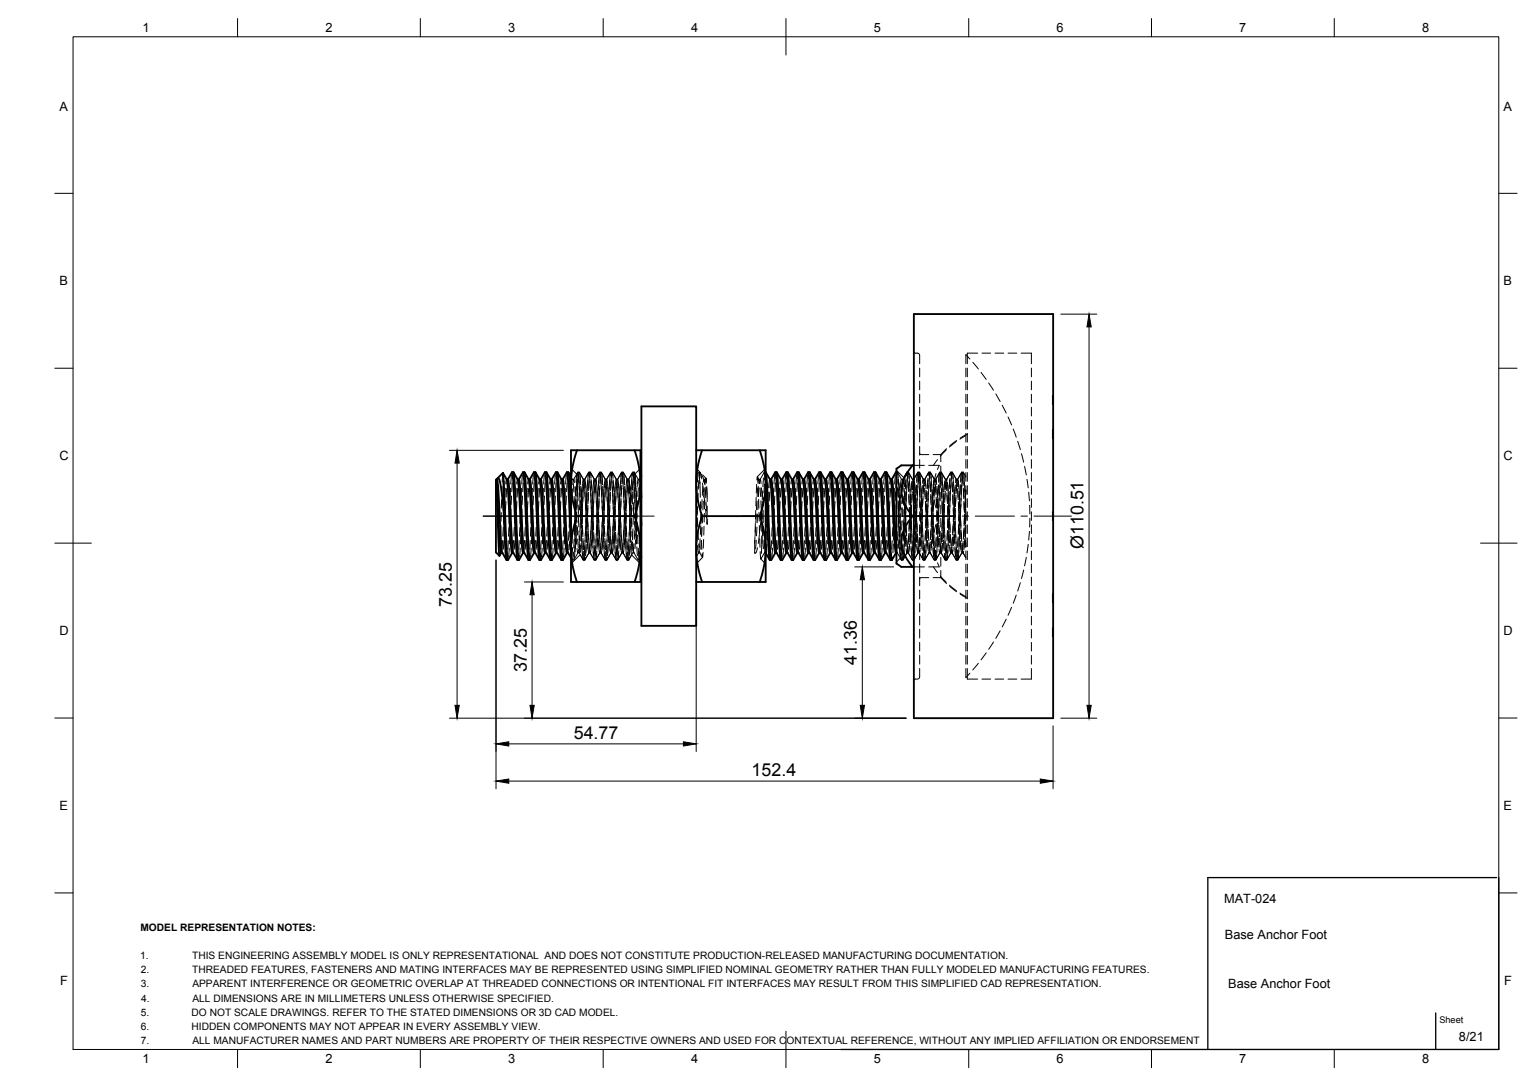
ISO-10303-21;
HEADER;
/* Generated by software containing ST-Developer
 * from STEP Tools, Inc. (www.steptools.com) 
 */

FILE_DESCRIPTION(
/* description */ ('STEP AP214'),
/* implementation_level */ '2;1');

FILE_NAME(
/* name */ 'Base Anchor Foot.step',
/* time_stamp */ '2026-11-14T06:34:07-08:00',
/* author */ (''),
/* organization */ (''),
/* preprocessor_version */ 'ST-DEVELOPER v20.2',
/* originating_system */ 'Autodesk Translation Framework v15.17.0.0',
/* authorisation */ '');

FILE_SCHEMA (('AUTOMOTIVE_DESIGN { 1 0 10303 214 3 1 1 }'));
ENDSEC;

DATA;
#10=MECHANICAL_DESIGN_GEOMETRIC_PRESENTATION_REPRESENTATION('',(#7314,#7315,#7316,#7317),#310623);
#11=ORIENTED_CLOSED_SHELL('',*,#93766,.F.);
#12=BREP_WITH_VOIDS('Body3',#93767,(#11));
#1065=SPHERICAL_SURFACE('',#104324,64.4688722290585);
#1066=SPHERICAL_SURFACE('',#104326,25.0876428025235);
#1067=SPHERICAL_SURFACE('',#104511,25.2860803025235);
#1539=(
BOUNDED_CURVE()
B_SPLINE_CURVE(2,(#275566,#275567,#275568),.UNSPECIFIED.,.F.,.F.)
B_SPLINE_CURVE_WITH_KNOTS((3,3),(0.701923076923077,0.701927534605613),
 .UNSPECIFIED.)
CURVE()
GEOMETRIC_REPRESENTATION_ITEM()
RATIONAL_B_SPLINE_CURVE((1.,0.99988654925346,0.999773624463427))
REPRESENTATION_ITEM('')
);
#1540=(
BOUNDED_CURVE()
B_SPLINE_CURVE(2,(#275574,#275575,#275576,#275577,#275578,#275579,#275580,
#275581,#275582,#275583,#275584,#275585,#275586,#275587,#275588,#275589,
#275590,#275591,#275592),.UNSPECIFIED.,.F.,.F.)
B_SPLINE_CURVE_WITH_KNOTS((3,2,2,2,2,2,2,2,2,3),(0.682692307692308,0.684615384615385,
0.686538461538462,0.688461538461538,0.690384615384615,0.692307692307692,
0.694230769230769,0.696153846153846,0.698076923076923,0.699514511997895),
 .UNSPECIFIED.)
CURVE()
GEOMETRIC_REPRESENTATION_ITEM()
RATIONAL_B_SPLINE_CURVE((1.,0.951056516295154,1.,0.951056516295154,1.,0.951056516295154,
1.,0.951056516295154,1.,0.951056516295154,1.,0.951056516295154,1.,0.951056516295154,
1.,0.951056516295154,1.,0.963412482837523,0.981526687366426))
REPRESENTATION_ITEM('')
);
#1541=(
BOUNDED_CURVE()
B_SPLINE_CURVE(2,(#275594,#275595,#275596,#275597,#275598,#275599,#275600,
#275601,#275602,#275603,#275604,#275605,#275606,#275607,#275608,#275609,
#275610,#275611,#275612,#275613,#275614),.UNSPECIFIED.,.F.,.F.)
B_SPLINE_CURVE_WITH_KNOTS((3,2,2,2,2,2,2,2,2,2,3),(0.682692307692308,0.684615384615385,
0.686538461538462,0.688461538461538,0.690384615384615,0.692307692307692,
0.694230769230769,0.696153846153846,0.698076923076923,0.7,0.701923076923077),
 .UNSPECIFIED.)
CURVE()
GEOMETRIC_REPRESENTATION_ITEM()
RATIONAL_B_SPLINE_CURVE((1.,0.951056516295154,1.,0.951056516295154,1.,0.951056516295154,
1.,0.951056516295154,1.,0.951056516295154,1.,0.951056516295154,1.,0.951056516295154,
1.,0.951056516295154,1.,0.951056516295154,1.,0.951056516295154,1.))
REPRESENTATION_ITEM('')
);
#1542=(
BOUNDED_CURVE()
B_SPLINE_CURVE(2,(#275619,#275620,#275621,#275622,#275623,#275624,#275625,
#275626,#275627,#275628,#275629,#275630,#275631,#275632,#275633,#275634,
#275635,#275636,#275637,#275638,#275639),.UNSPECIFIED.,.F.,.F.)
B_SPLINE_CURVE_WITH_KNOTS((3,2,2,2,2,2,2,2,2,2,3),(0.663461538461538,0.665384615384615,
0.667307692307692,0.669230769230769,0.671153846153846,0.673076923076923,
0.675,0.676923076923077,0.678846153846154,0.680769230769231,0.682692307692308),
 .UNSPECIFIED.)
CURVE()
GEOMETRIC_REPRESENTATION_ITEM()
RATIONAL_B_SPLINE_CURVE((1.,0.951056516295154,1.,0.951056516295154,1.,0.951056516295154,
1.,0.951056516295154,1.,0.951056516295154,1.,0.951056516295154,1.,0.951056516295154,
1.,0.951056516295154,1.,0.951056516295154,1.,0.951056516295154,1.))
REPRESENTATION_ITEM('')
);
#1543=(
BOUNDED_CURVE()
B_SPLINE_CURVE(2,(#275640,#275641,#275642,#275643,#275644,#275645,#275646,
#275647,#275648,#275649,#275650,#275651,#275652,#275653,#275654,#275655,
#275656,#275657,#275658,#275659,#275660),.UNSPECIFIED.,.F.,.F.)
B_SPLINE_CURVE_WITH_KNOTS((3,2,2,2,2,2,2,2,2,2,3),(0.663461538461538,0.665384615384615,
0.667307692307692,0.669230769230769,0.671153846153846,0.673076923076923,
0.675,0.676923076923077,0.678846153846154,0.680769230769231,0.682692307692308),
 .UNSPECIFIED.)
CURVE()
GEOMETRIC_REPRESENTATION_ITEM()
RATIONAL_B_SPLINE_CURVE((1.,0.951056516295154,1.,0.951056516295154,1.,0.951056516295154,
1.,0.951056516295154,1.,0.951056516295154,1.,0.951056516295154,1.,0.951056516295154,
1.,0.951056516295154,1.,0.951056516295154,1.,0.951056516295154,1.))
REPRESENTATION_ITEM('')
);
#1544=(
BOUNDED_CURVE()
B_SPLINE_CURVE(2,(#275665,#275666,#275667,#275668,#275669,#275670,#275671,
#275672,#275673,#275674,#275675,#275676,#275677,#275678,#275679,#275680,
#275681,#275682,#275683,#275684,#275685),.UNSPECIFIED.,.F.,.F.)
B_SPLINE_CURVE_WITH_KNOTS((3,2,2,2,2,2,2,2,2,2,3),(0.644230769230769,0.646153846153846,
0.648076923076923,0.65,0.651923076923077,0.653846153846154,0.655769230769231,
0.657692307692308,0.659615384615385,0.661538461538462,0.663461538461538),
 .UNSPECIFIED.)
CURVE()
GEOMETRIC_REPRESENTATION_ITEM()
RATIONAL_B_SPLINE_CURVE((1.,0.951056516295154,1.,0.951056516295154,1.,0.951056516295154,
1.,0.951056516295154,1.,0.951056516295154,1.,0.951056516295154,1.,0.951056516295154,
1.,0.951056516295154,1.,0.951056516295154,1.,0.951056516295154,1.))
REPRESENTATION_ITEM('')
);
#1545=(
BOUNDED_CURVE()
B_SPLINE_CURVE(2,(#275686,#275687,#275688,#275689,#275690,#275691,#275692,
#275693,#275694,#275695,#275696,#275697,#275698,#275699,#275700,#275701,
#275702,#275703,#275704,#275705,#275706),.UNSPECIFIED.,.F.,.F.)
B_SPLINE_CURVE_WITH_KNOTS((3,2,2,2,2,2,2,2,2,2,3),(0.644230769230769,0.646153846153846,
0.648076923076923,0.65,0.651923076923077,0.653846153846154,0.655769230769231,
0.657692307692308,0.659615384615385,0.661538461538462,0.663461538461538),
 .UNSPECIFIED.)
CURVE()
GEOMETRIC_REPRESENTATION_ITEM()
RATIONAL_B_SPLINE_CURVE((1.,0.951056516295154,1.,0.951056516295154,1.,0.951056516295154,
1.,0.951056516295154,1.,0.951056516295154,1.,0.951056516295154,1.,0.951056516295154,
1.,0.951056516295154,1.,0.951056516295154,1.,0.951056516295154,1.))
REPRESENTATION_ITEM('')
);
#1546=(
BOUNDED_CURVE()
B_SPLINE_CURVE(2,(#275712,#275713,#275714,#275715,#275716,#275717,#275718,
#275719,#275720),.UNSPECIFIED.,.F.,.F.)
B_SPLINE_CURVE_WITH_KNOTS((3,2,2,2,3),(0.618568719050757,0.619230769230769,
0.621153846153846,0.623076923076923,0.625),.UNSPECIFIED.)
CURVE()
GEOMETRIC_REPRESENTATION_ITEM()
RATIONAL_B_SPLINE_CURVE((0.977902315623412,0.983150418057436,1.,0.951056516295154,
1.,0.951056516295154,1.,0.951056516295154,1.))
REPRESENTATION_ITEM('')
);
#1547=(
BOUNDED_CURVE()
B_SPLINE_CURVE(2,(#275723,#275724,#275725,#275726,#275727,#275728,#275729,
#275730,#275731,#275732,#275733),.UNSPECIFIED.,.F.,.F.)
B_SPLINE_CURVE_WITH_KNOTS((3,2,2,2,2,3),(0.616175777003085,0.617307692307692,
0.619230769230769,0.621153846153846,0.623076923076923,0.625),
 .UNSPECIFIED.)
CURVE()
GEOMETRIC_REPRESENTATION_ITEM()
RATIONAL_B_SPLINE_CURVE((0.976296596823935,0.971192063301508,1.,0.951056516295154,
1.,0.951056516295154,1.,0.951056516295154,1.,0.951056516295154,1.))
REPRESENTATION_ITEM('')
);
#1548=(
BOUNDED_CURVE()
B_SPLINE_CURVE(2,(#276333,#276334,#276335),.UNSPECIFIED.,.F.,.F.)
B_SPLINE_CURVE_WITH_KNOTS((3,3),(-7.37746868484566,-5.33580039117808),
 .UNSPECIFIED.)
CURVE()
GEOMETRIC_REPRESENTATION_ITEM()
RATIONAL_B_SPLINE_CURVE((1.82136720504436,1.96225044864938,1.96225044864938))
REPRESENTATION_ITEM('')
);
#1549=(
BOUNDED_CURVE()
B_SPLINE_CURVE(2,(#276339,#276340,#276341),.UNSPECIFIED.,.F.,.F.)
B_SPLINE_CURVE_WITH_KNOTS((3,3),(3.29413209751051,5.33580039117807),
 .UNSPECIFIED.)
CURVE()
GEOMETRIC_REPRESENTATION_ITEM()
RATIONAL_B_SPLINE_CURVE((1.82136720504436,1.96225044864938,1.96225044864938))
REPRESENTATION_ITEM('')
);
#1550=(
BOUNDED_CURVE()
B_SPLINE_CURVE(2,(#276343,#276344,#276345),.UNSPECIFIED.,.F.,.F.)
B_SPLINE_CURVE_WITH_KNOTS((3,3),(5.33580039117807,7.37746868484567),
 .UNSPECIFIED.)
CURVE()
GEOMETRIC_REPRESENTATION_ITEM()
RATIONAL_B_SPLINE_CURVE((1.96225044864938,1.96225044864939,1.82136720504436))
REPRESENTATION_ITEM('')
);
#1551=(
BOUNDED_CURVE()
B_SPLINE_CURVE(2,(#276348,#276349,#276350),.UNSPECIFIED.,.F.,.F.)
B_SPLINE_CURVE_WITH_KNOTS((3,3),(-5.33580039117808,-3.2941320975105),
 .UNSPECIFIED.)
CURVE()
GEOMETRIC_REPRESENTATION_ITEM()
RATIONAL_B_SPLINE_CURVE((1.96225044864938,1.96225044864938,1.82136720504436))
REPRESENTATION_ITEM('')
);
#1552=(
BOUNDED_CURVE()
B_SPLINE_CURVE(2,(#276352,#276353,#276354),.UNSPECIFIED.,.F.,.F.)
B_SPLINE_CURVE_WITH_KNOTS((3,3),(-7.37746868484565,-5.33580039117808),
 .UNSPECIFIED.)
CURVE()
GEOMETRIC_REPRESENTATION_ITEM()
RATIONAL_B_SPLINE_CURVE((1.82136720504435,1.96225044864937,1.96225044864937))
REPRESENTATION_ITEM('')
);
#1553=(
BOUNDED_CURVE()
B_SPLINE_CURVE(2,(#276356,#276357,#276358),.UNSPECIFIED.,.F.,.F.)
B_SPLINE_CURVE_WITH_KNOTS((3,3),(3.29413209751051,5.33580039117807),
 .UNSPECIFIED.)
CURVE()
GEOMETRIC_REPRESENTATION_ITEM()
RATIONAL_B_SPLINE_CURVE((1.82136720504436,1.96225044864937,1.96225044864937))
REPRESENTATION_ITEM('')
);
#1554=(
BOUNDED_CURVE()
B_SPLINE_CURVE(2,(#276360,#276361,#276362),.UNSPECIFIED.,.F.,.F.)
B_SPLINE_CURVE_WITH_KNOTS((3,3),(5.33580039117807,7.37746868484565),
 .UNSPECIFIED.)
CURVE()
GEOMETRIC_REPRESENTATION_ITEM()
RATIONAL_B_SPLINE_CURVE((1.96225044864937,1.96225044864937,1.82136720504436))
REPRESENTATION_ITEM('')
);
#1555=(
BOUNDED_CURVE()
B_SPLINE_CURVE(2,(#276365,#276366,#276367),.UNSPECIFIED.,.F.,.F.)
B_SPLINE_CURVE_WITH_KNOTS((3,3),(-5.33580039117808,-3.29413209751051),
 .UNSPECIFIED.)
CURVE()
GEOMETRIC_REPRESENTATION_ITEM()
RATIONAL_B_SPLINE_CURVE((1.96225044864937,1.96225044864937,1.82136720504436))
REPRESENTATION_ITEM('')
);
#1556=(
BOUNDED_CURVE()
B_SPLINE_CURVE(2,(#276369,#276370,#276371),.UNSPECIFIED.,.F.,.F.)
B_SPLINE_CURVE_WITH_KNOTS((3,3),(-7.37746868484568,-5.33580039117808),
 .UNSPECIFIED.)
CURVE()
GEOMETRIC_REPRESENTATION_ITEM()
RATIONAL_B_SPLINE_CURVE((1.82136720504436,1.96225044864938,1.96225044864938))
REPRESENTATION_ITEM('')
);
#1557=(
BOUNDED_CURVE()
B_SPLINE_CURVE(2,(#276373,#276374,#276375),.UNSPECIFIED.,.F.,.F.)
B_SPLINE_CURVE_WITH_KNOTS((3,3),(3.29413209751049,5.3358003911781),
 .UNSPECIFIED.)
CURVE()
GEOMETRIC_REPRESENTATION_ITEM()
RATIONAL_B_SPLINE_CURVE((1.82136720504436,1.96225044864939,1.96225044864938))
REPRESENTATION_ITEM('')
);
#1558=(
BOUNDED_CURVE()
B_SPLINE_CURVE(2,(#276377,#276378,#276379),.UNSPECIFIED.,.F.,.F.)
B_SPLINE_CURVE_WITH_KNOTS((3,3),(5.3358003911781,7.37746868484565),
 .UNSPECIFIED.)
CURVE()
GEOMETRIC_REPRESENTATION_ITEM()
RATIONAL_B_SPLINE_CURVE((1.96225044864938,1.96225044864938,1.82136720504436))
REPRESENTATION_ITEM('')
);
#1559=(
BOUNDED_CURVE()
B_SPLINE_CURVE(2,(#276382,#276383,#276384),.UNSPECIFIED.,.F.,.F.)
B_SPLINE_CURVE_WITH_KNOTS((3,3),(-5.33580039117808,-3.29413209751051),
 .UNSPECIFIED.)
CURVE()
GEOMETRIC_REPRESENTATION_ITEM()
RATIONAL_B_SPLINE_CURVE((1.96225044864938,1.96225044864938,1.82136720504436))
REPRESENTATION_ITEM('')
);
#1560=(
BOUNDED_CURVE()
B_SPLINE_CURVE(2,(#276386,#276387,#276388),.UNSPECIFIED.,.F.,.F.)
B_SPLINE_CURVE_WITH_KNOTS((3,3),(-7.37746868484567,-5.33580039117808),
 .UNSPECIFIED.)
CURVE()
GEOMETRIC_REPRESENTATION_ITEM()
RATIONAL_B_SPLINE_CURVE((1.82136720504436,1.96225044864938,1.96225044864938))
REPRESENTATION_ITEM('')
);
#1561=(
BOUNDED_CURVE()
B_SPLINE_CURVE(2,(#276390,#276391,#276392),.UNSPECIFIED.,.F.,.F.)
B_SPLINE_CURVE_WITH_KNOTS((3,3),(3.29413209751051,5.33580039117811),
 .UNSPECIFIED.)
CURVE()
GEOMETRIC_REPRESENTATION_ITEM()
RATIONAL_B_SPLINE_CURVE((1.82136720504437,1.96225044864939,1.96225044864939))
REPRESENTATION_ITEM('')
);
#1562=(
BOUNDED_CURVE()
B_SPLINE_CURVE(2,(#276394,#276395,#276396),.UNSPECIFIED.,.F.,.F.)
B_SPLINE_CURVE_WITH_KNOTS((3,3),(5.33580039117811,7.37746868484567),
 .UNSPECIFIED.)
CURVE()
GEOMETRIC_REPRESENTATION_ITEM()
RATIONAL_B_SPLINE_CURVE((1.96225044864939,1.96225044864939,1.82136720504437))
REPRESENTATION_ITEM('')
);
#1563=(
BOUNDED_CURVE()
B_SPLINE_CURVE(2,(#276399,#276400,#276401),.UNSPECIFIED.,.F.,.F.)
B_SPLINE_CURVE_WITH_KNOTS((3,3),(-5.3358003911781,-3.29413209751052),
 .UNSPECIFIED.)
CURVE()
GEOMETRIC_REPRESENTATION_ITEM()
RATIONAL_B_SPLINE_CURVE((1.96225044864939,1.96225044864939,1.82136720504437))
REPRESENTATION_ITEM('')
);
#1564=(
BOUNDED_CURVE()
B_SPLINE_CURVE(2,(#276403,#276404,#276405),.UNSPECIFIED.,.F.,.F.)
B_SPLINE_CURVE_WITH_KNOTS((3,3),(-7.37746868484567,-5.33580039117809),
 .UNSPECIFIED.)
CURVE()
GEOMETRIC_REPRESENTATION_ITEM()
RATIONAL_B_SPLINE_CURVE((1.82136720504437,1.96225044864939,1.96225044864939))
REPRESENTATION_ITEM('')
);
#1565=(
BOUNDED_CURVE()
B_SPLINE_CURVE(2,(#276407,#276408,#276409),.UNSPECIFIED.,.F.,.F.)
B_SPLINE_CURVE_WITH_KNOTS((3,3),(3.29413209751051,5.33580039117809),
 .UNSPECIFIED.)
CURVE()
GEOMETRIC_REPRESENTATION_ITEM()
RATIONAL_B_SPLINE_CURVE((1.82136720504437,1.96225044864939,1.96225044864939))
REPRESENTATION_ITEM('')
);
#1566=(
BOUNDED_CURVE()
B_SPLINE_CURVE(2,(#276411,#276412,#276413),.UNSPECIFIED.,.F.,.F.)
B_SPLINE_CURVE_WITH_KNOTS((3,3),(5.33580039117809,7.37746868484569),
 .UNSPECIFIED.)
CURVE()
GEOMETRIC_REPRESENTATION_ITEM()
RATIONAL_B_SPLINE_CURVE((1.96225044864939,1.96225044864939,1.82136720504436))
REPRESENTATION_ITEM('')
);
#1567=(
BOUNDED_CURVE()
B_SPLINE_CURVE(2,(#276416,#276417,#276418),.UNSPECIFIED.,.F.,.F.)
B_SPLINE_CURVE_WITH_KNOTS((3,3),(-5.33580039117809,-3.29413209751051),
 .UNSPECIFIED.)
CURVE()
GEOMETRIC_REPRESENTATION_ITEM()
RATIONAL_B_SPLINE_CURVE((1.96225044864939,1.96225044864939,1.82136720504436))
REPRESENTATION_ITEM('')
);
#1568=(
BOUNDED_CURVE()
B_SPLINE_CURVE(2,(#276420,#276421,#276422),.UNSPECIFIED.,.F.,.F.)
B_SPLINE_CURVE_WITH_KNOTS((3,3),(-7.37746868484564,-5.33580039117808),
 .UNSPECIFIED.)
CURVE()
GEOMETRIC_REPRESENTATION_ITEM()
RATIONAL_B_SPLINE_CURVE((1.82136720504437,1.96225044864938,1.96225044864938))
REPRESENTATION_ITEM('')
);
#1569=(
BOUNDED_CURVE()
B_SPLINE_CURVE(2,(#276424,#276425,#276426),.UNSPECIFIED.,.F.,.F.)
B_SPLINE_CURVE_WITH_KNOTS((3,3),(3.29413209751051,5.3358003911781),
 .UNSPECIFIED.)
CURVE()
GEOMETRIC_REPRESENTATION_ITEM()
RATIONAL_B_SPLINE_CURVE((1.82136720504436,1.96225044864939,1.96225044864938))
REPRESENTATION_ITEM('')
);
#1570=(
BOUNDED_CURVE()
B_SPLINE_CURVE(2,(#276427,#276428,#276429),.UNSPECIFIED.,.F.,.F.)
B_SPLINE_CURVE_WITH_KNOTS((3,3),(5.3358003911781,7.37746868484565),
 .UNSPECIFIED.)
CURVE()
GEOMETRIC_REPRESENTATION_ITEM()
RATIONAL_B_SPLINE_CURVE((1.96225044864938,1.96225044864938,1.82136720504436))
REPRESENTATION_ITEM('')
);
#1571=(
BOUNDED_CURVE()
B_SPLINE_CURVE(2,(#276430,#276431,#276432),.UNSPECIFIED.,.F.,.F.)
B_SPLINE_CURVE_WITH_KNOTS((3,3),(-5.33580039117809,-3.2941320975105),
 .UNSPECIFIED.)
CURVE()
GEOMETRIC_REPRESENTATION_ITEM()
RATIONAL_B_SPLINE_CURVE((1.96225044864938,1.96225044864938,1.82136720504436))
REPRESENTATION_ITEM('')
);
#1572=(
BOUNDED_CURVE()
B_SPLINE_CURVE(2,(#278526,#278527,#278528,#278529,#278530,#278531,#278532,
#278533,#278534,#278535,#278536,#278537,#278538,#278539,#278540,#278541,
#278542,#278543,#278544,#278545,#278546),.UNSPECIFIED.,.F.,.F.)
B_SPLINE_CURVE_WITH_KNOTS((3,2,2,2,2,2,2,2,2,2,3),(0.625,0.626923076923077,
0.628846153846154,0.630769230769231,0.632692307692308,0.634615384615385,
0.636538461538461,0.638461538461538,0.640384615384615,0.642307692307692,
0.644230769230769),.UNSPECIFIED.)
CURVE()
GEOMETRIC_REPRESENTATION_ITEM()
RATIONAL_B_SPLINE_CURVE((1.,0.951056516295154,1.,0.951056516295154,1.,0.951056516295154,
1.,0.951056516295154,1.,0.951056516295154,1.,0.951056516295154,1.,0.951056516295154,
1.,0.951056516295154,1.,0.951056516295154,1.,0.951056516295154,1.))
REPRESENTATION_ITEM('')
);
#1573=(
BOUNDED_CURVE()
B_SPLINE_CURVE(2,(#280621,#280622,#280623,#280624,#280625,#280626,#280627,
#280628,#280629,#280630,#280631,#280632,#280633,#280634,#280635,#280636,
#280637,#280638,#280639,#280640,#280641),.UNSPECIFIED.,.F.,.F.)
B_SPLINE_CURVE_WITH_KNOTS((3,2,2,2,2,2,2,2,2,2,3),(0.625,0.626923076923077,
0.628846153846154,0.630769230769231,0.632692307692308,0.634615384615385,
0.636538461538461,0.638461538461538,0.640384615384615,0.642307692307692,
0.644230769230769),.UNSPECIFIED.)
CURVE()
GEOMETRIC_REPRESENTATION_ITEM()
RATIONAL_B_SPLINE_CURVE((1.,0.951056516295154,1.,0.951056516295154,1.,0.951056516295154,
1.,0.951056516295154,1.,0.951056516295154,1.,0.951056516295154,1.,0.951056516295154,
1.,0.951056516295154,1.,0.951056516295154,1.,0.951056516295154,1.))
REPRESENTATION_ITEM('')
);
#1574=(
BOUNDED_CURVE()
B_SPLINE_CURVE(2,(#280648,#280649,#280650,#280651,#280652,#280653,#280654,
#280655,#280656),.UNSPECIFIED.,.F.,.F.)
B_SPLINE_CURVE_WITH_KNOTS((3,2,2,2,3),(0.125,0.126923076923077,0.128846153846154,
0.130769230769231,0.132372212319224),.UNSPECIFIED.)
CURVE()
GEOMETRIC_REPRESENTATION_ITEM()
RATIONAL_B_SPLINE_CURVE((1.,0.951056516295154,1.,0.951056516295154,1.,0.951056516295154,
1.,0.959203139286952,0.986418758195375))
REPRESENTATION_ITEM('')
);
#1575=(
BOUNDED_CURVE()
B_SPLINE_CURVE(2,(#280659,#280660,#280661,#280662,#280663,#280664,#280665,
#280666,#280667,#280668,#280669,#280670,#280671),.UNSPECIFIED.,.F.,.F.)
B_SPLINE_CURVE_WITH_KNOTS((3,2,2,2,2,2,3),(0.125,0.126923076923077,0.128846153846154,
0.130769230769231,0.132692307692308,0.134615384615385,0.134791334496805),
 .UNSPECIFIED.)
CURVE()
GEOMETRIC_REPRESENTATION_ITEM()
RATIONAL_B_SPLINE_CURVE((1.,0.951056516295154,1.,0.951056516295154,1.,0.951056516295154,
1.,0.951056516295154,1.,0.951056516295154,1.,0.99552196791982,0.991863361421687))
REPRESENTATION_ITEM('')
);
#1576=(
BOUNDED_CURVE()
B_SPLINE_CURVE(2,(#280676,#280677,#280678,#280679,#280680,#280681,#280682,
#280683,#280684,#280685,#280686,#280687,#280688,#280689,#280690,#280691,
#280692,#280693,#280694,#280695,#280696),.UNSPECIFIED.,.F.,.F.)
B_SPLINE_CURVE_WITH_KNOTS((3,2,2,2,2,2,2,2,2,2,3),(0.105769230769231,0.107692307692308,
0.109615384615385,0.111538461538462,0.113461538461538,0.115384615384615,
0.117307692307692,0.119230769230769,0.121153846153846,0.123076923076923,
0.125),.UNSPECIFIED.)
CURVE()
GEOMETRIC_REPRESENTATION_ITEM()
RATIONAL_B_SPLINE_CURVE((1.,0.951056516295154,1.,0.951056516295154,1.,0.951056516295154,
1.,0.951056516295154,1.,0.951056516295154,1.,0.951056516295154,1.,0.951056516295154,
1.,0.951056516295154,1.,0.951056516295154,1.,0.951056516295154,1.))
REPRESENTATION_ITEM('')
);
#1577=(
BOUNDED_CURVE()
B_SPLINE_CURVE(2,(#280697,#280698,#280699,#280700,#280701,#280702,#280703,
#280704,#280705,#280706,#280707,#280708,#280709,#280710,#280711,#280712,
#280713,#280714,#280715,#280716,#280717),.UNSPECIFIED.,.F.,.F.)
B_SPLINE_CURVE_WITH_KNOTS((3,2,2,2,2,2,2,2,2,2,3),(0.105769230769231,0.107692307692308,
0.109615384615385,0.111538461538462,0.113461538461538,0.115384615384615,
0.117307692307692,0.119230769230769,0.121153846153846,0.123076923076923,
0.125),.UNSPECIFIED.)
CURVE()
GEOMETRIC_REPRESENTATION_ITEM()
RATIONAL_B_SPLINE_CURVE((1.,0.951056516295154,1.,0.951056516295154,1.,0.951056516295154,
1.,0.951056516295154,1.,0.951056516295154,1.,0.951056516295154,1.,0.951056516295154,
1.,0.951056516295154,1.,0.951056516295154,1.,0.951056516295154,1.))
REPRESENTATION_ITEM('')
);
#1578=(
BOUNDED_CURVE()
B_SPLINE_CURVE(2,(#280722,#280723,#280724,#280725,#280726,#280727,#280728,
#280729,#280730,#280731,#280732,#280733,#280734,#280735,#280736,#280737,
#280738,#280739,#280740,#280741,#280742),.UNSPECIFIED.,.F.,.F.)
B_SPLINE_CURVE_WITH_KNOTS((3,2,2,2,2,2,2,2,2,2,3),(0.0865384615384615,0.0884615384615385,
0.0903846153846154,0.0923076923076923,0.0942307692307692,0.0961538461538462,
0.0980769230769231,0.1,0.101923076923077,0.103846153846154,0.105769230769231),
 .UNSPECIFIED.)
CURVE()
GEOMETRIC_REPRESENTATION_ITEM()
RATIONAL_B_SPLINE_CURVE((1.,0.951056516295154,1.,0.951056516295154,1.,0.951056516295154,
1.,0.951056516295154,1.,0.951056516295154,1.,0.951056516295154,1.,0.951056516295154,
1.,0.951056516295154,1.,0.951056516295154,1.,0.951056516295154,1.))
REPRESENTATION_ITEM('')
);
#1579=(
BOUNDED_CURVE()
B_SPLINE_CURVE(2,(#280743,#280744,#280745,#280746,#280747,#280748,#280749,
#280750,#280751,#280752,#280753,#280754,#280755,#280756,#280757,#280758,
#280759,#280760,#280761,#280762,#280763),.UNSPECIFIED.,.F.,.F.)
B_SPLINE_CURVE_WITH_KNOTS((3,2,2,2,2,2,2,2,2,2,3),(0.0865384615384615,0.0884615384615385,
0.0903846153846154,0.0923076923076923,0.0942307692307692,0.0961538461538462,
0.0980769230769231,0.1,0.101923076923077,0.103846153846154,0.105769230769231),
 .UNSPECIFIED.)
CURVE()
GEOMETRIC_REPRESENTATION_ITEM()
RATIONAL_B_SPLINE_CURVE((1.,0.951056516295154,1.,0.951056516295154,1.,0.951056516295154,
1.,0.951056516295154,1.,0.951056516295154,1.,0.951056516295154,1.,0.951056516295154,
1.,0.951056516295154,1.,0.951056516295154,1.,0.951056516295154,1.))
REPRESENTATION_ITEM('')
);
#1580=(
BOUNDED_CURVE()
B_SPLINE_CURVE(2,(#280768,#280769,#280770,#280771,#280772,#280773,#280774,
#280775,#280776,#280777,#280778,#280779,#280780,#280781,#280782,#280783,
#280784,#280785,#280786,#280787,#280788),.UNSPECIFIED.,.F.,.F.)
B_SPLINE_CURVE_WITH_KNOTS((3,2,2,2,2,2,2,2,2,2,3),(0.0673076923076923,0.0692307692307692,
0.0711538461538461,0.0730769230769231,0.075,0.0769230769230769,0.0788461538461538,
0.0807692307692308,0.0826923076923077,0.0846153846153846,0.0865384615384615),
 .UNSPECIFIED.)
CURVE()
GEOMETRIC_REPRESENTATION_ITEM()
RATIONAL_B_SPLINE_CURVE((1.,0.951056516295154,1.,0.951056516295154,1.,0.951056516295154,
1.,0.951056516295154,1.,0.951056516295154,1.,0.951056516295154,1.,0.951056516295154,
1.,0.951056516295154,1.,0.951056516295154,1.,0.951056516295154,1.))
REPRESENTATION_ITEM('')
);
#1581=(
BOUNDED_CURVE()
B_SPLINE_CURVE(2,(#280789,#280790,#280791,#280792,#280793,#280794,#280795,
#280796,#280797,#280798,#280799,#280800,#280801,#280802,#280803,#280804,
#280805,#280806,#280807,#280808,#280809),.UNSPECIFIED.,.F.,.F.)
B_SPLINE_CURVE_WITH_KNOTS((3,2,2,2,2,2,2,2,2,2,3),(0.0673076923076923,0.0692307692307692,
0.0711538461538462,0.0730769230769231,0.075,0.0769230769230769,0.0788461538461538,
0.0807692307692308,0.0826923076923077,0.0846153846153846,0.0865384615384615),
 .UNSPECIFIED.)
CURVE()
GEOMETRIC_REPRESENTATION_ITEM()
RATIONAL_B_SPLINE_CURVE((1.,0.951056516295154,1.,0.951056516295154,1.,0.951056516295154,
1.,0.951056516295154,1.,0.951056516295154,1.,0.951056516295154,1.,0.951056516295154,
1.,0.951056516295154,1.,0.951056516295154,1.,0.951056516295154,1.))
REPRESENTATION_ITEM('')
);
#1582=(
BOUNDED_CURVE()
B_SPLINE_CURVE(2,(#280814,#280815,#280816,#280817,#280818,#280819,#280820,
#280821,#280822,#280823,#280824,#280825,#280826,#280827,#280828,#280829,
#280830,#280831,#280832,#280833,#280834),.UNSPECIFIED.,.F.,.F.)
B_SPLINE_CURVE_WITH_KNOTS((3,2,2,2,2,2,2,2,2,2,3),(0.0480769230769231,0.05,
0.0519230769230769,0.0538461538461538,0.0557692307692308,0.0576923076923077,
0.0596153846153846,0.0615384615384615,0.0634615384615385,0.0653846153846154,
0.0673076923076923),.UNSPECIFIED.)
CURVE()
GEOMETRIC_REPRESENTATION_ITEM()
RATIONAL_B_SPLINE_CURVE((1.,0.951056516295154,1.,0.951056516295154,1.,0.951056516295154,
1.,0.951056516295154,1.,0.951056516295154,1.,0.951056516295154,1.,0.951056516295154,
1.,0.951056516295154,1.,0.951056516295154,1.,0.951056516295154,1.))
REPRESENTATION_ITEM('')
);
#1583=(
BOUNDED_CURVE()
B_SPLINE_CURVE(2,(#280835,#280836,#280837,#280838,#280839,#280840,#280841,
#280842,#280843,#280844,#280845,#280846,#280847,#280848,#280849,#280850,
#280851,#280852,#280853,#280854,#280855),.UNSPECIFIED.,.F.,.F.)
B_SPLINE_CURVE_WITH_KNOTS((3,2,2,2,2,2,2,2,2,2,3),(0.0480769230769231,0.05,
0.0519230769230769,0.0538461538461538,0.0557692307692308,0.0576923076923077,
0.0596153846153846,0.0615384615384615,0.0634615384615385,0.0653846153846154,
0.0673076923076923),.UNSPECIFIED.)
CURVE()
GEOMETRIC_REPRESENTATION_ITEM()
RATIONAL_B_SPLINE_CURVE((1.,0.951056516295154,1.,0.951056516295154,1.,0.951056516295154,
1.,0.951056516295154,1.,0.951056516295154,1.,0.951056516295154,1.,0.951056516295154,
1.,0.951056516295154,1.,0.951056516295154,1.,0.951056516295154,1.))
REPRESENTATION_ITEM('')
);
#1584=(
BOUNDED_CURVE()
B_SPLINE_CURVE(2,(#280862,#280863,#280864,#280865,#280866),
 .UNSPECIFIED.,.F.,.F.)
B_SPLINE_CURVE_WITH_KNOTS((3,2,3),(0.0264333754686713,0.0269230769230769,
0.0288461538461538),.UNSPECIFIED.)
CURVE()
GEOMETRIC_REPRESENTATION_ITEM()
RATIONAL_B_SPLINE_CURVE((0.981420974846885,0.987536798519951,1.,0.951056516295154,
1.))
REPRESENTATION_ITEM('')
);
#1585=(
BOUNDED_CURVE()
B_SPLINE_CURVE(2,(#281378,#281379,#281380),.UNSPECIFIED.,.F.,.F.)
B_SPLINE_CURVE_WITH_KNOTS((3,3),(-3.18750279702086,-0.878323675844115),
 .UNSPECIFIED.)
CURVE()
GEOMETRIC_REPRESENTATION_ITEM()
RATIONAL_B_SPLINE_CURVE((1.1939543172175,1.37865969289105,1.1939543172175))
REPRESENTATION_ITEM('')
);
#1586=(
BOUNDED_CURVE()
B_SPLINE_CURVE(2,(#281382,#281383,#281384),.UNSPECIFIED.,.F.,.F.)
B_SPLINE_CURVE_WITH_KNOTS((3,3),(0.878323675844114,3.18750279702085),
 .UNSPECIFIED.)
CURVE()
GEOMETRIC_REPRESENTATION_ITEM()
RATIONAL_B_SPLINE_CURVE((1.1939543172175,1.37865969289105,1.1939543172175))
REPRESENTATION_ITEM('')
);
#1587=(
BOUNDED_CURVE()
B_SPLINE_CURVE(2,(#281386,#281387,#281388),.UNSPECIFIED.,.F.,.F.)
B_SPLINE_CURVE_WITH_KNOTS((3,3),(0.878323675844118,3.18750279702086),
 .UNSPECIFIED.)
CURVE()
GEOMETRIC_REPRESENTATION_ITEM()
RATIONAL_B_SPLINE_CURVE((1.1939543172175,1.37865969289105,1.1939543172175))
REPRESENTATION_ITEM('')
);
#1588=(
BOUNDED_CURVE()
B_SPLINE_CURVE(2,(#281390,#281391,#281392),.UNSPECIFIED.,.F.,.F.)
B_SPLINE_CURVE_WITH_KNOTS((3,3),(0.878323675844117,2.03291323643249),
 .UNSPECIFIED.)
CURVE()
GEOMETRIC_REPRESENTATION_ITEM()
RATIONAL_B_SPLINE_CURVE((1.1939543172175,1.28630700505428,1.28630700505428))
REPRESENTATION_ITEM('')
);
#1589=(
BOUNDED_CURVE()
B_SPLINE_CURVE(2,(#281397,#281398,#281399),.UNSPECIFIED.,.F.,.F.)
B_SPLINE_CURVE_WITH_KNOTS((3,3),(2.03291323643249,3.18750279702086),
 .UNSPECIFIED.)
CURVE()
GEOMETRIC_REPRESENTATION_ITEM()
RATIONAL_B_SPLINE_CURVE((1.28630700505428,1.28630700505428,1.1939543172175))
REPRESENTATION_ITEM('')
);
#1590=(
BOUNDED_CURVE()
B_SPLINE_CURVE(2,(#281401,#281402,#281403),.UNSPECIFIED.,.F.,.F.)
B_SPLINE_CURVE_WITH_KNOTS((3,3),(-3.18750279702086,-0.878323675844113),
 .UNSPECIFIED.)
CURVE()
GEOMETRIC_REPRESENTATION_ITEM()
RATIONAL_B_SPLINE_CURVE((1.1939543172175,1.37865969289105,1.1939543172175))
REPRESENTATION_ITEM('')
);
#1591=(
BOUNDED_CURVE()
B_SPLINE_CURVE(2,(#281404,#281405,#281406),.UNSPECIFIED.,.F.,.F.)
B_SPLINE_CURVE_WITH_KNOTS((3,3),(-3.18750279702087,-0.878323675844119),
 .UNSPECIFIED.)
CURVE()
GEOMETRIC_REPRESENTATION_ITEM()
RATIONAL_B_SPLINE_CURVE((1.1939543172175,1.37865969289105,1.1939543172175))
REPRESENTATION_ITEM('')
);
#1592=(
BOUNDED_CURVE()
B_SPLINE_CURVE(2,(#283589,#283590,#283591,#283592,#283593,#283594,#283595,
#283596,#283597,#283598,#283599,#283600,#283601,#283602,#283603,#283604,
#283605,#283606,#283607,#283608,#283609),.UNSPECIFIED.,.F.,.F.)
B_SPLINE_CURVE_WITH_KNOTS((3,2,2,2,2,2,2,2,2,2,3),(0.0288461538461538,0.0307692307692308,
0.0326923076923077,0.0346153846153846,0.0365384615384615,0.0384615384615385,
0.0403846153846154,0.0423076923076923,0.0442307692307692,0.0461538461538462,
0.0480769230769231),.UNSPECIFIED.)
CURVE()
GEOMETRIC_REPRESENTATION_ITEM()
RATIONAL_B_SPLINE_CURVE((1.,0.951056516295154,1.,0.951056516295154,1.,0.951056516295154,
1.,0.951056516295154,1.,0.951056516295154,1.,0.951056516295154,1.,0.951056516295154,
1.,0.951056516295154,1.,0.951056516295154,1.,0.951056516295154,1.))
REPRESENTATION_ITEM('')
);
#1593=(
BOUNDED_CURVE()
B_SPLINE_CURVE(2,(#285684,#285685,#285686,#285687,#285688,#285689,#285690,
#285691,#285692,#285693,#285694,#285695,#285696,#285697,#285698,#285699,
#285700,#285701,#285702,#285703,#285704),.UNSPECIFIED.,.F.,.F.)
B_SPLINE_CURVE_WITH_KNOTS((3,2,2,2,2,2,2,2,2,2,3),(0.0288461538461538,0.0307692307692308,
0.0326923076923077,0.0346153846153846,0.0365384615384615,0.0384615384615385,
0.0403846153846154,0.0423076923076923,0.0442307692307692,0.0461538461538462,
0.0480769230769231),.UNSPECIFIED.)
CURVE()
GEOMETRIC_REPRESENTATION_ITEM()
RATIONAL_B_SPLINE_CURVE((1.,0.951056516295154,1.,0.951056516295154,1.,0.951056516295154,
1.,0.951056516295154,1.,0.951056516295154,1.,0.951056516295154,1.,0.951056516295154,
1.,0.951056516295154,1.,0.951056516295154,1.,0.951056516295154,1.))
REPRESENTATION_ITEM('')
);
#1594=(
BOUNDED_CURVE()
B_SPLINE_CURVE(2,(#285711,#285712,#285713,#285714,#285715,#285716,#285717,
#285718,#285719,#285720,#285721,#285722,#285723),.UNSPECIFIED.,.F.,.F.)
B_SPLINE_CURVE_WITH_KNOTS((3,2,2,2,2,2,3),(0.480090915688519,0.480769230769231,
0.482692307692308,0.484615384615385,0.486538461538462,0.488461538461538,
0.490384615384615),.UNSPECIFIED.)
CURVE()
GEOMETRIC_REPRESENTATION_ITEM()
RATIONAL_B_SPLINE_CURVE((0.977651452579507,0.982736466388236,1.,0.951056516295154,
1.,0.951056516295154,1.,0.951056516295154,1.,0.951056516295154,1.,0.951056516295154,
1.))
REPRESENTATION_ITEM('')
);
#1595=(
BOUNDED_CURVE()
B_SPLINE_CURVE(2,(#285726,#285727,#285728,#285729,#285730,#285731,#285732,
#285733,#285734,#285735,#285736),.UNSPECIFIED.,.F.,.F.)
B_SPLINE_CURVE_WITH_KNOTS((3,2,2,2,2,3),(0.482494269360453,0.482692307692308,
0.484615384615385,0.486538461538462,0.488461538461538,0.490384615384615),
 .UNSPECIFIED.)
CURVE()
GEOMETRIC_REPRESENTATION_ITEM()
RATIONAL_B_SPLINE_CURVE((0.990957684919766,0.994959803348612,1.,0.951056516295154,
1.,0.951056516295154,1.,0.951056516295154,1.,0.951056516295154,1.))
REPRESENTATION_ITEM('')
);
#1596=(
BOUNDED_CURVE()
B_SPLINE_CURVE(2,(#285805,#285806,#285807,#285808,#285809,#285810,#285811,
#285812,#285813),.UNSPECIFIED.,.F.,.F.)
B_SPLINE_CURVE_WITH_KNOTS((3,2,2,2,3),(0.48722585646854,0.488461538461539,
0.490384615384615,0.492307692307692,0.493941807988044),.UNSPECIFIED.)
CURVE()
GEOMETRIC_REPRESENTATION_ITEM()
RATIONAL_B_SPLINE_CURVE((0.97751749990519,0.968551137625873,1.,0.951056516295154,
1.,0.951056516295154,1.,0.958410756629963,0.987501613373882))
REPRESENTATION_ITEM('')
);
#1597=(
BOUNDED_CURVE()
B_SPLINE_CURVE(2,(#287903,#287904,#287905,#287906,#287907,#287908,#287909,
#287910,#287911,#287912,#287913),.UNSPECIFIED.,.F.,.F.)
B_SPLINE_CURVE_WITH_KNOTS((3,2,2,2,2,3),(0.490384615384615,0.492307692307692,
0.494230769230769,0.496153846153846,0.498076923076923,0.499312605069927),
 .UNSPECIFIED.)
CURVE()
GEOMETRIC_REPRESENTATION_ITEM()
RATIONAL_B_SPLINE_CURVE((1.,0.951056516295154,1.,0.951056516295154,1.,0.951056516295154,
1.,0.951056516295154,1.,0.968551137625747,0.977517499905262))
REPRESENTATION_ITEM('')
);
#1598=(
BOUNDED_CURVE()
B_SPLINE_CURVE(2,(#290023,#290024,#290025,#290026,#290027,#290028,#290029,
#290030,#290031,#290032,#290033,#290034,#290035),.UNSPECIFIED.,.F.,.F.)
B_SPLINE_CURVE_WITH_KNOTS((3,2,2,2,2,2,3),(0.490384615384615,0.492307692307692,
0.494230769230769,0.496153846153846,0.498076923076923,0.5,0.501715584159741),
 .UNSPECIFIED.)
CURVE()
GEOMETRIC_REPRESENTATION_ITEM()
RATIONAL_B_SPLINE_CURVE((1.,0.951056516295154,1.,0.951056516295154,1.,0.951056516295154,
1.,0.951056516295154,1.,0.951056516295154,1.,0.956337334009382,0.99057792529015))
REPRESENTATION_ITEM('')
);
#1599=(
BOUNDED_CURVE()
B_SPLINE_CURVE(2,(#290044,#290045,#290046,#290047,#290048),
 .UNSPECIFIED.,.F.,.F.)
B_SPLINE_CURVE_WITH_KNOTS((3,2,3),(0.0264333754686713,0.0269230769230769,
0.0288461538461538),.UNSPECIFIED.)
CURVE()
GEOMETRIC_REPRESENTATION_ITEM()
RATIONAL_B_SPLINE_CURVE((0.981420974846885,0.987536798519951,1.,0.951056516295154,
1.))
REPRESENTATION_ITEM('')
);
#1600=(
BOUNDED_CURVE()
B_SPLINE_CURVE(2,(#290054,#290055,#290056,#290057,#290058,#290059,#290060,
#290061,#290062,#290063,#290064,#290065,#290066,#290067,#290068,#290069,
#290070,#290071,#290072,#290073,#290074),.UNSPECIFIED.,.F.,.F.)
B_SPLINE_CURVE_WITH_KNOTS((3,2,2,2,2,2,2,2,2,2,3),(0.0288461538461538,0.0307692307692308,
0.0326923076923077,0.0346153846153846,0.0365384615384615,0.0384615384615385,
0.0403846153846154,0.0423076923076923,0.0442307692307692,0.0461538461538462,
0.0480769230769231),.UNSPECIFIED.)
CURVE()
GEOMETRIC_REPRESENTATION_ITEM()
RATIONAL_B_SPLINE_CURVE((1.,0.951056516295154,1.,0.951056516295154,1.,0.951056516295154,
1.,0.951056516295154,1.,0.951056516295154,1.,0.951056516295154,1.,0.951056516295154,
1.,0.951056516295154,1.,0.951056516295154,1.,0.951056516295154,1.))
REPRESENTATION_ITEM('')
);
#1601=(
BOUNDED_CURVE()
B_SPLINE_CURVE(2,(#290075,#290076,#290077,#290078,#290079,#290080,#290081,
#290082,#290083,#290084,#290085,#290086,#290087,#290088,#290089,#290090,
#290091,#290092,#290093,#290094,#290095),.UNSPECIFIED.,.F.,.F.)
B_SPLINE_CURVE_WITH_KNOTS((3,2,2,2,2,2,2,2,2,2,3),(0.0288461538461538,0.0307692307692308,
0.0326923076923077,0.0346153846153846,0.0365384615384615,0.0384615384615385,
0.0403846153846154,0.0423076923076923,0.0442307692307692,0.0461538461538462,
0.0480769230769231),.UNSPECIFIED.)
CURVE()
GEOMETRIC_REPRESENTATION_ITEM()
RATIONAL_B_SPLINE_CURVE((1.,0.951056516295154,1.,0.951056516295154,1.,0.951056516295154,
1.,0.951056516295154,1.,0.951056516295154,1.,0.951056516295154,1.,0.951056516295154,
1.,0.951056516295154,1.,0.951056516295154,1.,0.951056516295154,1.))
REPRESENTATION_ITEM('')
);
#1602=(
BOUNDED_CURVE()
B_SPLINE_CURVE(2,(#290100,#290101,#290102,#290103,#290104,#290105,#290106,
#290107,#290108,#290109,#290110,#290111,#290112,#290113,#290114,#290115,
#290116,#290117,#290118,#290119,#290120),.UNSPECIFIED.,.F.,.F.)
B_SPLINE_CURVE_WITH_KNOTS((3,2,2,2,2,2,2,2,2,2,3),(0.0480769230769231,0.05,
0.0519230769230769,0.0538461538461538,0.0557692307692308,0.0576923076923077,
0.0596153846153846,0.0615384615384615,0.0634615384615385,0.0653846153846154,
0.0673076923076923),.UNSPECIFIED.)
CURVE()
GEOMETRIC_REPRESENTATION_ITEM()
RATIONAL_B_SPLINE_CURVE((1.,0.951056516295154,1.,0.951056516295154,1.,0.951056516295154,
1.,0.951056516295154,1.,0.951056516295154,1.,0.951056516295154,1.,0.951056516295154,
1.,0.951056516295154,1.,0.951056516295154,1.,0.951056516295154,1.))
REPRESENTATION_ITEM('')
);
#1603=(
BOUNDED_CURVE()
B_SPLINE_CURVE(2,(#290121,#290122,#290123,#290124,#290125,#290126,#290127,
#290128,#290129,#290130,#290131,#290132,#290133,#290134,#290135,#290136,
#290137,#290138,#290139,#290140,#290141),.UNSPECIFIED.,.F.,.F.)
B_SPLINE_CURVE_WITH_KNOTS((3,2,2,2,2,2,2,2,2,2,3),(0.0480769230769231,0.05,
0.0519230769230769,0.0538461538461538,0.0557692307692308,0.0576923076923077,
0.0596153846153846,0.0615384615384615,0.0634615384615385,0.0653846153846154,
0.0673076923076923),.UNSPECIFIED.)
CURVE()
GEOMETRIC_REPRESENTATION_ITEM()
RATIONAL_B_SPLINE_CURVE((1.,0.951056516295154,1.,0.951056516295154,1.,0.951056516295154,
1.,0.951056516295154,1.,0.951056516295154,1.,0.951056516295154,1.,0.951056516295154,
1.,0.951056516295154,1.,0.951056516295154,1.,0.951056516295154,1.))
REPRESENTATION_ITEM('')
);
#1604=(
BOUNDED_CURVE()
B_SPLINE_CURVE(2,(#290146,#290147,#290148,#290149,#290150,#290151,#290152,
#290153,#290154,#290155,#290156,#290157,#290158,#290159,#290160,#290161,
#290162,#290163,#290164,#290165,#290166),.UNSPECIFIED.,.F.,.F.)
B_SPLINE_CURVE_WITH_KNOTS((3,2,2,2,2,2,2,2,2,2,3),(0.0673076923076923,0.0692307692307692,
0.0711538461538462,0.0730769230769231,0.075,0.0769230769230769,0.0788461538461538,
0.0807692307692308,0.0826923076923077,0.0846153846153846,0.0865384615384615),
 .UNSPECIFIED.)
CURVE()
GEOMETRIC_REPRESENTATION_ITEM()
RATIONAL_B_SPLINE_CURVE((1.,0.951056516295154,1.,0.951056516295154,1.,0.951056516295154,
1.,0.951056516295154,1.,0.951056516295154,1.,0.951056516295154,1.,0.951056516295154,
1.,0.951056516295154,1.,0.951056516295154,1.,0.951056516295154,1.))
REPRESENTATION_ITEM('')
);
#1605=(
BOUNDED_CURVE()
B_SPLINE_CURVE(2,(#290167,#290168,#290169,#290170,#290171,#290172,#290173,
#290174,#290175,#290176,#290177,#290178,#290179,#290180,#290181,#290182,
#290183,#290184,#290185,#290186,#290187),.UNSPECIFIED.,.F.,.F.)
B_SPLINE_CURVE_WITH_KNOTS((3,2,2,2,2,2,2,2,2,2,3),(0.0673076923076923,0.0692307692307692,
0.0711538461538462,0.0730769230769231,0.075,0.0769230769230769,0.0788461538461538,
0.0807692307692308,0.0826923076923077,0.0846153846153846,0.0865384615384615),
 .UNSPECIFIED.)
CURVE()
GEOMETRIC_REPRESENTATION_ITEM()
RATIONAL_B_SPLINE_CURVE((1.,0.951056516295154,1.,0.951056516295154,1.,0.951056516295154,
1.,0.951056516295154,1.,0.951056516295154,1.,0.951056516295154,1.,0.951056516295154,
1.,0.951056516295154,1.,0.951056516295154,1.,0.951056516295154,1.))
REPRESENTATION_ITEM('')
);
#1606=(
BOUNDED_CURVE()
B_SPLINE_CURVE(2,(#290192,#290193,#290194,#290195,#290196,#290197,#290198,
#290199,#290200,#290201,#290202,#290203,#290204,#290205,#290206,#290207,
#290208,#290209,#290210,#290211,#290212),.UNSPECIFIED.,.F.,.F.)
B_SPLINE_CURVE_WITH_KNOTS((3,2,2,2,2,2,2,2,2,2,3),(0.0865384615384615,0.0884615384615385,
0.0903846153846154,0.0923076923076923,0.0942307692307692,0.0961538461538462,
0.0980769230769231,0.1,0.101923076923077,0.103846153846154,0.105769230769231),
 .UNSPECIFIED.)
CURVE()
GEOMETRIC_REPRESENTATION_ITEM()
RATIONAL_B_SPLINE_CURVE((1.,0.951056516295154,1.,0.951056516295154,1.,0.951056516295154,
1.,0.951056516295154,1.,0.951056516295154,1.,0.951056516295154,1.,0.951056516295154,
1.,0.951056516295154,1.,0.951056516295154,1.,0.951056516295154,1.))
REPRESENTATION_ITEM('')
);
#1607=(
BOUNDED_CURVE()
B_SPLINE_CURVE(2,(#290213,#290214,#290215,#290216,#290217,#290218,#290219,
#290220,#290221,#290222,#290223,#290224,#290225,#290226,#290227,#290228,
#290229,#290230,#290231,#290232,#290233),.UNSPECIFIED.,.F.,.F.)
B_SPLINE_CURVE_WITH_KNOTS((3,2,2,2,2,2,2,2,2,2,3),(0.0865384615384615,0.0884615384615385,
0.0903846153846154,0.0923076923076923,0.0942307692307692,0.0961538461538462,
0.0980769230769231,0.1,0.101923076923077,0.103846153846154,0.105769230769231),
 .UNSPECIFIED.)
CURVE()
GEOMETRIC_REPRESENTATION_ITEM()
RATIONAL_B_SPLINE_CURVE((1.,0.951056516295154,1.,0.951056516295154,1.,0.951056516295154,
1.,0.951056516295154,1.,0.951056516295154,1.,0.951056516295154,1.,0.951056516295154,
1.,0.951056516295154,1.,0.951056516295154,1.,0.951056516295154,1.))
REPRESENTATION_ITEM('')
);
#1608=(
BOUNDED_CURVE()
B_SPLINE_CURVE(2,(#290238,#290239,#290240,#290241,#290242,#290243,#290244,
#290245,#290246,#290247,#290248,#290249,#290250,#290251,#290252,#290253,
#290254,#290255,#290256,#290257,#290258),.UNSPECIFIED.,.F.,.F.)
B_SPLINE_CURVE_WITH_KNOTS((3,2,2,2,2,2,2,2,2,2,3),(0.105769230769231,0.107692307692308,
0.109615384615385,0.111538461538462,0.113461538461538,0.115384615384615,
0.117307692307692,0.119230769230769,0.121153846153846,0.123076923076923,
0.125),.UNSPECIFIED.)
CURVE()
GEOMETRIC_REPRESENTATION_ITEM()
RATIONAL_B_SPLINE_CURVE((1.,0.951056516295154,1.,0.951056516295154,1.,0.951056516295154,
1.,0.951056516295154,1.,0.951056516295154,1.,0.951056516295154,1.,0.951056516295154,
1.,0.951056516295154,1.,0.951056516295154,1.,0.951056516295154,1.))
REPRESENTATION_ITEM('')
);
#1609=(
BOUNDED_CURVE()
B_SPLINE_CURVE(2,(#290259,#290260,#290261,#290262,#290263,#290264,#290265,
#290266,#290267,#290268,#290269,#290270,#290271,#290272,#290273,#290274,
#290275,#290276,#290277,#290278,#290279),.UNSPECIFIED.,.F.,.F.)
B_SPLINE_CURVE_WITH_KNOTS((3,2,2,2,2,2,2,2,2,2,3),(0.105769230769231,0.107692307692308,
0.109615384615385,0.111538461538462,0.113461538461538,0.115384615384615,
0.117307692307692,0.119230769230769,0.121153846153846,0.123076923076923,
0.125),.UNSPECIFIED.)
CURVE()
GEOMETRIC_REPRESENTATION_ITEM()
RATIONAL_B_SPLINE_CURVE((1.,0.951056516295154,1.,0.951056516295154,1.,0.951056516295154,
1.,0.951056516295154,1.,0.951056516295154,1.,0.951056516295154,1.,0.951056516295154,
1.,0.951056516295154,1.,0.951056516295154,1.,0.951056516295154,1.))
REPRESENTATION_ITEM('')
);
#1610=(
BOUNDED_CURVE()
B_SPLINE_CURVE(2,(#290284,#290285,#290286,#290287,#290288,#290289,#290290,
#290291,#290292,#290293,#290294,#290295,#290296,#290297,#290298,#290299,
#290300,#290301,#290302,#290303,#290304),.UNSPECIFIED.,.F.,.F.)
B_SPLINE_CURVE_WITH_KNOTS((3,2,2,2,2,2,2,2,2,2,3),(0.125,0.126923076923077,
0.128846153846154,0.130769230769231,0.132692307692308,0.134615384615385,
0.136538461538462,0.138461538461538,0.140384615384615,0.142307692307692,
0.144230769230769),.UNSPECIFIED.)
CURVE()
GEOMETRIC_REPRESENTATION_ITEM()
RATIONAL_B_SPLINE_CURVE((1.,0.951056516295154,1.,0.951056516295154,1.,0.951056516295154,
1.,0.951056516295154,1.,0.951056516295154,1.,0.951056516295154,1.,0.951056516295154,
1.,0.951056516295154,1.,0.951056516295154,1.,0.951056516295154,1.))
REPRESENTATION_ITEM('')
);
#1611=(
BOUNDED_CURVE()
B_SPLINE_CURVE(2,(#290305,#290306,#290307,#290308,#290309,#290310,#290311,
#290312,#290313,#290314,#290315,#290316,#290317,#290318,#290319,#290320,
#290321,#290322,#290323,#290324,#290325),.UNSPECIFIED.,.F.,.F.)
B_SPLINE_CURVE_WITH_KNOTS((3,2,2,2,2,2,2,2,2,2,3),(0.125,0.126923076923077,
0.128846153846154,0.130769230769231,0.132692307692308,0.134615384615385,
0.136538461538462,0.138461538461538,0.140384615384615,0.142307692307692,
0.144230769230769),.UNSPECIFIED.)
CURVE()
GEOMETRIC_REPRESENTATION_ITEM()
RATIONAL_B_SPLINE_CURVE((1.,0.951056516295154,1.,0.951056516295154,1.,0.951056516295154,
1.,0.951056516295154,1.,0.951056516295154,1.,0.951056516295154,1.,0.951056516295154,
1.,0.951056516295154,1.,0.951056516295154,1.,0.951056516295154,1.))
REPRESENTATION_ITEM('')
);
#1612=(
BOUNDED_CURVE()
B_SPLINE_CURVE(2,(#290330,#290331,#290332,#290333,#290334,#290335,#290336,
#290337,#290338,#290339,#290340,#290341,#290342,#290343,#290344,#290345,
#290346,#290347,#290348,#290349,#290350),.UNSPECIFIED.,.F.,.F.)
B_SPLINE_CURVE_WITH_KNOTS((3,2,2,2,2,2,2,2,2,2,3),(0.144230769230769,0.146153846153846,
0.148076923076923,0.15,0.151923076923077,0.153846153846154,0.155769230769231,
0.157692307692308,0.159615384615385,0.161538461538462,0.163461538461538),
 .UNSPECIFIED.)
CURVE()
GEOMETRIC_REPRESENTATION_ITEM()
RATIONAL_B_SPLINE_CURVE((1.,0.951056516295154,1.,0.951056516295154,1.,0.951056516295154,
1.,0.951056516295154,1.,0.951056516295154,1.,0.951056516295154,1.,0.951056516295154,
1.,0.951056516295154,1.,0.951056516295154,1.,0.951056516295154,1.))
REPRESENTATION_ITEM('')
);
#1613=(
BOUNDED_CURVE()
B_SPLINE_CURVE(2,(#290351,#290352,#290353,#290354,#290355,#290356,#290357,
#290358,#290359,#290360,#290361,#290362,#290363,#290364,#290365,#290366,
#290367,#290368,#290369,#290370,#290371),.UNSPECIFIED.,.F.,.F.)
B_SPLINE_CURVE_WITH_KNOTS((3,2,2,2,2,2,2,2,2,2,3),(0.144230769230769,0.146153846153846,
0.148076923076923,0.15,0.151923076923077,0.153846153846154,0.155769230769231,
0.157692307692308,0.159615384615385,0.161538461538462,0.163461538461538),
 .UNSPECIFIED.)
CURVE()
GEOMETRIC_REPRESENTATION_ITEM()
RATIONAL_B_SPLINE_CURVE((1.,0.951056516295154,1.,0.951056516295154,1.,0.951056516295154,
1.,0.951056516295154,1.,0.951056516295154,1.,0.951056516295154,1.,0.951056516295154,
1.,0.951056516295154,1.,0.951056516295154,1.,0.951056516295154,1.))
REPRESENTATION_ITEM('')
);
#1614=(
BOUNDED_CURVE()
B_SPLINE_CURVE(2,(#290376,#290377,#290378,#290379,#290380,#290381,#290382,
#290383,#290384,#290385,#290386,#290387,#290388,#290389,#290390,#290391,
#290392,#290393,#290394,#290395,#290396),.UNSPECIFIED.,.F.,.F.)
B_SPLINE_CURVE_WITH_KNOTS((3,2,2,2,2,2,2,2,2,2,3),(0.163461538461538,0.165384615384615,
0.167307692307692,0.169230769230769,0.171153846153846,0.173076923076923,
0.175,0.176923076923077,0.178846153846154,0.180769230769231,0.182692307692308),
 .UNSPECIFIED.)
CURVE()
GEOMETRIC_REPRESENTATION_ITEM()
RATIONAL_B_SPLINE_CURVE((1.,0.951056516295154,1.,0.951056516295154,1.,0.951056516295154,
1.,0.951056516295154,1.,0.951056516295154,1.,0.951056516295154,1.,0.951056516295154,
1.,0.951056516295154,1.,0.951056516295154,1.,0.951056516295154,1.))
REPRESENTATION_ITEM('')
);
#1615=(
BOUNDED_CURVE()
B_SPLINE_CURVE(2,(#290397,#290398,#290399,#290400,#290401,#290402,#290403,
#290404,#290405,#290406,#290407,#290408,#290409,#290410,#290411,#290412,
#290413,#290414,#290415,#290416,#290417),.UNSPECIFIED.,.F.,.F.)
B_SPLINE_CURVE_WITH_KNOTS((3,2,2,2,2,2,2,2,2,2,3),(0.163461538461538,0.165384615384615,
0.167307692307692,0.169230769230769,0.171153846153846,0.173076923076923,
0.175,0.176923076923077,0.178846153846154,0.180769230769231,0.182692307692308),
 .UNSPECIFIED.)
CURVE()
GEOMETRIC_REPRESENTATION_ITEM()
RATIONAL_B_SPLINE_CURVE((1.,0.951056516295154,1.,0.951056516295154,1.,0.951056516295154,
1.,0.951056516295154,1.,0.951056516295154,1.,0.951056516295154,1.,0.951056516295154,
1.,0.951056516295154,1.,0.951056516295154,1.,0.951056516295154,1.))
REPRESENTATION_ITEM('')
);
#1616=(
BOUNDED_CURVE()
B_SPLINE_CURVE(2,(#290422,#290423,#290424,#290425,#290426,#290427,#290428,
#290429,#290430,#290431,#290432,#290433,#290434,#290435,#290436,#290437,
#290438,#290439,#290440,#290441,#290442),.UNSPECIFIED.,.F.,.F.)
B_SPLINE_CURVE_WITH_KNOTS((3,2,2,2,2,2,2,2,2,2,3),(0.182692307692308,0.184615384615385,
0.186538461538462,0.188461538461538,0.190384615384615,0.192307692307692,
0.194230769230769,0.196153846153846,0.198076923076923,0.2,0.201923076923077),
 .UNSPECIFIED.)
CURVE()
GEOMETRIC_REPRESENTATION_ITEM()
RATIONAL_B_SPLINE_CURVE((1.,0.951056516295154,1.,0.951056516295154,1.,0.951056516295154,
1.,0.951056516295154,1.,0.951056516295154,1.,0.951056516295154,1.,0.951056516295154,
1.,0.951056516295154,1.,0.951056516295154,1.,0.951056516295154,1.))
REPRESENTATION_ITEM('')
);
#1617=(
BOUNDED_CURVE()
B_SPLINE_CURVE(2,(#290443,#290444,#290445,#290446,#290447,#290448,#290449,
#290450,#290451,#290452,#290453,#290454,#290455,#290456,#290457,#290458,
#290459,#290460,#290461,#290462,#290463),.UNSPECIFIED.,.F.,.F.)
B_SPLINE_CURVE_WITH_KNOTS((3,2,2,2,2,2,2,2,2,2,3),(0.182692307692308,0.184615384615385,
0.186538461538462,0.188461538461538,0.190384615384615,0.192307692307692,
0.194230769230769,0.196153846153846,0.198076923076923,0.2,0.201923076923077),
 .UNSPECIFIED.)
CURVE()
GEOMETRIC_REPRESENTATION_ITEM()
RATIONAL_B_SPLINE_CURVE((1.,0.951056516295154,1.,0.951056516295154,1.,0.951056516295154,
1.,0.951056516295154,1.,0.951056516295154,1.,0.951056516295154,1.,0.951056516295154,
1.,0.951056516295154,1.,0.951056516295154,1.,0.951056516295154,1.))
REPRESENTATION_ITEM('')
);
#1618=(
BOUNDED_CURVE()
B_SPLINE_CURVE(2,(#290468,#290469,#290470,#290471,#290472,#290473,#290474,
#290475,#290476,#290477,#290478,#290479,#290480,#290481,#290482,#290483,
#290484,#290485,#290486,#290487,#290488),.UNSPECIFIED.,.F.,.F.)
B_SPLINE_CURVE_WITH_KNOTS((3,2,2,2,2,2,2,2,2,2,3),(0.201923076923077,0.203846153846154,
0.205769230769231,0.207692307692308,0.209615384615385,0.211538461538462,
0.213461538461538,0.215384615384615,0.217307692307692,0.219230769230769,
0.221153846153846),.UNSPECIFIED.)
CURVE()
GEOMETRIC_REPRESENTATION_ITEM()
RATIONAL_B_SPLINE_CURVE((1.,0.951056516295154,1.,0.951056516295154,1.,0.951056516295154,
1.,0.951056516295154,1.,0.951056516295154,1.,0.951056516295154,1.,0.951056516295154,
1.,0.951056516295154,1.,0.951056516295154,1.,0.951056516295154,1.))
REPRESENTATION_ITEM('')
);
#1619=(
BOUNDED_CURVE()
B_SPLINE_CURVE(2,(#290489,#290490,#290491,#290492,#290493,#290494,#290495,
#290496,#290497,#290498,#290499,#290500,#290501,#290502,#290503,#290504,
#290505,#290506,#290507,#290508,#290509),.UNSPECIFIED.,.F.,.F.)
B_SPLINE_CURVE_WITH_KNOTS((3,2,2,2,2,2,2,2,2,2,3),(0.201923076923077,0.203846153846154,
0.205769230769231,0.207692307692308,0.209615384615385,0.211538461538462,
0.213461538461538,0.215384615384615,0.217307692307692,0.219230769230769,
0.221153846153846),.UNSPECIFIED.)
CURVE()
GEOMETRIC_REPRESENTATION_ITEM()
RATIONAL_B_SPLINE_CURVE((1.,0.951056516295154,1.,0.951056516295154,1.,0.951056516295154,
1.,0.951056516295154,1.,0.951056516295154,1.,0.951056516295154,1.,0.951056516295154,
1.,0.951056516295154,1.,0.951056516295154,1.,0.951056516295154,1.))
REPRESENTATION_ITEM('')
);
#1620=(
BOUNDED_CURVE()
B_SPLINE_CURVE(2,(#290514,#290515,#290516,#290517,#290518,#290519,#290520,
#290521,#290522,#290523,#290524,#290525,#290526,#290527,#290528,#290529,
#290530,#290531,#290532,#290533,#290534),.UNSPECIFIED.,.F.,.F.)
B_SPLINE_CURVE_WITH_KNOTS((3,2,2,2,2,2,2,2,2,2,3),(0.221153846153846,0.223076923076923,
0.225,0.226923076923077,0.228846153846154,0.230769230769231,0.232692307692308,
0.234615384615385,0.236538461538462,0.238461538461538,0.240384615384615),
 .UNSPECIFIED.)
CURVE()
GEOMETRIC_REPRESENTATION_ITEM()
RATIONAL_B_SPLINE_CURVE((1.,0.951056516295154,1.,0.951056516295154,1.,0.951056516295154,
1.,0.951056516295154,1.,0.951056516295154,1.,0.951056516295154,1.,0.951056516295154,
1.,0.951056516295154,1.,0.951056516295154,1.,0.951056516295154,1.))
REPRESENTATION_ITEM('')
);
#1621=(
BOUNDED_CURVE()
B_SPLINE_CURVE(2,(#290535,#290536,#290537,#290538,#290539,#290540,#290541,
#290542,#290543,#290544,#290545,#290546,#290547,#290548,#290549,#290550,
#290551,#290552,#290553,#290554,#290555),.UNSPECIFIED.,.F.,.F.)
B_SPLINE_CURVE_WITH_KNOTS((3,2,2,2,2,2,2,2,2,2,3),(0.221153846153846,0.223076923076923,
0.225,0.226923076923077,0.228846153846154,0.230769230769231,0.232692307692308,
0.234615384615385,0.236538461538462,0.238461538461538,0.240384615384615),
 .UNSPECIFIED.)
CURVE()
GEOMETRIC_REPRESENTATION_ITEM()
RATIONAL_B_SPLINE_CURVE((1.,0.951056516295154,1.,0.951056516295154,1.,0.951056516295154,
1.,0.951056516295154,1.,0.951056516295154,1.,0.951056516295154,1.,0.951056516295154,
1.,0.951056516295154,1.,0.951056516295154,1.,0.951056516295154,1.))
REPRESENTATION_ITEM('')
);
#1622=(
BOUNDED_CURVE()
B_SPLINE_CURVE(2,(#290560,#290561,#290562,#290563,#290564,#290565,#290566,
#290567,#290568,#290569,#290570,#290571,#290572,#290573,#290574,#290575,
#290576,#290577,#290578,#290579,#290580),.UNSPECIFIED.,.F.,.F.)
B_SPLINE_CURVE_WITH_KNOTS((3,2,2,2,2,2,2,2,2,2,3),(0.240384615384615,0.242307692307692,
0.244230769230769,0.246153846153846,0.248076923076923,0.25,0.251923076923077,
0.253846153846154,0.255769230769231,0.257692307692308,0.259615384615385),
 .UNSPECIFIED.)
CURVE()
GEOMETRIC_REPRESENTATION_ITEM()
RATIONAL_B_SPLINE_CURVE((1.,0.951056516295154,1.,0.951056516295154,1.,0.951056516295154,
1.,0.951056516295154,1.,0.951056516295154,1.,0.951056516295154,1.,0.951056516295154,
1.,0.951056516295154,1.,0.951056516295154,1.,0.951056516295154,1.))
REPRESENTATION_ITEM('')
);
#1623=(
BOUNDED_CURVE()
B_SPLINE_CURVE(2,(#290581,#290582,#290583,#290584,#290585,#290586,#290587,
#290588,#290589,#290590,#290591,#290592,#290593,#290594,#290595,#290596,
#290597,#290598,#290599,#290600,#290601),.UNSPECIFIED.,.F.,.F.)
B_SPLINE_CURVE_WITH_KNOTS((3,2,2,2,2,2,2,2,2,2,3),(0.240384615384615,0.242307692307692,
0.244230769230769,0.246153846153846,0.248076923076923,0.25,0.251923076923077,
0.253846153846154,0.255769230769231,0.257692307692308,0.259615384615385),
 .UNSPECIFIED.)
CURVE()
GEOMETRIC_REPRESENTATION_ITEM()
RATIONAL_B_SPLINE_CURVE((1.,0.951056516295154,1.,0.951056516295154,1.,0.951056516295154,
1.,0.951056516295154,1.,0.951056516295154,1.,0.951056516295154,1.,0.951056516295154,
1.,0.951056516295154,1.,0.951056516295154,1.,0.951056516295154,1.))
REPRESENTATION_ITEM('')
);
#1624=(
BOUNDED_CURVE()
B_SPLINE_CURVE(2,(#290606,#290607,#290608,#290609,#290610,#290611,#290612,
#290613,#290614,#290615,#290616,#290617,#290618,#290619,#290620,#290621,
#290622,#290623,#290624,#290625,#290626),.UNSPECIFIED.,.F.,.F.)
B_SPLINE_CURVE_WITH_KNOTS((3,2,2,2,2,2,2,2,2,2,3),(0.259615384615385,0.261538461538462,
0.263461538461538,0.265384615384615,0.267307692307692,0.269230769230769,
0.271153846153846,0.273076923076923,0.275,0.276923076923077,0.278846153846154),
 .UNSPECIFIED.)
CURVE()
GEOMETRIC_REPRESENTATION_ITEM()
RATIONAL_B_SPLINE_CURVE((1.,0.951056516295154,1.,0.951056516295154,1.,0.951056516295154,
1.,0.951056516295154,1.,0.951056516295154,1.,0.951056516295154,1.,0.951056516295154,
1.,0.951056516295154,1.,0.951056516295154,1.,0.951056516295154,1.))
REPRESENTATION_ITEM('')
);
#1625=(
BOUNDED_CURVE()
B_SPLINE_CURVE(2,(#290627,#290628,#290629,#290630,#290631,#290632,#290633,
#290634,#290635,#290636,#290637,#290638,#290639,#290640,#290641,#290642,
#290643,#290644,#290645,#290646,#290647),.UNSPECIFIED.,.F.,.F.)
B_SPLINE_CURVE_WITH_KNOTS((3,2,2,2,2,2,2,2,2,2,3),(0.259615384615385,0.261538461538462,
0.263461538461538,0.265384615384615,0.267307692307692,0.269230769230769,
0.271153846153846,0.273076923076923,0.275,0.276923076923077,0.278846153846154),
 .UNSPECIFIED.)
CURVE()
GEOMETRIC_REPRESENTATION_ITEM()
RATIONAL_B_SPLINE_CURVE((1.,0.951056516295154,1.,0.951056516295154,1.,0.951056516295154,
1.,0.951056516295154,1.,0.951056516295154,1.,0.951056516295154,1.,0.951056516295154,
1.,0.951056516295154,1.,0.951056516295154,1.,0.951056516295154,1.))
REPRESENTATION_ITEM('')
);
#1626=(
BOUNDED_CURVE()
B_SPLINE_CURVE(2,(#290652,#290653,#290654,#290655,#290656,#290657,#290658,
#290659,#290660,#290661,#290662,#290663,#290664,#290665,#290666,#290667,
#290668,#290669,#290670,#290671,#290672),.UNSPECIFIED.,.F.,.F.)
B_SPLINE_CURVE_WITH_KNOTS((3,2,2,2,2,2,2,2,2,2,3),(0.278846153846154,0.280769230769231,
0.282692307692308,0.284615384615385,0.286538461538462,0.288461538461538,
0.290384615384615,0.292307692307692,0.294230769230769,0.296153846153846,
0.298076923076923),.UNSPECIFIED.)
CURVE()
GEOMETRIC_REPRESENTATION_ITEM()
RATIONAL_B_SPLINE_CURVE((1.,0.951056516295154,1.,0.951056516295154,1.,0.951056516295154,
1.,0.951056516295154,1.,0.951056516295154,1.,0.951056516295154,1.,0.951056516295154,
1.,0.951056516295154,1.,0.951056516295154,1.,0.951056516295154,1.))
REPRESENTATION_ITEM('')
);
#1627=(
BOUNDED_CURVE()
B_SPLINE_CURVE(2,(#290673,#290674,#290675,#290676,#290677,#290678,#290679,
#290680,#290681,#290682,#290683,#290684,#290685,#290686,#290687,#290688,
#290689,#290690,#290691,#290692,#290693),.UNSPECIFIED.,.F.,.F.)
B_SPLINE_CURVE_WITH_KNOTS((3,2,2,2,2,2,2,2,2,2,3),(0.278846153846154,0.280769230769231,
0.282692307692308,0.284615384615385,0.286538461538462,0.288461538461538,
0.290384615384615,0.292307692307692,0.294230769230769,0.296153846153846,
0.298076923076923),.UNSPECIFIED.)
CURVE()
GEOMETRIC_REPRESENTATION_ITEM()
RATIONAL_B_SPLINE_CURVE((1.,0.951056516295154,1.,0.951056516295154,1.,0.951056516295154,
1.,0.951056516295154,1.,0.951056516295154,1.,0.951056516295154,1.,0.951056516295154,
1.,0.951056516295154,1.,0.951056516295154,1.,0.951056516295154,1.))
REPRESENTATION_ITEM('')
);
#1628=(
BOUNDED_CURVE()
B_SPLINE_CURVE(2,(#290698,#290699,#290700,#290701,#290702,#290703,#290704,
#290705,#290706,#290707,#290708,#290709,#290710,#290711,#290712,#290713,
#290714,#290715,#290716,#290717,#290718),.UNSPECIFIED.,.F.,.F.)
B_SPLINE_CURVE_WITH_KNOTS((3,2,2,2,2,2,2,2,2,2,3),(0.298076923076923,0.3,
0.301923076923077,0.303846153846154,0.305769230769231,0.307692307692308,
0.309615384615385,0.311538461538462,0.313461538461538,0.315384615384615,
0.317307692307692),.UNSPECIFIED.)
CURVE()
GEOMETRIC_REPRESENTATION_ITEM()
RATIONAL_B_SPLINE_CURVE((1.,0.951056516295154,1.,0.951056516295154,1.,0.951056516295154,
1.,0.951056516295154,1.,0.951056516295154,1.,0.951056516295154,1.,0.951056516295154,
1.,0.951056516295154,1.,0.951056516295154,1.,0.951056516295154,1.))
REPRESENTATION_ITEM('')
);
#1629=(
BOUNDED_CURVE()
B_SPLINE_CURVE(2,(#290719,#290720,#290721,#290722,#290723,#290724,#290725,
#290726,#290727,#290728,#290729,#290730,#290731,#290732,#290733,#290734,
#290735,#290736,#290737,#290738,#290739),.UNSPECIFIED.,.F.,.F.)
B_SPLINE_CURVE_WITH_KNOTS((3,2,2,2,2,2,2,2,2,2,3),(0.298076923076923,0.3,
0.301923076923077,0.303846153846154,0.305769230769231,0.307692307692308,
0.309615384615385,0.311538461538462,0.313461538461538,0.315384615384615,
0.317307692307692),.UNSPECIFIED.)
CURVE()
GEOMETRIC_REPRESENTATION_ITEM()
RATIONAL_B_SPLINE_CURVE((1.,0.951056516295154,1.,0.951056516295154,1.,0.951056516295154,
1.,0.951056516295154,1.,0.951056516295154,1.,0.951056516295154,1.,0.951056516295154,
1.,0.951056516295154,1.,0.951056516295154,1.,0.951056516295154,1.))
REPRESENTATION_ITEM('')
);
#1630=(
BOUNDED_CURVE()
B_SPLINE_CURVE(2,(#290744,#290745,#290746,#290747,#290748,#290749,#290750,
#290751,#290752,#290753,#290754,#290755,#290756,#290757,#290758,#290759,
#290760,#290761,#290762,#290763,#290764),.UNSPECIFIED.,.F.,.F.)
B_SPLINE_CURVE_WITH_KNOTS((3,2,2,2,2,2,2,2,2,2,3),(0.317307692307692,0.319230769230769,
0.321153846153846,0.323076923076923,0.325,0.326923076923077,0.328846153846154,
0.330769230769231,0.332692307692308,0.334615384615385,0.336538461538462),
 .UNSPECIFIED.)
CURVE()
GEOMETRIC_REPRESENTATION_ITEM()
RATIONAL_B_SPLINE_CURVE((1.,0.951056516295154,1.,0.951056516295154,1.,0.951056516295154,
1.,0.951056516295154,1.,0.951056516295154,1.,0.951056516295154,1.,0.951056516295154,
1.,0.951056516295154,1.,0.951056516295154,1.,0.951056516295154,1.))
REPRESENTATION_ITEM('')
);
#1631=(
BOUNDED_CURVE()
B_SPLINE_CURVE(2,(#290765,#290766,#290767,#290768,#290769,#290770,#290771,
#290772,#290773,#290774,#290775,#290776,#290777,#290778,#290779,#290780,
#290781,#290782,#290783,#290784,#290785),.UNSPECIFIED.,.F.,.F.)
B_SPLINE_CURVE_WITH_KNOTS((3,2,2,2,2,2,2,2,2,2,3),(0.317307692307692,0.319230769230769,
0.321153846153846,0.323076923076923,0.325,0.326923076923077,0.328846153846154,
0.330769230769231,0.332692307692308,0.334615384615385,0.336538461538462),
 .UNSPECIFIED.)
CURVE()
GEOMETRIC_REPRESENTATION_ITEM()
RATIONAL_B_SPLINE_CURVE((1.,0.951056516295154,1.,0.951056516295154,1.,0.951056516295154,
1.,0.951056516295154,1.,0.951056516295154,1.,0.951056516295154,1.,0.951056516295154,
1.,0.951056516295154,1.,0.951056516295154,1.,0.951056516295154,1.))
REPRESENTATION_ITEM('')
);
#1632=(
BOUNDED_CURVE()
B_SPLINE_CURVE(2,(#290790,#290791,#290792,#290793,#290794,#290795,#290796,
#290797,#290798,#290799,#290800,#290801,#290802,#290803,#290804,#290805,
#290806,#290807,#290808,#290809,#290810),.UNSPECIFIED.,.F.,.F.)
B_SPLINE_CURVE_WITH_KNOTS((3,2,2,2,2,2,2,2,2,2,3),(0.336538461538462,0.338461538461538,
0.340384615384615,0.342307692307692,0.344230769230769,0.346153846153846,
0.348076923076923,0.35,0.351923076923077,0.353846153846154,0.355769230769231),
 .UNSPECIFIED.)
CURVE()
GEOMETRIC_REPRESENTATION_ITEM()
RATIONAL_B_SPLINE_CURVE((1.,0.951056516295154,1.,0.951056516295154,1.,0.951056516295154,
1.,0.951056516295154,1.,0.951056516295154,1.,0.951056516295154,1.,0.951056516295154,
1.,0.951056516295154,1.,0.951056516295154,1.,0.951056516295154,1.))
REPRESENTATION_ITEM('')
);
#1633=(
BOUNDED_CURVE()
B_SPLINE_CURVE(2,(#290811,#290812,#290813,#290814,#290815,#290816,#290817,
#290818,#290819,#290820,#290821,#290822,#290823,#290824,#290825,#290826,
#290827,#290828,#290829,#290830,#290831),.UNSPECIFIED.,.F.,.F.)
B_SPLINE_CURVE_WITH_KNOTS((3,2,2,2,2,2,2,2,2,2,3),(0.336538461538462,0.338461538461538,
0.340384615384615,0.342307692307692,0.344230769230769,0.346153846153846,
0.348076923076923,0.35,0.351923076923077,0.353846153846154,0.355769230769231),
 .UNSPECIFIED.)
CURVE()
GEOMETRIC_REPRESENTATION_ITEM()
RATIONAL_B_SPLINE_CURVE((1.,0.951056516295154,1.,0.951056516295154,1.,0.951056516295154,
1.,0.951056516295154,1.,0.951056516295154,1.,0.951056516295154,1.,0.951056516295154,
1.,0.951056516295154,1.,0.951056516295154,1.,0.951056516295154,1.))
REPRESENTATION_ITEM('')
);
#1634=(
BOUNDED_CURVE()
B_SPLINE_CURVE(2,(#290836,#290837,#290838,#290839,#290840,#290841,#290842,
#290843,#290844,#290845,#290846,#290847,#290848,#290849,#290850,#290851,
#290852,#290853,#290854,#290855,#290856),.UNSPECIFIED.,.F.,.F.)
B_SPLINE_CURVE_WITH_KNOTS((3,2,2,2,2,2,2,2,2,2,3),(0.355769230769231,0.357692307692308,
0.359615384615385,0.361538461538462,0.363461538461538,0.365384615384615,
0.367307692307692,0.369230769230769,0.371153846153846,0.373076923076923,
0.375),.UNSPECIFIED.)
CURVE()
GEOMETRIC_REPRESENTATION_ITEM()
RATIONAL_B_SPLINE_CURVE((1.,0.951056516295154,1.,0.951056516295154,1.,0.951056516295154,
1.,0.951056516295154,1.,0.951056516295154,1.,0.951056516295154,1.,0.951056516295154,
1.,0.951056516295154,1.,0.951056516295154,1.,0.951056516295154,1.))
REPRESENTATION_ITEM('')
);
#1635=(
BOUNDED_CURVE()
B_SPLINE_CURVE(2,(#290857,#290858,#290859,#290860,#290861,#290862,#290863,
#290864,#290865,#290866,#290867,#290868,#290869,#290870,#290871,#290872,
#290873,#290874,#290875,#290876,#290877),.UNSPECIFIED.,.F.,.F.)
B_SPLINE_CURVE_WITH_KNOTS((3,2,2,2,2,2,2,2,2,2,3),(0.355769230769231,0.357692307692308,
0.359615384615385,0.361538461538462,0.363461538461538,0.365384615384615,
0.367307692307692,0.369230769230769,0.371153846153846,0.373076923076923,
0.375),.UNSPECIFIED.)
CURVE()
GEOMETRIC_REPRESENTATION_ITEM()
RATIONAL_B_SPLINE_CURVE((1.,0.951056516295154,1.,0.951056516295154,1.,0.951056516295154,
1.,0.951056516295154,1.,0.951056516295154,1.,0.951056516295154,1.,0.951056516295154,
1.,0.951056516295154,1.,0.951056516295154,1.,0.951056516295154,1.))
REPRESENTATION_ITEM('')
);
#1636=(
BOUNDED_CURVE()
B_SPLINE_CURVE(2,(#290882,#290883,#290884,#290885,#290886,#290887,#290888,
#290889,#290890,#290891,#290892,#290893,#290894,#290895,#290896,#290897,
#290898,#290899,#290900,#290901,#290902),.UNSPECIFIED.,.F.,.F.)
B_SPLINE_CURVE_WITH_KNOTS((3,2,2,2,2,2,2,2,2,2,3),(0.375,0.376923076923077,
0.378846153846154,0.380769230769231,0.382692307692308,0.384615384615385,
0.386538461538462,0.388461538461538,0.390384615384615,0.392307692307692,
0.394230769230769),.UNSPECIFIED.)
CURVE()
GEOMETRIC_REPRESENTATION_ITEM()
RATIONAL_B_SPLINE_CURVE((1.,0.951056516295154,1.,0.951056516295154,1.,0.951056516295154,
1.,0.951056516295154,1.,0.951056516295154,1.,0.951056516295154,1.,0.951056516295154,
1.,0.951056516295154,1.,0.951056516295154,1.,0.951056516295154,1.))
REPRESENTATION_ITEM('')
);
#1637=(
BOUNDED_CURVE()
B_SPLINE_CURVE(2,(#290903,#290904,#290905,#290906,#290907,#290908,#290909,
#290910,#290911,#290912,#290913,#290914,#290915,#290916,#290917,#290918,
#290919,#290920,#290921,#290922,#290923),.UNSPECIFIED.,.F.,.F.)
B_SPLINE_CURVE_WITH_KNOTS((3,2,2,2,2,2,2,2,2,2,3),(0.375,0.376923076923077,
0.378846153846154,0.380769230769231,0.382692307692308,0.384615384615385,
0.386538461538462,0.388461538461538,0.390384615384615,0.392307692307692,
0.394230769230769),.UNSPECIFIED.)
CURVE()
GEOMETRIC_REPRESENTATION_ITEM()
RATIONAL_B_SPLINE_CURVE((1.,0.951056516295154,1.,0.951056516295154,1.,0.951056516295154,
1.,0.951056516295154,1.,0.951056516295154,1.,0.951056516295154,1.,0.951056516295154,
1.,0.951056516295154,1.,0.951056516295154,1.,0.951056516295154,1.))
REPRESENTATION_ITEM('')
);
#1638=(
BOUNDED_CURVE()
B_SPLINE_CURVE(2,(#290929,#290930,#290931,#290932,#290933,#290934,#290935,
#290936,#290937,#290938,#290939,#290940,#290941),.UNSPECIFIED.,.F.,.F.)
B_SPLINE_CURVE_WITH_KNOTS((3,2,2,2,2,2,3),(0.595378520967158,0.596153846153846,
0.598076923076923,0.6,0.601923076923077,0.603846153846154,0.605769230769231),
 .UNSPECIFIED.)
CURVE()
GEOMETRIC_REPRESENTATION_ITEM()
RATIONAL_B_SPLINE_CURVE((0.976446068257266,0.980267499866866,1.,0.951056516295154,
1.,0.951056516295154,1.,0.951056516295154,1.,0.951056516295154,1.,0.951056516295154,
1.))
REPRESENTATION_ITEM('')
);
#1639=(
BOUNDED_CURVE()
B_SPLINE_CURVE(2,(#290944,#290945,#290946,#290947,#290948,#290949,#290950,
#290951,#290952,#290953,#290954),.UNSPECIFIED.,.F.,.F.)
B_SPLINE_CURVE_WITH_KNOTS((3,2,2,2,2,3),(0.597778235786775,0.598076923076923,
0.6,0.601923076923077,0.603846153846154,0.605769230769231),
 .UNSPECIFIED.)
CURVE()
GEOMETRIC_REPRESENTATION_ITEM()
RATIONAL_B_SPLINE_CURVE((0.987157827087347,0.992398225810528,1.,0.951056516295154,
1.,0.951056516295154,1.,0.951056516295154,1.,0.951056516295154,1.))
REPRESENTATION_ITEM('')
);
#1640=(
BOUNDED_CURVE()
B_SPLINE_CURVE(2,(#290959,#290960,#290961,#290962,#290963,#290964,#290965,
#290966,#290967,#290968,#290969,#290970,#290971,#290972,#290973,#290974,
#290975,#290976,#290977,#290978,#290979),.UNSPECIFIED.,.F.,.F.)
B_SPLINE_CURVE_WITH_KNOTS((3,2,2,2,2,2,2,2,2,2,3),(0.605769230769231,0.607692307692308,
0.609615384615385,0.611538461538462,0.613461538461539,0.615384615384615,
0.617307692307692,0.619230769230769,0.621153846153846,0.623076923076923,
0.625),.UNSPECIFIED.)
CURVE()
GEOMETRIC_REPRESENTATION_ITEM()
RATIONAL_B_SPLINE_CURVE((1.,0.951056516295154,1.,0.951056516295154,1.,0.951056516295154,
1.,0.951056516295154,1.,0.951056516295154,1.,0.951056516295154,1.,0.951056516295154,
1.,0.951056516295154,1.,0.951056516295154,1.,0.951056516295154,1.))
REPRESENTATION_ITEM('')
);
#1641=(
BOUNDED_CURVE()
B_SPLINE_CURVE(2,(#290980,#290981,#290982,#290983,#290984,#290985,#290986,
#290987,#290988,#290989,#290990,#290991,#290992,#290993,#290994,#290995,
#290996,#290997,#290998,#290999,#291000),.UNSPECIFIED.,.F.,.F.)
B_SPLINE_CURVE_WITH_KNOTS((3,2,2,2,2,2,2,2,2,2,3),(0.605769230769231,0.607692307692308,
0.609615384615385,0.611538461538462,0.613461538461539,0.615384615384615,
0.617307692307692,0.619230769230769,0.621153846153846,0.623076923076923,
0.625),.UNSPECIFIED.)
CURVE()
GEOMETRIC_REPRESENTATION_ITEM()
RATIONAL_B_SPLINE_CURVE((1.,0.951056516295154,1.,0.951056516295154,1.,0.951056516295154,
1.,0.951056516295154,1.,0.951056516295154,1.,0.951056516295154,1.,0.951056516295154,
1.,0.951056516295154,1.,0.951056516295154,1.,0.951056516295154,1.))
REPRESENTATION_ITEM('')
);
#1642=(
BOUNDED_CURVE()
B_SPLINE_CURVE(2,(#291005,#291006,#291007,#291008,#291009,#291010,#291011,
#291012,#291013,#291014,#291015,#291016,#291017,#291018,#291019,#291020,
#291021,#291022,#291023,#291024,#291025),.UNSPECIFIED.,.F.,.F.)
B_SPLINE_CURVE_WITH_KNOTS((3,2,2,2,2,2,2,2,2,2,3),(0.625,0.626923076923077,
0.628846153846154,0.630769230769231,0.632692307692308,0.634615384615385,
0.636538461538461,0.638461538461538,0.640384615384615,0.642307692307692,
0.644230769230769),.UNSPECIFIED.)
CURVE()
GEOMETRIC_REPRESENTATION_ITEM()
RATIONAL_B_SPLINE_CURVE((1.,0.951056516295154,1.,0.951056516295154,1.,0.951056516295154,
1.,0.951056516295154,1.,0.951056516295154,1.,0.951056516295154,1.,0.951056516295154,
1.,0.951056516295154,1.,0.951056516295154,1.,0.951056516295154,1.))
REPRESENTATION_ITEM('')
);
#1643=(
BOUNDED_CURVE()
B_SPLINE_CURVE(2,(#291026,#291027,#291028,#291029,#291030,#291031,#291032,
#291033,#291034,#291035,#291036,#291037,#291038,#291039,#291040,#291041,
#291042,#291043,#291044,#291045,#291046),.UNSPECIFIED.,.F.,.F.)
B_SPLINE_CURVE_WITH_KNOTS((3,2,2,2,2,2,2,2,2,2,3),(0.625,0.626923076923077,
0.628846153846154,0.630769230769231,0.632692307692308,0.634615384615385,
0.636538461538461,0.638461538461538,0.640384615384615,0.642307692307692,
0.644230769230769),.UNSPECIFIED.)
CURVE()
GEOMETRIC_REPRESENTATION_ITEM()
RATIONAL_B_SPLINE_CURVE((1.,0.951056516295154,1.,0.951056516295154,1.,0.951056516295154,
1.,0.951056516295154,1.,0.951056516295154,1.,0.951056516295154,1.,0.951056516295154,
1.,0.951056516295154,1.,0.951056516295154,1.,0.951056516295154,1.))
REPRESENTATION_ITEM('')
);
#1644=(
BOUNDED_CURVE()
B_SPLINE_CURVE(2,(#291051,#291052,#291053,#291054,#291055,#291056,#291057,
#291058,#291059,#291060,#291061,#291062,#291063,#291064,#291065,#291066,
#291067,#291068,#291069,#291070,#291071),.UNSPECIFIED.,.F.,.F.)
B_SPLINE_CURVE_WITH_KNOTS((3,2,2,2,2,2,2,2,2,2,3),(0.644230769230769,0.646153846153846,
0.648076923076923,0.65,0.651923076923077,0.653846153846154,0.655769230769231,
0.657692307692308,0.659615384615385,0.661538461538462,0.663461538461538),
 .UNSPECIFIED.)
CURVE()
GEOMETRIC_REPRESENTATION_ITEM()
RATIONAL_B_SPLINE_CURVE((1.,0.951056516295154,1.,0.951056516295154,1.,0.951056516295154,
1.,0.951056516295154,1.,0.951056516295154,1.,0.951056516295154,1.,0.951056516295154,
1.,0.951056516295154,1.,0.951056516295154,1.,0.951056516295154,1.))
REPRESENTATION_ITEM('')
);
#1645=(
BOUNDED_CURVE()
B_SPLINE_CURVE(2,(#291072,#291073,#291074,#291075,#291076,#291077,#291078,
#291079,#291080,#291081,#291082,#291083,#291084,#291085,#291086,#291087,
#291088,#291089,#291090,#291091,#291092),.UNSPECIFIED.,.F.,.F.)
B_SPLINE_CURVE_WITH_KNOTS((3,2,2,2,2,2,2,2,2,2,3),(0.644230769230769,0.646153846153846,
0.648076923076923,0.65,0.651923076923077,0.653846153846154,0.655769230769231,
0.657692307692308,0.659615384615385,0.661538461538462,0.663461538461538),
 .UNSPECIFIED.)
CURVE()
GEOMETRIC_REPRESENTATION_ITEM()
RATIONAL_B_SPLINE_CURVE((1.,0.951056516295154,1.,0.951056516295154,1.,0.951056516295154,
1.,0.951056516295154,1.,0.951056516295154,1.,0.951056516295154,1.,0.951056516295154,
1.,0.951056516295154,1.,0.951056516295154,1.,0.951056516295154,1.))
REPRESENTATION_ITEM('')
);
#1646=(
BOUNDED_CURVE()
B_SPLINE_CURVE(2,(#291097,#291098,#291099,#291100,#291101,#291102,#291103,
#291104,#291105,#291106,#291107,#291108,#291109,#291110,#291111,#291112,
#291113,#291114,#291115,#291116,#291117),.UNSPECIFIED.,.F.,.F.)
B_SPLINE_CURVE_WITH_KNOTS((3,2,2,2,2,2,2,2,2,2,3),(0.663461538461538,0.665384615384615,
0.667307692307692,0.669230769230769,0.671153846153846,0.673076923076923,
0.675,0.676923076923077,0.678846153846154,0.680769230769231,0.682692307692308),
 .UNSPECIFIED.)
CURVE()
GEOMETRIC_REPRESENTATION_ITEM()
RATIONAL_B_SPLINE_CURVE((1.,0.951056516295154,1.,0.951056516295154,1.,0.951056516295154,
1.,0.951056516295154,1.,0.951056516295154,1.,0.951056516295154,1.,0.951056516295154,
1.,0.951056516295154,1.,0.951056516295154,1.,0.951056516295154,1.))
REPRESENTATION_ITEM('')
);
#1647=(
BOUNDED_CURVE()
B_SPLINE_CURVE(2,(#291118,#291119,#291120,#291121,#291122,#291123,#291124,
#291125,#291126,#291127,#291128,#291129,#291130,#291131,#291132,#291133,
#291134,#291135,#291136,#291137,#291138),.UNSPECIFIED.,.F.,.F.)
B_SPLINE_CURVE_WITH_KNOTS((3,2,2,2,2,2,2,2,2,2,3),(0.663461538461538,0.665384615384615,
0.667307692307692,0.669230769230769,0.671153846153846,0.673076923076923,
0.675,0.676923076923077,0.678846153846154,0.680769230769231,0.682692307692308),
 .UNSPECIFIED.)
CURVE()
GEOMETRIC_REPRESENTATION_ITEM()
RATIONAL_B_SPLINE_CURVE((1.,0.951056516295154,1.,0.951056516295154,1.,0.951056516295154,
1.,0.951056516295154,1.,0.951056516295154,1.,0.951056516295154,1.,0.951056516295154,
1.,0.951056516295154,1.,0.951056516295154,1.,0.951056516295154,1.))
REPRESENTATION_ITEM('')
);
#1648=(
BOUNDED_CURVE()
B_SPLINE_CURVE(2,(#291143,#291144,#291145,#291146,#291147,#291148,#291149,
#291150,#291151,#291152,#291153,#291154,#291155,#291156,#291157,#291158,
#291159,#291160,#291161,#291162,#291163),.UNSPECIFIED.,.F.,.F.)
B_SPLINE_CURVE_WITH_KNOTS((3,2,2,2,2,2,2,2,2,2,3),(0.682692307692308,0.684615384615385,
0.686538461538462,0.688461538461538,0.690384615384615,0.692307692307692,
0.694230769230769,0.696153846153846,0.698076923076923,0.7,0.701923076923077),
 .UNSPECIFIED.)
CURVE()
GEOMETRIC_REPRESENTATION_ITEM()
RATIONAL_B_SPLINE_CURVE((1.,0.951056516295154,1.,0.951056516295154,1.,0.951056516295154,
1.,0.951056516295154,1.,0.951056516295154,1.,0.951056516295154,1.,0.951056516295154,
1.,0.951056516295154,1.,0.951056516295154,1.,0.951056516295154,1.))
REPRESENTATION_ITEM('')
);
#1649=(
BOUNDED_CURVE()
B_SPLINE_CURVE(2,(#291164,#291165,#291166,#291167,#291168,#291169,#291170,
#291171,#291172,#291173,#291174,#291175,#291176,#291177,#291178,#291179,
#291180,#291181,#291182,#291183,#291184),.UNSPECIFIED.,.F.,.F.)
B_SPLINE_CURVE_WITH_KNOTS((3,2,2,2,2,2,2,2,2,2,3),(0.682692307692308,0.684615384615385,
0.686538461538462,0.688461538461538,0.690384615384615,0.692307692307692,
0.694230769230769,0.696153846153846,0.698076923076923,0.7,0.701923076923077),
 .UNSPECIFIED.)
CURVE()
GEOMETRIC_REPRESENTATION_ITEM()
RATIONAL_B_SPLINE_CURVE((1.,0.951056516295154,1.,0.951056516295154,1.,0.951056516295154,
1.,0.951056516295154,1.,0.951056516295154,1.,0.951056516295154,1.,0.951056516295154,
1.,0.951056516295154,1.,0.951056516295154,1.,0.951056516295154,1.))
REPRESENTATION_ITEM('')
);
#1650=(
BOUNDED_CURVE()
B_SPLINE_CURVE(2,(#291189,#291190,#291191,#291192,#291193,#291194,#291195,
#291196,#291197,#291198,#291199,#291200,#291201,#291202,#291203,#291204,
#291205,#291206,#291207,#291208,#291209),.UNSPECIFIED.,.F.,.F.)
B_SPLINE_CURVE_WITH_KNOTS((3,2,2,2,2,2,2,2,2,2,3),(0.701923076923077,0.703846153846154,
0.705769230769231,0.707692307692308,0.709615384615385,0.711538461538462,
0.713461538461538,0.715384615384615,0.717307692307692,0.719230769230769,
0.721153846153846),.UNSPECIFIED.)
CURVE()
GEOMETRIC_REPRESENTATION_ITEM()
RATIONAL_B_SPLINE_CURVE((1.,0.951056516295154,1.,0.951056516295154,1.,0.951056516295154,
1.,0.951056516295154,1.,0.951056516295154,1.,0.951056516295154,1.,0.951056516295154,
1.,0.951056516295154,1.,0.951056516295154,1.,0.951056516295154,1.))
REPRESENTATION_ITEM('')
);
#1651=(
BOUNDED_CURVE()
B_SPLINE_CURVE(2,(#291210,#291211,#291212,#291213,#291214,#291215,#291216,
#291217,#291218,#291219,#291220,#291221,#291222,#291223,#291224,#291225,
#291226,#291227,#291228,#291229,#291230),.UNSPECIFIED.,.F.,.F.)
B_SPLINE_CURVE_WITH_KNOTS((3,2,2,2,2,2,2,2,2,2,3),(0.701923076923077,0.703846153846154,
0.705769230769231,0.707692307692308,0.709615384615385,0.711538461538462,
0.713461538461538,0.715384615384615,0.717307692307692,0.719230769230769,
0.721153846153846),.UNSPECIFIED.)
CURVE()
GEOMETRIC_REPRESENTATION_ITEM()
RATIONAL_B_SPLINE_CURVE((1.,0.951056516295154,1.,0.951056516295154,1.,0.951056516295154,
1.,0.951056516295154,1.,0.951056516295154,1.,0.951056516295154,1.,0.951056516295154,
1.,0.951056516295154,1.,0.951056516295154,1.,0.951056516295154,1.))
REPRESENTATION_ITEM('')
);
#1652=(
BOUNDED_CURVE()
B_SPLINE_CURVE(2,(#291235,#291236,#291237,#291238,#291239,#291240,#291241,
#291242,#291243,#291244,#291245,#291246,#291247,#291248,#291249,#291250,
#291251,#291252,#291253,#291254,#291255),.UNSPECIFIED.,.F.,.F.)
B_SPLINE_CURVE_WITH_KNOTS((3,2,2,2,2,2,2,2,2,2,3),(0.721153846153846,0.723076923076923,
0.725,0.726923076923077,0.728846153846154,0.730769230769231,0.732692307692308,
0.734615384615385,0.736538461538462,0.738461538461539,0.740384615384615),
 .UNSPECIFIED.)
CURVE()
GEOMETRIC_REPRESENTATION_ITEM()
RATIONAL_B_SPLINE_CURVE((1.,0.951056516295154,1.,0.951056516295154,1.,0.951056516295154,
1.,0.951056516295154,1.,0.951056516295154,1.,0.951056516295154,1.,0.951056516295154,
1.,0.951056516295154,1.,0.951056516295154,1.,0.951056516295154,1.))
REPRESENTATION_ITEM('')
);
#1653=(
BOUNDED_CURVE()
B_SPLINE_CURVE(2,(#291256,#291257,#291258,#291259,#291260,#291261,#291262,
#291263,#291264,#291265,#291266,#291267,#291268,#291269,#291270,#291271,
#291272,#291273,#291274,#291275,#291276),.UNSPECIFIED.,.F.,.F.)
B_SPLINE_CURVE_WITH_KNOTS((3,2,2,2,2,2,2,2,2,2,3),(0.721153846153846,0.723076923076923,
0.725,0.726923076923077,0.728846153846154,0.730769230769231,0.732692307692308,
0.734615384615385,0.736538461538462,0.738461538461539,0.740384615384615),
 .UNSPECIFIED.)
CURVE()
GEOMETRIC_REPRESENTATION_ITEM()
RATIONAL_B_SPLINE_CURVE((1.,0.951056516295154,1.,0.951056516295154,1.,0.951056516295154,
1.,0.951056516295154,1.,0.951056516295154,1.,0.951056516295154,1.,0.951056516295154,
1.,0.951056516295154,1.,0.951056516295154,1.,0.951056516295154,1.))
REPRESENTATION_ITEM('')
);
#1654=(
BOUNDED_CURVE()
B_SPLINE_CURVE(2,(#291281,#291282,#291283,#291284,#291285,#291286,#291287,
#291288,#291289,#291290,#291291,#291292,#291293,#291294,#291295,#291296,
#291297,#291298,#291299,#291300,#291301),.UNSPECIFIED.,.F.,.F.)
B_SPLINE_CURVE_WITH_KNOTS((3,2,2,2,2,2,2,2,2,2,3),(0.740384615384615,0.742307692307692,
0.744230769230769,0.746153846153846,0.748076923076923,0.75,0.751923076923077,
0.753846153846154,0.755769230769231,0.757692307692308,0.759615384615385),
 .UNSPECIFIED.)
CURVE()
GEOMETRIC_REPRESENTATION_ITEM()
RATIONAL_B_SPLINE_CURVE((1.,0.951056516295154,1.,0.951056516295154,1.,0.951056516295154,
1.,0.951056516295154,1.,0.951056516295154,1.,0.951056516295154,1.,0.951056516295154,
1.,0.951056516295154,1.,0.951056516295154,1.,0.951056516295154,1.))
REPRESENTATION_ITEM('')
);
#1655=(
BOUNDED_CURVE()
B_SPLINE_CURVE(2,(#291302,#291303,#291304,#291305,#291306,#291307,#291308,
#291309,#291310,#291311,#291312,#291313,#291314,#291315,#291316,#291317,
#291318,#291319,#291320,#291321,#291322),.UNSPECIFIED.,.F.,.F.)
B_SPLINE_CURVE_WITH_KNOTS((3,2,2,2,2,2,2,2,2,2,3),(0.740384615384615,0.742307692307692,
0.744230769230769,0.746153846153846,0.748076923076923,0.75,0.751923076923077,
0.753846153846154,0.755769230769231,0.757692307692308,0.759615384615385),
 .UNSPECIFIED.)
CURVE()
GEOMETRIC_REPRESENTATION_ITEM()
RATIONAL_B_SPLINE_CURVE((1.,0.951056516295154,1.,0.951056516295154,1.,0.951056516295154,
1.,0.951056516295154,1.,0.951056516295154,1.,0.951056516295154,1.,0.951056516295154,
1.,0.951056516295154,1.,0.951056516295154,1.,0.951056516295154,1.))
REPRESENTATION_ITEM('')
);
#1656=(
BOUNDED_CURVE()
B_SPLINE_CURVE(2,(#291327,#291328,#291329,#291330,#291331,#291332,#291333,
#291334,#291335,#291336,#291337,#291338,#291339,#291340,#291341,#291342,
#291343,#291344,#291345,#291346,#291347),.UNSPECIFIED.,.F.,.F.)
B_SPLINE_CURVE_WITH_KNOTS((3,2,2,2,2,2,2,2,2,2,3),(0.759615384615385,0.761538461538461,
0.763461538461538,0.765384615384615,0.767307692307692,0.769230769230769,
0.771153846153846,0.773076923076923,0.775,0.776923076923077,0.778846153846154),
 .UNSPECIFIED.)
CURVE()
GEOMETRIC_REPRESENTATION_ITEM()
RATIONAL_B_SPLINE_CURVE((1.,0.951056516295154,1.,0.951056516295154,1.,0.951056516295154,
1.,0.951056516295154,1.,0.951056516295154,1.,0.951056516295154,1.,0.951056516295154,
1.,0.951056516295154,1.,0.951056516295154,1.,0.951056516295154,1.))
REPRESENTATION_ITEM('')
);
#1657=(
BOUNDED_CURVE()
B_SPLINE_CURVE(2,(#291348,#291349,#291350,#291351,#291352,#291353,#291354,
#291355,#291356,#291357,#291358,#291359,#291360,#291361,#291362,#291363,
#291364,#291365,#291366,#291367,#291368),.UNSPECIFIED.,.F.,.F.)
B_SPLINE_CURVE_WITH_KNOTS((3,2,2,2,2,2,2,2,2,2,3),(0.759615384615385,0.761538461538461,
0.763461538461538,0.765384615384615,0.767307692307692,0.769230769230769,
0.771153846153846,0.773076923076923,0.775,0.776923076923077,0.778846153846154),
 .UNSPECIFIED.)
CURVE()
GEOMETRIC_REPRESENTATION_ITEM()
RATIONAL_B_SPLINE_CURVE((1.,0.951056516295154,1.,0.951056516295154,1.,0.951056516295154,
1.,0.951056516295154,1.,0.951056516295154,1.,0.951056516295154,1.,0.951056516295154,
1.,0.951056516295154,1.,0.951056516295154,1.,0.951056516295154,1.))
REPRESENTATION_ITEM('')
);
#1658=(
BOUNDED_CURVE()
B_SPLINE_CURVE(2,(#291373,#291374,#291375,#291376,#291377,#291378,#291379,
#291380,#291381,#291382,#291383,#291384,#291385,#291386,#291387,#291388,
#291389,#291390,#291391,#291392,#291393),.UNSPECIFIED.,.F.,.F.)
B_SPLINE_CURVE_WITH_KNOTS((3,2,2,2,2,2,2,2,2,2,3),(0.778846153846154,0.780769230769231,
0.782692307692308,0.784615384615385,0.786538461538462,0.788461538461538,
0.790384615384615,0.792307692307692,0.794230769230769,0.796153846153846,
0.798076923076923),.UNSPECIFIED.)
CURVE()
GEOMETRIC_REPRESENTATION_ITEM()
RATIONAL_B_SPLINE_CURVE((1.,0.951056516295154,1.,0.951056516295154,1.,0.951056516295154,
1.,0.951056516295154,1.,0.951056516295154,1.,0.951056516295154,1.,0.951056516295154,
1.,0.951056516295154,1.,0.951056516295154,1.,0.951056516295154,1.))
REPRESENTATION_ITEM('')
);
#1659=(
BOUNDED_CURVE()
B_SPLINE_CURVE(2,(#291394,#291395,#291396,#291397,#291398,#291399,#291400,
#291401,#291402,#291403,#291404,#291405,#291406,#291407,#291408,#291409,
#291410,#291411,#291412,#291413,#291414),.UNSPECIFIED.,.F.,.F.)
B_SPLINE_CURVE_WITH_KNOTS((3,2,2,2,2,2,2,2,2,2,3),(0.778846153846154,0.780769230769231,
0.782692307692308,0.784615384615385,0.786538461538462,0.788461538461538,
0.790384615384615,0.792307692307692,0.794230769230769,0.796153846153846,
0.798076923076923),.UNSPECIFIED.)
CURVE()
GEOMETRIC_REPRESENTATION_ITEM()
RATIONAL_B_SPLINE_CURVE((1.,0.951056516295154,1.,0.951056516295154,1.,0.951056516295154,
1.,0.951056516295154,1.,0.951056516295154,1.,0.951056516295154,1.,0.951056516295154,
1.,0.951056516295154,1.,0.951056516295154,1.,0.951056516295154,1.))
REPRESENTATION_ITEM('')
);
#1660=(
BOUNDED_CURVE()
B_SPLINE_CURVE(2,(#291419,#291420,#291421,#291422,#291423,#291424,#291425,
#291426,#291427,#291428,#291429,#291430,#291431,#291432,#291433,#291434,
#291435,#291436,#291437,#291438,#291439),.UNSPECIFIED.,.F.,.F.)
B_SPLINE_CURVE_WITH_KNOTS((3,2,2,2,2,2,2,2,2,2,3),(0.798076923076923,0.8,
0.801923076923077,0.803846153846154,0.805769230769231,0.807692307692308,
0.809615384615385,0.811538461538462,0.813461538461538,0.815384615384615,
0.817307692307692),.UNSPECIFIED.)
CURVE()
GEOMETRIC_REPRESENTATION_ITEM()
RATIONAL_B_SPLINE_CURVE((1.,0.951056516295154,1.,0.951056516295154,1.,0.951056516295154,
1.,0.951056516295154,1.,0.951056516295154,1.,0.951056516295154,1.,0.951056516295154,
1.,0.951056516295154,1.,0.951056516295154,1.,0.951056516295154,1.))
REPRESENTATION_ITEM('')
);
#1661=(
BOUNDED_CURVE()
B_SPLINE_CURVE(2,(#291440,#291441,#291442,#291443,#291444,#291445,#291446,
#291447,#291448,#291449,#291450,#291451,#291452,#291453,#291454,#291455,
#291456,#291457,#291458,#291459,#291460),.UNSPECIFIED.,.F.,.F.)
B_SPLINE_CURVE_WITH_KNOTS((3,2,2,2,2,2,2,2,2,2,3),(0.798076923076923,0.8,
0.801923076923077,0.803846153846154,0.805769230769231,0.807692307692308,
0.809615384615385,0.811538461538462,0.813461538461538,0.815384615384615,
0.817307692307692),.UNSPECIFIED.)
CURVE()
GEOMETRIC_REPRESENTATION_ITEM()
RATIONAL_B_SPLINE_CURVE((1.,0.951056516295154,1.,0.951056516295154,1.,0.951056516295154,
1.,0.951056516295154,1.,0.951056516295154,1.,0.951056516295154,1.,0.951056516295154,
1.,0.951056516295154,1.,0.951056516295154,1.,0.951056516295154,1.))
REPRESENTATION_ITEM('')
);
#1662=(
BOUNDED_CURVE()
B_SPLINE_CURVE(2,(#291465,#291466,#291467,#291468,#291469,#291470,#291471,
#291472,#291473,#291474,#291475,#291476,#291477,#291478,#291479,#291480,
#291481,#291482,#291483,#291484,#291485),.UNSPECIFIED.,.F.,.F.)
B_SPLINE_CURVE_WITH_KNOTS((3,2,2,2,2,2,2,2,2,2,3),(0.817307692307692,0.819230769230769,
0.821153846153846,0.823076923076923,0.825,0.826923076923077,0.828846153846154,
0.830769230769231,0.832692307692308,0.834615384615385,0.836538461538462),
 .UNSPECIFIED.)
CURVE()
GEOMETRIC_REPRESENTATION_ITEM()
RATIONAL_B_SPLINE_CURVE((1.,0.951056516295154,1.,0.951056516295154,1.,0.951056516295154,
1.,0.951056516295154,1.,0.951056516295154,1.,0.951056516295154,1.,0.951056516295154,
1.,0.951056516295154,1.,0.951056516295154,1.,0.951056516295154,1.))
REPRESENTATION_ITEM('')
);
#1663=(
BOUNDED_CURVE()
B_SPLINE_CURVE(2,(#291486,#291487,#291488,#291489,#291490,#291491,#291492,
#291493,#291494,#291495,#291496,#291497,#291498,#291499,#291500,#291501,
#291502,#291503,#291504,#291505,#291506),.UNSPECIFIED.,.F.,.F.)
B_SPLINE_CURVE_WITH_KNOTS((3,2,2,2,2,2,2,2,2,2,3),(0.817307692307692,0.819230769230769,
0.821153846153846,0.823076923076923,0.825,0.826923076923077,0.828846153846154,
0.830769230769231,0.832692307692308,0.834615384615385,0.836538461538462),
 .UNSPECIFIED.)
CURVE()
GEOMETRIC_REPRESENTATION_ITEM()
RATIONAL_B_SPLINE_CURVE((1.,0.951056516295154,1.,0.951056516295154,1.,0.951056516295154,
1.,0.951056516295154,1.,0.951056516295154,1.,0.951056516295154,1.,0.951056516295154,
1.,0.951056516295154,1.,0.951056516295154,1.,0.951056516295154,1.))
REPRESENTATION_ITEM('')
);
#1664=(
BOUNDED_CURVE()
B_SPLINE_CURVE(2,(#296144,#296145,#296146,#296147,#296148,#296149,#296150,
#296151,#296152,#296153,#296154,#296155,#296156,#296157,#296158),
 .UNSPECIFIED.,.F.,.F.)
B_SPLINE_CURVE_WITH_KNOTS((3,2,2,2,2,2,2,3),(0.836538461538462,0.838461538461538,
0.840384615384615,0.842307692307692,0.844230769230769,0.846153846153846,
0.848076923076923,0.849421797849676),.UNSPECIFIED.)
CURVE()
GEOMETRIC_REPRESENTATION_ITEM()
RATIONAL_B_SPLINE_CURVE((1.,0.951056516295154,1.,0.951056516295154,1.,0.951056516295154,
1.,0.951056516295154,1.,0.951056516295154,1.,0.951056516295154,1.,0.965772114606848,
0.979417737587222))
REPRESENTATION_ITEM('')
);
#1665=(
BOUNDED_CURVE()
B_SPLINE_CURVE(2,(#298251,#298252,#298253,#298254,#298255,#298256,#298257,
#298258,#298259,#298260,#298261,#298262,#298263,#298264,#298265,#298266,
#298267),.UNSPECIFIED.,.F.,.F.)
B_SPLINE_CURVE_WITH_KNOTS((3,2,2,2,2,2,2,2,3),(0.836538461538462,0.838461538461538,
0.840384615384615,0.842307692307692,0.844230769230769,0.846153846153846,
0.848076923076923,0.85,0.851829757961637),.UNSPECIFIED.)
CURVE()
GEOMETRIC_REPRESENTATION_ITEM()
RATIONAL_B_SPLINE_CURVE((1.,0.951056516295154,1.,0.951056516295154,1.,0.951056516295154,
1.,0.951056516295154,1.,0.951056516295154,1.,0.951056516295154,1.,0.951056516295154,
1.,0.953431540930822,0.995480450954353))
REPRESENTATION_ITEM('')
);
#1666=(
BOUNDED_CURVE()
B_SPLINE_CURVE(2,(#298312,#298313,#298314),.UNSPECIFIED.,.F.,.F.)
B_SPLINE_CURVE_WITH_KNOTS((3,3),(3.2941320975105,5.33580039117811),
 .UNSPECIFIED.)
CURVE()
GEOMETRIC_REPRESENTATION_ITEM()
RATIONAL_B_SPLINE_CURVE((1.82136720504436,1.96225044864938,1.96225044864938))
REPRESENTATION_ITEM('')
);
#1667=(
BOUNDED_CURVE()
B_SPLINE_CURVE(2,(#298316,#298317,#298318),.UNSPECIFIED.,.F.,.F.)
B_SPLINE_CURVE_WITH_KNOTS((3,3),(5.33580039117811,7.37746868484565),
 .UNSPECIFIED.)
CURVE()
GEOMETRIC_REPRESENTATION_ITEM()
RATIONAL_B_SPLINE_CURVE((1.96225044864938,1.96225044864938,1.82136720504436))
REPRESENTATION_ITEM('')
);
#1668=(
BOUNDED_CURVE()
B_SPLINE_CURVE(2,(#298322,#298323,#298324),.UNSPECIFIED.,.F.,.F.)
B_SPLINE_CURVE_WITH_KNOTS((3,3),(-5.33580039117806,-3.29413209751052),
 .UNSPECIFIED.)
CURVE()
GEOMETRIC_REPRESENTATION_ITEM()
RATIONAL_B_SPLINE_CURVE((1.96225044864938,1.96225044864937,1.82136720504436))
REPRESENTATION_ITEM('')
);
#1669=(
BOUNDED_CURVE()
B_SPLINE_CURVE(2,(#298325,#298326,#298327),.UNSPECIFIED.,.F.,.F.)
B_SPLINE_CURVE_WITH_KNOTS((3,3),(-7.37746868484564,-5.33580039117806),
 .UNSPECIFIED.)
CURVE()
GEOMETRIC_REPRESENTATION_ITEM()
RATIONAL_B_SPLINE_CURVE((1.82136720504435,1.96225044864937,1.96225044864937))
REPRESENTATION_ITEM('')
);
#1670=(
BOUNDED_CURVE()
B_SPLINE_CURVE(2,(#298329,#298330,#298331),.UNSPECIFIED.,.F.,.F.)
B_SPLINE_CURVE_WITH_KNOTS((3,3),(3.29413209751049,5.33580039117809),
 .UNSPECIFIED.)
CURVE()
GEOMETRIC_REPRESENTATION_ITEM()
RATIONAL_B_SPLINE_CURVE((1.82136720504436,1.96225044864938,1.96225044864938))
REPRESENTATION_ITEM('')
);
#1671=(
BOUNDED_CURVE()
B_SPLINE_CURVE(2,(#298333,#298334,#298335),.UNSPECIFIED.,.F.,.F.)
B_SPLINE_CURVE_WITH_KNOTS((3,3),(5.33580039117807,7.37746868484566),
 .UNSPECIFIED.)
CURVE()
GEOMETRIC_REPRESENTATION_ITEM()
RATIONAL_B_SPLINE_CURVE((1.96225044864938,1.96225044864938,1.82136720504436))
REPRESENTATION_ITEM('')
);
#1672=(
BOUNDED_CURVE()
B_SPLINE_CURVE(2,(#298339,#298340,#298341),.UNSPECIFIED.,.F.,.F.)
B_SPLINE_CURVE_WITH_KNOTS((3,3),(-5.33580039117809,-3.29413209751052),
 .UNSPECIFIED.)
CURVE()
GEOMETRIC_REPRESENTATION_ITEM()
RATIONAL_B_SPLINE_CURVE((1.96225044864938,1.96225044864938,1.82136720504436))
REPRESENTATION_ITEM('')
);
#1673=(
BOUNDED_CURVE()
B_SPLINE_CURVE(2,(#298342,#298343,#298344),.UNSPECIFIED.,.F.,.F.)
B_SPLINE_CURVE_WITH_KNOTS((3,3),(-7.37746868484567,-5.33580039117808),
 .UNSPECIFIED.)
CURVE()
GEOMETRIC_REPRESENTATION_ITEM()
RATIONAL_B_SPLINE_CURVE((1.82136720504436,1.96225044864939,1.96225044864939))
REPRESENTATION_ITEM('')
);
#1674=(
BOUNDED_CURVE()
B_SPLINE_CURVE(2,(#298346,#298347,#298348),.UNSPECIFIED.,.F.,.F.)
B_SPLINE_CURVE_WITH_KNOTS((3,3),(3.2941320975105,5.33580039117809),
 .UNSPECIFIED.)
CURVE()
GEOMETRIC_REPRESENTATION_ITEM()
RATIONAL_B_SPLINE_CURVE((1.82136720504437,1.9622504486494,1.9622504486494))
REPRESENTATION_ITEM('')
);
#1675=(
BOUNDED_CURVE()
B_SPLINE_CURVE(2,(#298350,#298351,#298352),.UNSPECIFIED.,.F.,.F.)
B_SPLINE_CURVE_WITH_KNOTS((3,3),(5.33580039117805,7.37746868484568),
 .UNSPECIFIED.)
CURVE()
GEOMETRIC_REPRESENTATION_ITEM()
RATIONAL_B_SPLINE_CURVE((1.96225044864939,1.9622504486494,1.82136720504437))
REPRESENTATION_ITEM('')
);
#1676=(
BOUNDED_CURVE()
B_SPLINE_CURVE(2,(#298356,#298357,#298358),.UNSPECIFIED.,.F.,.F.)
B_SPLINE_CURVE_WITH_KNOTS((3,3),(-5.33580039117813,-3.29413209751052),
 .UNSPECIFIED.)
CURVE()
GEOMETRIC_REPRESENTATION_ITEM()
RATIONAL_B_SPLINE_CURVE((1.96225044864939,1.96225044864939,1.82136720504437))
REPRESENTATION_ITEM('')
);
#1677=(
BOUNDED_CURVE()
B_SPLINE_CURVE(2,(#298359,#298360,#298361),.UNSPECIFIED.,.F.,.F.)
B_SPLINE_CURVE_WITH_KNOTS((3,3),(-7.37746868484571,-5.33580039117813),
 .UNSPECIFIED.)
CURVE()
GEOMETRIC_REPRESENTATION_ITEM()
RATIONAL_B_SPLINE_CURVE((1.82136720504437,1.96225044864939,1.96225044864939))
REPRESENTATION_ITEM('')
);
#1678=(
BOUNDED_CURVE()
B_SPLINE_CURVE(2,(#298363,#298364,#298365),.UNSPECIFIED.,.F.,.F.)
B_SPLINE_CURVE_WITH_KNOTS((3,3),(3.29413209751053,5.33580039117809),
 .UNSPECIFIED.)
CURVE()
GEOMETRIC_REPRESENTATION_ITEM()
RATIONAL_B_SPLINE_CURVE((1.82136720504437,1.96225044864939,1.96225044864939))
REPRESENTATION_ITEM('')
);
#1679=(
BOUNDED_CURVE()
B_SPLINE_CURVE(2,(#298367,#298368,#298369),.UNSPECIFIED.,.F.,.F.)
B_SPLINE_CURVE_WITH_KNOTS((3,3),(5.33580039117809,7.37746868484569),
 .UNSPECIFIED.)
CURVE()
GEOMETRIC_REPRESENTATION_ITEM()
RATIONAL_B_SPLINE_CURVE((1.96225044864938,1.96225044864938,1.82136720504436))
REPRESENTATION_ITEM('')
);
#1680=(
BOUNDED_CURVE()
B_SPLINE_CURVE(2,(#298373,#298374,#298375),.UNSPECIFIED.,.F.,.F.)
B_SPLINE_CURVE_WITH_KNOTS((3,3),(-5.33580039117811,-3.2941320975105),
 .UNSPECIFIED.)
CURVE()
GEOMETRIC_REPRESENTATION_ITEM()
RATIONAL_B_SPLINE_CURVE((1.96225044864939,1.96225044864939,1.82136720504437))
REPRESENTATION_ITEM('')
);
#1681=(
BOUNDED_CURVE()
B_SPLINE_CURVE(2,(#298376,#298377,#298378),.UNSPECIFIED.,.F.,.F.)
B_SPLINE_CURVE_WITH_KNOTS((3,3),(-7.37746868484567,-5.33580039117811),
 .UNSPECIFIED.)
CURVE()
GEOMETRIC_REPRESENTATION_ITEM()
RATIONAL_B_SPLINE_CURVE((1.82136720504437,1.96225044864939,1.96225044864939))
REPRESENTATION_ITEM('')
);
#1682=(
BOUNDED_CURVE()
B_SPLINE_CURVE(2,(#298380,#298381,#298382),.UNSPECIFIED.,.F.,.F.)
B_SPLINE_CURVE_WITH_KNOTS((3,3),(3.29413209751053,5.33580039117807),
 .UNSPECIFIED.)
CURVE()
GEOMETRIC_REPRESENTATION_ITEM()
RATIONAL_B_SPLINE_CURVE((1.82136720504437,1.96225044864938,1.96225044864938))
REPRESENTATION_ITEM('')
);
#1683=(
BOUNDED_CURVE()
B_SPLINE_CURVE(2,(#298384,#298385,#298386),.UNSPECIFIED.,.F.,.F.)
B_SPLINE_CURVE_WITH_KNOTS((3,3),(5.33580039117811,7.37746868484569),
 .UNSPECIFIED.)
CURVE()
GEOMETRIC_REPRESENTATION_ITEM()
RATIONAL_B_SPLINE_CURVE((1.96225044864938,1.96225044864938,1.82136720504436))
REPRESENTATION_ITEM('')
);
#1684=(
BOUNDED_CURVE()
B_SPLINE_CURVE(2,(#298390,#298391,#298392),.UNSPECIFIED.,.F.,.F.)
B_SPLINE_CURVE_WITH_KNOTS((3,3),(-5.33580039117809,-3.2941320975105),
 .UNSPECIFIED.)
CURVE()
GEOMETRIC_REPRESENTATION_ITEM()
RATIONAL_B_SPLINE_CURVE((1.96225044864938,1.96225044864938,1.82136720504436))
REPRESENTATION_ITEM('')
);
#1685=(
BOUNDED_CURVE()
B_SPLINE_CURVE(2,(#298393,#298394,#298395),.UNSPECIFIED.,.F.,.F.)
B_SPLINE_CURVE_WITH_KNOTS((3,3),(-7.37746868484566,-5.3358003911781),
 .UNSPECIFIED.)
CURVE()
GEOMETRIC_REPRESENTATION_ITEM()
RATIONAL_B_SPLINE_CURVE((1.82136720504436,1.96225044864938,1.96225044864938))
REPRESENTATION_ITEM('')
);
#1686=(
BOUNDED_CURVE()
B_SPLINE_CURVE(2,(#298397,#298398,#298399),.UNSPECIFIED.,.F.,.F.)
B_SPLINE_CURVE_WITH_KNOTS((3,3),(3.29413209751053,5.33580039117807),
 .UNSPECIFIED.)
CURVE()
GEOMETRIC_REPRESENTATION_ITEM()
RATIONAL_B_SPLINE_CURVE((1.82136720504436,1.96225044864937,1.96225044864937))
REPRESENTATION_ITEM('')
);
#1687=(
BOUNDED_CURVE()
B_SPLINE_CURVE(2,(#298400,#298401,#298402),.UNSPECIFIED.,.F.,.F.)
B_SPLINE_CURVE_WITH_KNOTS((3,3),(5.33580039117807,7.37746868484566),
 .UNSPECIFIED.)
CURVE()
GEOMETRIC_REPRESENTATION_ITEM()
RATIONAL_B_SPLINE_CURVE((1.96225044864937,1.96225044864937,1.82136720504435))
REPRESENTATION_ITEM('')
);
#1688=(
BOUNDED_CURVE()
B_SPLINE_CURVE(2,(#298404,#298405,#298406),.UNSPECIFIED.,.F.,.F.)
B_SPLINE_CURVE_WITH_KNOTS((3,3),(-5.33580039117805,-3.29413209751049),
 .UNSPECIFIED.)
CURVE()
GEOMETRIC_REPRESENTATION_ITEM()
RATIONAL_B_SPLINE_CURVE((1.96225044864937,1.96225044864937,1.82136720504435))
REPRESENTATION_ITEM('')
);
#1689=(
BOUNDED_CURVE()
B_SPLINE_CURVE(2,(#298407,#298408,#298409),.UNSPECIFIED.,.F.,.F.)
B_SPLINE_CURVE_WITH_KNOTS((3,3),(-7.37746868484564,-5.33580039117806),
 .UNSPECIFIED.)
CURVE()
GEOMETRIC_REPRESENTATION_ITEM()
RATIONAL_B_SPLINE_CURVE((1.82136720504436,1.96225044864938,1.96225044864938))
REPRESENTATION_ITEM('')
);
#1690=(
BOUNDED_CURVE()
B_SPLINE_CURVE(2,(#300536,#300537,#300538,#300539,#300540),
 .UNSPECIFIED.,.F.,.F.)
B_SPLINE_CURVE_WITH_KNOTS((3,2,3),(0.394230769230769,0.396153846153846,
0.396753325815344),.UNSPECIFIED.)
CURVE()
GEOMETRIC_REPRESENTATION_ITEM()
RATIONAL_B_SPLINE_CURVE((1.,0.951056516295154,1.,0.984742876017165,0.978997940975819))
REPRESENTATION_ITEM('')
);
#1691=(
BOUNDED_CURVE()
B_SPLINE_CURVE(2,(#302615,#302616,#302617,#302618,#302619,#302620,#302621),
 .UNSPECIFIED.,.F.,.F.)
B_SPLINE_CURVE_WITH_KNOTS((3,2,2,3),(0.394230769230769,0.396153846153846,
0.398076923076923,0.399146724305703),.UNSPECIFIED.)
CURVE()
GEOMETRIC_REPRESENTATION_ITEM()
RATIONAL_B_SPLINE_CURVE((1.,0.951056516295154,1.,0.951056516295154,1.,0.972772904515738,
0.975838492444844))
REPRESENTATION_ITEM('')
);
#3192=(
BOUNDED_SURFACE()
B_SPLINE_SURFACE(1,2,((#276452,#276453,#276454,#276455,#276456,#276457,
#276458,#276459,#276460,#276461,#276462,#276463,#276464,#276465,#276466,
#276467,#276468,#276469,#276470,#276471,#276472,#276473,#276474,#276475,
#276476,#276477,#276478,#276479,#276480,#276481,#276482,#276483,#276484,
#276485,#276486,#276487,#276488,#276489,#276490,#276491,#276492,#276493,
#276494,#276495,#276496,#276497,#276498,#276499,#276500,#276501,#276502,
#276503,#276504,#276505,#276506,#276507,#276508,#276509,#276510,#276511,
#276512,#276513,#276514,#276515,#276516,#276517,#276518,#276519,#276520,
#276521,#276522,#276523,#276524,#276525,#276526,#276527,#276528,#276529,
#276530,#276531,#276532,#276533,#276534,#276535,#276536,#276537,#276538,
#276539,#276540,#276541,#276542,#276543,#276544,#276545,#276546,#276547,
#276548,#276549,#276550,#276551,#276552,#276553,#276554,#276555,#276556,
#276557,#276558,#276559,#276560,#276561,#276562,#276563,#276564,#276565,
#276566,#276567,#276568,#276569,#276570,#276571,#276572,#276573,#276574,
#276575,#276576,#276577,#276578,#276579,#276580,#276581,#276582,#276583,
#276584,#276585,#276586,#276587,#276588,#276589,#276590,#276591,#276592,
#276593,#276594,#276595,#276596,#276597,#276598,#276599,#276600,#276601,
#276602,#276603,#276604,#276605,#276606,#276607,#276608,#276609,#276610,
#276611,#276612,#276613,#276614,#276615,#276616,#276617,#276618,#276619,
#276620,#276621,#276622,#276623,#276624,#276625,#276626,#276627,#276628,
#276629,#276630,#276631,#276632,#276633,#276634,#276635,#276636,#276637,
#276638,#276639,#276640,#276641,#276642,#276643,#276644,#276645,#276646,
#276647,#276648,#276649,#276650,#276651,#276652,#276653,#276654,#276655,
#276656,#276657,#276658,#276659,#276660,#276661,#276662,#276663,#276664,
#276665,#276666,#276667,#276668,#276669,#276670,#276671,#276672,#276673,
#276674,#276675,#276676,#276677,#276678,#276679,#276680,#276681,#276682,
#276683,#276684,#276685,#276686,#276687,#276688,#276689,#276690,#276691,
#276692,#276693,#276694,#276695,#276696,#276697,#276698,#276699,#276700,
#276701,#276702,#276703,#276704,#276705,#276706,#276707,#276708,#276709,
#276710,#276711,#276712,#276713,#276714,#276715,#276716,#276717,#276718,
#276719,#276720,#276721,#276722,#276723,#276724,#276725,#276726,#276727,
#276728,#276729,#276730,#276731,#276732,#276733,#276734,#276735,#276736,
#276737,#276738,#276739,#276740,#276741,#276742,#276743,#276744,#276745,
#276746,#276747,#276748,#276749,#276750,#276751,#276752,#276753,#276754,
#276755,#276756,#276757,#276758,#276759,#276760,#276761,#276762,#276763,
#276764,#276765,#276766,#276767,#276768,#276769,#276770,#276771,#276772,
#276773,#276774,#276775,#276776,#276777,#276778,#276779,#276780,#276781,
#276782,#276783,#276784,#276785,#276786,#276787,#276788,#276789,#276790,
#276791,#276792,#276793,#276794,#276795,#276796,#276797,#276798,#276799,
#276800,#276801,#276802,#276803,#276804,#276805,#276806,#276807,#276808,
#276809,#276810,#276811,#276812,#276813,#276814,#276815,#276816,#276817,
#276818,#276819,#276820,#276821,#276822,#276823,#276824,#276825,#276826,
#276827,#276828,#276829,#276830,#276831,#276832,#276833,#276834,#276835,
#276836,#276837,#276838,#276839,#276840,#276841,#276842,#276843,#276844,
#276845,#276846,#276847,#276848,#276849,#276850,#276851,#276852,#276853,
#276854,#276855,#276856,#276857,#276858,#276859,#276860,#276861,#276862,
#276863,#276864,#276865,#276866,#276867,#276868,#276869,#276870,#276871,
#276872,#276873,#276874,#276875,#276876,#276877,#276878,#276879,#276880,
#276881,#276882,#276883,#276884,#276885,#276886,#276887,#276888,#276889,
#276890,#276891,#276892,#276893,#276894,#276895,#276896,#276897,#276898,
#276899,#276900,#276901,#276902,#276903,#276904,#276905,#276906,#276907,
#276908,#276909,#276910,#276911,#276912,#276913,#276914,#276915,#276916,
#276917,#276918,#276919,#276920,#276921,#276922,#276923,#276924,#276925,
#276926,#276927,#276928,#276929,#276930,#276931,#276932,#276933,#276934,
#276935,#276936,#276937,#276938,#276939,#276940,#276941,#276942,#276943,
#276944,#276945,#276946,#276947,#276948,#276949,#276950,#276951,#276952,
#276953,#276954,#276955,#276956,#276957,#276958,#276959,#276960,#276961,
#276962,#276963,#276964,#276965,#276966,#276967,#276968,#276969,#276970,
#276971,#276972,#276973,#276974,#276975,#276976,#276977,#276978,#276979,
#276980,#276981,#276982,#276983,#276984,#276985,#276986,#276987,#276988,
#276989,#276990,#276991,#276992,#276993,#276994,#276995,#276996,#276997,
#276998,#276999,#277000,#277001,#277002,#277003,#277004,#277005,#277006,
#277007,#277008,#277009,#277010,#277011,#277012,#277013,#277014,#277015,
#277016,#277017,#277018,#277019,#277020,#277021,#277022,#277023,#277024,
#277025,#277026,#277027,#277028,#277029,#277030,#277031,#277032,#277033,
#277034,#277035,#277036,#277037,#277038,#277039,#277040,#277041,#277042,
#277043,#277044,#277045,#277046,#277047,#277048,#277049,#277050,#277051,
#277052,#277053,#277054,#277055,#277056,#277057,#277058,#277059,#277060,
#277061,#277062,#277063,#277064,#277065,#277066,#277067,#277068,#277069,
#277070,#277071,#277072,#277073,#277074,#277075,#277076,#277077,#277078,
#277079,#277080,#277081,#277082,#277083,#277084,#277085,#277086,#277087,
#277088,#277089,#277090,#277091,#277092,#277093,#277094,#277095,#277096,
#277097,#277098,#277099,#277100,#277101,#277102,#277103,#277104,#277105,
#277106,#277107,#277108,#277109,#277110,#277111,#277112,#277113,#277114,
#277115,#277116,#277117,#277118,#277119,#277120,#277121,#277122,#277123,
#277124,#277125,#277126,#277127,#277128,#277129,#277130,#277131,#277132,
#277133,#277134,#277135,#277136,#277137,#277138,#277139,#277140,#277141,
#277142,#277143,#277144,#277145,#277146,#277147,#277148,#277149,#277150,
#277151,#277152,#277153,#277154,#277155,#277156,#277157,#277158,#277159,
#277160,#277161,#277162,#277163,#277164,#277165,#277166,#277167,#277168,
#277169,#277170,#277171,#277172,#277173,#277174,#277175,#277176,#277177,
#277178,#277179,#277180,#277181,#277182,#277183,#277184,#277185,#277186,
#277187,#277188,#277189,#277190,#277191,#277192,#277193,#277194,#277195,
#277196,#277197,#277198,#277199,#277200,#277201,#277202,#277203,#277204,
#277205,#277206,#277207,#277208,#277209,#277210,#277211,#277212,#277213,
#277214,#277215,#277216,#277217,#277218,#277219,#277220,#277221,#277222,
#277223,#277224,#277225,#277226,#277227,#277228,#277229,#277230,#277231,
#277232,#277233,#277234,#277235,#277236,#277237,#277238,#277239,#277240,
#277241,#277242,#277243,#277244,#277245,#277246,#277247,#277248,#277249,
#277250,#277251,#277252,#277253,#277254,#277255,#277256,#277257,#277258,
#277259,#277260,#277261,#277262,#277263,#277264,#277265,#277266,#277267,
#277268,#277269,#277270,#277271,#277272,#277273,#277274,#277275,#277276,
#277277,#277278,#277279,#277280,#277281,#277282,#277283,#277284,#277285,
#277286,#277287,#277288,#277289,#277290,#277291,#277292,#277293,#277294,
#277295,#277296,#277297,#277298,#277299,#277300,#277301,#277302,#277303,
#277304,#277305,#277306,#277307,#277308,#277309,#277310,#277311,#277312,
#277313,#277314,#277315,#277316,#277317,#277318,#277319,#277320,#277321,
#277322,#277323,#277324,#277325,#277326,#277327,#277328,#277329,#277330,
#277331,#277332,#277333,#277334,#277335,#277336,#277337,#277338,#277339,
#277340,#277341,#277342,#277343,#277344,#277345,#277346,#277347,#277348,
#277349,#277350,#277351,#277352,#277353,#277354,#277355,#277356,#277357,
#277358,#277359,#277360,#277361,#277362,#277363,#277364,#277365,#277366,
#277367,#277368,#277369,#277370,#277371,#277372,#277373,#277374,#277375,
#277376,#277377,#277378,#277379,#277380,#277381,#277382,#277383,#277384,
#277385,#277386,#277387,#277388,#277389,#277390,#277391,#277392,#277393,
#277394,#277395,#277396,#277397,#277398,#277399,#277400,#277401,#277402,
#277403,#277404,#277405,#277406,#277407,#277408,#277409,#277410,#277411,
#277412,#277413,#277414,#277415,#277416,#277417,#277418,#277419,#277420,
#277421,#277422,#277423,#277424,#277425,#277426,#277427,#277428,#277429,
#277430,#277431,#277432,#277433,#277434,#277435,#277436,#277437,#277438,
#277439,#277440,#277441,#277442,#277443,#277444,#277445,#277446,#277447,
#277448,#277449,#277450,#277451,#277452,#277453,#277454,#277455,#277456,
#277457,#277458,#277459,#277460,#277461,#277462,#277463,#277464,#277465,
#277466,#277467,#277468,#277469,#277470,#277471,#277472,#277473,#277474,
#277475,#277476,#277477,#277478,#277479,#277480,#277481,#277482,#277483,
#277484,#277485,#277486,#277487,#277488),(#277489,#277490,#277491,#277492,
#277493,#277494,#277495,#277496,#277497,#277498,#277499,#277500,#277501,
#277502,#277503,#277504,#277505,#277506,#277507,#277508,#277509,#277510,
#277511,#277512,#277513,#277514,#277515,#277516,#277517,#277518,#277519,
#277520,#277521,#277522,#277523,#277524,#277525,#277526,#277527,#277528,
#277529,#277530,#277531,#277532,#277533,#277534,#277535,#277536,#277537,
#277538,#277539,#277540,#277541,#277542,#277543,#277544,#277545,#277546,
#277547,#277548,#277549,#277550,#277551,#277552,#277553,#277554,#277555,
#277556,#277557,#277558,#277559,#277560,#277561,#277562,#277563,#277564,
#277565,#277566,#277567,#277568,#277569,#277570,#277571,#277572,#277573,
#277574,#277575,#277576,#277577,#277578,#277579,#277580,#277581,#277582,
#277583,#277584,#277585,#277586,#277587,#277588,#277589,#277590,#277591,
#277592,#277593,#277594,#277595,#277596,#277597,#277598,#277599,#277600,
#277601,#277602,#277603,#277604,#277605,#277606,#277607,#277608,#277609,
#277610,#277611,#277612,#277613,#277614,#277615,#277616,#277617,#277618,
#277619,#277620,#277621,#277622,#277623,#277624,#277625,#277626,#277627,
#277628,#277629,#277630,#277631,#277632,#277633,#277634,#277635,#277636,
#277637,#277638,#277639,#277640,#277641,#277642,#277643,#277644,#277645,
#277646,#277647,#277648,#277649,#277650,#277651,#277652,#277653,#277654,
#277655,#277656,#277657,#277658,#277659,#277660,#277661,#277662,#277663,
#277664,#277665,#277666,#277667,#277668,#277669,#277670,#277671,#277672,
#277673,#277674,#277675,#277676,#277677,#277678,#277679,#277680,#277681,
#277682,#277683,#277684,#277685,#277686,#277687,#277688,#277689,#277690,
#277691,#277692,#277693,#277694,#277695,#277696,#277697,#277698,#277699,
#277700,#277701,#277702,#277703,#277704,#277705,#277706,#277707,#277708,
#277709,#277710,#277711,#277712,#277713,#277714,#277715,#277716,#277717,
#277718,#277719,#277720,#277721,#277722,#277723,#277724,#277725,#277726,
#277727,#277728,#277729,#277730,#277731,#277732,#277733,#277734,#277735,
#277736,#277737,#277738,#277739,#277740,#277741,#277742,#277743,#277744,
#277745,#277746,#277747,#277748,#277749,#277750,#277751,#277752,#277753,
#277754,#277755,#277756,#277757,#277758,#277759,#277760,#277761,#277762,
#277763,#277764,#277765,#277766,#277767,#277768,#277769,#277770,#277771,
#277772,#277773,#277774,#277775,#277776,#277777,#277778,#277779,#277780,
#277781,#277782,#277783,#277784,#277785,#277786,#277787,#277788,#277789,
#277790,#277791,#277792,#277793,#277794,#277795,#277796,#277797,#277798,
#277799,#277800,#277801,#277802,#277803,#277804,#277805,#277806,#277807,
#277808,#277809,#277810,#277811,#277812,#277813,#277814,#277815,#277816,
#277817,#277818,#277819,#277820,#277821,#277822,#277823,#277824,#277825,
#277826,#277827,#277828,#277829,#277830,#277831,#277832,#277833,#277834,
#277835,#277836,#277837,#277838,#277839,#277840,#277841,#277842,#277843,
#277844,#277845,#277846,#277847,#277848,#277849,#277850,#277851,#277852,
#277853,#277854,#277855,#277856,#277857,#277858,#277859,#277860,#277861,
#277862,#277863,#277864,#277865,#277866,#277867,#277868,#277869,#277870,
#277871,#277872,#277873,#277874,#277875,#277876,#277877,#277878,#277879,
#277880,#277881,#277882,#277883,#277884,#277885,#277886,#277887,#277888,
#277889,#277890,#277891,#277892,#277893,#277894,#277895,#277896,#277897,
#277898,#277899,#277900,#277901,#277902,#277903,#277904,#277905,#277906,
#277907,#277908,#277909,#277910,#277911,#277912,#277913,#277914,#277915,
#277916,#277917,#277918,#277919,#277920,#277921,#277922,#277923,#277924,
#277925,#277926,#277927,#277928,#277929,#277930,#277931,#277932,#277933,
#277934,#277935,#277936,#277937,#277938,#277939,#277940,#277941,#277942,
#277943,#277944,#277945,#277946,#277947,#277948,#277949,#277950,#277951,
#277952,#277953,#277954,#277955,#277956,#277957,#277958,#277959,#277960,
#277961,#277962,#277963,#277964,#277965,#277966,#277967,#277968,#277969,
#277970,#277971,#277972,#277973,#277974,#277975,#277976,#277977,#277978,
#277979,#277980,#277981,#277982,#277983,#277984,#277985,#277986,#277987,
#277988,#277989,#277990,#277991,#277992,#277993,#277994,#277995,#277996,
#277997,#277998,#277999,#278000,#278001,#278002,#278003,#278004,#278005,
#278006,#278007,#278008,#278009,#278010,#278011,#278012,#278013,#278014,
#278015,#278016,#278017,#278018,#278019,#278020,#278021,#278022,#278023,
#278024,#278025,#278026,#278027,#278028,#278029,#278030,#278031,#278032,
#278033,#278034,#278035,#278036,#278037,#278038,#278039,#278040,#278041,
#278042,#278043,#278044,#278045,#278046,#278047,#278048,#278049,#278050,
#278051,#278052,#278053,#278054,#278055,#278056,#278057,#278058,#278059,
#278060,#278061,#278062,#278063,#278064,#278065,#278066,#278067,#278068,
#278069,#278070,#278071,#278072,#278073,#278074,#278075,#278076,#278077,
#278078,#278079,#278080,#278081,#278082,#278083,#278084,#278085,#278086,
#278087,#278088,#278089,#278090,#278091,#278092,#278093,#278094,#278095,
#278096,#278097,#278098,#278099,#278100,#278101,#278102,#278103,#278104,
#278105,#278106,#278107,#278108,#278109,#278110,#278111,#278112,#278113,
#278114,#278115,#278116,#278117,#278118,#278119,#278120,#278121,#278122,
#278123,#278124,#278125,#278126,#278127,#278128,#278129,#278130,#278131,
#278132,#278133,#278134,#278135,#278136,#278137,#278138,#278139,#278140,
#278141,#278142,#278143,#278144,#278145,#278146,#278147,#278148,#278149,
#278150,#278151,#278152,#278153,#278154,#278155,#278156,#278157,#278158,
#278159,#278160,#278161,#278162,#278163,#278164,#278165,#278166,#278167,
#278168,#278169,#278170,#278171,#278172,#278173,#278174,#278175,#278176,
#278177,#278178,#278179,#278180,#278181,#278182,#278183,#278184,#278185,
#278186,#278187,#278188,#278189,#278190,#278191,#278192,#278193,#278194,
#278195,#278196,#278197,#278198,#278199,#278200,#278201,#278202,#278203,
#278204,#278205,#278206,#278207,#278208,#278209,#278210,#278211,#278212,
#278213,#278214,#278215,#278216,#278217,#278218,#278219,#278220,#278221,
#278222,#278223,#278224,#278225,#278226,#278227,#278228,#278229,#278230,
#278231,#278232,#278233,#278234,#278235,#278236,#278237,#278238,#278239,
#278240,#278241,#278242,#278243,#278244,#278245,#278246,#278247,#278248,
#278249,#278250,#278251,#278252,#278253,#278254,#278255,#278256,#278257,
#278258,#278259,#278260,#278261,#278262,#278263,#278264,#278265,#278266,
#278267,#278268,#278269,#278270,#278271,#278272,#278273,#278274,#278275,
#278276,#278277,#278278,#278279,#278280,#278281,#278282,#278283,#278284,
#278285,#278286,#278287,#278288,#278289,#278290,#278291,#278292,#278293,
#278294,#278295,#278296,#278297,#278298,#278299,#278300,#278301,#278302,
#278303,#278304,#278305,#278306,#278307,#278308,#278309,#278310,#278311,
#278312,#278313,#278314,#278315,#278316,#278317,#278318,#278319,#278320,
#278321,#278322,#278323,#278324,#278325,#278326,#278327,#278328,#278329,
#278330,#278331,#278332,#278333,#278334,#278335,#278336,#278337,#278338,
#278339,#278340,#278341,#278342,#278343,#278344,#278345,#278346,#278347,
#278348,#278349,#278350,#278351,#278352,#278353,#278354,#278355,#278356,
#278357,#278358,#278359,#278360,#278361,#278362,#278363,#278364,#278365,
#278366,#278367,#278368,#278369,#278370,#278371,#278372,#278373,#278374,
#278375,#278376,#278377,#278378,#278379,#278380,#278381,#278382,#278383,
#278384,#278385,#278386,#278387,#278388,#278389,#278390,#278391,#278392,
#278393,#278394,#278395,#278396,#278397,#278398,#278399,#278400,#278401,
#278402,#278403,#278404,#278405,#278406,#278407,#278408,#278409,#278410,
#278411,#278412,#278413,#278414,#278415,#278416,#278417,#278418,#278419,
#278420,#278421,#278422,#278423,#278424,#278425,#278426,#278427,#278428,
#278429,#278430,#278431,#278432,#278433,#278434,#278435,#278436,#278437,
#278438,#278439,#278440,#278441,#278442,#278443,#278444,#278445,#278446,
#278447,#278448,#278449,#278450,#278451,#278452,#278453,#278454,#278455,
#278456,#278457,#278458,#278459,#278460,#278461,#278462,#278463,#278464,
#278465,#278466,#278467,#278468,#278469,#278470,#278471,#278472,#278473,
#278474,#278475,#278476,#278477,#278478,#278479,#278480,#278481,#278482,
#278483,#278484,#278485,#278486,#278487,#278488,#278489,#278490,#278491,
#278492,#278493,#278494,#278495,#278496,#278497,#278498,#278499,#278500,
#278501,#278502,#278503,#278504,#278505,#278506,#278507,#278508,#278509,
#278510,#278511,#278512,#278513,#278514,#278515,#278516,#278517,#278518,
#278519,#278520,#278521,#278522,#278523,#278524,#278525)),.UNSPECIFIED.,
 .F.,.F.,.F.)
B_SPLINE_SURFACE_WITH_KNOTS((2,2),(3,2,2,2,2,2,2,2,2,2,2,2,2,2,2,2,2,2,
2,2,2,2,2,2,2,2,2,2,2,2,2,2,2,2,2,2,2,2,2,2,2,2,2,2,2,2,2,2,2,2,2,2,2,2,
2,2,2,2,2,2,2,2,2,2,2,2,2,2,2,2,2,2,2,2,2,2,2,2,2,2,2,2,2,2,2,2,2,2,2,2,
2,2,2,2,2,2,2,2,2,2,2,2,2,2,2,2,2,2,2,2,2,2,2,2,2,2,2,2,2,2,2,2,2,2,2,2,
2,2,2,2,2,2,2,2,2,2,2,2,2,2,2,2,2,2,2,2,2,2,2,2,2,2,2,2,2,2,2,2,2,2,2,2,
2,2,2,2,2,2,2,2,2,2,2,2,2,2,2,2,2,2,2,2,2,2,2,2,2,2,2,2,2,2,2,2,2,2,2,2,
2,2,2,2,2,2,2,2,2,2,2,2,2,2,2,2,2,2,2,2,2,2,2,2,2,2,2,2,2,2,2,2,2,2,2,2,
2,2,2,2,2,2,2,2,2,2,2,2,2,2,2,2,2,2,2,2,2,2,2,2,2,2,2,2,2,2,2,2,2,2,2,2,
2,2,2,2,2,2,2,2,2,2,2,2,2,2,2,2,2,2,2,2,2,2,2,2,2,2,2,2,2,2,2,2,2,2,2,2,
2,2,2,2,2,2,2,2,2,2,2,2,2,2,2,2,2,2,2,2,2,2,2,2,2,2,2,2,2,2,2,2,2,2,2,2,
2,2,2,2,2,2,2,2,2,2,2,2,2,2,2,2,2,2,2,2,2,2,2,2,2,2,2,2,2,2,2,2,2,2,2,2,
2,2,2,2,2,2,2,2,2,2,2,2,2,2,2,2,2,2,2,2,2,2,2,2,2,2,2,2,2,2,2,2,2,2,2,2,
2,2,2,2,2,2,2,2,2,2,2,2,2,2,2,2,2,2,2,2,2,2,2,2,2,2,2,2,2,2,2,2,2,2,2,2,
2,2,2,2,2,2,2,2,2,2,2,2,2,2,2,2,2,2,2,2,2,2,2,2,2,2,2,2,2,2,2,2,2,2,2,2,
2,2,2,2,2,2,2,2,2,2,2,2,2,2,2,2,2,2,2,2,2,2,2,2,2,2,2,2,2,2,2,2,3),(-2.04414063882605E-6,
1.),(0.,0.00192307692307692,0.00384615384615385,0.00576923076923077,0.00769230769230769,
0.00961538461538462,0.0115384615384615,0.0134615384615385,0.0153846153846154,
0.0173076923076923,0.0192307692307692,0.0211538461538462,0.0230769230769231,
0.025,0.0269230769230769,0.0288461538461538,0.0307692307692308,0.0326923076923077,
0.0346153846153846,0.0365384615384615,0.0384615384615385,0.0403846153846154,
0.0423076923076923,0.0442307692307692,0.0461538461538462,0.0480769230769231,
0.05,0.0519230769230769,0.0538461538461538,0.0557692307692308,0.0576923076923077,
0.0596153846153846,0.0615384615384615,0.0634615384615385,0.0653846153846154,
0.0673076923076923,0.0692307692307692,0.0711538461538462,0.0730769230769231,
0.075,0.0769230769230769,0.0788461538461538,0.0807692307692308,0.0826923076923077,
0.0846153846153846,0.0865384615384615,0.0884615384615385,0.0903846153846154,
0.0923076923076923,0.0942307692307692,0.0961538461538462,0.0980769230769231,
0.1,0.101923076923077,0.103846153846154,0.105769230769231,0.107692307692308,
0.109615384615385,0.111538461538462,0.113461538461538,0.115384615384615,
0.117307692307692,0.119230769230769,0.121153846153846,0.123076923076923,
0.125,0.126923076923077,0.128846153846154,0.130769230769231,0.132692307692308,
0.134615384615385,0.136538461538462,0.138461538461538,0.140384615384615,
0.142307692307692,0.144230769230769,0.146153846153846,0.148076923076923,
0.15,0.151923076923077,0.153846153846154,0.155769230769231,0.157692307692308,
0.159615384615385,0.161538461538462,0.163461538461538,0.165384615384615,
0.167307692307692,0.169230769230769,0.171153846153846,0.173076923076923,
0.175,0.176923076923077,0.178846153846154,0.180769230769231,0.182692307692308,
0.184615384615385,0.186538461538462,0.188461538461538,0.190384615384615,
0.192307692307692,0.194230769230769,0.196153846153846,0.198076923076923,
0.2,0.201923076923077,0.203846153846154,0.205769230769231,0.207692307692308,
0.209615384615385,0.211538461538462,0.213461538461538,0.215384615384615,
0.217307692307692,0.219230769230769,0.221153846153846,0.223076923076923,
0.225,0.226923076923077,0.228846153846154,0.230769230769231,0.232692307692308,
0.234615384615385,0.236538461538462,0.238461538461538,0.240384615384615,
0.242307692307692,0.244230769230769,0.246153846153846,0.248076923076923,
0.25,0.251923076923077,0.253846153846154,0.255769230769231,0.257692307692308,
0.259615384615385,0.261538461538462,0.263461538461538,0.265384615384615,
0.267307692307692,0.269230769230769,0.271153846153846,0.273076923076923,
0.275,0.276923076923077,0.278846153846154,0.280769230769231,0.282692307692308,
0.284615384615385,0.286538461538462,0.288461538461538,0.290384615384615,
0.292307692307692,0.294230769230769,0.296153846153846,0.298076923076923,
0.3,0.301923076923077,0.303846153846154,0.305769230769231,0.307692307692308,
0.309615384615385,0.311538461538462,0.313461538461538,0.315384615384615,
0.317307692307692,0.319230769230769,0.321153846153846,0.323076923076923,
0.325,0.326923076923077,0.328846153846154,0.330769230769231,0.332692307692308,
0.334615384615385,0.336538461538462,0.338461538461538,0.340384615384615,
0.342307692307692,0.344230769230769,0.346153846153846,0.348076923076923,
0.35,0.351923076923077,0.353846153846154,0.355769230769231,0.357692307692308,
0.359615384615385,0.361538461538462,0.363461538461538,0.365384615384615,
0.367307692307692,0.369230769230769,0.371153846153846,0.373076923076923,
0.375,0.376923076923077,0.378846153846154,0.380769230769231,0.382692307692308,
0.384615384615385,0.386538461538462,0.388461538461538,0.390384615384615,
0.392307692307692,0.394230769230769,0.396153846153846,0.398076923076923,
0.4,0.401923076923077,0.403846153846154,0.405769230769231,0.407692307692308,
0.409615384615385,0.411538461538462,0.413461538461538,0.415384615384615,
0.417307692307692,0.419230769230769,0.421153846153846,0.423076923076923,
0.425,0.426923076923077,0.428846153846154,0.430769230769231,0.432692307692308,
0.434615384615385,0.436538461538462,0.438461538461538,0.440384615384615,
0.442307692307692,0.444230769230769,0.446153846153846,0.448076923076923,
0.45,0.451923076923077,0.453846153846154,0.455769230769231,0.457692307692308,
0.459615384615385,0.461538461538462,0.463461538461538,0.465384615384615,
0.467307692307692,0.469230769230769,0.471153846153846,0.473076923076923,
0.475,0.476923076923077,0.478846153846154,0.480769230769231,0.482692307692308,
0.484615384615385,0.486538461538462,0.488461538461538,0.490384615384615,
0.492307692307692,0.494230769230769,0.496153846153846,0.498076923076923,
0.5,0.501923076923077,0.503846153846154,0.505769230769231,0.507692307692308,
0.509615384615385,0.511538461538461,0.513461538461538,0.515384615384615,
0.517307692307692,0.519230769230769,0.521153846153846,0.523076923076923,
0.525,0.526923076923077,0.528846153846154,0.530769230769231,0.532692307692308,
0.534615384615385,0.536538461538462,0.538461538461538,0.540384615384615,
0.542307692307692,0.544230769230769,0.546153846153846,0.548076923076923,
0.55,0.551923076923077,0.553846153846154,0.555769230769231,0.557692307692308,
0.559615384615385,0.561538461538462,0.563461538461538,0.565384615384615,
0.567307692307692,0.569230769230769,0.571153846153846,0.573076923076923,
0.575,0.576923076923077,0.578846153846154,0.580769230769231,0.582692307692308,
0.584615384615385,0.586538461538462,0.588461538461538,0.590384615384615,
0.592307692307692,0.594230769230769,0.596153846153846,0.598076923076923,
0.6,0.601923076923077,0.603846153846154,0.605769230769231,0.607692307692308,
0.609615384615385,0.611538461538462,0.613461538461539,0.615384615384615,
0.617307692307692,0.619230769230769,0.621153846153846,0.623076923076923,
0.625,0.626923076923077,0.628846153846154,0.630769230769231,0.632692307692308,
0.634615384615385,0.636538461538461,0.638461538461538,0.640384615384615,
0.642307692307692,0.644230769230769,0.646153846153846,0.648076923076923,
0.65,0.651923076923077,0.653846153846154,0.655769230769231,0.657692307692308,
0.659615384615385,0.661538461538462,0.663461538461538,0.665384615384615,
0.667307692307692,0.669230769230769,0.671153846153846,0.673076923076923,
0.675,0.676923076923077,0.678846153846154,0.680769230769231,0.682692307692308,
0.684615384615385,0.686538461538462,0.688461538461538,0.690384615384615,
0.692307692307692,0.694230769230769,0.696153846153846,0.698076923076923,
0.7,0.701923076923077,0.703846153846154,0.705769230769231,0.707692307692308,
0.709615384615385,0.711538461538462,0.713461538461538,0.715384615384615,
0.717307692307692,0.719230769230769,0.721153846153846,0.723076923076923,
0.725,0.726923076923077,0.728846153846154,0.730769230769231,0.732692307692308,
0.734615384615385,0.736538461538462,0.738461538461539,0.740384615384615,
0.742307692307692,0.744230769230769,0.746153846153846,0.748076923076923,
0.75,0.751923076923077,0.753846153846154,0.755769230769231,0.757692307692308,
0.759615384615385,0.761538461538461,0.763461538461538,0.765384615384615,
0.767307692307692,0.769230769230769,0.771153846153846,0.773076923076923,
0.775,0.776923076923077,0.778846153846154,0.780769230769231,0.782692307692308,
0.784615384615385,0.786538461538462,0.788461538461538,0.790384615384615,
0.792307692307692,0.794230769230769,0.796153846153846,0.798076923076923,
0.8,0.801923076923077,0.803846153846154,0.805769230769231,0.807692307692308,
0.809615384615385,0.811538461538462,0.813461538461538,0.815384615384615,
0.817307692307692,0.819230769230769,0.821153846153846,0.823076923076923,
0.825,0.826923076923077,0.828846153846154,0.830769230769231,0.832692307692308,
0.834615384615385,0.836538461538462,0.838461538461538,0.840384615384615,
0.842307692307692,0.844230769230769,0.846153846153846,0.848076923076923,
0.85,0.851923076923077,0.853846153846154,0.855769230769231,0.857692307692308,
0.859615384615385,0.861538461538462,0.863461538461539,0.865384615384615,
0.867307692307692,0.869230769230769,0.871153846153846,0.873076923076923,
0.875,0.876923076923077,0.878846153846154,0.880769230769231,0.882692307692308,
0.884615384615385,0.886538461538461,0.888461538461538,0.890384615384615,
0.892307692307692,0.894230769230769,0.896153846153846,0.898076923076923,
0.9,0.901923076923077,0.903846153846154,0.905769230769231,0.907692307692308,
0.909615384615385,0.911538461538462,0.913461538461538,0.915384615384615,
0.917307692307692,0.919230769230769,0.921153846153846,0.923076923076923,
0.925,0.926923076923077,0.928846153846154,0.930769230769231,0.932692307692308,
0.934615384615385,0.936538461538462,0.938461538461538,0.940384615384615,
0.942307692307692,0.944230769230769,0.946153846153846,0.948076923076923,
0.95,0.951923076923077,0.953846153846154,0.955769230769231,0.957692307692308,
0.959615384615385,0.961538461538462,0.963461538461538,0.965384615384615,
0.967307692307692,0.969230769230769,0.971153846153846,0.973076923076923,
0.975,0.976923076923077,0.978846153846154,0.980769230769231,0.982692307692308,
0.984615384615385,0.986538461538462,0.988461538461539,0.990384615384615,
0.992307692307692,0.994230769230769,0.996153846153846),.UNSPECIFIED.)
GEOMETRIC_REPRESENTATION_ITEM()
RATIONAL_B_SPLINE_SURFACE(((1.,0.951056516295153,1.,0.951056516295153,1.,
0.951056516295153,1.,0.951056516295153,1.,0.951056516295153,1.,0.951056516295153,
1.,0.951056516295153,1.,0.951056516295153,1.,0.951056516295153,1.,0.951056516295153,
1.,0.951056516295153,1.,0.951056516295153,1.,0.951056516295153,1.,0.951056516295153,
1.,0.951056516295153,1.,0.951056516295153,1.,0.951056516295153,1.,0.951056516295153,
1.,0.951056516295153,1.,0.951056516295153,1.,0.951056516295153,1.,0.951056516295153,
1.,0.951056516295153,1.,0.951056516295153,1.,0.951056516295153,1.,0.951056516295153,
1.,0.951056516295153,1.,0.951056516295153,1.,0.951056516295153,1.,0.951056516295153,
1.,0.951056516295153,1.,0.951056516295153,1.,0.951056516295153,1.,0.951056516295153,
1.,0.951056516295153,1.,0.951056516295153,1.,0.951056516295153,1.,0.951056516295153,
1.,0.951056516295153,1.,0.951056516295153,1.,0.951056516295153,1.,0.951056516295153,
1.,0.951056516295153,1.,0.951056516295153,1.,0.951056516295153,1.,0.951056516295153,
1.,0.951056516295153,1.,0.951056516295153,1.,0.951056516295153,1.,0.951056516295153,
1.,0.951056516295153,1.,0.951056516295153,1.,0.951056516295153,1.,0.951056516295153,
1.,0.951056516295153,1.,0.951056516295153,1.,0.951056516295153,1.,0.951056516295153,
1.,0.951056516295153,1.,0.951056516295153,1.,0.951056516295153,1.,0.951056516295153,
1.,0.951056516295153,1.,0.951056516295153,1.,0.951056516295153,1.,0.951056516295153,
1.,0.951056516295153,1.,0.951056516295153,1.,0.951056516295153,1.,0.951056516295153,
1.,0.951056516295153,1.,0.951056516295153,1.,0.951056516295153,1.,0.951056516295153,
1.,0.951056516295153,1.,0.951056516295153,1.,0.951056516295153,1.,0.951056516295153,
1.,0.951056516295153,1.,0.951056516295153,1.,0.951056516295153,1.,0.951056516295153,
1.,0.951056516295153,1.,0.951056516295153,1.,0.951056516295153,1.,0.951056516295153,
1.,0.951056516295153,1.,0.951056516295153,1.,0.951056516295153,1.,0.951056516295153,
1.,0.951056516295153,1.,0.951056516295153,1.,0.951056516295153,1.,0.951056516295153,
1.,0.951056516295153,1.,0.951056516295153,1.,0.951056516295153,1.,0.951056516295153,
1.,0.951056516295153,1.,0.951056516295153,1.,0.951056516295153,1.,0.951056516295153,
1.,0.951056516295153,1.,0.951056516295153,1.,0.951056516295153,1.,0.951056516295153,
1.,0.951056516295153,1.,0.951056516295153,1.,0.951056516295153,1.,0.951056516295153,
1.,0.951056516295153,1.,0.951056516295153,1.,0.951056516295153,1.,0.951056516295153,
1.,0.951056516295153,1.,0.951056516295153,1.,0.951056516295153,1.,0.951056516295153,
1.,0.951056516295153,1.,0.951056516295153,1.,0.951056516295153,1.,0.951056516295153,
1.,0.951056516295153,1.,0.951056516295153,1.,0.951056516295153,1.,0.951056516295153,
1.,0.951056516295153,1.,0.951056516295153,1.,0.951056516295153,1.,0.951056516295153,
1.,0.951056516295153,1.,0.951056516295153,1.,0.951056516295153,1.,0.951056516295153,
1.,0.951056516295153,1.,0.951056516295153,1.,0.951056516295153,1.,0.951056516295153,
1.,0.951056516295153,1.,0.951056516295153,1.,0.951056516295153,1.,0.951056516295153,
1.,0.951056516295153,1.,0.951056516295153,1.,0.951056516295153,1.,0.951056516295153,
1.,0.951056516295153,1.,0.951056516295153,1.,0.951056516295153,1.,0.951056516295153,
1.,0.951056516295153,1.,0.951056516295153,1.,0.951056516295153,1.,0.951056516295153,
1.,0.951056516295153,1.,0.951056516295153,1.,0.951056516295153,1.,0.951056516295153,
1.,0.951056516295153,1.,0.951056516295153,1.,0.951056516295153,1.,0.951056516295153,
1.,0.951056516295153,1.,0.951056516295153,1.,0.951056516295153,1.,0.951056516295153,
1.,0.951056516295153,1.,0.951056516295153,1.,0.951056516295153,1.,0.951056516295153,
1.,0.951056516295153,1.,0.951056516295153,1.,0.951056516295153,1.,0.951056516295153,
1.,0.951056516295153,1.,0.951056516295153,1.,0.951056516295153,1.,0.951056516295153,
1.,0.951056516295153,1.,0.951056516295153,1.,0.951056516295153,1.,0.951056516295153,
1.,0.951056516295153,1.,0.951056516295153,1.,0.951056516295153,1.,0.951056516295153,
1.,0.951056516295153,1.,0.951056516295153,1.,0.951056516295153,1.,0.951056516295153,
1.,0.951056516295153,1.,0.951056516295153,1.,0.951056516295153,1.,0.951056516295153,
1.,0.951056516295153,1.,0.951056516295153,1.,0.951056516295153,1.,0.951056516295153,
1.,0.951056516295153,1.,0.951056516295153,1.,0.951056516295153,1.,0.951056516295153,
1.,0.951056516295153,1.,0.951056516295153,1.,0.951056516295153,1.,0.951056516295153,
1.,0.951056516295153,1.,0.951056516295153,1.,0.951056516295153,1.,0.951056516295153,
1.,0.951056516295153,1.,0.951056516295153,1.,0.951056516295153,1.,0.951056516295153,
1.,0.951056516295153,1.,0.951056516295153,1.,0.951056516295153,1.,0.951056516295153,
1.,0.951056516295153,1.,0.951056516295153,1.,0.951056516295153,1.,0.951056516295153,
1.,0.951056516295153,1.,0.951056516295153,1.,0.951056516295153,1.,0.951056516295153,
1.,0.951056516295153,1.,0.951056516295153,1.,0.951056516295153,1.,0.951056516295153,
1.,0.951056516295153,1.,0.951056516295153,1.,0.951056516295153,1.,0.951056516295153,
1.,0.951056516295153,1.,0.951056516295153,1.,0.951056516295153,1.,0.951056516295153,
1.,0.951056516295153,1.,0.951056516295153,1.,0.951056516295153,1.,0.951056516295153,
1.,0.951056516295153,1.,0.951056516295153,1.,0.951056516295153,1.,0.951056516295153,
1.,0.951056516295153,1.,0.951056516295153,1.,0.951056516295153,1.,0.951056516295153,
1.,0.951056516295153,1.,0.951056516295153,1.,0.951056516295153,1.,0.951056516295153,
1.,0.951056516295153,1.,0.951056516295153,1.,0.951056516295153,1.,0.951056516295153,
1.,0.951056516295153,1.,0.951056516295153,1.,0.951056516295153,1.,0.951056516295153,
1.,0.951056516295153,1.,0.951056516295153,1.,0.951056516295153,1.,0.951056516295153,
1.,0.951056516295153,1.,0.951056516295153,1.,0.951056516295153,1.,0.951056516295153,
1.,0.951056516295153,1.,0.951056516295153,1.,0.951056516295153,1.,0.951056516295153,
1.,0.951056516295153,1.,0.951056516295153,1.,0.951056516295153,1.,0.951056516295153,
1.,0.951056516295153,1.,0.951056516295153,1.,0.951056516295153,1.,0.951056516295153,
1.,0.951056516295153,1.,0.951056516295153,1.,0.951056516295153,1.,0.951056516295153,
1.,0.951056516295153,1.,0.951056516295153,1.,0.951056516295153,1.,0.951056516295153,
1.,0.951056516295153,1.,0.951056516295153,1.,0.951056516295153,1.,0.951056516295153,
1.,0.951056516295153,1.,0.951056516295153,1.,0.951056516295153,1.,0.951056516295153,
1.,0.951056516295153,1.,0.951056516295153,1.,0.951056516295153,1.,0.951056516295153,
1.,0.951056516295153,1.,0.951056516295153,1.,0.951056516295153,1.,0.951056516295153,
1.,0.951056516295153,1.,0.951056516295153,1.,0.951056516295153,1.,0.951056516295153,
1.,0.951056516295153,1.,0.951056516295153,1.,0.951056516295153,1.,0.951056516295153,
1.,0.951056516295153,1.,0.951056516295153,1.,0.951056516295153,1.,0.951056516295153,
1.,0.951056516295153,1.,0.951056516295153,1.,0.951056516295153,1.,0.951056516295153,
1.,0.951056516295153,1.,0.951056516295153,1.,0.951056516295153,1.,0.951056516295153,
1.,0.951056516295153,1.,0.951056516295153,1.,0.951056516295153,1.,0.951056516295153,
1.,0.951056516295153,1.,0.951056516295153,1.,0.951056516295153,1.,0.951056516295153,
1.,0.951056516295153,1.,0.951056516295153,1.,0.951056516295153,1.,0.951056516295153,
1.,0.951056516295153,1.,0.951056516295153,1.,0.951056516295153,1.,0.951056516295153,
1.,0.951056516295153,1.,0.951056516295153,1.,0.951056516295153,1.,0.951056516295153,
1.,0.951056516295153,1.,0.951056516295153,1.,0.951056516295153,1.,0.951056516295153,
1.,0.951056516295153,1.,0.951056516295153,1.,0.951056516295153,1.,0.951056516295153,
1.,0.951056516295153,1.,0.951056516295153,1.,0.951056516295153,1.,0.951056516295153,
1.,0.951056516295153,1.,0.951056516295153,1.,0.951056516295153,1.,0.951056516295153,
1.,0.951056516295153,1.,0.951056516295153,1.,0.951056516295153,1.,0.951056516295153,
1.,0.951056516295153,1.,0.951056516295153,1.,0.951056516295153,1.,0.951056516295153,
1.,0.951056516295153,1.,0.951056516295153,1.,0.951056516295153,1.,0.951056516295153,
1.,0.951056516295153,1.,0.951056516295153,1.,0.951056516295153,1.,0.951056516295153,
1.,0.951056516295153,1.,0.951056516295153,1.,0.951056516295153,1.,0.951056516295153,
1.,0.951056516295153,1.,0.951056516295153,1.,0.951056516295153,1.,0.951056516295153,
1.,0.951056516295153,1.,0.951056516295153,1.,0.951056516295153,1.,0.951056516295153,
1.,0.951056516295153,1.,0.951056516295153,1.,0.951056516295153,1.,0.951056516295153,
1.,0.951056516295153,1.,0.951056516295153,1.,0.951056516295153,1.,0.951056516295153,
1.,0.951056516295153,1.,0.951056516295153,1.,0.951056516295153,1.,0.951056516295153,
1.,0.951056516295153,1.,0.951056516295153,1.,0.951056516295153,1.,0.951056516295153,
1.,0.951056516295153,1.,0.951056516295153,1.,0.951056516295153,1.,0.951056516295153,
1.,0.951056516295153,1.,0.951056516295153,1.,0.951056516295153,1.,0.951056516295153,
1.,0.951056516295153,1.,0.951056516295153,1.,0.951056516295153,1.,0.951056516295153,
1.,0.951056516295153,1.,0.951056516295153,1.,0.951056516295153,1.,0.951056516295153,
1.,0.951056516295153,1.,0.951056516295153,1.,0.951056516295153,1.,0.951056516295153,
1.,0.951056516295153,1.,0.951056516295153,1.,0.951056516295153,1.,0.951056516295153,
1.,0.951056516295153,1.,0.951056516295153,1.,0.951056516295153,1.,0.951056516295153,
1.,0.951056516295153,1.,0.951056516295153,1.,0.951056516295153,1.,0.951056516295153,
1.,0.951056516295153,1.,0.951056516295153,1.,0.951056516295153,1.,0.951056516295153,
1.,0.951056516295153,1.,0.951056516295153,1.,0.951056516295153,1.,0.951056516295153,
1.,0.951056516295153,1.,0.951056516295153,1.,0.951056516295153,1.,0.951056516295153,
1.,0.951056516295153,1.,0.951056516295153,1.,0.951056516295153,1.,0.951056516295153,
1.,0.951056516295153,1.,0.951056516295153,1.,0.951056516295153,1.,0.951056516295153,
1.,0.951056516295153,1.,0.951056516295153,1.,0.951056516295153,1.,0.951056516295153,
1.,0.951056516295153,1.,0.951056516295153,1.,0.951056516295153,1.,0.951056516295153,
1.,0.951056516295153,1.,0.951056516295153,1.,0.951056516295153,1.,0.951056516295153,
1.,0.951056516295153,1.,0.951056516295153,1.,0.951056516295153,1.,0.951056516295153,
1.,0.951056516295153,1.,0.951056516295153,1.,0.951056516295153,1.,0.951056516295153,
1.,0.951056516295153,1.,0.951056516295153,1.,0.951056516295153,1.,0.951056516295153,
1.,0.951056516295153,1.,0.951056516295153,1.,0.951056516295153,1.,0.951056516295153,
1.,0.951056516295153,1.,0.951056516295153,1.,0.951056516295153,1.,0.951056516295153,
1.,0.951056516295153,1.,0.951056516295153,1.,0.951056516295153,1.,0.951056516295153,
1.,0.951056516295153,1.,0.951056516295153,1.,0.951056516295153,1.,0.951056516295153,
1.,0.951056516295153,1.,0.951056516295153,1.,0.951056516295153,1.,0.951056516295153,
1.,0.951056516295153,1.,0.951056516295153,1.,0.951056516295153,1.,0.951056516295153,
1.,0.951056516295153,1.,0.951056516295153,1.,0.951056516295153,1.,0.951056516295153,
1.,0.951056516295153,1.,0.951056516295153,1.,0.951056516295153,1.,0.951056516295153,
1.,0.951056516295153,1.,0.951056516295153,1.,0.951056516295153,1.,0.951056516295153,
1.),(1.,0.951056516295154,1.,0.951056516295154,1.,0.951056516295154,1.,
0.951056516295154,1.,0.951056516295154,1.,0.951056516295154,1.,0.951056516295154,
1.,0.951056516295154,1.,0.951056516295154,1.,0.951056516295154,1.,0.951056516295154,
1.,0.951056516295154,1.,0.951056516295154,1.,0.951056516295154,1.,0.951056516295154,
1.,0.951056516295154,1.,0.951056516295154,1.,0.951056516295154,1.,0.951056516295154,
1.,0.951056516295154,1.,0.951056516295154,1.,0.951056516295154,1.,0.951056516295154,
1.,0.951056516295154,1.,0.951056516295154,1.,0.951056516295154,1.,0.951056516295154,
1.,0.951056516295154,1.,0.951056516295154,1.,0.951056516295154,1.,0.951056516295154,
1.,0.951056516295154,1.,0.951056516295154,1.,0.951056516295154,1.,0.951056516295154,
1.,0.951056516295154,1.,0.951056516295154,1.,0.951056516295154,1.,0.951056516295154,
1.,0.951056516295154,1.,0.951056516295154,1.,0.951056516295154,1.,0.951056516295154,
1.,0.951056516295154,1.,0.951056516295154,1.,0.951056516295154,1.,0.951056516295154,
1.,0.951056516295154,1.,0.951056516295154,1.,0.951056516295154,1.,0.951056516295154,
1.,0.951056516295154,1.,0.951056516295154,1.,0.951056516295154,1.,0.951056516295154,
1.,0.951056516295154,1.,0.951056516295154,1.,0.951056516295154,1.,0.951056516295154,
1.,0.951056516295154,1.,0.951056516295154,1.,0.951056516295154,1.,0.951056516295154,
1.,0.951056516295154,1.,0.951056516295154,1.,0.951056516295154,1.,0.951056516295154,
1.,0.951056516295154,1.,0.951056516295154,1.,0.951056516295154,1.,0.951056516295154,
1.,0.951056516295154,1.,0.951056516295154,1.,0.951056516295154,1.,0.951056516295154,
1.,0.951056516295154,1.,0.951056516295154,1.,0.951056516295154,1.,0.951056516295154,
1.,0.951056516295154,1.,0.951056516295154,1.,0.951056516295154,1.,0.951056516295154,
1.,0.951056516295154,1.,0.951056516295154,1.,0.951056516295154,1.,0.951056516295154,
1.,0.951056516295154,1.,0.951056516295154,1.,0.951056516295154,1.,0.951056516295154,
1.,0.951056516295154,1.,0.951056516295154,1.,0.951056516295154,1.,0.951056516295154,
1.,0.951056516295154,1.,0.951056516295154,1.,0.951056516295154,1.,0.951056516295154,
1.,0.951056516295154,1.,0.951056516295154,1.,0.951056516295154,1.,0.951056516295154,
1.,0.951056516295154,1.,0.951056516295154,1.,0.951056516295154,1.,0.951056516295154,
1.,0.951056516295154,1.,0.951056516295154,1.,0.951056516295154,1.,0.951056516295154,
1.,0.951056516295154,1.,0.951056516295154,1.,0.951056516295154,1.,0.951056516295154,
1.,0.951056516295154,1.,0.951056516295154,1.,0.951056516295154,1.,0.951056516295154,
1.,0.951056516295154,1.,0.951056516295154,1.,0.951056516295154,1.,0.951056516295154,
1.,0.951056516295154,1.,0.951056516295154,1.,0.951056516295154,1.,0.951056516295154,
1.,0.951056516295154,1.,0.951056516295154,1.,0.951056516295154,1.,0.951056516295154,
1.,0.951056516295154,1.,0.951056516295154,1.,0.951056516295154,1.,0.951056516295154,
1.,0.951056516295154,1.,0.951056516295154,1.,0.951056516295154,1.,0.951056516295154,
1.,0.951056516295154,1.,0.951056516295154,1.,0.951056516295154,1.,0.951056516295154,
1.,0.951056516295154,1.,0.951056516295154,1.,0.951056516295154,1.,0.951056516295154,
1.,0.951056516295154,1.,0.951056516295154,1.,0.951056516295154,1.,0.951056516295154,
1.,0.951056516295154,1.,0.951056516295154,1.,0.951056516295154,1.,0.951056516295154,
1.,0.951056516295154,1.,0.951056516295154,1.,0.951056516295154,1.,0.951056516295154,
1.,0.951056516295154,1.,0.951056516295154,1.,0.951056516295154,1.,0.951056516295154,
1.,0.951056516295154,1.,0.951056516295154,1.,0.951056516295154,1.,0.951056516295154,
1.,0.951056516295154,1.,0.951056516295154,1.,0.951056516295154,1.,0.951056516295154,
1.,0.951056516295154,1.,0.951056516295154,1.,0.951056516295154,1.,0.951056516295154,
1.,0.951056516295154,1.,0.951056516295154,1.,0.951056516295154,1.,0.951056516295154,
1.,0.951056516295154,1.,0.951056516295154,1.,0.951056516295154,1.,0.951056516295154,
1.,0.951056516295154,1.,0.951056516295154,1.,0.951056516295154,1.,0.951056516295154,
1.,0.951056516295154,1.,0.951056516295154,1.,0.951056516295154,1.,0.951056516295154,
1.,0.951056516295154,1.,0.951056516295154,1.,0.951056516295154,1.,0.951056516295154,
1.,0.951056516295154,1.,0.951056516295154,1.,0.951056516295154,1.,0.951056516295154,
1.,0.951056516295154,1.,0.951056516295154,1.,0.951056516295154,1.,0.951056516295154,
1.,0.951056516295154,1.,0.951056516295154,1.,0.951056516295154,1.,0.951056516295154,
1.,0.951056516295154,1.,0.951056516295154,1.,0.951056516295154,1.,0.951056516295154,
1.,0.951056516295154,1.,0.951056516295154,1.,0.951056516295154,1.,0.951056516295154,
1.,0.951056516295154,1.,0.951056516295154,1.,0.951056516295154,1.,0.951056516295154,
1.,0.951056516295154,1.,0.951056516295154,1.,0.951056516295154,1.,0.951056516295154,
1.,0.951056516295154,1.,0.951056516295154,1.,0.951056516295154,1.,0.951056516295154,
1.,0.951056516295154,1.,0.951056516295154,1.,0.951056516295154,1.,0.951056516295154,
1.,0.951056516295154,1.,0.951056516295154,1.,0.951056516295154,1.,0.951056516295154,
1.,0.951056516295154,1.,0.951056516295154,1.,0.951056516295154,1.,0.951056516295154,
1.,0.951056516295154,1.,0.951056516295154,1.,0.951056516295154,1.,0.951056516295154,
1.,0.951056516295154,1.,0.951056516295154,1.,0.951056516295154,1.,0.951056516295154,
1.,0.951056516295154,1.,0.951056516295154,1.,0.951056516295154,1.,0.951056516295154,
1.,0.951056516295154,1.,0.951056516295154,1.,0.951056516295154,1.,0.951056516295154,
1.,0.951056516295154,1.,0.951056516295154,1.,0.951056516295154,1.,0.951056516295154,
1.,0.951056516295154,1.,0.951056516295154,1.,0.951056516295154,1.,0.951056516295154,
1.,0.951056516295154,1.,0.951056516295154,1.,0.951056516295154,1.,0.951056516295154,
1.,0.951056516295154,1.,0.951056516295154,1.,0.951056516295154,1.,0.951056516295154,
1.,0.951056516295154,1.,0.951056516295154,1.,0.951056516295154,1.,0.951056516295154,
1.,0.951056516295154,1.,0.951056516295154,1.,0.951056516295154,1.,0.951056516295154,
1.,0.951056516295154,1.,0.951056516295154,1.,0.951056516295154,1.,0.951056516295154,
1.,0.951056516295154,1.,0.951056516295154,1.,0.951056516295154,1.,0.951056516295154,
1.,0.951056516295154,1.,0.951056516295154,1.,0.951056516295154,1.,0.951056516295154,
1.,0.951056516295154,1.,0.951056516295154,1.,0.951056516295154,1.,0.951056516295154,
1.,0.951056516295154,1.,0.951056516295154,1.,0.951056516295154,1.,0.951056516295154,
1.,0.951056516295154,1.,0.951056516295154,1.,0.951056516295154,1.,0.951056516295154,
1.,0.951056516295154,1.,0.951056516295154,1.,0.951056516295154,1.,0.951056516295154,
1.,0.951056516295154,1.,0.951056516295154,1.,0.951056516295154,1.,0.951056516295154,
1.,0.951056516295154,1.,0.951056516295154,1.,0.951056516295154,1.,0.951056516295154,
1.,0.951056516295154,1.,0.951056516295154,1.,0.951056516295154,1.,0.951056516295154,
1.,0.951056516295154,1.,0.951056516295154,1.,0.951056516295154,1.,0.951056516295154,
1.,0.951056516295154,1.,0.951056516295154,1.,0.951056516295154,1.,0.951056516295154,
1.,0.951056516295154,1.,0.951056516295154,1.,0.951056516295154,1.,0.951056516295154,
1.,0.951056516295154,1.,0.951056516295154,1.,0.951056516295154,1.,0.951056516295154,
1.,0.951056516295154,1.,0.951056516295154,1.,0.951056516295154,1.,0.951056516295154,
1.,0.951056516295154,1.,0.951056516295154,1.,0.951056516295154,1.,0.951056516295154,
1.,0.951056516295154,1.,0.951056516295154,1.,0.951056516295154,1.,0.951056516295154,
1.,0.951056516295154,1.,0.951056516295154,1.,0.951056516295154,1.,0.951056516295154,
1.,0.951056516295154,1.,0.951056516295154,1.,0.951056516295154,1.,0.951056516295154,
1.,0.951056516295154,1.,0.951056516295154,1.,0.951056516295154,1.,0.951056516295154,
1.,0.951056516295154,1.,0.951056516295154,1.,0.951056516295154,1.,0.951056516295154,
1.,0.951056516295154,1.,0.951056516295154,1.,0.951056516295154,1.,0.951056516295154,
1.,0.951056516295154,1.,0.951056516295154,1.,0.951056516295154,1.,0.951056516295154,
1.,0.951056516295154,1.,0.951056516295154,1.,0.951056516295154,1.,0.951056516295154,
1.,0.951056516295154,1.,0.951056516295154,1.,0.951056516295154,1.,0.951056516295154,
1.,0.951056516295154,1.,0.951056516295154,1.,0.951056516295154,1.,0.951056516295154,
1.,0.951056516295154,1.,0.951056516295154,1.,0.951056516295154,1.,0.951056516295154,
1.,0.951056516295154,1.,0.951056516295154,1.,0.951056516295154,1.,0.951056516295154,
1.,0.951056516295154,1.,0.951056516295154,1.,0.951056516295154,1.,0.951056516295154,
1.,0.951056516295154,1.,0.951056516295154,1.,0.951056516295154,1.,0.951056516295154,
1.,0.951056516295154,1.,0.951056516295154,1.,0.951056516295154,1.,0.951056516295154,
1.,0.951056516295154,1.,0.951056516295154,1.,0.951056516295154,1.,0.951056516295154,
1.,0.951056516295154,1.,0.951056516295154,1.,0.951056516295154,1.,0.951056516295154,
1.,0.951056516295154,1.,0.951056516295154,1.,0.951056516295154,1.,0.951056516295154,
1.,0.951056516295154,1.,0.951056516295154,1.,0.951056516295154,1.,0.951056516295154,
1.,0.951056516295154,1.,0.951056516295154,1.,0.951056516295154,1.,0.951056516295154,
1.,0.951056516295154,1.,0.951056516295154,1.,0.951056516295154,1.,0.951056516295154,
1.,0.951056516295154,1.,0.951056516295154,1.,0.951056516295154,1.,0.951056516295154,
1.,0.951056516295154,1.,0.951056516295154,1.,0.951056516295154,1.,0.951056516295154,
1.,0.951056516295154,1.,0.951056516295154,1.,0.951056516295154,1.,0.951056516295154,
1.,0.951056516295154,1.,0.951056516295154,1.,0.951056516295154,1.,0.951056516295154,
1.,0.951056516295154,1.,0.951056516295154,1.,0.951056516295154,1.,0.951056516295154,
1.,0.951056516295154,1.,0.951056516295154,1.,0.951056516295154,1.,0.951056516295154,
1.,0.951056516295154,1.,0.951056516295154,1.,0.951056516295154,1.,0.951056516295154,
1.,0.951056516295154,1.,0.951056516295154,1.,0.951056516295154,1.,0.951056516295154,
1.,0.951056516295154,1.,0.951056516295154,1.,0.951056516295154,1.,0.951056516295154,
1.,0.951056516295154,1.,0.951056516295154,1.,0.951056516295154,1.,0.951056516295154,
1.,0.951056516295154,1.,0.951056516295154,1.,0.951056516295154,1.,0.951056516295154,
1.,0.951056516295154,1.,0.951056516295154,1.,0.951056516295154,1.,0.951056516295154,
1.,0.951056516295154,1.,0.951056516295154,1.,0.951056516295154,1.,0.951056516295154,
1.,0.951056516295154,1.,0.951056516295154,1.,0.951056516295154,1.,0.951056516295154,
1.,0.951056516295154,1.,0.951056516295154,1.,0.951056516295154,1.,0.951056516295154,
1.,0.951056516295154,1.,0.951056516295154,1.,0.951056516295154,1.,0.951056516295154,
1.,0.951056516295154,1.,0.951056516295154,1.,0.951056516295154,1.,0.951056516295154,
1.,0.951056516295154,1.,0.951056516295154,1.,0.951056516295154,1.,0.951056516295154,
1.,0.951056516295154,1.,0.951056516295154,1.,0.951056516295154,1.,0.951056516295154,
1.,0.951056516295154,1.,0.951056516295154,1.,0.951056516295154,1.,0.951056516295154,
1.,0.951056516295154,1.,0.951056516295154,1.,0.951056516295154,1.,0.951056516295154,
1.,0.951056516295154,1.,0.951056516295154,1.,0.951056516295154,1.,0.951056516295154,
1.,0.951056516295154,1.,0.951056516295154,1.,0.951056516295154,1.)))
REPRESENTATION_ITEM('')
SURFACE()
);
#3193=(
BOUNDED_SURFACE()
B_SPLINE_SURFACE(1,2,((#278547,#278548,#278549,#278550,#278551,#278552,
#278553,#278554,#278555,#278556,#278557,#278558,#278559,#278560,#278561,
#278562,#278563,#278564,#278565,#278566,#278567,#278568,#278569,#278570,
#278571,#278572,#278573,#278574,#278575,#278576,#278577,#278578,#278579,
#278580,#278581,#278582,#278583,#278584,#278585,#278586,#278587,#278588,
#278589,#278590,#278591,#278592,#278593,#278594,#278595,#278596,#278597,
#278598,#278599,#278600,#278601,#278602,#278603,#278604,#278605,#278606,
#278607,#278608,#278609,#278610,#278611,#278612,#278613,#278614,#278615,
#278616,#278617,#278618,#278619,#278620,#278621,#278622,#278623,#278624,
#278625,#278626,#278627,#278628,#278629,#278630,#278631,#278632,#278633,
#278634,#278635,#278636,#278637,#278638,#278639,#278640,#278641,#278642,
#278643,#278644,#278645,#278646,#278647,#278648,#278649,#278650,#278651,
#278652,#278653,#278654,#278655,#278656,#278657,#278658,#278659,#278660,
#278661,#278662,#278663,#278664,#278665,#278666,#278667,#278668,#278669,
#278670,#278671,#278672,#278673,#278674,#278675,#278676,#278677,#278678,
#278679,#278680,#278681,#278682,#278683,#278684,#278685,#278686,#278687,
#278688,#278689,#278690,#278691,#278692,#278693,#278694,#278695,#278696,
#278697,#278698,#278699,#278700,#278701,#278702,#278703,#278704,#278705,
#278706,#278707,#278708,#278709,#278710,#278711,#278712,#278713,#278714,
#278715,#278716,#278717,#278718,#278719,#278720,#278721,#278722,#278723,
#278724,#278725,#278726,#278727,#278728,#278729,#278730,#278731,#278732,
#278733,#278734,#278735,#278736,#278737,#278738,#278739,#278740,#278741,
#278742,#278743,#278744,#278745,#278746,#278747,#278748,#278749,#278750,
#278751,#278752,#278753,#278754,#278755,#278756,#278757,#278758,#278759,
#278760,#278761,#278762,#278763,#278764,#278765,#278766,#278767,#278768,
#278769,#278770,#278771,#278772,#278773,#278774,#278775,#278776,#278777,
#278778,#278779,#278780,#278781,#278782,#278783,#278784,#278785,#278786,
#278787,#278788,#278789,#278790,#278791,#278792,#278793,#278794,#278795,
#278796,#278797,#278798,#278799,#278800,#278801,#278802,#278803,#278804,
#278805,#278806,#278807,#278808,#278809,#278810,#278811,#278812,#278813,
#278814,#278815,#278816,#278817,#278818,#278819,#278820,#278821,#278822,
#278823,#278824,#278825,#278826,#278827,#278828,#278829,#278830,#278831,
#278832,#278833,#278834,#278835,#278836,#278837,#278838,#278839,#278840,
#278841,#278842,#278843,#278844,#278845,#278846,#278847,#278848,#278849,
#278850,#278851,#278852,#278853,#278854,#278855,#278856,#278857,#278858,
#278859,#278860,#278861,#278862,#278863,#278864,#278865,#278866,#278867,
#278868,#278869,#278870,#278871,#278872,#278873,#278874,#278875,#278876,
#278877,#278878,#278879,#278880,#278881,#278882,#278883,#278884,#278885,
#278886,#278887,#278888,#278889,#278890,#278891,#278892,#278893,#278894,
#278895,#278896,#278897,#278898,#278899,#278900,#278901,#278902,#278903,
#278904,#278905,#278906,#278907,#278908,#278909,#278910,#278911,#278912,
#278913,#278914,#278915,#278916,#278917,#278918,#278919,#278920,#278921,
#278922,#278923,#278924,#278925,#278926,#278927,#278928,#278929,#278930,
#278931,#278932,#278933,#278934,#278935,#278936,#278937,#278938,#278939,
#278940,#278941,#278942,#278943,#278944,#278945,#278946,#278947,#278948,
#278949,#278950,#278951,#278952,#278953,#278954,#278955,#278956,#278957,
#278958,#278959,#278960,#278961,#278962,#278963,#278964,#278965,#278966,
#278967,#278968,#278969,#278970,#278971,#278972,#278973,#278974,#278975,
#278976,#278977,#278978,#278979,#278980,#278981,#278982,#278983,#278984,
#278985,#278986,#278987,#278988,#278989,#278990,#278991,#278992,#278993,
#278994,#278995,#278996,#278997,#278998,#278999,#279000,#279001,#279002,
#279003,#279004,#279005,#279006,#279007,#279008,#279009,#279010,#279011,
#279012,#279013,#279014,#279015,#279016,#279017,#279018,#279019,#279020,
#279021,#279022,#279023,#279024,#279025,#279026,#279027,#279028,#279029,
#279030,#279031,#279032,#279033,#279034,#279035,#279036,#279037,#279038,
#279039,#279040,#279041,#279042,#279043,#279044,#279045,#279046,#279047,
#279048,#279049,#279050,#279051,#279052,#279053,#279054,#279055,#279056,
#279057,#279058,#279059,#279060,#279061,#279062,#279063,#279064,#279065,
#279066,#279067,#279068,#279069,#279070,#279071,#279072,#279073,#279074,
#279075,#279076,#279077,#279078,#279079,#279080,#279081,#279082,#279083,
#279084,#279085,#279086,#279087,#279088,#279089,#279090,#279091,#279092,
#279093,#279094,#279095,#279096,#279097,#279098,#279099,#279100,#279101,
#279102,#279103,#279104,#279105,#279106,#279107,#279108,#279109,#279110,
#279111,#279112,#279113,#279114,#279115,#279116,#279117,#279118,#279119,
#279120,#279121,#279122,#279123,#279124,#279125,#279126,#279127,#279128,
#279129,#279130,#279131,#279132,#279133,#279134,#279135,#279136,#279137,
#279138,#279139,#279140,#279141,#279142,#279143,#279144,#279145,#279146,
#279147,#279148,#279149,#279150,#279151,#279152,#279153,#279154,#279155,
#279156,#279157,#279158,#279159,#279160,#279161,#279162,#279163,#279164,
#279165,#279166,#279167,#279168,#279169,#279170,#279171,#279172,#279173,
#279174,#279175,#279176,#279177,#279178,#279179,#279180,#279181,#279182,
#279183,#279184,#279185,#279186,#279187,#279188,#279189,#279190,#279191,
#279192,#279193,#279194,#279195,#279196,#279197,#279198,#279199,#279200,
#279201,#279202,#279203,#279204,#279205,#279206,#279207,#279208,#279209,
#279210,#279211,#279212,#279213,#279214,#279215,#279216,#279217,#279218,
#279219,#279220,#279221,#279222,#279223,#279224,#279225,#279226,#279227,
#279228,#279229,#279230,#279231,#279232,#279233,#279234,#279235,#279236,
#279237,#279238,#279239,#279240,#279241,#279242,#279243,#279244,#279245,
#279246,#279247,#279248,#279249,#279250,#279251,#279252,#279253,#279254,
#279255,#279256,#279257,#279258,#279259,#279260,#279261,#279262,#279263,
#279264,#279265,#279266,#279267,#279268,#279269,#279270,#279271,#279272,
#279273,#279274,#279275,#279276,#279277,#279278,#279279,#279280,#279281,
#279282,#279283,#279284,#279285,#279286,#279287,#279288,#279289,#279290,
#279291,#279292,#279293,#279294,#279295,#279296,#279297,#279298,#279299,
#279300,#279301,#279302,#279303,#279304,#279305,#279306,#279307,#279308,
#279309,#279310,#279311,#279312,#279313,#279314,#279315,#279316,#279317,
#279318,#279319,#279320,#279321,#279322,#279323,#279324,#279325,#279326,
#279327,#279328,#279329,#279330,#279331,#279332,#279333,#279334,#279335,
#279336,#279337,#279338,#279339,#279340,#279341,#279342,#279343,#279344,
#279345,#279346,#279347,#279348,#279349,#279350,#279351,#279352,#279353,
#279354,#279355,#279356,#279357,#279358,#279359,#279360,#279361,#279362,
#279363,#279364,#279365,#279366,#279367,#279368,#279369,#279370,#279371,
#279372,#279373,#279374,#279375,#279376,#279377,#279378,#279379,#279380,
#279381,#279382,#279383,#279384,#279385,#279386,#279387,#279388,#279389,
#279390,#279391,#279392,#279393,#279394,#279395,#279396,#279397,#279398,
#279399,#279400,#279401,#279402,#279403,#279404,#279405,#279406,#279407,
#279408,#279409,#279410,#279411,#279412,#279413,#279414,#279415,#279416,
#279417,#279418,#279419,#279420,#279421,#279422,#279423,#279424,#279425,
#279426,#279427,#279428,#279429,#279430,#279431,#279432,#279433,#279434,
#279435,#279436,#279437,#279438,#279439,#279440,#279441,#279442,#279443,
#279444,#279445,#279446,#279447,#279448,#279449,#279450,#279451,#279452,
#279453,#279454,#279455,#279456,#279457,#279458,#279459,#279460,#279461,
#279462,#279463,#279464,#279465,#279466,#279467,#279468,#279469,#279470,
#279471,#279472,#279473,#279474,#279475,#279476,#279477,#279478,#279479,
#279480,#279481,#279482,#279483,#279484,#279485,#279486,#279487,#279488,
#279489,#279490,#279491,#279492,#279493,#279494,#279495,#279496,#279497,
#279498,#279499,#279500,#279501,#279502,#279503,#279504,#279505,#279506,
#279507,#279508,#279509,#279510,#279511,#279512,#279513,#279514,#279515,
#279516,#279517,#279518,#279519,#279520,#279521,#279522,#279523,#279524,
#279525,#279526,#279527,#279528,#279529,#279530,#279531,#279532,#279533,
#279534,#279535,#279536,#279537,#279538,#279539,#279540,#279541,#279542,
#279543,#279544,#279545,#279546,#279547,#279548,#279549,#279550,#279551,
#279552,#279553,#279554,#279555,#279556,#279557,#279558,#279559,#279560,
#279561,#279562,#279563,#279564,#279565,#279566,#279567,#279568,#279569,
#279570,#279571,#279572,#279573,#279574,#279575,#279576,#279577,#279578,
#279579,#279580,#279581,#279582,#279583),(#279584,#279585,#279586,#279587,
#279588,#279589,#279590,#279591,#279592,#279593,#279594,#279595,#279596,
#279597,#279598,#279599,#279600,#279601,#279602,#279603,#279604,#279605,
#279606,#279607,#279608,#279609,#279610,#279611,#279612,#279613,#279614,
#279615,#279616,#279617,#279618,#279619,#279620,#279621,#279622,#279623,
#279624,#279625,#279626,#279627,#279628,#279629,#279630,#279631,#279632,
#279633,#279634,#279635,#279636,#279637,#279638,#279639,#279640,#279641,
#279642,#279643,#279644,#279645,#279646,#279647,#279648,#279649,#279650,
#279651,#279652,#279653,#279654,#279655,#279656,#279657,#279658,#279659,
#279660,#279661,#279662,#279663,#279664,#279665,#279666,#279667,#279668,
#279669,#279670,#279671,#279672,#279673,#279674,#279675,#279676,#279677,
#279678,#279679,#279680,#279681,#279682,#279683,#279684,#279685,#279686,
#279687,#279688,#279689,#279690,#279691,#279692,#279693,#279694,#279695,
#279696,#279697,#279698,#279699,#279700,#279701,#279702,#279703,#279704,
#279705,#279706,#279707,#279708,#279709,#279710,#279711,#279712,#279713,
#279714,#279715,#279716,#279717,#279718,#279719,#279720,#279721,#279722,
#279723,#279724,#279725,#279726,#279727,#279728,#279729,#279730,#279731,
#279732,#279733,#279734,#279735,#279736,#279737,#279738,#279739,#279740,
#279741,#279742,#279743,#279744,#279745,#279746,#279747,#279748,#279749,
#279750,#279751,#279752,#279753,#279754,#279755,#279756,#279757,#279758,
#279759,#279760,#279761,#279762,#279763,#279764,#279765,#279766,#279767,
#279768,#279769,#279770,#279771,#279772,#279773,#279774,#279775,#279776,
#279777,#279778,#279779,#279780,#279781,#279782,#279783,#279784,#279785,
#279786,#279787,#279788,#279789,#279790,#279791,#279792,#279793,#279794,
#279795,#279796,#279797,#279798,#279799,#279800,#279801,#279802,#279803,
#279804,#279805,#279806,#279807,#279808,#279809,#279810,#279811,#279812,
#279813,#279814,#279815,#279816,#279817,#279818,#279819,#279820,#279821,
#279822,#279823,#279824,#279825,#279826,#279827,#279828,#279829,#279830,
#279831,#279832,#279833,#279834,#279835,#279836,#279837,#279838,#279839,
#279840,#279841,#279842,#279843,#279844,#279845,#279846,#279847,#279848,
#279849,#279850,#279851,#279852,#279853,#279854,#279855,#279856,#279857,
#279858,#279859,#279860,#279861,#279862,#279863,#279864,#279865,#279866,
#279867,#279868,#279869,#279870,#279871,#279872,#279873,#279874,#279875,
#279876,#279877,#279878,#279879,#279880,#279881,#279882,#279883,#279884,
#279885,#279886,#279887,#279888,#279889,#279890,#279891,#279892,#279893,
#279894,#279895,#279896,#279897,#279898,#279899,#279900,#279901,#279902,
#279903,#279904,#279905,#279906,#279907,#279908,#279909,#279910,#279911,
#279912,#279913,#279914,#279915,#279916,#279917,#279918,#279919,#279920,
#279921,#279922,#279923,#279924,#279925,#279926,#279927,#279928,#279929,
#279930,#279931,#279932,#279933,#279934,#279935,#279936,#279937,#279938,
#279939,#279940,#279941,#279942,#279943,#279944,#279945,#279946,#279947,
#279948,#279949,#279950,#279951,#279952,#279953,#279954,#279955,#279956,
#279957,#279958,#279959,#279960,#279961,#279962,#279963,#279964,#279965,
#279966,#279967,#279968,#279969,#279970,#279971,#279972,#279973,#279974,
#279975,#279976,#279977,#279978,#279979,#279980,#279981,#279982,#279983,
#279984,#279985,#279986,#279987,#279988,#279989,#279990,#279991,#279992,
#279993,#279994,#279995,#279996,#279997,#279998,#279999,#280000,#280001,
#280002,#280003,#280004,#280005,#280006,#280007,#280008,#280009,#280010,
#280011,#280012,#280013,#280014,#280015,#280016,#280017,#280018,#280019,
#280020,#280021,#280022,#280023,#280024,#280025,#280026,#280027,#280028,
#280029,#280030,#280031,#280032,#280033,#280034,#280035,#280036,#280037,
#280038,#280039,#280040,#280041,#280042,#280043,#280044,#280045,#280046,
#280047,#280048,#280049,#280050,#280051,#280052,#280053,#280054,#280055,
#280056,#280057,#280058,#280059,#280060,#280061,#280062,#280063,#280064,
#280065,#280066,#280067,#280068,#280069,#280070,#280071,#280072,#280073,
#280074,#280075,#280076,#280077,#280078,#280079,#280080,#280081,#280082,
#280083,#280084,#280085,#280086,#280087,#280088,#280089,#280090,#280091,
#280092,#280093,#280094,#280095,#280096,#280097,#280098,#280099,#280100,
#280101,#280102,#280103,#280104,#280105,#280106,#280107,#280108,#280109,
#280110,#280111,#280112,#280113,#280114,#280115,#280116,#280117,#280118,
#280119,#280120,#280121,#280122,#280123,#280124,#280125,#280126,#280127,
#280128,#280129,#280130,#280131,#280132,#280133,#280134,#280135,#280136,
#280137,#280138,#280139,#280140,#280141,#280142,#280143,#280144,#280145,
#280146,#280147,#280148,#280149,#280150,#280151,#280152,#280153,#280154,
#280155,#280156,#280157,#280158,#280159,#280160,#280161,#280162,#280163,
#280164,#280165,#280166,#280167,#280168,#280169,#280170,#280171,#280172,
#280173,#280174,#280175,#280176,#280177,#280178,#280179,#280180,#280181,
#280182,#280183,#280184,#280185,#280186,#280187,#280188,#280189,#280190,
#280191,#280192,#280193,#280194,#280195,#280196,#280197,#280198,#280199,
#280200,#280201,#280202,#280203,#280204,#280205,#280206,#280207,#280208,
#280209,#280210,#280211,#280212,#280213,#280214,#280215,#280216,#280217,
#280218,#280219,#280220,#280221,#280222,#280223,#280224,#280225,#280226,
#280227,#280228,#280229,#280230,#280231,#280232,#280233,#280234,#280235,
#280236,#280237,#280238,#280239,#280240,#280241,#280242,#280243,#280244,
#280245,#280246,#280247,#280248,#280249,#280250,#280251,#280252,#280253,
#280254,#280255,#280256,#280257,#280258,#280259,#280260,#280261,#280262,
#280263,#280264,#280265,#280266,#280267,#280268,#280269,#280270,#280271,
#280272,#280273,#280274,#280275,#280276,#280277,#280278,#280279,#280280,
#280281,#280282,#280283,#280284,#280285,#280286,#280287,#280288,#280289,
#280290,#280291,#280292,#280293,#280294,#280295,#280296,#280297,#280298,
#280299,#280300,#280301,#280302,#280303,#280304,#280305,#280306,#280307,
#280308,#280309,#280310,#280311,#280312,#280313,#280314,#280315,#280316,
#280317,#280318,#280319,#280320,#280321,#280322,#280323,#280324,#280325,
#280326,#280327,#280328,#280329,#280330,#280331,#280332,#280333,#280334,
#280335,#280336,#280337,#280338,#280339,#280340,#280341,#280342,#280343,
#280344,#280345,#280346,#280347,#280348,#280349,#280350,#280351,#280352,
#280353,#280354,#280355,#280356,#280357,#280358,#280359,#280360,#280361,
#280362,#280363,#280364,#280365,#280366,#280367,#280368,#280369,#280370,
#280371,#280372,#280373,#280374,#280375,#280376,#280377,#280378,#280379,
#280380,#280381,#280382,#280383,#280384,#280385,#280386,#280387,#280388,
#280389,#280390,#280391,#280392,#280393,#280394,#280395,#280396,#280397,
#280398,#280399,#280400,#280401,#280402,#280403,#280404,#280405,#280406,
#280407,#280408,#280409,#280410,#280411,#280412,#280413,#280414,#280415,
#280416,#280417,#280418,#280419,#280420,#280421,#280422,#280423,#280424,
#280425,#280426,#280427,#280428,#280429,#280430,#280431,#280432,#280433,
#280434,#280435,#280436,#280437,#280438,#280439,#280440,#280441,#280442,
#280443,#280444,#280445,#280446,#280447,#280448,#280449,#280450,#280451,
#280452,#280453,#280454,#280455,#280456,#280457,#280458,#280459,#280460,
#280461,#280462,#280463,#280464,#280465,#280466,#280467,#280468,#280469,
#280470,#280471,#280472,#280473,#280474,#280475,#280476,#280477,#280478,
#280479,#280480,#280481,#280482,#280483,#280484,#280485,#280486,#280487,
#280488,#280489,#280490,#280491,#280492,#280493,#280494,#280495,#280496,
#280497,#280498,#280499,#280500,#280501,#280502,#280503,#280504,#280505,
#280506,#280507,#280508,#280509,#280510,#280511,#280512,#280513,#280514,
#280515,#280516,#280517,#280518,#280519,#280520,#280521,#280522,#280523,
#280524,#280525,#280526,#280527,#280528,#280529,#280530,#280531,#280532,
#280533,#280534,#280535,#280536,#280537,#280538,#280539,#280540,#280541,
#280542,#280543,#280544,#280545,#280546,#280547,#280548,#280549,#280550,
#280551,#280552,#280553,#280554,#280555,#280556,#280557,#280558,#280559,
#280560,#280561,#280562,#280563,#280564,#280565,#280566,#280567,#280568,
#280569,#280570,#280571,#280572,#280573,#280574,#280575,#280576,#280577,
#280578,#280579,#280580,#280581,#280582,#280583,#280584,#280585,#280586,
#280587,#280588,#280589,#280590,#280591,#280592,#280593,#280594,#280595,
#280596,#280597,#280598,#280599,#280600,#280601,#280602,#280603,#280604,
#280605,#280606,#280607,#280608,#280609,#280610,#280611,#280612,#280613,
#280614,#280615,#280616,#280617,#280618,#280619,#280620)),.UNSPECIFIED.,
 .F.,.F.,.F.)
B_SPLINE_SURFACE_WITH_KNOTS((2,2),(3,2,2,2,2,2,2,2,2,2,2,2,2,2,2,2,2,2,
2,2,2,2,2,2,2,2,2,2,2,2,2,2,2,2,2,2,2,2,2,2,2,2,2,2,2,2,2,2,2,2,2,2,2,2,
2,2,2,2,2,2,2,2,2,2,2,2,2,2,2,2,2,2,2,2,2,2,2,2,2,2,2,2,2,2,2,2,2,2,2,2,
2,2,2,2,2,2,2,2,2,2,2,2,2,2,2,2,2,2,2,2,2,2,2,2,2,2,2,2,2,2,2,2,2,2,2,2,
2,2,2,2,2,2,2,2,2,2,2,2,2,2,2,2,2,2,2,2,2,2,2,2,2,2,2,2,2,2,2,2,2,2,2,2,
2,2,2,2,2,2,2,2,2,2,2,2,2,2,2,2,2,2,2,2,2,2,2,2,2,2,2,2,2,2,2,2,2,2,2,2,
2,2,2,2,2,2,2,2,2,2,2,2,2,2,2,2,2,2,2,2,2,2,2,2,2,2,2,2,2,2,2,2,2,2,2,2,
2,2,2,2,2,2,2,2,2,2,2,2,2,2,2,2,2,2,2,2,2,2,2,2,2,2,2,2,2,2,2,2,2,2,2,2,
2,2,2,2,2,2,2,2,2,2,2,2,2,2,2,2,2,2,2,2,2,2,2,2,2,2,2,2,2,2,2,2,2,2,2,2,
2,2,2,2,2,2,2,2,2,2,2,2,2,2,2,2,2,2,2,2,2,2,2,2,2,2,2,2,2,2,2,2,2,2,2,2,
2,2,2,2,2,2,2,2,2,2,2,2,2,2,2,2,2,2,2,2,2,2,2,2,2,2,2,2,2,2,2,2,2,2,2,2,
2,2,2,2,2,2,2,2,2,2,2,2,2,2,2,2,2,2,2,2,2,2,2,2,2,2,2,2,2,2,2,2,2,2,2,2,
2,2,2,2,2,2,2,2,2,2,2,2,2,2,2,2,2,2,2,2,2,2,2,2,2,2,2,2,2,2,2,2,2,2,2,2,
2,2,2,2,2,2,2,2,2,2,2,2,2,2,2,2,2,2,2,2,2,2,2,2,2,2,2,2,2,2,2,2,2,2,2,2,
2,2,2,2,2,2,2,2,2,2,2,2,2,2,2,2,2,2,2,2,2,2,2,2,2,2,2,2,2,2,2,2,3),(0.,
1.00000707949272),(0.,0.00192307692307692,0.00384615384615385,0.00576923076923077,
0.00769230769230769,0.00961538461538462,0.0115384615384615,0.0134615384615385,
0.0153846153846154,0.0173076923076923,0.0192307692307692,0.0211538461538462,
0.0230769230769231,0.025,0.0269230769230769,0.0288461538461538,0.0307692307692308,
0.0326923076923077,0.0346153846153846,0.0365384615384615,0.0384615384615385,
0.0403846153846154,0.0423076923076923,0.0442307692307692,0.0461538461538462,
0.0480769230769231,0.05,0.0519230769230769,0.0538461538461538,0.0557692307692308,
0.0576923076923077,0.0596153846153846,0.0615384615384615,0.0634615384615385,
0.0653846153846154,0.0673076923076923,0.0692307692307692,0.0711538461538462,
0.0730769230769231,0.075,0.0769230769230769,0.0788461538461538,0.0807692307692308,
0.0826923076923077,0.0846153846153846,0.0865384615384615,0.0884615384615385,
0.0903846153846154,0.0923076923076923,0.0942307692307692,0.0961538461538462,
0.0980769230769231,0.1,0.101923076923077,0.103846153846154,0.105769230769231,
0.107692307692308,0.109615384615385,0.111538461538462,0.113461538461538,
0.115384615384615,0.117307692307692,0.119230769230769,0.121153846153846,
0.123076923076923,0.125,0.126923076923077,0.128846153846154,0.130769230769231,
0.132692307692308,0.134615384615385,0.136538461538462,0.138461538461538,
0.140384615384615,0.142307692307692,0.144230769230769,0.146153846153846,
0.148076923076923,0.15,0.151923076923077,0.153846153846154,0.155769230769231,
0.157692307692308,0.159615384615385,0.161538461538462,0.163461538461538,
0.165384615384615,0.167307692307692,0.169230769230769,0.171153846153846,
0.173076923076923,0.175,0.176923076923077,0.178846153846154,0.180769230769231,
0.182692307692308,0.184615384615385,0.186538461538462,0.188461538461538,
0.190384615384615,0.192307692307692,0.194230769230769,0.196153846153846,
0.198076923076923,0.2,0.201923076923077,0.203846153846154,0.205769230769231,
0.207692307692308,0.209615384615385,0.211538461538462,0.213461538461538,
0.215384615384615,0.217307692307692,0.219230769230769,0.221153846153846,
0.223076923076923,0.225,0.226923076923077,0.228846153846154,0.230769230769231,
0.232692307692308,0.234615384615385,0.236538461538462,0.238461538461538,
0.240384615384615,0.242307692307692,0.244230769230769,0.246153846153846,
0.248076923076923,0.25,0.251923076923077,0.253846153846154,0.255769230769231,
0.257692307692308,0.259615384615385,0.261538461538462,0.263461538461538,
0.265384615384615,0.267307692307692,0.269230769230769,0.271153846153846,
0.273076923076923,0.275,0.276923076923077,0.278846153846154,0.280769230769231,
0.282692307692308,0.284615384615385,0.286538461538462,0.288461538461538,
0.290384615384615,0.292307692307692,0.294230769230769,0.296153846153846,
0.298076923076923,0.3,0.301923076923077,0.303846153846154,0.305769230769231,
0.307692307692308,0.309615384615385,0.311538461538462,0.313461538461538,
0.315384615384615,0.317307692307692,0.319230769230769,0.321153846153846,
0.323076923076923,0.325,0.326923076923077,0.328846153846154,0.330769230769231,
0.332692307692308,0.334615384615385,0.336538461538462,0.338461538461538,
0.340384615384615,0.342307692307692,0.344230769230769,0.346153846153846,
0.348076923076923,0.35,0.351923076923077,0.353846153846154,0.355769230769231,
0.357692307692308,0.359615384615385,0.361538461538462,0.363461538461538,
0.365384615384615,0.367307692307692,0.369230769230769,0.371153846153846,
0.373076923076923,0.375,0.376923076923077,0.378846153846154,0.380769230769231,
0.382692307692308,0.384615384615385,0.386538461538462,0.388461538461538,
0.390384615384615,0.392307692307692,0.394230769230769,0.396153846153846,
0.398076923076923,0.4,0.401923076923077,0.403846153846154,0.405769230769231,
0.407692307692308,0.409615384615385,0.411538461538462,0.413461538461538,
0.415384615384615,0.417307692307692,0.419230769230769,0.421153846153846,
0.423076923076923,0.425,0.426923076923077,0.428846153846154,0.430769230769231,
0.432692307692308,0.434615384615385,0.436538461538462,0.438461538461538,
0.440384615384615,0.442307692307692,0.444230769230769,0.446153846153846,
0.448076923076923,0.45,0.451923076923077,0.453846153846154,0.455769230769231,
0.457692307692308,0.459615384615385,0.461538461538462,0.463461538461538,
0.465384615384615,0.467307692307692,0.469230769230769,0.471153846153846,
0.473076923076923,0.475,0.476923076923077,0.478846153846154,0.480769230769231,
0.482692307692308,0.484615384615385,0.486538461538462,0.488461538461538,
0.490384615384615,0.492307692307692,0.494230769230769,0.496153846153846,
0.498076923076923,0.5,0.501923076923077,0.503846153846154,0.505769230769231,
0.507692307692308,0.509615384615385,0.511538461538461,0.513461538461538,
0.515384615384615,0.517307692307692,0.519230769230769,0.521153846153846,
0.523076923076923,0.525,0.526923076923077,0.528846153846154,0.530769230769231,
0.532692307692308,0.534615384615385,0.536538461538462,0.538461538461538,
0.540384615384615,0.542307692307692,0.544230769230769,0.546153846153846,
0.548076923076923,0.55,0.551923076923077,0.553846153846154,0.555769230769231,
0.557692307692308,0.559615384615385,0.561538461538462,0.563461538461538,
0.565384615384615,0.567307692307692,0.569230769230769,0.571153846153846,
0.573076923076923,0.575,0.576923076923077,0.578846153846154,0.580769230769231,
0.582692307692308,0.584615384615385,0.586538461538462,0.588461538461538,
0.590384615384615,0.592307692307692,0.594230769230769,0.596153846153846,
0.598076923076923,0.6,0.601923076923077,0.603846153846154,0.605769230769231,
0.607692307692308,0.609615384615385,0.611538461538462,0.613461538461539,
0.615384615384615,0.617307692307692,0.619230769230769,0.621153846153846,
0.623076923076923,0.625,0.626923076923077,0.628846153846154,0.630769230769231,
0.632692307692308,0.634615384615385,0.636538461538461,0.638461538461538,
0.640384615384615,0.642307692307692,0.644230769230769,0.646153846153846,
0.648076923076923,0.65,0.651923076923077,0.653846153846154,0.655769230769231,
0.657692307692308,0.659615384615385,0.661538461538462,0.663461538461538,
0.665384615384615,0.667307692307692,0.669230769230769,0.671153846153846,
0.673076923076923,0.675,0.676923076923077,0.678846153846154,0.680769230769231,
0.682692307692308,0.684615384615385,0.686538461538462,0.688461538461538,
0.690384615384615,0.692307692307692,0.694230769230769,0.696153846153846,
0.698076923076923,0.7,0.701923076923077,0.703846153846154,0.705769230769231,
0.707692307692308,0.709615384615385,0.711538461538462,0.713461538461538,
0.715384615384615,0.717307692307692,0.719230769230769,0.721153846153846,
0.723076923076923,0.725,0.726923076923077,0.728846153846154,0.730769230769231,
0.732692307692308,0.734615384615385,0.736538461538462,0.738461538461539,
0.740384615384615,0.742307692307692,0.744230769230769,0.746153846153846,
0.748076923076923,0.75,0.751923076923077,0.753846153846154,0.755769230769231,
0.757692307692308,0.759615384615385,0.761538461538461,0.763461538461538,
0.765384615384615,0.767307692307692,0.769230769230769,0.771153846153846,
0.773076923076923,0.775,0.776923076923077,0.778846153846154,0.780769230769231,
0.782692307692308,0.784615384615385,0.786538461538462,0.788461538461538,
0.790384615384615,0.792307692307692,0.794230769230769,0.796153846153846,
0.798076923076923,0.8,0.801923076923077,0.803846153846154,0.805769230769231,
0.807692307692308,0.809615384615385,0.811538461538462,0.813461538461538,
0.815384615384615,0.817307692307692,0.819230769230769,0.821153846153846,
0.823076923076923,0.825,0.826923076923077,0.828846153846154,0.830769230769231,
0.832692307692308,0.834615384615385,0.836538461538462,0.838461538461538,
0.840384615384615,0.842307692307692,0.844230769230769,0.846153846153846,
0.848076923076923,0.85,0.851923076923077,0.853846153846154,0.855769230769231,
0.857692307692308,0.859615384615385,0.861538461538462,0.863461538461539,
0.865384615384615,0.867307692307692,0.869230769230769,0.871153846153846,
0.873076923076923,0.875,0.876923076923077,0.878846153846154,0.880769230769231,
0.882692307692308,0.884615384615385,0.886538461538461,0.888461538461538,
0.890384615384615,0.892307692307692,0.894230769230769,0.896153846153846,
0.898076923076923,0.9,0.901923076923077,0.903846153846154,0.905769230769231,
0.907692307692308,0.909615384615385,0.911538461538462,0.913461538461538,
0.915384615384615,0.917307692307692,0.919230769230769,0.921153846153846,
0.923076923076923,0.925,0.926923076923077,0.928846153846154,0.930769230769231,
0.932692307692308,0.934615384615385,0.936538461538462,0.938461538461538,
0.940384615384615,0.942307692307692,0.944230769230769,0.946153846153846,
0.948076923076923,0.95,0.951923076923077,0.953846153846154,0.955769230769231,
0.957692307692308,0.959615384615385,0.961538461538462,0.963461538461538,
0.965384615384615,0.967307692307692,0.969230769230769,0.971153846153846,
0.973076923076923,0.975,0.976923076923077,0.978846153846154,0.980769230769231,
0.982692307692308,0.984615384615385,0.986538461538462,0.988461538461539,
0.990384615384615,0.992307692307692,0.994230769230769,0.996153846153846),
 .UNSPECIFIED.)
GEOMETRIC_REPRESENTATION_ITEM()
RATIONAL_B_SPLINE_SURFACE(((1.,0.951056516295154,1.,0.951056516295154,1.,
0.951056516295154,1.,0.951056516295154,1.,0.951056516295154,1.,0.951056516295154,
1.,0.951056516295154,1.,0.951056516295154,1.,0.951056516295154,1.,0.951056516295154,
1.,0.951056516295154,1.,0.951056516295154,1.,0.951056516295154,1.,0.951056516295154,
1.,0.951056516295154,1.,0.951056516295154,1.,0.951056516295154,1.,0.951056516295154,
1.,0.951056516295154,1.,0.951056516295154,1.,0.951056516295154,1.,0.951056516295154,
1.,0.951056516295154,1.,0.951056516295154,1.,0.951056516295154,1.,0.951056516295154,
1.,0.951056516295154,1.,0.951056516295154,1.,0.951056516295154,1.,0.951056516295154,
1.,0.951056516295154,1.,0.951056516295154,1.,0.951056516295154,1.,0.951056516295154,
1.,0.951056516295154,1.,0.951056516295154,1.,0.951056516295154,1.,0.951056516295154,
1.,0.951056516295154,1.,0.951056516295154,1.,0.951056516295154,1.,0.951056516295154,
1.,0.951056516295154,1.,0.951056516295154,1.,0.951056516295154,1.,0.951056516295154,
1.,0.951056516295154,1.,0.951056516295154,1.,0.951056516295154,1.,0.951056516295154,
1.,0.951056516295154,1.,0.951056516295154,1.,0.951056516295154,1.,0.951056516295154,
1.,0.951056516295154,1.,0.951056516295154,1.,0.951056516295154,1.,0.951056516295154,
1.,0.951056516295154,1.,0.951056516295154,1.,0.951056516295154,1.,0.951056516295154,
1.,0.951056516295154,1.,0.951056516295154,1.,0.951056516295154,1.,0.951056516295154,
1.,0.951056516295154,1.,0.951056516295154,1.,0.951056516295154,1.,0.951056516295154,
1.,0.951056516295154,1.,0.951056516295154,1.,0.951056516295154,1.,0.951056516295154,
1.,0.951056516295154,1.,0.951056516295154,1.,0.951056516295154,1.,0.951056516295154,
1.,0.951056516295154,1.,0.951056516295154,1.,0.951056516295154,1.,0.951056516295154,
1.,0.951056516295154,1.,0.951056516295154,1.,0.951056516295154,1.,0.951056516295154,
1.,0.951056516295154,1.,0.951056516295154,1.,0.951056516295154,1.,0.951056516295154,
1.,0.951056516295154,1.,0.951056516295154,1.,0.951056516295154,1.,0.951056516295154,
1.,0.951056516295154,1.,0.951056516295154,1.,0.951056516295154,1.,0.951056516295154,
1.,0.951056516295154,1.,0.951056516295154,1.,0.951056516295154,1.,0.951056516295154,
1.,0.951056516295154,1.,0.951056516295154,1.,0.951056516295154,1.,0.951056516295154,
1.,0.951056516295154,1.,0.951056516295154,1.,0.951056516295154,1.,0.951056516295154,
1.,0.951056516295154,1.,0.951056516295154,1.,0.951056516295154,1.,0.951056516295154,
1.,0.951056516295154,1.,0.951056516295154,1.,0.951056516295154,1.,0.951056516295154,
1.,0.951056516295154,1.,0.951056516295154,1.,0.951056516295154,1.,0.951056516295154,
1.,0.951056516295154,1.,0.951056516295154,1.,0.951056516295154,1.,0.951056516295154,
1.,0.951056516295154,1.,0.951056516295154,1.,0.951056516295154,1.,0.951056516295154,
1.,0.951056516295154,1.,0.951056516295154,1.,0.951056516295154,1.,0.951056516295154,
1.,0.951056516295154,1.,0.951056516295154,1.,0.951056516295154,1.,0.951056516295154,
1.,0.951056516295154,1.,0.951056516295154,1.,0.951056516295154,1.,0.951056516295154,
1.,0.951056516295154,1.,0.951056516295154,1.,0.951056516295154,1.,0.951056516295154,
1.,0.951056516295154,1.,0.951056516295154,1.,0.951056516295154,1.,0.951056516295154,
1.,0.951056516295154,1.,0.951056516295154,1.,0.951056516295154,1.,0.951056516295154,
1.,0.951056516295154,1.,0.951056516295154,1.,0.951056516295154,1.,0.951056516295154,
1.,0.951056516295154,1.,0.951056516295154,1.,0.951056516295154,1.,0.951056516295154,
1.,0.951056516295154,1.,0.951056516295154,1.,0.951056516295154,1.,0.951056516295154,
1.,0.951056516295154,1.,0.951056516295154,1.,0.951056516295154,1.,0.951056516295154,
1.,0.951056516295154,1.,0.951056516295154,1.,0.951056516295154,1.,0.951056516295154,
1.,0.951056516295154,1.,0.951056516295154,1.,0.951056516295154,1.,0.951056516295154,
1.,0.951056516295154,1.,0.951056516295154,1.,0.951056516295154,1.,0.951056516295154,
1.,0.951056516295154,1.,0.951056516295154,1.,0.951056516295154,1.,0.951056516295154,
1.,0.951056516295154,1.,0.951056516295154,1.,0.951056516295154,1.,0.951056516295154,
1.,0.951056516295154,1.,0.951056516295154,1.,0.951056516295154,1.,0.951056516295154,
1.,0.951056516295154,1.,0.951056516295154,1.,0.951056516295154,1.,0.951056516295154,
1.,0.951056516295154,1.,0.951056516295154,1.,0.951056516295154,1.,0.951056516295154,
1.,0.951056516295154,1.,0.951056516295154,1.,0.951056516295154,1.,0.951056516295154,
1.,0.951056516295154,1.,0.951056516295154,1.,0.951056516295154,1.,0.951056516295154,
1.,0.951056516295154,1.,0.951056516295154,1.,0.951056516295154,1.,0.951056516295154,
1.,0.951056516295154,1.,0.951056516295154,1.,0.951056516295154,1.,0.951056516295154,
1.,0.951056516295154,1.,0.951056516295154,1.,0.951056516295154,1.,0.951056516295154,
1.,0.951056516295154,1.,0.951056516295154,1.,0.951056516295154,1.,0.951056516295154,
1.,0.951056516295154,1.,0.951056516295154,1.,0.951056516295154,1.,0.951056516295154,
1.,0.951056516295154,1.,0.951056516295154,1.,0.951056516295154,1.,0.951056516295154,
1.,0.951056516295154,1.,0.951056516295154,1.,0.951056516295154,1.,0.951056516295154,
1.,0.951056516295154,1.,0.951056516295154,1.,0.951056516295154,1.,0.951056516295154,
1.,0.951056516295154,1.,0.951056516295154,1.,0.951056516295154,1.,0.951056516295154,
1.,0.951056516295154,1.,0.951056516295154,1.,0.951056516295154,1.,0.951056516295154,
1.,0.951056516295154,1.,0.951056516295154,1.,0.951056516295154,1.,0.951056516295154,
1.,0.951056516295154,1.,0.951056516295154,1.,0.951056516295154,1.,0.951056516295154,
1.,0.951056516295154,1.,0.951056516295154,1.,0.951056516295154,1.,0.951056516295154,
1.,0.951056516295154,1.,0.951056516295154,1.,0.951056516295154,1.,0.951056516295154,
1.,0.951056516295154,1.,0.951056516295154,1.,0.951056516295154,1.,0.951056516295154,
1.,0.951056516295154,1.,0.951056516295154,1.,0.951056516295154,1.,0.951056516295154,
1.,0.951056516295154,1.,0.951056516295154,1.,0.951056516295154,1.,0.951056516295154,
1.,0.951056516295154,1.,0.951056516295154,1.,0.951056516295154,1.,0.951056516295154,
1.,0.951056516295154,1.,0.951056516295154,1.,0.951056516295154,1.,0.951056516295154,
1.,0.951056516295154,1.,0.951056516295154,1.,0.951056516295154,1.,0.951056516295154,
1.,0.951056516295154,1.,0.951056516295154,1.,0.951056516295154,1.,0.951056516295154,
1.,0.951056516295154,1.,0.951056516295154,1.,0.951056516295154,1.,0.951056516295154,
1.,0.951056516295154,1.,0.951056516295154,1.,0.951056516295154,1.,0.951056516295154,
1.,0.951056516295154,1.,0.951056516295154,1.,0.951056516295154,1.,0.951056516295154,
1.,0.951056516295154,1.,0.951056516295154,1.,0.951056516295154,1.,0.951056516295154,
1.,0.951056516295154,1.,0.951056516295154,1.,0.951056516295154,1.,0.951056516295154,
1.,0.951056516295154,1.,0.951056516295154,1.,0.951056516295154,1.,0.951056516295154,
1.,0.951056516295154,1.,0.951056516295154,1.,0.951056516295154,1.,0.951056516295154,
1.,0.951056516295154,1.,0.951056516295154,1.,0.951056516295154,1.,0.951056516295154,
1.,0.951056516295154,1.,0.951056516295154,1.,0.951056516295154,1.,0.951056516295154,
1.,0.951056516295154,1.,0.951056516295154,1.,0.951056516295154,1.,0.951056516295154,
1.,0.951056516295154,1.,0.951056516295154,1.,0.951056516295154,1.,0.951056516295154,
1.,0.951056516295154,1.,0.951056516295154,1.,0.951056516295154,1.,0.951056516295154,
1.,0.951056516295154,1.,0.951056516295154,1.,0.951056516295154,1.,0.951056516295154,
1.,0.951056516295154,1.,0.951056516295154,1.,0.951056516295154,1.,0.951056516295154,
1.,0.951056516295154,1.,0.951056516295154,1.,0.951056516295154,1.,0.951056516295154,
1.,0.951056516295154,1.,0.951056516295154,1.,0.951056516295154,1.,0.951056516295154,
1.,0.951056516295154,1.,0.951056516295154,1.,0.951056516295154,1.,0.951056516295154,
1.,0.951056516295154,1.,0.951056516295154,1.,0.951056516295154,1.,0.951056516295154,
1.,0.951056516295154,1.,0.951056516295154,1.,0.951056516295154,1.,0.951056516295154,
1.,0.951056516295154,1.,0.951056516295154,1.,0.951056516295154,1.,0.951056516295154,
1.,0.951056516295154,1.,0.951056516295154,1.,0.951056516295154,1.,0.951056516295154,
1.,0.951056516295154,1.,0.951056516295154,1.,0.951056516295154,1.,0.951056516295154,
1.,0.951056516295154,1.,0.951056516295154,1.,0.951056516295154,1.,0.951056516295154,
1.,0.951056516295154,1.,0.951056516295154,1.,0.951056516295154,1.,0.951056516295154,
1.,0.951056516295154,1.,0.951056516295154,1.,0.951056516295154,1.,0.951056516295154,
1.,0.951056516295154,1.,0.951056516295154,1.,0.951056516295154,1.,0.951056516295154,
1.,0.951056516295154,1.,0.951056516295154,1.,0.951056516295154,1.,0.951056516295154,
1.,0.951056516295154,1.,0.951056516295154,1.,0.951056516295154,1.,0.951056516295154,
1.,0.951056516295154,1.,0.951056516295154,1.,0.951056516295154,1.,0.951056516295154,
1.,0.951056516295154,1.,0.951056516295154,1.,0.951056516295154,1.,0.951056516295154,
1.,0.951056516295154,1.,0.951056516295154,1.,0.951056516295154,1.,0.951056516295154,
1.,0.951056516295154,1.,0.951056516295154,1.,0.951056516295154,1.,0.951056516295154,
1.,0.951056516295154,1.,0.951056516295154,1.,0.951056516295154,1.,0.951056516295154,
1.,0.951056516295154,1.,0.951056516295154,1.,0.951056516295154,1.,0.951056516295154,
1.,0.951056516295154,1.,0.951056516295154,1.,0.951056516295154,1.,0.951056516295154,
1.,0.951056516295154,1.,0.951056516295154,1.,0.951056516295154,1.,0.951056516295154,
1.,0.951056516295154,1.,0.951056516295154,1.,0.951056516295154,1.,0.951056516295154,
1.,0.951056516295154,1.,0.951056516295154,1.,0.951056516295154,1.,0.951056516295154,
1.,0.951056516295154,1.,0.951056516295154,1.,0.951056516295154,1.,0.951056516295154,
1.,0.951056516295154,1.,0.951056516295154,1.,0.951056516295154,1.,0.951056516295154,
1.,0.951056516295154,1.,0.951056516295154,1.,0.951056516295154,1.,0.951056516295154,
1.,0.951056516295154,1.,0.951056516295154,1.,0.951056516295154,1.,0.951056516295154,
1.,0.951056516295154,1.,0.951056516295154,1.,0.951056516295154,1.,0.951056516295154,
1.,0.951056516295154,1.,0.951056516295154,1.,0.951056516295154,1.,0.951056516295154,
1.,0.951056516295154,1.,0.951056516295154,1.,0.951056516295154,1.,0.951056516295154,
1.,0.951056516295154,1.,0.951056516295154,1.,0.951056516295154,1.,0.951056516295154,
1.,0.951056516295154,1.,0.951056516295154,1.,0.951056516295154,1.,0.951056516295154,
1.,0.951056516295154,1.,0.951056516295154,1.,0.951056516295154,1.,0.951056516295154,
1.,0.951056516295154,1.,0.951056516295154,1.,0.951056516295154,1.,0.951056516295154,
1.,0.951056516295154,1.,0.951056516295154,1.,0.951056516295154,1.,0.951056516295154,
1.,0.951056516295154,1.,0.951056516295154,1.,0.951056516295154,1.,0.951056516295154,
1.,0.951056516295154,1.,0.951056516295154,1.,0.951056516295154,1.,0.951056516295154,
1.,0.951056516295154,1.,0.951056516295154,1.,0.951056516295154,1.,0.951056516295154,
1.,0.951056516295154,1.,0.951056516295154,1.,0.951056516295154,1.,0.951056516295154,
1.,0.951056516295154,1.,0.951056516295154,1.,0.951056516295154,1.,0.951056516295154,
1.,0.951056516295154,1.,0.951056516295154,1.,0.951056516295154,1.,0.951056516295154,
1.),(1.,0.951056516295154,1.,0.951056516295154,1.,0.951056516295154,1.,
0.951056516295154,1.,0.951056516295154,1.,0.951056516295154,1.,0.951056516295154,
1.,0.951056516295154,1.,0.951056516295154,1.,0.951056516295154,1.,0.951056516295154,
1.,0.951056516295154,1.,0.951056516295154,1.,0.951056516295154,1.,0.951056516295154,
1.,0.951056516295154,1.,0.951056516295154,1.,0.951056516295154,1.,0.951056516295154,
1.,0.951056516295154,1.,0.951056516295154,1.,0.951056516295154,1.,0.951056516295154,
1.,0.951056516295154,1.,0.951056516295154,1.,0.951056516295154,1.,0.951056516295154,
1.,0.951056516295154,1.,0.951056516295154,1.,0.951056516295154,1.,0.951056516295154,
1.,0.951056516295154,1.,0.951056516295154,1.,0.951056516295154,1.,0.951056516295154,
1.,0.951056516295154,1.,0.951056516295154,1.,0.951056516295154,1.,0.951056516295154,
1.,0.951056516295154,1.,0.951056516295154,1.,0.951056516295154,1.,0.951056516295154,
1.,0.951056516295154,1.,0.951056516295154,1.,0.951056516295154,1.,0.951056516295154,
1.,0.951056516295154,1.,0.951056516295154,1.,0.951056516295154,1.,0.951056516295154,
1.,0.951056516295154,1.,0.951056516295154,1.,0.951056516295154,1.,0.951056516295154,
1.,0.951056516295154,1.,0.951056516295154,1.,0.951056516295154,1.,0.951056516295154,
1.,0.951056516295154,1.,0.951056516295154,1.,0.951056516295154,1.,0.951056516295154,
1.,0.951056516295154,1.,0.951056516295154,1.,0.951056516295154,1.,0.951056516295154,
1.,0.951056516295154,1.,0.951056516295154,1.,0.951056516295154,1.,0.951056516295154,
1.,0.951056516295154,1.,0.951056516295154,1.,0.951056516295154,1.,0.951056516295154,
1.,0.951056516295154,1.,0.951056516295154,1.,0.951056516295154,1.,0.951056516295154,
1.,0.951056516295154,1.,0.951056516295154,1.,0.951056516295154,1.,0.951056516295154,
1.,0.951056516295154,1.,0.951056516295154,1.,0.951056516295154,1.,0.951056516295154,
1.,0.951056516295154,1.,0.951056516295154,1.,0.951056516295154,1.,0.951056516295154,
1.,0.951056516295154,1.,0.951056516295154,1.,0.951056516295154,1.,0.951056516295154,
1.,0.951056516295154,1.,0.951056516295154,1.,0.951056516295154,1.,0.951056516295154,
1.,0.951056516295154,1.,0.951056516295154,1.,0.951056516295154,1.,0.951056516295154,
1.,0.951056516295154,1.,0.951056516295154,1.,0.951056516295154,1.,0.951056516295154,
1.,0.951056516295154,1.,0.951056516295154,1.,0.951056516295154,1.,0.951056516295154,
1.,0.951056516295154,1.,0.951056516295154,1.,0.951056516295154,1.,0.951056516295154,
1.,0.951056516295154,1.,0.951056516295154,1.,0.951056516295154,1.,0.951056516295154,
1.,0.951056516295154,1.,0.951056516295154,1.,0.951056516295154,1.,0.951056516295154,
1.,0.951056516295154,1.,0.951056516295154,1.,0.951056516295154,1.,0.951056516295154,
1.,0.951056516295154,1.,0.951056516295154,1.,0.951056516295154,1.,0.951056516295154,
1.,0.951056516295154,1.,0.951056516295154,1.,0.951056516295154,1.,0.951056516295154,
1.,0.951056516295154,1.,0.951056516295154,1.,0.951056516295154,1.,0.951056516295154,
1.,0.951056516295154,1.,0.951056516295154,1.,0.951056516295154,1.,0.951056516295154,
1.,0.951056516295154,1.,0.951056516295154,1.,0.951056516295154,1.,0.951056516295154,
1.,0.951056516295154,1.,0.951056516295154,1.,0.951056516295154,1.,0.951056516295154,
1.,0.951056516295154,1.,0.951056516295154,1.,0.951056516295154,1.,0.951056516295154,
1.,0.951056516295154,1.,0.951056516295154,1.,0.951056516295154,1.,0.951056516295154,
1.,0.951056516295154,1.,0.951056516295154,1.,0.951056516295154,1.,0.951056516295154,
1.,0.951056516295154,1.,0.951056516295154,1.,0.951056516295154,1.,0.951056516295154,
1.,0.951056516295154,1.,0.951056516295154,1.,0.951056516295154,1.,0.951056516295154,
1.,0.951056516295154,1.,0.951056516295154,1.,0.951056516295154,1.,0.951056516295154,
1.,0.951056516295154,1.,0.951056516295154,1.,0.951056516295154,1.,0.951056516295154,
1.,0.951056516295154,1.,0.951056516295154,1.,0.951056516295154,1.,0.951056516295154,
1.,0.951056516295154,1.,0.951056516295154,1.,0.951056516295154,1.,0.951056516295154,
1.,0.951056516295154,1.,0.951056516295154,1.,0.951056516295154,1.,0.951056516295154,
1.,0.951056516295154,1.,0.951056516295154,1.,0.951056516295154,1.,0.951056516295154,
1.,0.951056516295154,1.,0.951056516295154,1.,0.951056516295154,1.,0.951056516295154,
1.,0.951056516295154,1.,0.951056516295154,1.,0.951056516295154,1.,0.951056516295154,
1.,0.951056516295154,1.,0.951056516295154,1.,0.951056516295154,1.,0.951056516295154,
1.,0.951056516295154,1.,0.951056516295154,1.,0.951056516295154,1.,0.951056516295154,
1.,0.951056516295154,1.,0.951056516295154,1.,0.951056516295154,1.,0.951056516295154,
1.,0.951056516295154,1.,0.951056516295154,1.,0.951056516295154,1.,0.951056516295154,
1.,0.951056516295154,1.,0.951056516295154,1.,0.951056516295154,1.,0.951056516295154,
1.,0.951056516295154,1.,0.951056516295154,1.,0.951056516295154,1.,0.951056516295154,
1.,0.951056516295154,1.,0.951056516295154,1.,0.951056516295154,1.,0.951056516295154,
1.,0.951056516295154,1.,0.951056516295154,1.,0.951056516295154,1.,0.951056516295154,
1.,0.951056516295154,1.,0.951056516295154,1.,0.951056516295154,1.,0.951056516295154,
1.,0.951056516295154,1.,0.951056516295154,1.,0.951056516295154,1.,0.951056516295154,
1.,0.951056516295154,1.,0.951056516295154,1.,0.951056516295154,1.,0.951056516295154,
1.,0.951056516295154,1.,0.951056516295154,1.,0.951056516295154,1.,0.951056516295154,
1.,0.951056516295154,1.,0.951056516295154,1.,0.951056516295154,1.,0.951056516295154,
1.,0.951056516295154,1.,0.951056516295154,1.,0.951056516295154,1.,0.951056516295154,
1.,0.951056516295154,1.,0.951056516295154,1.,0.951056516295154,1.,0.951056516295154,
1.,0.951056516295154,1.,0.951056516295154,1.,0.951056516295154,1.,0.951056516295154,
1.,0.951056516295154,1.,0.951056516295154,1.,0.951056516295154,1.,0.951056516295154,
1.,0.951056516295154,1.,0.951056516295154,1.,0.951056516295154,1.,0.951056516295154,
1.,0.951056516295154,1.,0.951056516295154,1.,0.951056516295154,1.,0.951056516295154,
1.,0.951056516295154,1.,0.951056516295154,1.,0.951056516295154,1.,0.951056516295154,
1.,0.951056516295154,1.,0.951056516295154,1.,0.951056516295154,1.,0.951056516295154,
1.,0.951056516295154,1.,0.951056516295154,1.,0.951056516295154,1.,0.951056516295154,
1.,0.951056516295154,1.,0.951056516295154,1.,0.951056516295154,1.,0.951056516295154,
1.,0.951056516295154,1.,0.951056516295154,1.,0.951056516295154,1.,0.951056516295154,
1.,0.951056516295154,1.,0.951056516295154,1.,0.951056516295154,1.,0.951056516295154,
1.,0.951056516295154,1.,0.951056516295154,1.,0.951056516295154,1.,0.951056516295154,
1.,0.951056516295154,1.,0.951056516295154,1.,0.951056516295154,1.,0.951056516295154,
1.,0.951056516295154,1.,0.951056516295154,1.,0.951056516295154,1.,0.951056516295154,
1.,0.951056516295154,1.,0.951056516295154,1.,0.951056516295154,1.,0.951056516295154,
1.,0.951056516295154,1.,0.951056516295154,1.,0.951056516295154,1.,0.951056516295154,
1.,0.951056516295154,1.,0.951056516295154,1.,0.951056516295154,1.,0.951056516295154,
1.,0.951056516295154,1.,0.951056516295154,1.,0.951056516295154,1.,0.951056516295154,
1.,0.951056516295154,1.,0.951056516295154,1.,0.951056516295154,1.,0.951056516295154,
1.,0.951056516295154,1.,0.951056516295154,1.,0.951056516295154,1.,0.951056516295154,
1.,0.951056516295154,1.,0.951056516295154,1.,0.951056516295154,1.,0.951056516295154,
1.,0.951056516295154,1.,0.951056516295154,1.,0.951056516295154,1.,0.951056516295154,
1.,0.951056516295154,1.,0.951056516295154,1.,0.951056516295154,1.,0.951056516295154,
1.,0.951056516295154,1.,0.951056516295154,1.,0.951056516295154,1.,0.951056516295154,
1.,0.951056516295154,1.,0.951056516295154,1.,0.951056516295154,1.,0.951056516295154,
1.,0.951056516295154,1.,0.951056516295154,1.,0.951056516295154,1.,0.951056516295154,
1.,0.951056516295154,1.,0.951056516295154,1.,0.951056516295154,1.,0.951056516295154,
1.,0.951056516295154,1.,0.951056516295154,1.,0.951056516295154,1.,0.951056516295154,
1.,0.951056516295154,1.,0.951056516295154,1.,0.951056516295154,1.,0.951056516295154,
1.,0.951056516295154,1.,0.951056516295154,1.,0.951056516295154,1.,0.951056516295154,
1.,0.951056516295154,1.,0.951056516295154,1.,0.951056516295154,1.,0.951056516295154,
1.,0.951056516295154,1.,0.951056516295154,1.,0.951056516295154,1.,0.951056516295154,
1.,0.951056516295154,1.,0.951056516295154,1.,0.951056516295154,1.,0.951056516295154,
1.,0.951056516295154,1.,0.951056516295154,1.,0.951056516295154,1.,0.951056516295154,
1.,0.951056516295154,1.,0.951056516295154,1.,0.951056516295154,1.,0.951056516295154,
1.,0.951056516295154,1.,0.951056516295154,1.,0.951056516295154,1.,0.951056516295154,
1.,0.951056516295154,1.,0.951056516295154,1.,0.951056516295154,1.,0.951056516295154,
1.,0.951056516295154,1.,0.951056516295154,1.,0.951056516295154,1.,0.951056516295154,
1.,0.951056516295154,1.,0.951056516295154,1.,0.951056516295154,1.,0.951056516295154,
1.,0.951056516295154,1.,0.951056516295154,1.,0.951056516295154,1.,0.951056516295154,
1.,0.951056516295154,1.,0.951056516295154,1.,0.951056516295154,1.,0.951056516295154,
1.,0.951056516295154,1.,0.951056516295154,1.,0.951056516295154,1.,0.951056516295154,
1.,0.951056516295154,1.,0.951056516295154,1.,0.951056516295154,1.,0.951056516295154,
1.,0.951056516295154,1.,0.951056516295154,1.,0.951056516295154,1.,0.951056516295154,
1.,0.951056516295154,1.,0.951056516295154,1.,0.951056516295154,1.,0.951056516295154,
1.,0.951056516295154,1.,0.951056516295154,1.,0.951056516295154,1.,0.951056516295154,
1.,0.951056516295154,1.,0.951056516295154,1.,0.951056516295154,1.,0.951056516295154,
1.,0.951056516295154,1.,0.951056516295154,1.,0.951056516295154,1.,0.951056516295154,
1.,0.951056516295154,1.,0.951056516295154,1.,0.951056516295154,1.,0.951056516295154,
1.,0.951056516295154,1.,0.951056516295154,1.,0.951056516295154,1.,0.951056516295154,
1.,0.951056516295154,1.,0.951056516295154,1.,0.951056516295154,1.,0.951056516295154,
1.,0.951056516295154,1.,0.951056516295154,1.,0.951056516295154,1.,0.951056516295154,
1.,0.951056516295154,1.,0.951056516295154,1.,0.951056516295154,1.,0.951056516295154,
1.,0.951056516295154,1.,0.951056516295154,1.,0.951056516295154,1.,0.951056516295154,
1.,0.951056516295154,1.,0.951056516295154,1.,0.951056516295154,1.,0.951056516295154,
1.,0.951056516295154,1.,0.951056516295154,1.,0.951056516295154,1.,0.951056516295154,
1.,0.951056516295154,1.,0.951056516295154,1.,0.951056516295154,1.,0.951056516295154,
1.,0.951056516295154,1.,0.951056516295154,1.,0.951056516295154,1.,0.951056516295154,
1.,0.951056516295154,1.,0.951056516295154,1.,0.951056516295154,1.,0.951056516295154,
1.,0.951056516295154,1.,0.951056516295154,1.,0.951056516295154,1.,0.951056516295154,
1.,0.951056516295154,1.,0.951056516295154,1.,0.951056516295154,1.,0.951056516295154,
1.,0.951056516295154,1.,0.951056516295154,1.,0.951056516295154,1.,0.951056516295154,
1.,0.951056516295154,1.,0.951056516295154,1.,0.951056516295154,1.,0.951056516295154,
1.,0.951056516295154,1.,0.951056516295154,1.,0.951056516295154,1.,0.951056516295154,
1.,0.951056516295154,1.,0.951056516295154,1.,0.951056516295154,1.)))
REPRESENTATION_ITEM('')
SURFACE()
);
#3194=(
BOUNDED_SURFACE()
B_SPLINE_SURFACE(1,2,((#281515,#281516,#281517,#281518,#281519,#281520,
#281521,#281522,#281523,#281524,#281525,#281526,#281527,#281528,#281529,
#281530,#281531,#281532,#281533,#281534,#281535,#281536,#281537,#281538,
#281539,#281540,#281541,#281542,#281543,#281544,#281545,#281546,#281547,
#281548,#281549,#281550,#281551,#281552,#281553,#281554,#281555,#281556,
#281557,#281558,#281559,#281560,#281561,#281562,#281563,#281564,#281565,
#281566,#281567,#281568,#281569,#281570,#281571,#281572,#281573,#281574,
#281575,#281576,#281577,#281578,#281579,#281580,#281581,#281582,#281583,
#281584,#281585,#281586,#281587,#281588,#281589,#281590,#281591,#281592,
#281593,#281594,#281595,#281596,#281597,#281598,#281599,#281600,#281601,
#281602,#281603,#281604,#281605,#281606,#281607,#281608,#281609,#281610,
#281611,#281612,#281613,#281614,#281615,#281616,#281617,#281618,#281619,
#281620,#281621,#281622,#281623,#281624,#281625,#281626,#281627,#281628,
#281629,#281630,#281631,#281632,#281633,#281634,#281635,#281636,#281637,
#281638,#281639,#281640,#281641,#281642,#281643,#281644,#281645,#281646,
#281647,#281648,#281649,#281650,#281651,#281652,#281653,#281654,#281655,
#281656,#281657,#281658,#281659,#281660,#281661,#281662,#281663,#281664,
#281665,#281666,#281667,#281668,#281669,#281670,#281671,#281672,#281673,
#281674,#281675,#281676,#281677,#281678,#281679,#281680,#281681,#281682,
#281683,#281684,#281685,#281686,#281687,#281688,#281689,#281690,#281691,
#281692,#281693,#281694,#281695,#281696,#281697,#281698,#281699,#281700,
#281701,#281702,#281703,#281704,#281705,#281706,#281707,#281708,#281709,
#281710,#281711,#281712,#281713,#281714,#281715,#281716,#281717,#281718,
#281719,#281720,#281721,#281722,#281723,#281724,#281725,#281726,#281727,
#281728,#281729,#281730,#281731,#281732,#281733,#281734,#281735,#281736,
#281737,#281738,#281739,#281740,#281741,#281742,#281743,#281744,#281745,
#281746,#281747,#281748,#281749,#281750,#281751,#281752,#281753,#281754,
#281755,#281756,#281757,#281758,#281759,#281760,#281761,#281762,#281763,
#281764,#281765,#281766,#281767,#281768,#281769,#281770,#281771,#281772,
#281773,#281774,#281775,#281776,#281777,#281778,#281779,#281780,#281781,
#281782,#281783,#281784,#281785,#281786,#281787,#281788,#281789,#281790,
#281791,#281792,#281793,#281794,#281795,#281796,#281797,#281798,#281799,
#281800,#281801,#281802,#281803,#281804,#281805,#281806,#281807,#281808,
#281809,#281810,#281811,#281812,#281813,#281814,#281815,#281816,#281817,
#281818,#281819,#281820,#281821,#281822,#281823,#281824,#281825,#281826,
#281827,#281828,#281829,#281830,#281831,#281832,#281833,#281834,#281835,
#281836,#281837,#281838,#281839,#281840,#281841,#281842,#281843,#281844,
#281845,#281846,#281847,#281848,#281849,#281850,#281851,#281852,#281853,
#281854,#281855,#281856,#281857,#281858,#281859,#281860,#281861,#281862,
#281863,#281864,#281865,#281866,#281867,#281868,#281869,#281870,#281871,
#281872,#281873,#281874,#281875,#281876,#281877,#281878,#281879,#281880,
#281881,#281882,#281883,#281884,#281885,#281886,#281887,#281888,#281889,
#281890,#281891,#281892,#281893,#281894,#281895,#281896,#281897,#281898,
#281899,#281900,#281901,#281902,#281903,#281904,#281905,#281906,#281907,
#281908,#281909,#281910,#281911,#281912,#281913,#281914,#281915,#281916,
#281917,#281918,#281919,#281920,#281921,#281922,#281923,#281924,#281925,
#281926,#281927,#281928,#281929,#281930,#281931,#281932,#281933,#281934,
#281935,#281936,#281937,#281938,#281939,#281940,#281941,#281942,#281943,
#281944,#281945,#281946,#281947,#281948,#281949,#281950,#281951,#281952,
#281953,#281954,#281955,#281956,#281957,#281958,#281959,#281960,#281961,
#281962,#281963,#281964,#281965,#281966,#281967,#281968,#281969,#281970,
#281971,#281972,#281973,#281974,#281975,#281976,#281977,#281978,#281979,
#281980,#281981,#281982,#281983,#281984,#281985,#281986,#281987,#281988,
#281989,#281990,#281991,#281992,#281993,#281994,#281995,#281996,#281997,
#281998,#281999,#282000,#282001,#282002,#282003,#282004,#282005,#282006,
#282007,#282008,#282009,#282010,#282011,#282012,#282013,#282014,#282015,
#282016,#282017,#282018,#282019,#282020,#282021,#282022,#282023,#282024,
#282025,#282026,#282027,#282028,#282029,#282030,#282031,#282032,#282033,
#282034,#282035,#282036,#282037,#282038,#282039,#282040,#282041,#282042,
#282043,#282044,#282045,#282046,#282047,#282048,#282049,#282050,#282051,
#282052,#282053,#282054,#282055,#282056,#282057,#282058,#282059,#282060,
#282061,#282062,#282063,#282064,#282065,#282066,#282067,#282068,#282069,
#282070,#282071,#282072,#282073,#282074,#282075,#282076,#282077,#282078,
#282079,#282080,#282081,#282082,#282083,#282084,#282085,#282086,#282087,
#282088,#282089,#282090,#282091,#282092,#282093,#282094,#282095,#282096,
#282097,#282098,#282099,#282100,#282101,#282102,#282103,#282104,#282105,
#282106,#282107,#282108,#282109,#282110,#282111,#282112,#282113,#282114,
#282115,#282116,#282117,#282118,#282119,#282120,#282121,#282122,#282123,
#282124,#282125,#282126,#282127,#282128,#282129,#282130,#282131,#282132,
#282133,#282134,#282135,#282136,#282137,#282138,#282139,#282140,#282141,
#282142,#282143,#282144,#282145,#282146,#282147,#282148,#282149,#282150,
#282151,#282152,#282153,#282154,#282155,#282156,#282157,#282158,#282159,
#282160,#282161,#282162,#282163,#282164,#282165,#282166,#282167,#282168,
#282169,#282170,#282171,#282172,#282173,#282174,#282175,#282176,#282177,
#282178,#282179,#282180,#282181,#282182,#282183,#282184,#282185,#282186,
#282187,#282188,#282189,#282190,#282191,#282192,#282193,#282194,#282195,
#282196,#282197,#282198,#282199,#282200,#282201,#282202,#282203,#282204,
#282205,#282206,#282207,#282208,#282209,#282210,#282211,#282212,#282213,
#282214,#282215,#282216,#282217,#282218,#282219,#282220,#282221,#282222,
#282223,#282224,#282225,#282226,#282227,#282228,#282229,#282230,#282231,
#282232,#282233,#282234,#282235,#282236,#282237,#282238,#282239,#282240,
#282241,#282242,#282243,#282244,#282245,#282246,#282247,#282248,#282249,
#282250,#282251,#282252,#282253,#282254,#282255,#282256,#282257,#282258,
#282259,#282260,#282261,#282262,#282263,#282264,#282265,#282266,#282267,
#282268,#282269,#282270,#282271,#282272,#282273,#282274,#282275,#282276,
#282277,#282278,#282279,#282280,#282281,#282282,#282283,#282284,#282285,
#282286,#282287,#282288,#282289,#282290,#282291,#282292,#282293,#282294,
#282295,#282296,#282297,#282298,#282299,#282300,#282301,#282302,#282303,
#282304,#282305,#282306,#282307,#282308,#282309,#282310,#282311,#282312,
#282313,#282314,#282315,#282316,#282317,#282318,#282319,#282320,#282321,
#282322,#282323,#282324,#282325,#282326,#282327,#282328,#282329,#282330,
#282331,#282332,#282333,#282334,#282335,#282336,#282337,#282338,#282339,
#282340,#282341,#282342,#282343,#282344,#282345,#282346,#282347,#282348,
#282349,#282350,#282351,#282352,#282353,#282354,#282355,#282356,#282357,
#282358,#282359,#282360,#282361,#282362,#282363,#282364,#282365,#282366,
#282367,#282368,#282369,#282370,#282371,#282372,#282373,#282374,#282375,
#282376,#282377,#282378,#282379,#282380,#282381,#282382,#282383,#282384,
#282385,#282386,#282387,#282388,#282389,#282390,#282391,#282392,#282393,
#282394,#282395,#282396,#282397,#282398,#282399,#282400,#282401,#282402,
#282403,#282404,#282405,#282406,#282407,#282408,#282409,#282410,#282411,
#282412,#282413,#282414,#282415,#282416,#282417,#282418,#282419,#282420,
#282421,#282422,#282423,#282424,#282425,#282426,#282427,#282428,#282429,
#282430,#282431,#282432,#282433,#282434,#282435,#282436,#282437,#282438,
#282439,#282440,#282441,#282442,#282443,#282444,#282445,#282446,#282447,
#282448,#282449,#282450,#282451,#282452,#282453,#282454,#282455,#282456,
#282457,#282458,#282459,#282460,#282461,#282462,#282463,#282464,#282465,
#282466,#282467,#282468,#282469,#282470,#282471,#282472,#282473,#282474,
#282475,#282476,#282477,#282478,#282479,#282480,#282481,#282482,#282483,
#282484,#282485,#282486,#282487,#282488,#282489,#282490,#282491,#282492,
#282493,#282494,#282495,#282496,#282497,#282498,#282499,#282500,#282501,
#282502,#282503,#282504,#282505,#282506,#282507,#282508,#282509,#282510,
#282511,#282512,#282513,#282514,#282515,#282516,#282517,#282518,#282519,
#282520,#282521,#282522,#282523,#282524,#282525,#282526,#282527,#282528,
#282529,#282530,#282531,#282532,#282533,#282534,#282535,#282536,#282537,
#282538,#282539,#282540,#282541,#282542,#282543,#282544,#282545,#282546,
#282547,#282548,#282549,#282550,#282551),(#282552,#282553,#282554,#282555,
#282556,#282557,#282558,#282559,#282560,#282561,#282562,#282563,#282564,
#282565,#282566,#282567,#282568,#282569,#282570,#282571,#282572,#282573,
#282574,#282575,#282576,#282577,#282578,#282579,#282580,#282581,#282582,
#282583,#282584,#282585,#282586,#282587,#282588,#282589,#282590,#282591,
#282592,#282593,#282594,#282595,#282596,#282597,#282598,#282599,#282600,
#282601,#282602,#282603,#282604,#282605,#282606,#282607,#282608,#282609,
#282610,#282611,#282612,#282613,#282614,#282615,#282616,#282617,#282618,
#282619,#282620,#282621,#282622,#282623,#282624,#282625,#282626,#282627,
#282628,#282629,#282630,#282631,#282632,#282633,#282634,#282635,#282636,
#282637,#282638,#282639,#282640,#282641,#282642,#282643,#282644,#282645,
#282646,#282647,#282648,#282649,#282650,#282651,#282652,#282653,#282654,
#282655,#282656,#282657,#282658,#282659,#282660,#282661,#282662,#282663,
#282664,#282665,#282666,#282667,#282668,#282669,#282670,#282671,#282672,
#282673,#282674,#282675,#282676,#282677,#282678,#282679,#282680,#282681,
#282682,#282683,#282684,#282685,#282686,#282687,#282688,#282689,#282690,
#282691,#282692,#282693,#282694,#282695,#282696,#282697,#282698,#282699,
#282700,#282701,#282702,#282703,#282704,#282705,#282706,#282707,#282708,
#282709,#282710,#282711,#282712,#282713,#282714,#282715,#282716,#282717,
#282718,#282719,#282720,#282721,#282722,#282723,#282724,#282725,#282726,
#282727,#282728,#282729,#282730,#282731,#282732,#282733,#282734,#282735,
#282736,#282737,#282738,#282739,#282740,#282741,#282742,#282743,#282744,
#282745,#282746,#282747,#282748,#282749,#282750,#282751,#282752,#282753,
#282754,#282755,#282756,#282757,#282758,#282759,#282760,#282761,#282762,
#282763,#282764,#282765,#282766,#282767,#282768,#282769,#282770,#282771,
#282772,#282773,#282774,#282775,#282776,#282777,#282778,#282779,#282780,
#282781,#282782,#282783,#282784,#282785,#282786,#282787,#282788,#282789,
#282790,#282791,#282792,#282793,#282794,#282795,#282796,#282797,#282798,
#282799,#282800,#282801,#282802,#282803,#282804,#282805,#282806,#282807,
#282808,#282809,#282810,#282811,#282812,#282813,#282814,#282815,#282816,
#282817,#282818,#282819,#282820,#282821,#282822,#282823,#282824,#282825,
#282826,#282827,#282828,#282829,#282830,#282831,#282832,#282833,#282834,
#282835,#282836,#282837,#282838,#282839,#282840,#282841,#282842,#282843,
#282844,#282845,#282846,#282847,#282848,#282849,#282850,#282851,#282852,
#282853,#282854,#282855,#282856,#282857,#282858,#282859,#282860,#282861,
#282862,#282863,#282864,#282865,#282866,#282867,#282868,#282869,#282870,
#282871,#282872,#282873,#282874,#282875,#282876,#282877,#282878,#282879,
#282880,#282881,#282882,#282883,#282884,#282885,#282886,#282887,#282888,
#282889,#282890,#282891,#282892,#282893,#282894,#282895,#282896,#282897,
#282898,#282899,#282900,#282901,#282902,#282903,#282904,#282905,#282906,
#282907,#282908,#282909,#282910,#282911,#282912,#282913,#282914,#282915,
#282916,#282917,#282918,#282919,#282920,#282921,#282922,#282923,#282924,
#282925,#282926,#282927,#282928,#282929,#282930,#282931,#282932,#282933,
#282934,#282935,#282936,#282937,#282938,#282939,#282940,#282941,#282942,
#282943,#282944,#282945,#282946,#282947,#282948,#282949,#282950,#282951,
#282952,#282953,#282954,#282955,#282956,#282957,#282958,#282959,#282960,
#282961,#282962,#282963,#282964,#282965,#282966,#282967,#282968,#282969,
#282970,#282971,#282972,#282973,#282974,#282975,#282976,#282977,#282978,
#282979,#282980,#282981,#282982,#282983,#282984,#282985,#282986,#282987,
#282988,#282989,#282990,#282991,#282992,#282993,#282994,#282995,#282996,
#282997,#282998,#282999,#283000,#283001,#283002,#283003,#283004,#283005,
#283006,#283007,#283008,#283009,#283010,#283011,#283012,#283013,#283014,
#283015,#283016,#283017,#283018,#283019,#283020,#283021,#283022,#283023,
#283024,#283025,#283026,#283027,#283028,#283029,#283030,#283031,#283032,
#283033,#283034,#283035,#283036,#283037,#283038,#283039,#283040,#283041,
#283042,#283043,#283044,#283045,#283046,#283047,#283048,#283049,#283050,
#283051,#283052,#283053,#283054,#283055,#283056,#283057,#283058,#283059,
#283060,#283061,#283062,#283063,#283064,#283065,#283066,#283067,#283068,
#283069,#283070,#283071,#283072,#283073,#283074,#283075,#283076,#283077,
#283078,#283079,#283080,#283081,#283082,#283083,#283084,#283085,#283086,
#283087,#283088,#283089,#283090,#283091,#283092,#283093,#283094,#283095,
#283096,#283097,#283098,#283099,#283100,#283101,#283102,#283103,#283104,
#283105,#283106,#283107,#283108,#283109,#283110,#283111,#283112,#283113,
#283114,#283115,#283116,#283117,#283118,#283119,#283120,#283121,#283122,
#283123,#283124,#283125,#283126,#283127,#283128,#283129,#283130,#283131,
#283132,#283133,#283134,#283135,#283136,#283137,#283138,#283139,#283140,
#283141,#283142,#283143,#283144,#283145,#283146,#283147,#283148,#283149,
#283150,#283151,#283152,#283153,#283154,#283155,#283156,#283157,#283158,
#283159,#283160,#283161,#283162,#283163,#283164,#283165,#283166,#283167,
#283168,#283169,#283170,#283171,#283172,#283173,#283174,#283175,#283176,
#283177,#283178,#283179,#283180,#283181,#283182,#283183,#283184,#283185,
#283186,#283187,#283188,#283189,#283190,#283191,#283192,#283193,#283194,
#283195,#283196,#283197,#283198,#283199,#283200,#283201,#283202,#283203,
#283204,#283205,#283206,#283207,#283208,#283209,#283210,#283211,#283212,
#283213,#283214,#283215,#283216,#283217,#283218,#283219,#283220,#283221,
#283222,#283223,#283224,#283225,#283226,#283227,#283228,#283229,#283230,
#283231,#283232,#283233,#283234,#283235,#283236,#283237,#283238,#283239,
#283240,#283241,#283242,#283243,#283244,#283245,#283246,#283247,#283248,
#283249,#283250,#283251,#283252,#283253,#283254,#283255,#283256,#283257,
#283258,#283259,#283260,#283261,#283262,#283263,#283264,#283265,#283266,
#283267,#283268,#283269,#283270,#283271,#283272,#283273,#283274,#283275,
#283276,#283277,#283278,#283279,#283280,#283281,#283282,#283283,#283284,
#283285,#283286,#283287,#283288,#283289,#283290,#283291,#283292,#283293,
#283294,#283295,#283296,#283297,#283298,#283299,#283300,#283301,#283302,
#283303,#283304,#283305,#283306,#283307,#283308,#283309,#283310,#283311,
#283312,#283313,#283314,#283315,#283316,#283317,#283318,#283319,#283320,
#283321,#283322,#283323,#283324,#283325,#283326,#283327,#283328,#283329,
#283330,#283331,#283332,#283333,#283334,#283335,#283336,#283337,#283338,
#283339,#283340,#283341,#283342,#283343,#283344,#283345,#283346,#283347,
#283348,#283349,#283350,#283351,#283352,#283353,#283354,#283355,#283356,
#283357,#283358,#283359,#283360,#283361,#283362,#283363,#283364,#283365,
#283366,#283367,#283368,#283369,#283370,#283371,#283372,#283373,#283374,
#283375,#283376,#283377,#283378,#283379,#283380,#283381,#283382,#283383,
#283384,#283385,#283386,#283387,#283388,#283389,#283390,#283391,#283392,
#283393,#283394,#283395,#283396,#283397,#283398,#283399,#283400,#283401,
#283402,#283403,#283404,#283405,#283406,#283407,#283408,#283409,#283410,
#283411,#283412,#283413,#283414,#283415,#283416,#283417,#283418,#283419,
#283420,#283421,#283422,#283423,#283424,#283425,#283426,#283427,#283428,
#283429,#283430,#283431,#283432,#283433,#283434,#283435,#283436,#283437,
#283438,#283439,#283440,#283441,#283442,#283443,#283444,#283445,#283446,
#283447,#283448,#283449,#283450,#283451,#283452,#283453,#283454,#283455,
#283456,#283457,#283458,#283459,#283460,#283461,#283462,#283463,#283464,
#283465,#283466,#283467,#283468,#283469,#283470,#283471,#283472,#283473,
#283474,#283475,#283476,#283477,#283478,#283479,#283480,#283481,#283482,
#283483,#283484,#283485,#283486,#283487,#283488,#283489,#283490,#283491,
#283492,#283493,#283494,#283495,#283496,#283497,#283498,#283499,#283500,
#283501,#283502,#283503,#283504,#283505,#283506,#283507,#283508,#283509,
#283510,#283511,#283512,#283513,#283514,#283515,#283516,#283517,#283518,
#283519,#283520,#283521,#283522,#283523,#283524,#283525,#283526,#283527,
#283528,#283529,#283530,#283531,#283532,#283533,#283534,#283535,#283536,
#283537,#283538,#283539,#283540,#283541,#283542,#283543,#283544,#283545,
#283546,#283547,#283548,#283549,#283550,#283551,#283552,#283553,#283554,
#283555,#283556,#283557,#283558,#283559,#283560,#283561,#283562,#283563,
#283564,#283565,#283566,#283567,#283568,#283569,#283570,#283571,#283572,
#283573,#283574,#283575,#283576,#283577,#283578,#283579,#283580,#283581,
#283582,#283583,#283584,#283585,#283586,#283587,#283588)),.UNSPECIFIED.,
 .F.,.F.,.F.)
B_SPLINE_SURFACE_WITH_KNOTS((2,2),(3,2,2,2,2,2,2,2,2,2,2,2,2,2,2,2,2,2,
2,2,2,2,2,2,2,2,2,2,2,2,2,2,2,2,2,2,2,2,2,2,2,2,2,2,2,2,2,2,2,2,2,2,2,2,
2,2,2,2,2,2,2,2,2,2,2,2,2,2,2,2,2,2,2,2,2,2,2,2,2,2,2,2,2,2,2,2,2,2,2,2,
2,2,2,2,2,2,2,2,2,2,2,2,2,2,2,2,2,2,2,2,2,2,2,2,2,2,2,2,2,2,2,2,2,2,2,2,
2,2,2,2,2,2,2,2,2,2,2,2,2,2,2,2,2,2,2,2,2,2,2,2,2,2,2,2,2,2,2,2,2,2,2,2,
2,2,2,2,2,2,2,2,2,2,2,2,2,2,2,2,2,2,2,2,2,2,2,2,2,2,2,2,2,2,2,2,2,2,2,2,
2,2,2,2,2,2,2,2,2,2,2,2,2,2,2,2,2,2,2,2,2,2,2,2,2,2,2,2,2,2,2,2,2,2,2,2,
2,2,2,2,2,2,2,2,2,2,2,2,2,2,2,2,2,2,2,2,2,2,2,2,2,2,2,2,2,2,2,2,2,2,2,2,
2,2,2,2,2,2,2,2,2,2,2,2,2,2,2,2,2,2,2,2,2,2,2,2,2,2,2,2,2,2,2,2,2,2,2,2,
2,2,2,2,2,2,2,2,2,2,2,2,2,2,2,2,2,2,2,2,2,2,2,2,2,2,2,2,2,2,2,2,2,2,2,2,
2,2,2,2,2,2,2,2,2,2,2,2,2,2,2,2,2,2,2,2,2,2,2,2,2,2,2,2,2,2,2,2,2,2,2,2,
2,2,2,2,2,2,2,2,2,2,2,2,2,2,2,2,2,2,2,2,2,2,2,2,2,2,2,2,2,2,2,2,2,2,2,2,
2,2,2,2,2,2,2,2,2,2,2,2,2,2,2,2,2,2,2,2,2,2,2,2,2,2,2,2,2,2,2,2,2,2,2,2,
2,2,2,2,2,2,2,2,2,2,2,2,2,2,2,2,2,2,2,2,2,2,2,2,2,2,2,2,2,2,2,2,2,2,2,2,
2,2,2,2,2,2,2,2,2,2,2,2,2,2,2,2,2,2,2,2,2,2,2,2,2,2,2,2,2,2,2,2,3),(-2.99434144680572E-6,
1.),(0.,0.00192307692307692,0.00384615384615385,0.00576923076923077,0.00769230769230769,
0.00961538461538462,0.0115384615384615,0.0134615384615385,0.0153846153846154,
0.0173076923076923,0.0192307692307692,0.0211538461538462,0.0230769230769231,
0.025,0.0269230769230769,0.0288461538461538,0.0307692307692308,0.0326923076923077,
0.0346153846153846,0.0365384615384615,0.0384615384615385,0.0403846153846154,
0.0423076923076923,0.0442307692307692,0.0461538461538462,0.0480769230769231,
0.05,0.0519230769230769,0.0538461538461538,0.0557692307692308,0.0576923076923077,
0.0596153846153846,0.0615384615384615,0.0634615384615385,0.0653846153846154,
0.0673076923076923,0.0692307692307692,0.0711538461538462,0.0730769230769231,
0.075,0.0769230769230769,0.0788461538461538,0.0807692307692308,0.0826923076923077,
0.0846153846153846,0.0865384615384615,0.0884615384615385,0.0903846153846154,
0.0923076923076923,0.0942307692307692,0.0961538461538462,0.0980769230769231,
0.1,0.101923076923077,0.103846153846154,0.105769230769231,0.107692307692308,
0.109615384615385,0.111538461538462,0.113461538461538,0.115384615384615,
0.117307692307692,0.119230769230769,0.121153846153846,0.123076923076923,
0.125,0.126923076923077,0.128846153846154,0.130769230769231,0.132692307692308,
0.134615384615385,0.136538461538462,0.138461538461538,0.140384615384615,
0.142307692307692,0.144230769230769,0.146153846153846,0.148076923076923,
0.15,0.151923076923077,0.153846153846154,0.155769230769231,0.157692307692308,
0.159615384615385,0.161538461538462,0.163461538461538,0.165384615384615,
0.167307692307692,0.169230769230769,0.171153846153846,0.173076923076923,
0.175,0.176923076923077,0.178846153846154,0.180769230769231,0.182692307692308,
0.184615384615385,0.186538461538462,0.188461538461538,0.190384615384615,
0.192307692307692,0.194230769230769,0.196153846153846,0.198076923076923,
0.2,0.201923076923077,0.203846153846154,0.205769230769231,0.207692307692308,
0.209615384615385,0.211538461538462,0.213461538461538,0.215384615384615,
0.217307692307692,0.219230769230769,0.221153846153846,0.223076923076923,
0.225,0.226923076923077,0.228846153846154,0.230769230769231,0.232692307692308,
0.234615384615385,0.236538461538462,0.238461538461538,0.240384615384615,
0.242307692307692,0.244230769230769,0.246153846153846,0.248076923076923,
0.25,0.251923076923077,0.253846153846154,0.255769230769231,0.257692307692308,
0.259615384615385,0.261538461538462,0.263461538461538,0.265384615384615,
0.267307692307692,0.269230769230769,0.271153846153846,0.273076923076923,
0.275,0.276923076923077,0.278846153846154,0.280769230769231,0.282692307692308,
0.284615384615385,0.286538461538462,0.288461538461538,0.290384615384615,
0.292307692307692,0.294230769230769,0.296153846153846,0.298076923076923,
0.3,0.301923076923077,0.303846153846154,0.305769230769231,0.307692307692308,
0.309615384615385,0.311538461538462,0.313461538461538,0.315384615384615,
0.317307692307692,0.319230769230769,0.321153846153846,0.323076923076923,
0.325,0.326923076923077,0.328846153846154,0.330769230769231,0.332692307692308,
0.334615384615385,0.336538461538462,0.338461538461538,0.340384615384615,
0.342307692307692,0.344230769230769,0.346153846153846,0.348076923076923,
0.35,0.351923076923077,0.353846153846154,0.355769230769231,0.357692307692308,
0.359615384615385,0.361538461538462,0.363461538461538,0.365384615384615,
0.367307692307692,0.369230769230769,0.371153846153846,0.373076923076923,
0.375,0.376923076923077,0.378846153846154,0.380769230769231,0.382692307692308,
0.384615384615385,0.386538461538462,0.388461538461538,0.390384615384615,
0.392307692307692,0.394230769230769,0.396153846153846,0.398076923076923,
0.4,0.401923076923077,0.403846153846154,0.405769230769231,0.407692307692308,
0.409615384615385,0.411538461538462,0.413461538461538,0.415384615384615,
0.417307692307692,0.419230769230769,0.421153846153846,0.423076923076923,
0.425,0.426923076923077,0.428846153846154,0.430769230769231,0.432692307692308,
0.434615384615385,0.436538461538462,0.438461538461538,0.440384615384615,
0.442307692307692,0.444230769230769,0.446153846153846,0.448076923076923,
0.45,0.451923076923077,0.453846153846154,0.455769230769231,0.457692307692308,
0.459615384615385,0.461538461538462,0.463461538461538,0.465384615384615,
0.467307692307692,0.469230769230769,0.471153846153846,0.473076923076923,
0.475,0.476923076923077,0.478846153846154,0.480769230769231,0.482692307692308,
0.484615384615385,0.486538461538462,0.488461538461538,0.490384615384615,
0.492307692307692,0.494230769230769,0.496153846153846,0.498076923076923,
0.5,0.501923076923077,0.503846153846154,0.505769230769231,0.507692307692308,
0.509615384615385,0.511538461538461,0.513461538461538,0.515384615384615,
0.517307692307692,0.519230769230769,0.521153846153846,0.523076923076923,
0.525,0.526923076923077,0.528846153846154,0.530769230769231,0.532692307692308,
0.534615384615385,0.536538461538462,0.538461538461538,0.540384615384615,
0.542307692307692,0.544230769230769,0.546153846153846,0.548076923076923,
0.55,0.551923076923077,0.553846153846154,0.555769230769231,0.557692307692308,
0.559615384615385,0.561538461538462,0.563461538461538,0.565384615384615,
0.567307692307692,0.569230769230769,0.571153846153846,0.573076923076923,
0.575,0.576923076923077,0.578846153846154,0.580769230769231,0.582692307692308,
0.584615384615385,0.586538461538462,0.588461538461538,0.590384615384615,
0.592307692307692,0.594230769230769,0.596153846153846,0.598076923076923,
0.6,0.601923076923077,0.603846153846154,0.605769230769231,0.607692307692308,
0.609615384615385,0.611538461538462,0.613461538461539,0.615384615384615,
0.617307692307692,0.619230769230769,0.621153846153846,0.623076923076923,
0.625,0.626923076923077,0.628846153846154,0.630769230769231,0.632692307692308,
0.634615384615385,0.636538461538461,0.638461538461538,0.640384615384615,
0.642307692307692,0.644230769230769,0.646153846153846,0.648076923076923,
0.65,0.651923076923077,0.653846153846154,0.655769230769231,0.657692307692308,
0.659615384615385,0.661538461538462,0.663461538461538,0.665384615384615,
0.667307692307692,0.669230769230769,0.671153846153846,0.673076923076923,
0.675,0.676923076923077,0.678846153846154,0.680769230769231,0.682692307692308,
0.684615384615385,0.686538461538462,0.688461538461538,0.690384615384615,
0.692307692307692,0.694230769230769,0.696153846153846,0.698076923076923,
0.7,0.701923076923077,0.703846153846154,0.705769230769231,0.707692307692308,
0.709615384615385,0.711538461538462,0.713461538461538,0.715384615384615,
0.717307692307692,0.719230769230769,0.721153846153846,0.723076923076923,
0.725,0.726923076923077,0.728846153846154,0.730769230769231,0.732692307692308,
0.734615384615385,0.736538461538462,0.738461538461539,0.740384615384615,
0.742307692307692,0.744230769230769,0.746153846153846,0.748076923076923,
0.75,0.751923076923077,0.753846153846154,0.755769230769231,0.757692307692308,
0.759615384615385,0.761538461538461,0.763461538461538,0.765384615384615,
0.767307692307692,0.769230769230769,0.771153846153846,0.773076923076923,
0.775,0.776923076923077,0.778846153846154,0.780769230769231,0.782692307692308,
0.784615384615385,0.786538461538462,0.788461538461538,0.790384615384615,
0.792307692307692,0.794230769230769,0.796153846153846,0.798076923076923,
0.8,0.801923076923077,0.803846153846154,0.805769230769231,0.807692307692308,
0.809615384615385,0.811538461538462,0.813461538461538,0.815384615384615,
0.817307692307692,0.819230769230769,0.821153846153846,0.823076923076923,
0.825,0.826923076923077,0.828846153846154,0.830769230769231,0.832692307692308,
0.834615384615385,0.836538461538462,0.838461538461538,0.840384615384615,
0.842307692307692,0.844230769230769,0.846153846153846,0.848076923076923,
0.85,0.851923076923077,0.853846153846154,0.855769230769231,0.857692307692308,
0.859615384615385,0.861538461538462,0.863461538461539,0.865384615384615,
0.867307692307692,0.869230769230769,0.871153846153846,0.873076923076923,
0.875,0.876923076923077,0.878846153846154,0.880769230769231,0.882692307692308,
0.884615384615385,0.886538461538461,0.888461538461538,0.890384615384615,
0.892307692307692,0.894230769230769,0.896153846153846,0.898076923076923,
0.9,0.901923076923077,0.903846153846154,0.905769230769231,0.907692307692308,
0.909615384615385,0.911538461538462,0.913461538461538,0.915384615384615,
0.917307692307692,0.919230769230769,0.921153846153846,0.923076923076923,
0.925,0.926923076923077,0.928846153846154,0.930769230769231,0.932692307692308,
0.934615384615385,0.936538461538462,0.938461538461538,0.940384615384615,
0.942307692307692,0.944230769230769,0.946153846153846,0.948076923076923,
0.95,0.951923076923077,0.953846153846154,0.955769230769231,0.957692307692308,
0.959615384615385,0.961538461538462,0.963461538461538,0.965384615384615,
0.967307692307692,0.969230769230769,0.971153846153846,0.973076923076923,
0.975,0.976923076923077,0.978846153846154,0.980769230769231,0.982692307692308,
0.984615384615385,0.986538461538462,0.988461538461539,0.990384615384615,
0.992307692307692,0.994230769230769,0.996153846153846),.UNSPECIFIED.)
GEOMETRIC_REPRESENTATION_ITEM()
RATIONAL_B_SPLINE_SURFACE(((1.,0.951056516295154,1.,0.951056516295154,1.,
0.951056516295154,1.,0.951056516295154,1.,0.951056516295154,1.,0.951056516295154,
1.,0.951056516295154,1.,0.951056516295154,1.,0.951056516295154,1.,0.951056516295154,
1.,0.951056516295154,1.,0.951056516295154,1.,0.951056516295154,1.,0.951056516295154,
1.,0.951056516295154,1.,0.951056516295154,1.,0.951056516295154,1.,0.951056516295154,
1.,0.951056516295154,1.,0.951056516295154,1.,0.951056516295154,1.,0.951056516295154,
1.,0.951056516295154,1.,0.951056516295154,1.,0.951056516295154,1.,0.951056516295154,
1.,0.951056516295154,1.,0.951056516295154,1.,0.951056516295154,1.,0.951056516295154,
1.,0.951056516295154,1.,0.951056516295154,1.,0.951056516295154,1.,0.951056516295154,
1.,0.951056516295154,1.,0.951056516295154,1.,0.951056516295154,1.,0.951056516295154,
1.,0.951056516295154,1.,0.951056516295154,1.,0.951056516295154,1.,0.951056516295154,
1.,0.951056516295154,1.,0.951056516295154,1.,0.951056516295154,1.,0.951056516295154,
1.,0.951056516295154,1.,0.951056516295154,1.,0.951056516295154,1.,0.951056516295154,
1.,0.951056516295154,1.,0.951056516295154,1.,0.951056516295154,1.,0.951056516295154,
1.,0.951056516295154,1.,0.951056516295154,1.,0.951056516295154,1.,0.951056516295154,
1.,0.951056516295154,1.,0.951056516295154,1.,0.951056516295154,1.,0.951056516295154,
1.,0.951056516295154,1.,0.951056516295154,1.,0.951056516295154,1.,0.951056516295154,
1.,0.951056516295154,1.,0.951056516295154,1.,0.951056516295154,1.,0.951056516295154,
1.,0.951056516295154,1.,0.951056516295154,1.,0.951056516295154,1.,0.951056516295154,
1.,0.951056516295154,1.,0.951056516295154,1.,0.951056516295154,1.,0.951056516295154,
1.,0.951056516295154,1.,0.951056516295154,1.,0.951056516295154,1.,0.951056516295154,
1.,0.951056516295154,1.,0.951056516295154,1.,0.951056516295154,1.,0.951056516295154,
1.,0.951056516295154,1.,0.951056516295154,1.,0.951056516295154,1.,0.951056516295154,
1.,0.951056516295154,1.,0.951056516295154,1.,0.951056516295154,1.,0.951056516295154,
1.,0.951056516295154,1.,0.951056516295154,1.,0.951056516295154,1.,0.951056516295154,
1.,0.951056516295154,1.,0.951056516295154,1.,0.951056516295154,1.,0.951056516295154,
1.,0.951056516295154,1.,0.951056516295154,1.,0.951056516295154,1.,0.951056516295154,
1.,0.951056516295154,1.,0.951056516295154,1.,0.951056516295154,1.,0.951056516295154,
1.,0.951056516295154,1.,0.951056516295154,1.,0.951056516295154,1.,0.951056516295154,
1.,0.951056516295154,1.,0.951056516295154,1.,0.951056516295154,1.,0.951056516295154,
1.,0.951056516295154,1.,0.951056516295154,1.,0.951056516295154,1.,0.951056516295154,
1.,0.951056516295154,1.,0.951056516295154,1.,0.951056516295154,1.,0.951056516295154,
1.,0.951056516295154,1.,0.951056516295154,1.,0.951056516295154,1.,0.951056516295154,
1.,0.951056516295154,1.,0.951056516295154,1.,0.951056516295154,1.,0.951056516295154,
1.,0.951056516295154,1.,0.951056516295154,1.,0.951056516295154,1.,0.951056516295154,
1.,0.951056516295154,1.,0.951056516295154,1.,0.951056516295154,1.,0.951056516295154,
1.,0.951056516295154,1.,0.951056516295154,1.,0.951056516295154,1.,0.951056516295154,
1.,0.951056516295154,1.,0.951056516295154,1.,0.951056516295154,1.,0.951056516295154,
1.,0.951056516295154,1.,0.951056516295154,1.,0.951056516295154,1.,0.951056516295154,
1.,0.951056516295154,1.,0.951056516295154,1.,0.951056516295154,1.,0.951056516295154,
1.,0.951056516295154,1.,0.951056516295154,1.,0.951056516295154,1.,0.951056516295154,
1.,0.951056516295154,1.,0.951056516295154,1.,0.951056516295154,1.,0.951056516295154,
1.,0.951056516295154,1.,0.951056516295154,1.,0.951056516295154,1.,0.951056516295154,
1.,0.951056516295154,1.,0.951056516295154,1.,0.951056516295154,1.,0.951056516295154,
1.,0.951056516295154,1.,0.951056516295154,1.,0.951056516295154,1.,0.951056516295154,
1.,0.951056516295154,1.,0.951056516295154,1.,0.951056516295154,1.,0.951056516295154,
1.,0.951056516295154,1.,0.951056516295154,1.,0.951056516295154,1.,0.951056516295154,
1.,0.951056516295154,1.,0.951056516295154,1.,0.951056516295154,1.,0.951056516295154,
1.,0.951056516295154,1.,0.951056516295154,1.,0.951056516295154,1.,0.951056516295154,
1.,0.951056516295154,1.,0.951056516295154,1.,0.951056516295154,1.,0.951056516295154,
1.,0.951056516295154,1.,0.951056516295154,1.,0.951056516295154,1.,0.951056516295154,
1.,0.951056516295154,1.,0.951056516295154,1.,0.951056516295154,1.,0.951056516295154,
1.,0.951056516295154,1.,0.951056516295154,1.,0.951056516295154,1.,0.951056516295154,
1.,0.951056516295154,1.,0.951056516295154,1.,0.951056516295154,1.,0.951056516295154,
1.,0.951056516295154,1.,0.951056516295154,1.,0.951056516295154,1.,0.951056516295154,
1.,0.951056516295154,1.,0.951056516295154,1.,0.951056516295154,1.,0.951056516295154,
1.,0.951056516295154,1.,0.951056516295154,1.,0.951056516295154,1.,0.951056516295154,
1.,0.951056516295154,1.,0.951056516295154,1.,0.951056516295154,1.,0.951056516295154,
1.,0.951056516295154,1.,0.951056516295154,1.,0.951056516295154,1.,0.951056516295154,
1.,0.951056516295154,1.,0.951056516295154,1.,0.951056516295154,1.,0.951056516295154,
1.,0.951056516295154,1.,0.951056516295154,1.,0.951056516295154,1.,0.951056516295154,
1.,0.951056516295154,1.,0.951056516295154,1.,0.951056516295154,1.,0.951056516295154,
1.,0.951056516295154,1.,0.951056516295154,1.,0.951056516295154,1.,0.951056516295154,
1.,0.951056516295154,1.,0.951056516295154,1.,0.951056516295154,1.,0.951056516295154,
1.,0.951056516295154,1.,0.951056516295154,1.,0.951056516295154,1.,0.951056516295154,
1.,0.951056516295154,1.,0.951056516295154,1.,0.951056516295154,1.,0.951056516295154,
1.,0.951056516295154,1.,0.951056516295154,1.,0.951056516295154,1.,0.951056516295154,
1.,0.951056516295154,1.,0.951056516295154,1.,0.951056516295154,1.,0.951056516295154,
1.,0.951056516295154,1.,0.951056516295154,1.,0.951056516295154,1.,0.951056516295154,
1.,0.951056516295154,1.,0.951056516295154,1.,0.951056516295154,1.,0.951056516295154,
1.,0.951056516295154,1.,0.951056516295154,1.,0.951056516295154,1.,0.951056516295154,
1.,0.951056516295154,1.,0.951056516295154,1.,0.951056516295154,1.,0.951056516295154,
1.,0.951056516295154,1.,0.951056516295154,1.,0.951056516295154,1.,0.951056516295154,
1.,0.951056516295154,1.,0.951056516295154,1.,0.951056516295154,1.,0.951056516295154,
1.,0.951056516295154,1.,0.951056516295154,1.,0.951056516295154,1.,0.951056516295154,
1.,0.951056516295154,1.,0.951056516295154,1.,0.951056516295154,1.,0.951056516295154,
1.,0.951056516295154,1.,0.951056516295154,1.,0.951056516295154,1.,0.951056516295154,
1.,0.951056516295154,1.,0.951056516295154,1.,0.951056516295154,1.,0.951056516295154,
1.,0.951056516295154,1.,0.951056516295154,1.,0.951056516295154,1.,0.951056516295154,
1.,0.951056516295154,1.,0.951056516295154,1.,0.951056516295154,1.,0.951056516295154,
1.,0.951056516295154,1.,0.951056516295154,1.,0.951056516295154,1.,0.951056516295154,
1.,0.951056516295154,1.,0.951056516295154,1.,0.951056516295154,1.,0.951056516295154,
1.,0.951056516295154,1.,0.951056516295154,1.,0.951056516295154,1.,0.951056516295154,
1.,0.951056516295154,1.,0.951056516295154,1.,0.951056516295154,1.,0.951056516295154,
1.,0.951056516295154,1.,0.951056516295154,1.,0.951056516295154,1.,0.951056516295154,
1.,0.951056516295154,1.,0.951056516295154,1.,0.951056516295154,1.,0.951056516295154,
1.,0.951056516295154,1.,0.951056516295154,1.,0.951056516295154,1.,0.951056516295154,
1.,0.951056516295154,1.,0.951056516295154,1.,0.951056516295154,1.,0.951056516295154,
1.,0.951056516295154,1.,0.951056516295154,1.,0.951056516295154,1.,0.951056516295154,
1.,0.951056516295154,1.,0.951056516295154,1.,0.951056516295154,1.,0.951056516295154,
1.,0.951056516295154,1.,0.951056516295154,1.,0.951056516295154,1.,0.951056516295154,
1.,0.951056516295154,1.,0.951056516295154,1.,0.951056516295154,1.,0.951056516295154,
1.,0.951056516295154,1.,0.951056516295154,1.,0.951056516295154,1.,0.951056516295154,
1.,0.951056516295154,1.,0.951056516295154,1.,0.951056516295154,1.,0.951056516295154,
1.,0.951056516295154,1.,0.951056516295154,1.,0.951056516295154,1.,0.951056516295154,
1.,0.951056516295154,1.,0.951056516295154,1.,0.951056516295154,1.,0.951056516295154,
1.,0.951056516295154,1.,0.951056516295154,1.,0.951056516295154,1.,0.951056516295154,
1.,0.951056516295154,1.,0.951056516295154,1.,0.951056516295154,1.,0.951056516295154,
1.,0.951056516295154,1.,0.951056516295154,1.,0.951056516295154,1.,0.951056516295154,
1.,0.951056516295154,1.,0.951056516295154,1.,0.951056516295154,1.,0.951056516295154,
1.,0.951056516295154,1.,0.951056516295154,1.,0.951056516295154,1.,0.951056516295154,
1.,0.951056516295154,1.,0.951056516295154,1.,0.951056516295154,1.,0.951056516295154,
1.,0.951056516295154,1.,0.951056516295154,1.,0.951056516295154,1.,0.951056516295154,
1.,0.951056516295154,1.,0.951056516295154,1.,0.951056516295154,1.,0.951056516295154,
1.,0.951056516295154,1.,0.951056516295154,1.,0.951056516295154,1.,0.951056516295154,
1.,0.951056516295154,1.,0.951056516295154,1.,0.951056516295154,1.,0.951056516295154,
1.,0.951056516295154,1.,0.951056516295154,1.,0.951056516295154,1.,0.951056516295154,
1.,0.951056516295154,1.,0.951056516295154,1.,0.951056516295154,1.,0.951056516295154,
1.,0.951056516295154,1.,0.951056516295154,1.,0.951056516295154,1.,0.951056516295154,
1.,0.951056516295154,1.,0.951056516295154,1.,0.951056516295154,1.,0.951056516295154,
1.,0.951056516295154,1.,0.951056516295154,1.,0.951056516295154,1.,0.951056516295154,
1.,0.951056516295154,1.,0.951056516295154,1.,0.951056516295154,1.,0.951056516295154,
1.,0.951056516295154,1.,0.951056516295154,1.,0.951056516295154,1.,0.951056516295154,
1.,0.951056516295154,1.,0.951056516295154,1.,0.951056516295154,1.,0.951056516295154,
1.,0.951056516295154,1.,0.951056516295154,1.,0.951056516295154,1.,0.951056516295154,
1.,0.951056516295154,1.,0.951056516295154,1.,0.951056516295154,1.,0.951056516295154,
1.,0.951056516295154,1.,0.951056516295154,1.,0.951056516295154,1.,0.951056516295154,
1.,0.951056516295154,1.,0.951056516295154,1.,0.951056516295154,1.,0.951056516295154,
1.,0.951056516295154,1.,0.951056516295154,1.,0.951056516295154,1.,0.951056516295154,
1.,0.951056516295154,1.,0.951056516295154,1.,0.951056516295154,1.,0.951056516295154,
1.,0.951056516295154,1.,0.951056516295154,1.,0.951056516295154,1.,0.951056516295154,
1.,0.951056516295154,1.,0.951056516295154,1.,0.951056516295154,1.,0.951056516295154,
1.,0.951056516295154,1.,0.951056516295154,1.,0.951056516295154,1.,0.951056516295154,
1.,0.951056516295154,1.,0.951056516295154,1.,0.951056516295154,1.,0.951056516295154,
1.,0.951056516295154,1.,0.951056516295154,1.,0.951056516295154,1.,0.951056516295154,
1.,0.951056516295154,1.,0.951056516295154,1.,0.951056516295154,1.,0.951056516295154,
1.,0.951056516295154,1.,0.951056516295154,1.,0.951056516295154,1.,0.951056516295154,
1.,0.951056516295154,1.,0.951056516295154,1.,0.951056516295154,1.,0.951056516295154,
1.,0.951056516295154,1.,0.951056516295154,1.,0.951056516295154,1.,0.951056516295154,
1.,0.951056516295154,1.,0.951056516295154,1.,0.951056516295154,1.,0.951056516295154,
1.),(1.,0.951056516295154,1.,0.951056516295154,1.,0.951056516295154,1.,
0.951056516295154,1.,0.951056516295154,1.,0.951056516295154,1.,0.951056516295154,
1.,0.951056516295154,1.,0.951056516295154,1.,0.951056516295154,1.,0.951056516295154,
1.,0.951056516295154,1.,0.951056516295154,1.,0.951056516295154,1.,0.951056516295154,
1.,0.951056516295154,1.,0.951056516295154,1.,0.951056516295154,1.,0.951056516295154,
1.,0.951056516295154,1.,0.951056516295154,1.,0.951056516295154,1.,0.951056516295154,
1.,0.951056516295154,1.,0.951056516295154,1.,0.951056516295154,1.,0.951056516295154,
1.,0.951056516295154,1.,0.951056516295154,1.,0.951056516295154,1.,0.951056516295154,
1.,0.951056516295154,1.,0.951056516295154,1.,0.951056516295154,1.,0.951056516295154,
1.,0.951056516295154,1.,0.951056516295154,1.,0.951056516295154,1.,0.951056516295154,
1.,0.951056516295154,1.,0.951056516295154,1.,0.951056516295154,1.,0.951056516295154,
1.,0.951056516295154,1.,0.951056516295154,1.,0.951056516295154,1.,0.951056516295154,
1.,0.951056516295154,1.,0.951056516295154,1.,0.951056516295154,1.,0.951056516295154,
1.,0.951056516295154,1.,0.951056516295154,1.,0.951056516295154,1.,0.951056516295154,
1.,0.951056516295154,1.,0.951056516295154,1.,0.951056516295154,1.,0.951056516295154,
1.,0.951056516295154,1.,0.951056516295154,1.,0.951056516295154,1.,0.951056516295154,
1.,0.951056516295154,1.,0.951056516295154,1.,0.951056516295154,1.,0.951056516295154,
1.,0.951056516295154,1.,0.951056516295154,1.,0.951056516295154,1.,0.951056516295154,
1.,0.951056516295154,1.,0.951056516295154,1.,0.951056516295154,1.,0.951056516295154,
1.,0.951056516295154,1.,0.951056516295154,1.,0.951056516295154,1.,0.951056516295154,
1.,0.951056516295154,1.,0.951056516295154,1.,0.951056516295154,1.,0.951056516295154,
1.,0.951056516295154,1.,0.951056516295154,1.,0.951056516295154,1.,0.951056516295154,
1.,0.951056516295154,1.,0.951056516295154,1.,0.951056516295154,1.,0.951056516295154,
1.,0.951056516295154,1.,0.951056516295154,1.,0.951056516295154,1.,0.951056516295154,
1.,0.951056516295154,1.,0.951056516295154,1.,0.951056516295154,1.,0.951056516295154,
1.,0.951056516295154,1.,0.951056516295154,1.,0.951056516295154,1.,0.951056516295154,
1.,0.951056516295154,1.,0.951056516295154,1.,0.951056516295154,1.,0.951056516295154,
1.,0.951056516295154,1.,0.951056516295154,1.,0.951056516295154,1.,0.951056516295154,
1.,0.951056516295154,1.,0.951056516295154,1.,0.951056516295154,1.,0.951056516295154,
1.,0.951056516295154,1.,0.951056516295154,1.,0.951056516295154,1.,0.951056516295154,
1.,0.951056516295154,1.,0.951056516295154,1.,0.951056516295154,1.,0.951056516295154,
1.,0.951056516295154,1.,0.951056516295154,1.,0.951056516295154,1.,0.951056516295154,
1.,0.951056516295154,1.,0.951056516295154,1.,0.951056516295154,1.,0.951056516295154,
1.,0.951056516295154,1.,0.951056516295154,1.,0.951056516295154,1.,0.951056516295154,
1.,0.951056516295154,1.,0.951056516295154,1.,0.951056516295154,1.,0.951056516295154,
1.,0.951056516295154,1.,0.951056516295154,1.,0.951056516295154,1.,0.951056516295154,
1.,0.951056516295154,1.,0.951056516295154,1.,0.951056516295154,1.,0.951056516295154,
1.,0.951056516295154,1.,0.951056516295154,1.,0.951056516295154,1.,0.951056516295154,
1.,0.951056516295154,1.,0.951056516295154,1.,0.951056516295154,1.,0.951056516295154,
1.,0.951056516295154,1.,0.951056516295154,1.,0.951056516295154,1.,0.951056516295154,
1.,0.951056516295154,1.,0.951056516295154,1.,0.951056516295154,1.,0.951056516295154,
1.,0.951056516295154,1.,0.951056516295154,1.,0.951056516295154,1.,0.951056516295154,
1.,0.951056516295154,1.,0.951056516295154,1.,0.951056516295154,1.,0.951056516295154,
1.,0.951056516295154,1.,0.951056516295154,1.,0.951056516295154,1.,0.951056516295154,
1.,0.951056516295154,1.,0.951056516295154,1.,0.951056516295154,1.,0.951056516295154,
1.,0.951056516295154,1.,0.951056516295154,1.,0.951056516295154,1.,0.951056516295154,
1.,0.951056516295154,1.,0.951056516295154,1.,0.951056516295154,1.,0.951056516295154,
1.,0.951056516295154,1.,0.951056516295154,1.,0.951056516295154,1.,0.951056516295154,
1.,0.951056516295154,1.,0.951056516295154,1.,0.951056516295154,1.,0.951056516295154,
1.,0.951056516295154,1.,0.951056516295154,1.,0.951056516295154,1.,0.951056516295154,
1.,0.951056516295154,1.,0.951056516295154,1.,0.951056516295154,1.,0.951056516295154,
1.,0.951056516295154,1.,0.951056516295154,1.,0.951056516295154,1.,0.951056516295154,
1.,0.951056516295154,1.,0.951056516295154,1.,0.951056516295154,1.,0.951056516295154,
1.,0.951056516295154,1.,0.951056516295154,1.,0.951056516295154,1.,0.951056516295154,
1.,0.951056516295154,1.,0.951056516295154,1.,0.951056516295154,1.,0.951056516295154,
1.,0.951056516295154,1.,0.951056516295154,1.,0.951056516295154,1.,0.951056516295154,
1.,0.951056516295154,1.,0.951056516295154,1.,0.951056516295154,1.,0.951056516295154,
1.,0.951056516295154,1.,0.951056516295154,1.,0.951056516295154,1.,0.951056516295154,
1.,0.951056516295154,1.,0.951056516295154,1.,0.951056516295154,1.,0.951056516295154,
1.,0.951056516295154,1.,0.951056516295154,1.,0.951056516295154,1.,0.951056516295154,
1.,0.951056516295154,1.,0.951056516295154,1.,0.951056516295154,1.,0.951056516295154,
1.,0.951056516295154,1.,0.951056516295154,1.,0.951056516295154,1.,0.951056516295154,
1.,0.951056516295154,1.,0.951056516295154,1.,0.951056516295154,1.,0.951056516295154,
1.,0.951056516295154,1.,0.951056516295154,1.,0.951056516295154,1.,0.951056516295154,
1.,0.951056516295154,1.,0.951056516295154,1.,0.951056516295154,1.,0.951056516295154,
1.,0.951056516295154,1.,0.951056516295154,1.,0.951056516295154,1.,0.951056516295154,
1.,0.951056516295154,1.,0.951056516295154,1.,0.951056516295154,1.,0.951056516295154,
1.,0.951056516295154,1.,0.951056516295154,1.,0.951056516295154,1.,0.951056516295154,
1.,0.951056516295154,1.,0.951056516295154,1.,0.951056516295154,1.,0.951056516295154,
1.,0.951056516295154,1.,0.951056516295154,1.,0.951056516295154,1.,0.951056516295154,
1.,0.951056516295154,1.,0.951056516295154,1.,0.951056516295154,1.,0.951056516295154,
1.,0.951056516295154,1.,0.951056516295154,1.,0.951056516295154,1.,0.951056516295154,
1.,0.951056516295154,1.,0.951056516295154,1.,0.951056516295154,1.,0.951056516295154,
1.,0.951056516295154,1.,0.951056516295154,1.,0.951056516295154,1.,0.951056516295154,
1.,0.951056516295154,1.,0.951056516295154,1.,0.951056516295154,1.,0.951056516295154,
1.,0.951056516295154,1.,0.951056516295154,1.,0.951056516295154,1.,0.951056516295154,
1.,0.951056516295154,1.,0.951056516295154,1.,0.951056516295154,1.,0.951056516295154,
1.,0.951056516295154,1.,0.951056516295154,1.,0.951056516295154,1.,0.951056516295154,
1.,0.951056516295154,1.,0.951056516295154,1.,0.951056516295154,1.,0.951056516295154,
1.,0.951056516295154,1.,0.951056516295154,1.,0.951056516295154,1.,0.951056516295154,
1.,0.951056516295154,1.,0.951056516295154,1.,0.951056516295154,1.,0.951056516295154,
1.,0.951056516295154,1.,0.951056516295154,1.,0.951056516295154,1.,0.951056516295154,
1.,0.951056516295154,1.,0.951056516295154,1.,0.951056516295154,1.,0.951056516295154,
1.,0.951056516295154,1.,0.951056516295154,1.,0.951056516295154,1.,0.951056516295154,
1.,0.951056516295154,1.,0.951056516295154,1.,0.951056516295154,1.,0.951056516295154,
1.,0.951056516295154,1.,0.951056516295154,1.,0.951056516295154,1.,0.951056516295154,
1.,0.951056516295154,1.,0.951056516295154,1.,0.951056516295154,1.,0.951056516295154,
1.,0.951056516295154,1.,0.951056516295154,1.,0.951056516295154,1.,0.951056516295154,
1.,0.951056516295154,1.,0.951056516295154,1.,0.951056516295154,1.,0.951056516295154,
1.,0.951056516295154,1.,0.951056516295154,1.,0.951056516295154,1.,0.951056516295154,
1.,0.951056516295154,1.,0.951056516295154,1.,0.951056516295154,1.,0.951056516295154,
1.,0.951056516295154,1.,0.951056516295154,1.,0.951056516295154,1.,0.951056516295154,
1.,0.951056516295154,1.,0.951056516295154,1.,0.951056516295154,1.,0.951056516295154,
1.,0.951056516295154,1.,0.951056516295154,1.,0.951056516295154,1.,0.951056516295154,
1.,0.951056516295154,1.,0.951056516295154,1.,0.951056516295154,1.,0.951056516295154,
1.,0.951056516295154,1.,0.951056516295154,1.,0.951056516295154,1.,0.951056516295154,
1.,0.951056516295154,1.,0.951056516295154,1.,0.951056516295154,1.,0.951056516295154,
1.,0.951056516295154,1.,0.951056516295154,1.,0.951056516295154,1.,0.951056516295154,
1.,0.951056516295154,1.,0.951056516295154,1.,0.951056516295154,1.,0.951056516295154,
1.,0.951056516295154,1.,0.951056516295154,1.,0.951056516295154,1.,0.951056516295154,
1.,0.951056516295154,1.,0.951056516295154,1.,0.951056516295154,1.,0.951056516295154,
1.,0.951056516295154,1.,0.951056516295154,1.,0.951056516295154,1.,0.951056516295154,
1.,0.951056516295154,1.,0.951056516295154,1.,0.951056516295154,1.,0.951056516295154,
1.,0.951056516295154,1.,0.951056516295154,1.,0.951056516295154,1.,0.951056516295154,
1.,0.951056516295154,1.,0.951056516295154,1.,0.951056516295154,1.,0.951056516295154,
1.,0.951056516295154,1.,0.951056516295154,1.,0.951056516295154,1.,0.951056516295154,
1.,0.951056516295154,1.,0.951056516295154,1.,0.951056516295154,1.,0.951056516295154,
1.,0.951056516295154,1.,0.951056516295154,1.,0.951056516295154,1.,0.951056516295154,
1.,0.951056516295154,1.,0.951056516295154,1.,0.951056516295154,1.,0.951056516295154,
1.,0.951056516295154,1.,0.951056516295154,1.,0.951056516295154,1.,0.951056516295154,
1.,0.951056516295154,1.,0.951056516295154,1.,0.951056516295154,1.,0.951056516295154,
1.,0.951056516295154,1.,0.951056516295154,1.,0.951056516295154,1.,0.951056516295154,
1.,0.951056516295154,1.,0.951056516295154,1.,0.951056516295154,1.,0.951056516295154,
1.,0.951056516295154,1.,0.951056516295154,1.,0.951056516295154,1.,0.951056516295154,
1.,0.951056516295154,1.,0.951056516295154,1.,0.951056516295154,1.,0.951056516295154,
1.,0.951056516295154,1.,0.951056516295154,1.,0.951056516295154,1.,0.951056516295154,
1.,0.951056516295154,1.,0.951056516295154,1.,0.951056516295154,1.,0.951056516295154,
1.,0.951056516295154,1.,0.951056516295154,1.,0.951056516295154,1.,0.951056516295154,
1.,0.951056516295154,1.,0.951056516295154,1.,0.951056516295154,1.,0.951056516295154,
1.,0.951056516295154,1.,0.951056516295154,1.,0.951056516295154,1.,0.951056516295154,
1.,0.951056516295154,1.,0.951056516295154,1.,0.951056516295154,1.,0.951056516295154,
1.,0.951056516295154,1.,0.951056516295154,1.,0.951056516295154,1.,0.951056516295154,
1.,0.951056516295154,1.,0.951056516295154,1.,0.951056516295154,1.,0.951056516295154,
1.,0.951056516295154,1.,0.951056516295154,1.,0.951056516295154,1.,0.951056516295154,
1.,0.951056516295154,1.,0.951056516295154,1.,0.951056516295154,1.,0.951056516295154,
1.,0.951056516295154,1.,0.951056516295154,1.,0.951056516295154,1.,0.951056516295154,
1.,0.951056516295154,1.,0.951056516295154,1.,0.951056516295154,1.,0.951056516295154,
1.,0.951056516295154,1.,0.951056516295154,1.,0.951056516295154,1.,0.951056516295154,
1.,0.951056516295154,1.,0.951056516295154,1.,0.951056516295154,1.,0.951056516295154,
1.,0.951056516295154,1.,0.951056516295154,1.,0.951056516295154,1.)))
REPRESENTATION_ITEM('')
SURFACE()
);
#3195=(
BOUNDED_SURFACE()
B_SPLINE_SURFACE(1,2,((#283610,#283611,#283612,#283613,#283614,#283615,
#283616,#283617,#283618,#283619,#283620,#283621,#283622,#283623,#283624,
#283625,#283626,#283627,#283628,#283629,#283630,#283631,#283632,#283633,
#283634,#283635,#283636,#283637,#283638,#283639,#283640,#283641,#283642,
#283643,#283644,#283645,#283646,#283647,#283648,#283649,#283650,#283651,
#283652,#283653,#283654,#283655,#283656,#283657,#283658,#283659,#283660,
#283661,#283662,#283663,#283664,#283665,#283666,#283667,#283668,#283669,
#283670,#283671,#283672,#283673,#283674,#283675,#283676,#283677,#283678,
#283679,#283680,#283681,#283682,#283683,#283684,#283685,#283686,#283687,
#283688,#283689,#283690,#283691,#283692,#283693,#283694,#283695,#283696,
#283697,#283698,#283699,#283700,#283701,#283702,#283703,#283704,#283705,
#283706,#283707,#283708,#283709,#283710,#283711,#283712,#283713,#283714,
#283715,#283716,#283717,#283718,#283719,#283720,#283721,#283722,#283723,
#283724,#283725,#283726,#283727,#283728,#283729,#283730,#283731,#283732,
#283733,#283734,#283735,#283736,#283737,#283738,#283739,#283740,#283741,
#283742,#283743,#283744,#283745,#283746,#283747,#283748,#283749,#283750,
#283751,#283752,#283753,#283754,#283755,#283756,#283757,#283758,#283759,
#283760,#283761,#283762,#283763,#283764,#283765,#283766,#283767,#283768,
#283769,#283770,#283771,#283772,#283773,#283774,#283775,#283776,#283777,
#283778,#283779,#283780,#283781,#283782,#283783,#283784,#283785,#283786,
#283787,#283788,#283789,#283790,#283791,#283792,#283793,#283794,#283795,
#283796,#283797,#283798,#283799,#283800,#283801,#283802,#283803,#283804,
#283805,#283806,#283807,#283808,#283809,#283810,#283811,#283812,#283813,
#283814,#283815,#283816,#283817,#283818,#283819,#283820,#283821,#283822,
#283823,#283824,#283825,#283826,#283827,#283828,#283829,#283830,#283831,
#283832,#283833,#283834,#283835,#283836,#283837,#283838,#283839,#283840,
#283841,#283842,#283843,#283844,#283845,#283846,#283847,#283848,#283849,
#283850,#283851,#283852,#283853,#283854,#283855,#283856,#283857,#283858,
#283859,#283860,#283861,#283862,#283863,#283864,#283865,#283866,#283867,
#283868,#283869,#283870,#283871,#283872,#283873,#283874,#283875,#283876,
#283877,#283878,#283879,#283880,#283881,#283882,#283883,#283884,#283885,
#283886,#283887,#283888,#283889,#283890,#283891,#283892,#283893,#283894,
#283895,#283896,#283897,#283898,#283899,#283900,#283901,#283902,#283903,
#283904,#283905,#283906,#283907,#283908,#283909,#283910,#283911,#283912,
#283913,#283914,#283915,#283916,#283917,#283918,#283919,#283920,#283921,
#283922,#283923,#283924,#283925,#283926,#283927,#283928,#283929,#283930,
#283931,#283932,#283933,#283934,#283935,#283936,#283937,#283938,#283939,
#283940,#283941,#283942,#283943,#283944,#283945,#283946,#283947,#283948,
#283949,#283950,#283951,#283952,#283953,#283954,#283955,#283956,#283957,
#283958,#283959,#283960,#283961,#283962,#283963,#283964,#283965,#283966,
#283967,#283968,#283969,#283970,#283971,#283972,#283973,#283974,#283975,
#283976,#283977,#283978,#283979,#283980,#283981,#283982,#283983,#283984,
#283985,#283986,#283987,#283988,#283989,#283990,#283991,#283992,#283993,
#283994,#283995,#283996,#283997,#283998,#283999,#284000,#284001,#284002,
#284003,#284004,#284005,#284006,#284007,#284008,#284009,#284010,#284011,
#284012,#284013,#284014,#284015,#284016,#284017,#284018,#284019,#284020,
#284021,#284022,#284023,#284024,#284025,#284026,#284027,#284028,#284029,
#284030,#284031,#284032,#284033,#284034,#284035,#284036,#284037,#284038,
#284039,#284040,#284041,#284042,#284043,#284044,#284045,#284046,#284047,
#284048,#284049,#284050,#284051,#284052,#284053,#284054,#284055,#284056,
#284057,#284058,#284059,#284060,#284061,#284062,#284063,#284064,#284065,
#284066,#284067,#284068,#284069,#284070,#284071,#284072,#284073,#284074,
#284075,#284076,#284077,#284078,#284079,#284080,#284081,#284082,#284083,
#284084,#284085,#284086,#284087,#284088,#284089,#284090,#284091,#284092,
#284093,#284094,#284095,#284096,#284097,#284098,#284099,#284100,#284101,
#284102,#284103,#284104,#284105,#284106,#284107,#284108,#284109,#284110,
#284111,#284112,#284113,#284114,#284115,#284116,#284117,#284118,#284119,
#284120,#284121,#284122,#284123,#284124,#284125,#284126,#284127,#284128,
#284129,#284130,#284131,#284132,#284133,#284134,#284135,#284136,#284137,
#284138,#284139,#284140,#284141,#284142,#284143,#284144,#284145,#284146,
#284147,#284148,#284149,#284150,#284151,#284152,#284153,#284154,#284155,
#284156,#284157,#284158,#284159,#284160,#284161,#284162,#284163,#284164,
#284165,#284166,#284167,#284168,#284169,#284170,#284171,#284172,#284173,
#284174,#284175,#284176,#284177,#284178,#284179,#284180,#284181,#284182,
#284183,#284184,#284185,#284186,#284187,#284188,#284189,#284190,#284191,
#284192,#284193,#284194,#284195,#284196,#284197,#284198,#284199,#284200,
#284201,#284202,#284203,#284204,#284205,#284206,#284207,#284208,#284209,
#284210,#284211,#284212,#284213,#284214,#284215,#284216,#284217,#284218,
#284219,#284220,#284221,#284222,#284223,#284224,#284225,#284226,#284227,
#284228,#284229,#284230,#284231,#284232,#284233,#284234,#284235,#284236,
#284237,#284238,#284239,#284240,#284241,#284242,#284243,#284244,#284245,
#284246,#284247,#284248,#284249,#284250,#284251,#284252,#284253,#284254,
#284255,#284256,#284257,#284258,#284259,#284260,#284261,#284262,#284263,
#284264,#284265,#284266,#284267,#284268,#284269,#284270,#284271,#284272,
#284273,#284274,#284275,#284276,#284277,#284278,#284279,#284280,#284281,
#284282,#284283,#284284,#284285,#284286,#284287,#284288,#284289,#284290,
#284291,#284292,#284293,#284294,#284295,#284296,#284297,#284298,#284299,
#284300,#284301,#284302,#284303,#284304,#284305,#284306,#284307,#284308,
#284309,#284310,#284311,#284312,#284313,#284314,#284315,#284316,#284317,
#284318,#284319,#284320,#284321,#284322,#284323,#284324,#284325,#284326,
#284327,#284328,#284329,#284330,#284331,#284332,#284333,#284334,#284335,
#284336,#284337,#284338,#284339,#284340,#284341,#284342,#284343,#284344,
#284345,#284346,#284347,#284348,#284349,#284350,#284351,#284352,#284353,
#284354,#284355,#284356,#284357,#284358,#284359,#284360,#284361,#284362,
#284363,#284364,#284365,#284366,#284367,#284368,#284369,#284370,#284371,
#284372,#284373,#284374,#284375,#284376,#284377,#284378,#284379,#284380,
#284381,#284382,#284383,#284384,#284385,#284386,#284387,#284388,#284389,
#284390,#284391,#284392,#284393,#284394,#284395,#284396,#284397,#284398,
#284399,#284400,#284401,#284402,#284403,#284404,#284405,#284406,#284407,
#284408,#284409,#284410,#284411,#284412,#284413,#284414,#284415,#284416,
#284417,#284418,#284419,#284420,#284421,#284422,#284423,#284424,#284425,
#284426,#284427,#284428,#284429,#284430,#284431,#284432,#284433,#284434,
#284435,#284436,#284437,#284438,#284439,#284440,#284441,#284442,#284443,
#284444,#284445,#284446,#284447,#284448,#284449,#284450,#284451,#284452,
#284453,#284454,#284455,#284456,#284457,#284458,#284459,#284460,#284461,
#284462,#284463,#284464,#284465,#284466,#284467,#284468,#284469,#284470,
#284471,#284472,#284473,#284474,#284475,#284476,#284477,#284478,#284479,
#284480,#284481,#284482,#284483,#284484,#284485,#284486,#284487,#284488,
#284489,#284490,#284491,#284492,#284493,#284494,#284495,#284496,#284497,
#284498,#284499,#284500,#284501,#284502,#284503,#284504,#284505,#284506,
#284507,#284508,#284509,#284510,#284511,#284512,#284513,#284514,#284515,
#284516,#284517,#284518,#284519,#284520,#284521,#284522,#284523,#284524,
#284525,#284526,#284527,#284528,#284529,#284530,#284531,#284532,#284533,
#284534,#284535,#284536,#284537,#284538,#284539,#284540,#284541,#284542,
#284543,#284544,#284545,#284546,#284547,#284548,#284549,#284550,#284551,
#284552,#284553,#284554,#284555,#284556,#284557,#284558,#284559,#284560,
#284561,#284562,#284563,#284564,#284565,#284566,#284567,#284568,#284569,
#284570,#284571,#284572,#284573,#284574,#284575,#284576,#284577,#284578,
#284579,#284580,#284581,#284582,#284583,#284584,#284585,#284586,#284587,
#284588,#284589,#284590,#284591,#284592,#284593,#284594,#284595,#284596,
#284597,#284598,#284599,#284600,#284601,#284602,#284603,#284604,#284605,
#284606,#284607,#284608,#284609,#284610,#284611,#284612,#284613,#284614,
#284615,#284616,#284617,#284618,#284619,#284620,#284621,#284622,#284623,
#284624,#284625,#284626,#284627,#284628,#284629,#284630,#284631,#284632,
#284633,#284634,#284635,#284636,#284637,#284638,#284639,#284640,#284641,
#284642,#284643,#284644,#284645,#284646),(#284647,#284648,#284649,#284650,
#284651,#284652,#284653,#284654,#284655,#284656,#284657,#284658,#284659,
#284660,#284661,#284662,#284663,#284664,#284665,#284666,#284667,#284668,
#284669,#284670,#284671,#284672,#284673,#284674,#284675,#284676,#284677,
#284678,#284679,#284680,#284681,#284682,#284683,#284684,#284685,#284686,
#284687,#284688,#284689,#284690,#284691,#284692,#284693,#284694,#284695,
#284696,#284697,#284698,#284699,#284700,#284701,#284702,#284703,#284704,
#284705,#284706,#284707,#284708,#284709,#284710,#284711,#284712,#284713,
#284714,#284715,#284716,#284717,#284718,#284719,#284720,#284721,#284722,
#284723,#284724,#284725,#284726,#284727,#284728,#284729,#284730,#284731,
#284732,#284733,#284734,#284735,#284736,#284737,#284738,#284739,#284740,
#284741,#284742,#284743,#284744,#284745,#284746,#284747,#284748,#284749,
#284750,#284751,#284752,#284753,#284754,#284755,#284756,#284757,#284758,
#284759,#284760,#284761,#284762,#284763,#284764,#284765,#284766,#284767,
#284768,#284769,#284770,#284771,#284772,#284773,#284774,#284775,#284776,
#284777,#284778,#284779,#284780,#284781,#284782,#284783,#284784,#284785,
#284786,#284787,#284788,#284789,#284790,#284791,#284792,#284793,#284794,
#284795,#284796,#284797,#284798,#284799,#284800,#284801,#284802,#284803,
#284804,#284805,#284806,#284807,#284808,#284809,#284810,#284811,#284812,
#284813,#284814,#284815,#284816,#284817,#284818,#284819,#284820,#284821,
#284822,#284823,#284824,#284825,#284826,#284827,#284828,#284829,#284830,
#284831,#284832,#284833,#284834,#284835,#284836,#284837,#284838,#284839,
#284840,#284841,#284842,#284843,#284844,#284845,#284846,#284847,#284848,
#284849,#284850,#284851,#284852,#284853,#284854,#284855,#284856,#284857,
#284858,#284859,#284860,#284861,#284862,#284863,#284864,#284865,#284866,
#284867,#284868,#284869,#284870,#284871,#284872,#284873,#284874,#284875,
#284876,#284877,#284878,#284879,#284880,#284881,#284882,#284883,#284884,
#284885,#284886,#284887,#284888,#284889,#284890,#284891,#284892,#284893,
#284894,#284895,#284896,#284897,#284898,#284899,#284900,#284901,#284902,
#284903,#284904,#284905,#284906,#284907,#284908,#284909,#284910,#284911,
#284912,#284913,#284914,#284915,#284916,#284917,#284918,#284919,#284920,
#284921,#284922,#284923,#284924,#284925,#284926,#284927,#284928,#284929,
#284930,#284931,#284932,#284933,#284934,#284935,#284936,#284937,#284938,
#284939,#284940,#284941,#284942,#284943,#284944,#284945,#284946,#284947,
#284948,#284949,#284950,#284951,#284952,#284953,#284954,#284955,#284956,
#284957,#284958,#284959,#284960,#284961,#284962,#284963,#284964,#284965,
#284966,#284967,#284968,#284969,#284970,#284971,#284972,#284973,#284974,
#284975,#284976,#284977,#284978,#284979,#284980,#284981,#284982,#284983,
#284984,#284985,#284986,#284987,#284988,#284989,#284990,#284991,#284992,
#284993,#284994,#284995,#284996,#284997,#284998,#284999,#285000,#285001,
#285002,#285003,#285004,#285005,#285006,#285007,#285008,#285009,#285010,
#285011,#285012,#285013,#285014,#285015,#285016,#285017,#285018,#285019,
#285020,#285021,#285022,#285023,#285024,#285025,#285026,#285027,#285028,
#285029,#285030,#285031,#285032,#285033,#285034,#285035,#285036,#285037,
#285038,#285039,#285040,#285041,#285042,#285043,#285044,#285045,#285046,
#285047,#285048,#285049,#285050,#285051,#285052,#285053,#285054,#285055,
#285056,#285057,#285058,#285059,#285060,#285061,#285062,#285063,#285064,
#285065,#285066,#285067,#285068,#285069,#285070,#285071,#285072,#285073,
#285074,#285075,#285076,#285077,#285078,#285079,#285080,#285081,#285082,
#285083,#285084,#285085,#285086,#285087,#285088,#285089,#285090,#285091,
#285092,#285093,#285094,#285095,#285096,#285097,#285098,#285099,#285100,
#285101,#285102,#285103,#285104,#285105,#285106,#285107,#285108,#285109,
#285110,#285111,#285112,#285113,#285114,#285115,#285116,#285117,#285118,
#285119,#285120,#285121,#285122,#285123,#285124,#285125,#285126,#285127,
#285128,#285129,#285130,#285131,#285132,#285133,#285134,#285135,#285136,
#285137,#285138,#285139,#285140,#285141,#285142,#285143,#285144,#285145,
#285146,#285147,#285148,#285149,#285150,#285151,#285152,#285153,#285154,
#285155,#285156,#285157,#285158,#285159,#285160,#285161,#285162,#285163,
#285164,#285165,#285166,#285167,#285168,#285169,#285170,#285171,#285172,
#285173,#285174,#285175,#285176,#285177,#285178,#285179,#285180,#285181,
#285182,#285183,#285184,#285185,#285186,#285187,#285188,#285189,#285190,
#285191,#285192,#285193,#285194,#285195,#285196,#285197,#285198,#285199,
#285200,#285201,#285202,#285203,#285204,#285205,#285206,#285207,#285208,
#285209,#285210,#285211,#285212,#285213,#285214,#285215,#285216,#285217,
#285218,#285219,#285220,#285221,#285222,#285223,#285224,#285225,#285226,
#285227,#285228,#285229,#285230,#285231,#285232,#285233,#285234,#285235,
#285236,#285237,#285238,#285239,#285240,#285241,#285242,#285243,#285244,
#285245,#285246,#285247,#285248,#285249,#285250,#285251,#285252,#285253,
#285254,#285255,#285256,#285257,#285258,#285259,#285260,#285261,#285262,
#285263,#285264,#285265,#285266,#285267,#285268,#285269,#285270,#285271,
#285272,#285273,#285274,#285275,#285276,#285277,#285278,#285279,#285280,
#285281,#285282,#285283,#285284,#285285,#285286,#285287,#285288,#285289,
#285290,#285291,#285292,#285293,#285294,#285295,#285296,#285297,#285298,
#285299,#285300,#285301,#285302,#285303,#285304,#285305,#285306,#285307,
#285308,#285309,#285310,#285311,#285312,#285313,#285314,#285315,#285316,
#285317,#285318,#285319,#285320,#285321,#285322,#285323,#285324,#285325,
#285326,#285327,#285328,#285329,#285330,#285331,#285332,#285333,#285334,
#285335,#285336,#285337,#285338,#285339,#285340,#285341,#285342,#285343,
#285344,#285345,#285346,#285347,#285348,#285349,#285350,#285351,#285352,
#285353,#285354,#285355,#285356,#285357,#285358,#285359,#285360,#285361,
#285362,#285363,#285364,#285365,#285366,#285367,#285368,#285369,#285370,
#285371,#285372,#285373,#285374,#285375,#285376,#285377,#285378,#285379,
#285380,#285381,#285382,#285383,#285384,#285385,#285386,#285387,#285388,
#285389,#285390,#285391,#285392,#285393,#285394,#285395,#285396,#285397,
#285398,#285399,#285400,#285401,#285402,#285403,#285404,#285405,#285406,
#285407,#285408,#285409,#285410,#285411,#285412,#285413,#285414,#285415,
#285416,#285417,#285418,#285419,#285420,#285421,#285422,#285423,#285424,
#285425,#285426,#285427,#285428,#285429,#285430,#285431,#285432,#285433,
#285434,#285435,#285436,#285437,#285438,#285439,#285440,#285441,#285442,
#285443,#285444,#285445,#285446,#285447,#285448,#285449,#285450,#285451,
#285452,#285453,#285454,#285455,#285456,#285457,#285458,#285459,#285460,
#285461,#285462,#285463,#285464,#285465,#285466,#285467,#285468,#285469,
#285470,#285471,#285472,#285473,#285474,#285475,#285476,#285477,#285478,
#285479,#285480,#285481,#285482,#285483,#285484,#285485,#285486,#285487,
#285488,#285489,#285490,#285491,#285492,#285493,#285494,#285495,#285496,
#285497,#285498,#285499,#285500,#285501,#285502,#285503,#285504,#285505,
#285506,#285507,#285508,#285509,#285510,#285511,#285512,#285513,#285514,
#285515,#285516,#285517,#285518,#285519,#285520,#285521,#285522,#285523,
#285524,#285525,#285526,#285527,#285528,#285529,#285530,#285531,#285532,
#285533,#285534,#285535,#285536,#285537,#285538,#285539,#285540,#285541,
#285542,#285543,#285544,#285545,#285546,#285547,#285548,#285549,#285550,
#285551,#285552,#285553,#285554,#285555,#285556,#285557,#285558,#285559,
#285560,#285561,#285562,#285563,#285564,#285565,#285566,#285567,#285568,
#285569,#285570,#285571,#285572,#285573,#285574,#285575,#285576,#285577,
#285578,#285579,#285580,#285581,#285582,#285583,#285584,#285585,#285586,
#285587,#285588,#285589,#285590,#285591,#285592,#285593,#285594,#285595,
#285596,#285597,#285598,#285599,#285600,#285601,#285602,#285603,#285604,
#285605,#285606,#285607,#285608,#285609,#285610,#285611,#285612,#285613,
#285614,#285615,#285616,#285617,#285618,#285619,#285620,#285621,#285622,
#285623,#285624,#285625,#285626,#285627,#285628,#285629,#285630,#285631,
#285632,#285633,#285634,#285635,#285636,#285637,#285638,#285639,#285640,
#285641,#285642,#285643,#285644,#285645,#285646,#285647,#285648,#285649,
#285650,#285651,#285652,#285653,#285654,#285655,#285656,#285657,#285658,
#285659,#285660,#285661,#285662,#285663,#285664,#285665,#285666,#285667,
#285668,#285669,#285670,#285671,#285672,#285673,#285674,#285675,#285676,
#285677,#285678,#285679,#285680,#285681,#285682,#285683)),.UNSPECIFIED.,
 .F.,.F.,.F.)
B_SPLINE_SURFACE_WITH_KNOTS((2,2),(3,2,2,2,2,2,2,2,2,2,2,2,2,2,2,2,2,2,
2,2,2,2,2,2,2,2,2,2,2,2,2,2,2,2,2,2,2,2,2,2,2,2,2,2,2,2,2,2,2,2,2,2,2,2,
2,2,2,2,2,2,2,2,2,2,2,2,2,2,2,2,2,2,2,2,2,2,2,2,2,2,2,2,2,2,2,2,2,2,2,2,
2,2,2,2,2,2,2,2,2,2,2,2,2,2,2,2,2,2,2,2,2,2,2,2,2,2,2,2,2,2,2,2,2,2,2,2,
2,2,2,2,2,2,2,2,2,2,2,2,2,2,2,2,2,2,2,2,2,2,2,2,2,2,2,2,2,2,2,2,2,2,2,2,
2,2,2,2,2,2,2,2,2,2,2,2,2,2,2,2,2,2,2,2,2,2,2,2,2,2,2,2,2,2,2,2,2,2,2,2,
2,2,2,2,2,2,2,2,2,2,2,2,2,2,2,2,2,2,2,2,2,2,2,2,2,2,2,2,2,2,2,2,2,2,2,2,
2,2,2,2,2,2,2,2,2,2,2,2,2,2,2,2,2,2,2,2,2,2,2,2,2,2,2,2,2,2,2,2,2,2,2,2,
2,2,2,2,2,2,2,2,2,2,2,2,2,2,2,2,2,2,2,2,2,2,2,2,2,2,2,2,2,2,2,2,2,2,2,2,
2,2,2,2,2,2,2,2,2,2,2,2,2,2,2,2,2,2,2,2,2,2,2,2,2,2,2,2,2,2,2,2,2,2,2,2,
2,2,2,2,2,2,2,2,2,2,2,2,2,2,2,2,2,2,2,2,2,2,2,2,2,2,2,2,2,2,2,2,2,2,2,2,
2,2,2,2,2,2,2,2,2,2,2,2,2,2,2,2,2,2,2,2,2,2,2,2,2,2,2,2,2,2,2,2,2,2,2,2,
2,2,2,2,2,2,2,2,2,2,2,2,2,2,2,2,2,2,2,2,2,2,2,2,2,2,2,2,2,2,2,2,2,2,2,2,
2,2,2,2,2,2,2,2,2,2,2,2,2,2,2,2,2,2,2,2,2,2,2,2,2,2,2,2,2,2,2,2,2,2,2,2,
2,2,2,2,2,2,2,2,2,2,2,2,2,2,2,2,2,2,2,2,2,2,2,2,2,2,2,2,2,2,2,2,3),(0.,
1.00000449367228),(0.,0.00192307692307692,0.00384615384615385,0.00576923076923077,
0.00769230769230769,0.00961538461538462,0.0115384615384615,0.0134615384615385,
0.0153846153846154,0.0173076923076923,0.0192307692307692,0.0211538461538462,
0.0230769230769231,0.025,0.0269230769230769,0.0288461538461538,0.0307692307692308,
0.0326923076923077,0.0346153846153846,0.0365384615384615,0.0384615384615385,
0.0403846153846154,0.0423076923076923,0.0442307692307692,0.0461538461538462,
0.0480769230769231,0.05,0.0519230769230769,0.0538461538461538,0.0557692307692308,
0.0576923076923077,0.0596153846153846,0.0615384615384615,0.0634615384615385,
0.0653846153846154,0.0673076923076923,0.0692307692307692,0.0711538461538462,
0.0730769230769231,0.075,0.0769230769230769,0.0788461538461538,0.0807692307692308,
0.0826923076923077,0.0846153846153846,0.0865384615384615,0.0884615384615385,
0.0903846153846154,0.0923076923076923,0.0942307692307692,0.0961538461538462,
0.0980769230769231,0.1,0.101923076923077,0.103846153846154,0.105769230769231,
0.107692307692308,0.109615384615385,0.111538461538462,0.113461538461538,
0.115384615384615,0.117307692307692,0.119230769230769,0.121153846153846,
0.123076923076923,0.125,0.126923076923077,0.128846153846154,0.130769230769231,
0.132692307692308,0.134615384615385,0.136538461538462,0.138461538461538,
0.140384615384615,0.142307692307692,0.144230769230769,0.146153846153846,
0.148076923076923,0.15,0.151923076923077,0.153846153846154,0.155769230769231,
0.157692307692308,0.159615384615385,0.161538461538462,0.163461538461538,
0.165384615384615,0.167307692307692,0.169230769230769,0.171153846153846,
0.173076923076923,0.175,0.176923076923077,0.178846153846154,0.180769230769231,
0.182692307692308,0.184615384615385,0.186538461538462,0.188461538461538,
0.190384615384615,0.192307692307692,0.194230769230769,0.196153846153846,
0.198076923076923,0.2,0.201923076923077,0.203846153846154,0.205769230769231,
0.207692307692308,0.209615384615385,0.211538461538462,0.213461538461538,
0.215384615384615,0.217307692307692,0.219230769230769,0.221153846153846,
0.223076923076923,0.225,0.226923076923077,0.228846153846154,0.230769230769231,
0.232692307692308,0.234615384615385,0.236538461538462,0.238461538461538,
0.240384615384615,0.242307692307692,0.244230769230769,0.246153846153846,
0.248076923076923,0.25,0.251923076923077,0.253846153846154,0.255769230769231,
0.257692307692308,0.259615384615385,0.261538461538462,0.263461538461538,
0.265384615384615,0.267307692307692,0.269230769230769,0.271153846153846,
0.273076923076923,0.275,0.276923076923077,0.278846153846154,0.280769230769231,
0.282692307692308,0.284615384615385,0.286538461538462,0.288461538461538,
0.290384615384615,0.292307692307692,0.294230769230769,0.296153846153846,
0.298076923076923,0.3,0.301923076923077,0.303846153846154,0.305769230769231,
0.307692307692308,0.309615384615385,0.311538461538462,0.313461538461538,
0.315384615384615,0.317307692307692,0.319230769230769,0.321153846153846,
0.323076923076923,0.325,0.326923076923077,0.328846153846154,0.330769230769231,
0.332692307692308,0.334615384615385,0.336538461538462,0.338461538461538,
0.340384615384615,0.342307692307692,0.344230769230769,0.346153846153846,
0.348076923076923,0.35,0.351923076923077,0.353846153846154,0.355769230769231,
0.357692307692308,0.359615384615385,0.361538461538462,0.363461538461538,
0.365384615384615,0.367307692307692,0.369230769230769,0.371153846153846,
0.373076923076923,0.375,0.376923076923077,0.378846153846154,0.380769230769231,
0.382692307692308,0.384615384615385,0.386538461538462,0.388461538461538,
0.390384615384615,0.392307692307692,0.394230769230769,0.396153846153846,
0.398076923076923,0.4,0.401923076923077,0.403846153846154,0.405769230769231,
0.407692307692308,0.409615384615385,0.411538461538462,0.413461538461538,
0.415384615384615,0.417307692307692,0.419230769230769,0.421153846153846,
0.423076923076923,0.425,0.426923076923077,0.428846153846154,0.430769230769231,
0.432692307692308,0.434615384615385,0.436538461538462,0.438461538461538,
0.440384615384615,0.442307692307692,0.444230769230769,0.446153846153846,
0.448076923076923,0.45,0.451923076923077,0.453846153846154,0.455769230769231,
0.457692307692308,0.459615384615385,0.461538461538462,0.463461538461538,
0.465384615384615,0.467307692307692,0.469230769230769,0.471153846153846,
0.473076923076923,0.475,0.476923076923077,0.478846153846154,0.480769230769231,
0.482692307692308,0.484615384615385,0.486538461538462,0.488461538461538,
0.490384615384615,0.492307692307692,0.494230769230769,0.496153846153846,
0.498076923076923,0.5,0.501923076923077,0.503846153846154,0.505769230769231,
0.507692307692308,0.509615384615385,0.511538461538461,0.513461538461538,
0.515384615384615,0.517307692307692,0.519230769230769,0.521153846153846,
0.523076923076923,0.525,0.526923076923077,0.528846153846154,0.530769230769231,
0.532692307692308,0.534615384615385,0.536538461538462,0.538461538461538,
0.540384615384615,0.542307692307692,0.544230769230769,0.546153846153846,
0.548076923076923,0.55,0.551923076923077,0.553846153846154,0.555769230769231,
0.557692307692308,0.559615384615385,0.561538461538462,0.563461538461538,
0.565384615384615,0.567307692307692,0.569230769230769,0.571153846153846,
0.573076923076923,0.575,0.576923076923077,0.578846153846154,0.580769230769231,
0.582692307692308,0.584615384615385,0.586538461538462,0.588461538461538,
0.590384615384615,0.592307692307692,0.594230769230769,0.596153846153846,
0.598076923076923,0.6,0.601923076923077,0.603846153846154,0.605769230769231,
0.607692307692308,0.609615384615385,0.611538461538462,0.613461538461539,
0.615384615384615,0.617307692307692,0.619230769230769,0.621153846153846,
0.623076923076923,0.625,0.626923076923077,0.628846153846154,0.630769230769231,
0.632692307692308,0.634615384615385,0.636538461538461,0.638461538461538,
0.640384615384615,0.642307692307692,0.644230769230769,0.646153846153846,
0.648076923076923,0.65,0.651923076923077,0.653846153846154,0.655769230769231,
0.657692307692308,0.659615384615385,0.661538461538462,0.663461538461538,
0.665384615384615,0.667307692307692,0.669230769230769,0.671153846153846,
0.673076923076923,0.675,0.676923076923077,0.678846153846154,0.680769230769231,
0.682692307692308,0.684615384615385,0.686538461538462,0.688461538461538,
0.690384615384615,0.692307692307692,0.694230769230769,0.696153846153846,
0.698076923076923,0.7,0.701923076923077,0.703846153846154,0.705769230769231,
0.707692307692308,0.709615384615385,0.711538461538462,0.713461538461538,
0.715384615384615,0.717307692307692,0.719230769230769,0.721153846153846,
0.723076923076923,0.725,0.726923076923077,0.728846153846154,0.730769230769231,
0.732692307692308,0.734615384615385,0.736538461538462,0.738461538461539,
0.740384615384615,0.742307692307692,0.744230769230769,0.746153846153846,
0.748076923076923,0.75,0.751923076923077,0.753846153846154,0.755769230769231,
0.757692307692308,0.759615384615385,0.761538461538461,0.763461538461538,
0.765384615384615,0.767307692307692,0.769230769230769,0.771153846153846,
0.773076923076923,0.775,0.776923076923077,0.778846153846154,0.780769230769231,
0.782692307692308,0.784615384615385,0.786538461538462,0.788461538461538,
0.790384615384615,0.792307692307692,0.794230769230769,0.796153846153846,
0.798076923076923,0.8,0.801923076923077,0.803846153846154,0.805769230769231,
0.807692307692308,0.809615384615385,0.811538461538462,0.813461538461538,
0.815384615384615,0.817307692307692,0.819230769230769,0.821153846153846,
0.823076923076923,0.825,0.826923076923077,0.828846153846154,0.830769230769231,
0.832692307692308,0.834615384615385,0.836538461538462,0.838461538461538,
0.840384615384615,0.842307692307692,0.844230769230769,0.846153846153846,
0.848076923076923,0.85,0.851923076923077,0.853846153846154,0.855769230769231,
0.857692307692308,0.859615384615385,0.861538461538462,0.863461538461539,
0.865384615384615,0.867307692307692,0.869230769230769,0.871153846153846,
0.873076923076923,0.875,0.876923076923077,0.878846153846154,0.880769230769231,
0.882692307692308,0.884615384615385,0.886538461538461,0.888461538461538,
0.890384615384615,0.892307692307692,0.894230769230769,0.896153846153846,
0.898076923076923,0.9,0.901923076923077,0.903846153846154,0.905769230769231,
0.907692307692308,0.909615384615385,0.911538461538462,0.913461538461538,
0.915384615384615,0.917307692307692,0.919230769230769,0.921153846153846,
0.923076923076923,0.925,0.926923076923077,0.928846153846154,0.930769230769231,
0.932692307692308,0.934615384615385,0.936538461538462,0.938461538461538,
0.940384615384615,0.942307692307692,0.944230769230769,0.946153846153846,
0.948076923076923,0.95,0.951923076923077,0.953846153846154,0.955769230769231,
0.957692307692308,0.959615384615385,0.961538461538462,0.963461538461538,
0.965384615384615,0.967307692307692,0.969230769230769,0.971153846153846,
0.973076923076923,0.975,0.976923076923077,0.978846153846154,0.980769230769231,
0.982692307692308,0.984615384615385,0.986538461538462,0.988461538461539,
0.990384615384615,0.992307692307692,0.994230769230769,0.996153846153846),
 .UNSPECIFIED.)
GEOMETRIC_REPRESENTATION_ITEM()
RATIONAL_B_SPLINE_SURFACE(((1.,0.951056516295154,1.,0.951056516295154,1.,
0.951056516295154,1.,0.951056516295154,1.,0.951056516295154,1.,0.951056516295154,
1.,0.951056516295154,1.,0.951056516295154,1.,0.951056516295154,1.,0.951056516295154,
1.,0.951056516295154,1.,0.951056516295154,1.,0.951056516295154,1.,0.951056516295154,
1.,0.951056516295154,1.,0.951056516295154,1.,0.951056516295154,1.,0.951056516295154,
1.,0.951056516295154,1.,0.951056516295154,1.,0.951056516295154,1.,0.951056516295154,
1.,0.951056516295154,1.,0.951056516295154,1.,0.951056516295154,1.,0.951056516295154,
1.,0.951056516295154,1.,0.951056516295154,1.,0.951056516295154,1.,0.951056516295154,
1.,0.951056516295154,1.,0.951056516295154,1.,0.951056516295154,1.,0.951056516295154,
1.,0.951056516295154,1.,0.951056516295154,1.,0.951056516295154,1.,0.951056516295154,
1.,0.951056516295154,1.,0.951056516295154,1.,0.951056516295154,1.,0.951056516295154,
1.,0.951056516295154,1.,0.951056516295154,1.,0.951056516295154,1.,0.951056516295154,
1.,0.951056516295154,1.,0.951056516295154,1.,0.951056516295154,1.,0.951056516295154,
1.,0.951056516295154,1.,0.951056516295154,1.,0.951056516295154,1.,0.951056516295154,
1.,0.951056516295154,1.,0.951056516295154,1.,0.951056516295154,1.,0.951056516295154,
1.,0.951056516295154,1.,0.951056516295154,1.,0.951056516295154,1.,0.951056516295154,
1.,0.951056516295154,1.,0.951056516295154,1.,0.951056516295154,1.,0.951056516295154,
1.,0.951056516295154,1.,0.951056516295154,1.,0.951056516295154,1.,0.951056516295154,
1.,0.951056516295154,1.,0.951056516295154,1.,0.951056516295154,1.,0.951056516295154,
1.,0.951056516295154,1.,0.951056516295154,1.,0.951056516295154,1.,0.951056516295154,
1.,0.951056516295154,1.,0.951056516295154,1.,0.951056516295154,1.,0.951056516295154,
1.,0.951056516295154,1.,0.951056516295154,1.,0.951056516295154,1.,0.951056516295154,
1.,0.951056516295154,1.,0.951056516295154,1.,0.951056516295154,1.,0.951056516295154,
1.,0.951056516295154,1.,0.951056516295154,1.,0.951056516295154,1.,0.951056516295154,
1.,0.951056516295154,1.,0.951056516295154,1.,0.951056516295154,1.,0.951056516295154,
1.,0.951056516295154,1.,0.951056516295154,1.,0.951056516295154,1.,0.951056516295154,
1.,0.951056516295154,1.,0.951056516295154,1.,0.951056516295154,1.,0.951056516295154,
1.,0.951056516295154,1.,0.951056516295154,1.,0.951056516295154,1.,0.951056516295154,
1.,0.951056516295154,1.,0.951056516295154,1.,0.951056516295154,1.,0.951056516295154,
1.,0.951056516295154,1.,0.951056516295154,1.,0.951056516295154,1.,0.951056516295154,
1.,0.951056516295154,1.,0.951056516295154,1.,0.951056516295154,1.,0.951056516295154,
1.,0.951056516295154,1.,0.951056516295154,1.,0.951056516295154,1.,0.951056516295154,
1.,0.951056516295154,1.,0.951056516295154,1.,0.951056516295154,1.,0.951056516295154,
1.,0.951056516295154,1.,0.951056516295154,1.,0.951056516295154,1.,0.951056516295154,
1.,0.951056516295154,1.,0.951056516295154,1.,0.951056516295154,1.,0.951056516295154,
1.,0.951056516295154,1.,0.951056516295154,1.,0.951056516295154,1.,0.951056516295154,
1.,0.951056516295154,1.,0.951056516295154,1.,0.951056516295154,1.,0.951056516295154,
1.,0.951056516295154,1.,0.951056516295154,1.,0.951056516295154,1.,0.951056516295154,
1.,0.951056516295154,1.,0.951056516295154,1.,0.951056516295154,1.,0.951056516295154,
1.,0.951056516295154,1.,0.951056516295154,1.,0.951056516295154,1.,0.951056516295154,
1.,0.951056516295154,1.,0.951056516295154,1.,0.951056516295154,1.,0.951056516295154,
1.,0.951056516295154,1.,0.951056516295154,1.,0.951056516295154,1.,0.951056516295154,
1.,0.951056516295154,1.,0.951056516295154,1.,0.951056516295154,1.,0.951056516295154,
1.,0.951056516295154,1.,0.951056516295154,1.,0.951056516295154,1.,0.951056516295154,
1.,0.951056516295154,1.,0.951056516295154,1.,0.951056516295154,1.,0.951056516295154,
1.,0.951056516295154,1.,0.951056516295154,1.,0.951056516295154,1.,0.951056516295154,
1.,0.951056516295154,1.,0.951056516295154,1.,0.951056516295154,1.,0.951056516295154,
1.,0.951056516295154,1.,0.951056516295154,1.,0.951056516295154,1.,0.951056516295154,
1.,0.951056516295154,1.,0.951056516295154,1.,0.951056516295154,1.,0.951056516295154,
1.,0.951056516295154,1.,0.951056516295154,1.,0.951056516295154,1.,0.951056516295154,
1.,0.951056516295154,1.,0.951056516295154,1.,0.951056516295154,1.,0.951056516295154,
1.,0.951056516295154,1.,0.951056516295154,1.,0.951056516295154,1.,0.951056516295154,
1.,0.951056516295154,1.,0.951056516295154,1.,0.951056516295154,1.,0.951056516295154,
1.,0.951056516295154,1.,0.951056516295154,1.,0.951056516295154,1.,0.951056516295154,
1.,0.951056516295154,1.,0.951056516295154,1.,0.951056516295154,1.,0.951056516295154,
1.,0.951056516295154,1.,0.951056516295154,1.,0.951056516295154,1.,0.951056516295154,
1.,0.951056516295154,1.,0.951056516295154,1.,0.951056516295154,1.,0.951056516295154,
1.,0.951056516295154,1.,0.951056516295154,1.,0.951056516295154,1.,0.951056516295154,
1.,0.951056516295154,1.,0.951056516295154,1.,0.951056516295154,1.,0.951056516295154,
1.,0.951056516295154,1.,0.951056516295154,1.,0.951056516295154,1.,0.951056516295154,
1.,0.951056516295154,1.,0.951056516295154,1.,0.951056516295154,1.,0.951056516295154,
1.,0.951056516295154,1.,0.951056516295154,1.,0.951056516295154,1.,0.951056516295154,
1.,0.951056516295154,1.,0.951056516295154,1.,0.951056516295154,1.,0.951056516295154,
1.,0.951056516295154,1.,0.951056516295154,1.,0.951056516295154,1.,0.951056516295154,
1.,0.951056516295154,1.,0.951056516295154,1.,0.951056516295154,1.,0.951056516295154,
1.,0.951056516295154,1.,0.951056516295154,1.,0.951056516295154,1.,0.951056516295154,
1.,0.951056516295154,1.,0.951056516295154,1.,0.951056516295154,1.,0.951056516295154,
1.,0.951056516295154,1.,0.951056516295154,1.,0.951056516295154,1.,0.951056516295154,
1.,0.951056516295154,1.,0.951056516295154,1.,0.951056516295154,1.,0.951056516295154,
1.,0.951056516295154,1.,0.951056516295154,1.,0.951056516295154,1.,0.951056516295154,
1.,0.951056516295154,1.,0.951056516295154,1.,0.951056516295154,1.,0.951056516295154,
1.,0.951056516295154,1.,0.951056516295154,1.,0.951056516295154,1.,0.951056516295154,
1.,0.951056516295154,1.,0.951056516295154,1.,0.951056516295154,1.,0.951056516295154,
1.,0.951056516295154,1.,0.951056516295154,1.,0.951056516295154,1.,0.951056516295154,
1.,0.951056516295154,1.,0.951056516295154,1.,0.951056516295154,1.,0.951056516295154,
1.,0.951056516295154,1.,0.951056516295154,1.,0.951056516295154,1.,0.951056516295154,
1.,0.951056516295154,1.,0.951056516295154,1.,0.951056516295154,1.,0.951056516295154,
1.,0.951056516295154,1.,0.951056516295154,1.,0.951056516295154,1.,0.951056516295154,
1.,0.951056516295154,1.,0.951056516295154,1.,0.951056516295154,1.,0.951056516295154,
1.,0.951056516295154,1.,0.951056516295154,1.,0.951056516295154,1.,0.951056516295154,
1.,0.951056516295154,1.,0.951056516295154,1.,0.951056516295154,1.,0.951056516295154,
1.,0.951056516295154,1.,0.951056516295154,1.,0.951056516295154,1.,0.951056516295154,
1.,0.951056516295154,1.,0.951056516295154,1.,0.951056516295154,1.,0.951056516295154,
1.,0.951056516295154,1.,0.951056516295154,1.,0.951056516295154,1.,0.951056516295154,
1.,0.951056516295154,1.,0.951056516295154,1.,0.951056516295154,1.,0.951056516295154,
1.,0.951056516295154,1.,0.951056516295154,1.,0.951056516295154,1.,0.951056516295154,
1.,0.951056516295154,1.,0.951056516295154,1.,0.951056516295154,1.,0.951056516295154,
1.,0.951056516295154,1.,0.951056516295154,1.,0.951056516295154,1.,0.951056516295154,
1.,0.951056516295154,1.,0.951056516295154,1.,0.951056516295154,1.,0.951056516295154,
1.,0.951056516295154,1.,0.951056516295154,1.,0.951056516295154,1.,0.951056516295154,
1.,0.951056516295154,1.,0.951056516295154,1.,0.951056516295154,1.,0.951056516295154,
1.,0.951056516295154,1.,0.951056516295154,1.,0.951056516295154,1.,0.951056516295154,
1.,0.951056516295154,1.,0.951056516295154,1.,0.951056516295154,1.,0.951056516295154,
1.,0.951056516295154,1.,0.951056516295154,1.,0.951056516295154,1.,0.951056516295154,
1.,0.951056516295154,1.,0.951056516295154,1.,0.951056516295154,1.,0.951056516295154,
1.,0.951056516295154,1.,0.951056516295154,1.,0.951056516295154,1.,0.951056516295154,
1.,0.951056516295154,1.,0.951056516295154,1.,0.951056516295154,1.,0.951056516295154,
1.,0.951056516295154,1.,0.951056516295154,1.,0.951056516295154,1.,0.951056516295154,
1.,0.951056516295154,1.,0.951056516295154,1.,0.951056516295154,1.,0.951056516295154,
1.,0.951056516295154,1.,0.951056516295154,1.,0.951056516295154,1.,0.951056516295154,
1.,0.951056516295154,1.,0.951056516295154,1.,0.951056516295154,1.,0.951056516295154,
1.,0.951056516295154,1.,0.951056516295154,1.,0.951056516295154,1.,0.951056516295154,
1.,0.951056516295154,1.,0.951056516295154,1.,0.951056516295154,1.,0.951056516295154,
1.,0.951056516295154,1.,0.951056516295154,1.,0.951056516295154,1.,0.951056516295154,
1.,0.951056516295154,1.,0.951056516295154,1.,0.951056516295154,1.,0.951056516295154,
1.,0.951056516295154,1.,0.951056516295154,1.,0.951056516295154,1.,0.951056516295154,
1.,0.951056516295154,1.,0.951056516295154,1.,0.951056516295154,1.,0.951056516295154,
1.,0.951056516295154,1.,0.951056516295154,1.,0.951056516295154,1.,0.951056516295154,
1.,0.951056516295154,1.,0.951056516295154,1.,0.951056516295154,1.,0.951056516295154,
1.,0.951056516295154,1.,0.951056516295154,1.,0.951056516295154,1.,0.951056516295154,
1.,0.951056516295154,1.,0.951056516295154,1.,0.951056516295154,1.,0.951056516295154,
1.,0.951056516295154,1.,0.951056516295154,1.,0.951056516295154,1.,0.951056516295154,
1.,0.951056516295154,1.,0.951056516295154,1.,0.951056516295154,1.,0.951056516295154,
1.,0.951056516295154,1.,0.951056516295154,1.,0.951056516295154,1.,0.951056516295154,
1.,0.951056516295154,1.,0.951056516295154,1.,0.951056516295154,1.,0.951056516295154,
1.,0.951056516295154,1.,0.951056516295154,1.,0.951056516295154,1.,0.951056516295154,
1.,0.951056516295154,1.,0.951056516295154,1.,0.951056516295154,1.,0.951056516295154,
1.,0.951056516295154,1.,0.951056516295154,1.,0.951056516295154,1.,0.951056516295154,
1.,0.951056516295154,1.,0.951056516295154,1.,0.951056516295154,1.,0.951056516295154,
1.,0.951056516295154,1.,0.951056516295154,1.,0.951056516295154,1.,0.951056516295154,
1.,0.951056516295154,1.,0.951056516295154,1.,0.951056516295154,1.,0.951056516295154,
1.,0.951056516295154,1.,0.951056516295154,1.,0.951056516295154,1.,0.951056516295154,
1.,0.951056516295154,1.,0.951056516295154,1.,0.951056516295154,1.,0.951056516295154,
1.,0.951056516295154,1.,0.951056516295154,1.,0.951056516295154,1.,0.951056516295154,
1.,0.951056516295154,1.,0.951056516295154,1.,0.951056516295154,1.,0.951056516295154,
1.,0.951056516295154,1.,0.951056516295154,1.,0.951056516295154,1.,0.951056516295154,
1.,0.951056516295154,1.,0.951056516295154,1.,0.951056516295154,1.,0.951056516295154,
1.,0.951056516295154,1.,0.951056516295154,1.,0.951056516295154,1.,0.951056516295154,
1.,0.951056516295154,1.,0.951056516295154,1.,0.951056516295154,1.,0.951056516295154,
1.,0.951056516295154,1.,0.951056516295154,1.,0.951056516295154,1.,0.951056516295154,
1.),(1.,0.951056516295154,1.,0.951056516295154,1.,0.951056516295154,1.,
0.951056516295154,1.,0.951056516295154,1.,0.951056516295154,1.,0.951056516295154,
1.,0.951056516295154,1.,0.951056516295154,1.,0.951056516295154,1.,0.951056516295154,
1.,0.951056516295154,1.,0.951056516295154,1.,0.951056516295154,1.,0.951056516295154,
1.,0.951056516295154,1.,0.951056516295154,1.,0.951056516295154,1.,0.951056516295154,
1.,0.951056516295154,1.,0.951056516295154,1.,0.951056516295154,1.,0.951056516295154,
1.,0.951056516295154,1.,0.951056516295154,1.,0.951056516295154,1.,0.951056516295154,
1.,0.951056516295154,1.,0.951056516295154,1.,0.951056516295154,1.,0.951056516295154,
1.,0.951056516295154,1.,0.951056516295154,1.,0.951056516295154,1.,0.951056516295154,
1.,0.951056516295154,1.,0.951056516295154,1.,0.951056516295154,1.,0.951056516295154,
1.,0.951056516295154,1.,0.951056516295154,1.,0.951056516295154,1.,0.951056516295154,
1.,0.951056516295154,1.,0.951056516295154,1.,0.951056516295154,1.,0.951056516295154,
1.,0.951056516295154,1.,0.951056516295154,1.,0.951056516295154,1.,0.951056516295154,
1.,0.951056516295154,1.,0.951056516295154,1.,0.951056516295154,1.,0.951056516295154,
1.,0.951056516295154,1.,0.951056516295154,1.,0.951056516295154,1.,0.951056516295154,
1.,0.951056516295154,1.,0.951056516295154,1.,0.951056516295154,1.,0.951056516295154,
1.,0.951056516295154,1.,0.951056516295154,1.,0.951056516295154,1.,0.951056516295154,
1.,0.951056516295154,1.,0.951056516295154,1.,0.951056516295154,1.,0.951056516295154,
1.,0.951056516295154,1.,0.951056516295154,1.,0.951056516295154,1.,0.951056516295154,
1.,0.951056516295154,1.,0.951056516295154,1.,0.951056516295154,1.,0.951056516295154,
1.,0.951056516295154,1.,0.951056516295154,1.,0.951056516295154,1.,0.951056516295154,
1.,0.951056516295154,1.,0.951056516295154,1.,0.951056516295154,1.,0.951056516295154,
1.,0.951056516295154,1.,0.951056516295154,1.,0.951056516295154,1.,0.951056516295154,
1.,0.951056516295154,1.,0.951056516295154,1.,0.951056516295154,1.,0.951056516295154,
1.,0.951056516295154,1.,0.951056516295154,1.,0.951056516295154,1.,0.951056516295154,
1.,0.951056516295154,1.,0.951056516295154,1.,0.951056516295154,1.,0.951056516295154,
1.,0.951056516295154,1.,0.951056516295154,1.,0.951056516295154,1.,0.951056516295154,
1.,0.951056516295154,1.,0.951056516295154,1.,0.951056516295154,1.,0.951056516295154,
1.,0.951056516295154,1.,0.951056516295154,1.,0.951056516295154,1.,0.951056516295154,
1.,0.951056516295154,1.,0.951056516295154,1.,0.951056516295154,1.,0.951056516295154,
1.,0.951056516295154,1.,0.951056516295154,1.,0.951056516295154,1.,0.951056516295154,
1.,0.951056516295154,1.,0.951056516295154,1.,0.951056516295154,1.,0.951056516295154,
1.,0.951056516295154,1.,0.951056516295154,1.,0.951056516295154,1.,0.951056516295154,
1.,0.951056516295154,1.,0.951056516295154,1.,0.951056516295154,1.,0.951056516295154,
1.,0.951056516295154,1.,0.951056516295154,1.,0.951056516295154,1.,0.951056516295154,
1.,0.951056516295154,1.,0.951056516295154,1.,0.951056516295154,1.,0.951056516295154,
1.,0.951056516295154,1.,0.951056516295154,1.,0.951056516295154,1.,0.951056516295154,
1.,0.951056516295154,1.,0.951056516295154,1.,0.951056516295154,1.,0.951056516295154,
1.,0.951056516295154,1.,0.951056516295154,1.,0.951056516295154,1.,0.951056516295154,
1.,0.951056516295154,1.,0.951056516295154,1.,0.951056516295154,1.,0.951056516295154,
1.,0.951056516295154,1.,0.951056516295154,1.,0.951056516295154,1.,0.951056516295154,
1.,0.951056516295154,1.,0.951056516295154,1.,0.951056516295154,1.,0.951056516295154,
1.,0.951056516295154,1.,0.951056516295154,1.,0.951056516295154,1.,0.951056516295154,
1.,0.951056516295154,1.,0.951056516295154,1.,0.951056516295154,1.,0.951056516295154,
1.,0.951056516295154,1.,0.951056516295154,1.,0.951056516295154,1.,0.951056516295154,
1.,0.951056516295154,1.,0.951056516295154,1.,0.951056516295154,1.,0.951056516295154,
1.,0.951056516295154,1.,0.951056516295154,1.,0.951056516295154,1.,0.951056516295154,
1.,0.951056516295154,1.,0.951056516295154,1.,0.951056516295154,1.,0.951056516295154,
1.,0.951056516295154,1.,0.951056516295154,1.,0.951056516295154,1.,0.951056516295154,
1.,0.951056516295154,1.,0.951056516295154,1.,0.951056516295154,1.,0.951056516295154,
1.,0.951056516295154,1.,0.951056516295154,1.,0.951056516295154,1.,0.951056516295154,
1.,0.951056516295154,1.,0.951056516295154,1.,0.951056516295154,1.,0.951056516295154,
1.,0.951056516295154,1.,0.951056516295154,1.,0.951056516295154,1.,0.951056516295154,
1.,0.951056516295154,1.,0.951056516295154,1.,0.951056516295154,1.,0.951056516295154,
1.,0.951056516295154,1.,0.951056516295154,1.,0.951056516295154,1.,0.951056516295154,
1.,0.951056516295154,1.,0.951056516295154,1.,0.951056516295154,1.,0.951056516295154,
1.,0.951056516295154,1.,0.951056516295154,1.,0.951056516295154,1.,0.951056516295154,
1.,0.951056516295154,1.,0.951056516295154,1.,0.951056516295154,1.,0.951056516295154,
1.,0.951056516295154,1.,0.951056516295154,1.,0.951056516295154,1.,0.951056516295154,
1.,0.951056516295154,1.,0.951056516295154,1.,0.951056516295154,1.,0.951056516295154,
1.,0.951056516295154,1.,0.951056516295154,1.,0.951056516295154,1.,0.951056516295154,
1.,0.951056516295154,1.,0.951056516295154,1.,0.951056516295154,1.,0.951056516295154,
1.,0.951056516295154,1.,0.951056516295154,1.,0.951056516295154,1.,0.951056516295154,
1.,0.951056516295154,1.,0.951056516295154,1.,0.951056516295154,1.,0.951056516295154,
1.,0.951056516295154,1.,0.951056516295154,1.,0.951056516295154,1.,0.951056516295154,
1.,0.951056516295154,1.,0.951056516295154,1.,0.951056516295154,1.,0.951056516295154,
1.,0.951056516295154,1.,0.951056516295154,1.,0.951056516295154,1.,0.951056516295154,
1.,0.951056516295154,1.,0.951056516295154,1.,0.951056516295154,1.,0.951056516295154,
1.,0.951056516295154,1.,0.951056516295154,1.,0.951056516295154,1.,0.951056516295154,
1.,0.951056516295154,1.,0.951056516295154,1.,0.951056516295154,1.,0.951056516295154,
1.,0.951056516295154,1.,0.951056516295154,1.,0.951056516295154,1.,0.951056516295154,
1.,0.951056516295154,1.,0.951056516295154,1.,0.951056516295154,1.,0.951056516295154,
1.,0.951056516295154,1.,0.951056516295154,1.,0.951056516295154,1.,0.951056516295154,
1.,0.951056516295154,1.,0.951056516295154,1.,0.951056516295154,1.,0.951056516295154,
1.,0.951056516295154,1.,0.951056516295154,1.,0.951056516295154,1.,0.951056516295154,
1.,0.951056516295154,1.,0.951056516295154,1.,0.951056516295154,1.,0.951056516295154,
1.,0.951056516295154,1.,0.951056516295154,1.,0.951056516295154,1.,0.951056516295154,
1.,0.951056516295154,1.,0.951056516295154,1.,0.951056516295154,1.,0.951056516295154,
1.,0.951056516295154,1.,0.951056516295154,1.,0.951056516295154,1.,0.951056516295154,
1.,0.951056516295154,1.,0.951056516295154,1.,0.951056516295154,1.,0.951056516295154,
1.,0.951056516295154,1.,0.951056516295154,1.,0.951056516295154,1.,0.951056516295154,
1.,0.951056516295154,1.,0.951056516295154,1.,0.951056516295154,1.,0.951056516295154,
1.,0.951056516295154,1.,0.951056516295154,1.,0.951056516295154,1.,0.951056516295154,
1.,0.951056516295154,1.,0.951056516295154,1.,0.951056516295154,1.,0.951056516295154,
1.,0.951056516295154,1.,0.951056516295154,1.,0.951056516295154,1.,0.951056516295154,
1.,0.951056516295154,1.,0.951056516295154,1.,0.951056516295154,1.,0.951056516295154,
1.,0.951056516295154,1.,0.951056516295154,1.,0.951056516295154,1.,0.951056516295154,
1.,0.951056516295154,1.,0.951056516295154,1.,0.951056516295154,1.,0.951056516295154,
1.,0.951056516295154,1.,0.951056516295154,1.,0.951056516295154,1.,0.951056516295154,
1.,0.951056516295154,1.,0.951056516295154,1.,0.951056516295154,1.,0.951056516295154,
1.,0.951056516295154,1.,0.951056516295154,1.,0.951056516295154,1.,0.951056516295154,
1.,0.951056516295154,1.,0.951056516295154,1.,0.951056516295154,1.,0.951056516295154,
1.,0.951056516295154,1.,0.951056516295154,1.,0.951056516295154,1.,0.951056516295154,
1.,0.951056516295154,1.,0.951056516295154,1.,0.951056516295154,1.,0.951056516295154,
1.,0.951056516295154,1.,0.951056516295154,1.,0.951056516295154,1.,0.951056516295154,
1.,0.951056516295154,1.,0.951056516295154,1.,0.951056516295154,1.,0.951056516295154,
1.,0.951056516295154,1.,0.951056516295154,1.,0.951056516295154,1.,0.951056516295154,
1.,0.951056516295154,1.,0.951056516295154,1.,0.951056516295154,1.,0.951056516295154,
1.,0.951056516295154,1.,0.951056516295154,1.,0.951056516295154,1.,0.951056516295154,
1.,0.951056516295154,1.,0.951056516295154,1.,0.951056516295154,1.,0.951056516295154,
1.,0.951056516295154,1.,0.951056516295154,1.,0.951056516295154,1.,0.951056516295154,
1.,0.951056516295154,1.,0.951056516295154,1.,0.951056516295154,1.,0.951056516295154,
1.,0.951056516295154,1.,0.951056516295154,1.,0.951056516295154,1.,0.951056516295154,
1.,0.951056516295154,1.,0.951056516295154,1.,0.951056516295154,1.,0.951056516295154,
1.,0.951056516295154,1.,0.951056516295154,1.,0.951056516295154,1.,0.951056516295154,
1.,0.951056516295154,1.,0.951056516295154,1.,0.951056516295154,1.,0.951056516295154,
1.,0.951056516295154,1.,0.951056516295154,1.,0.951056516295154,1.,0.951056516295154,
1.,0.951056516295154,1.,0.951056516295154,1.,0.951056516295154,1.,0.951056516295154,
1.,0.951056516295154,1.,0.951056516295154,1.,0.951056516295154,1.,0.951056516295154,
1.,0.951056516295154,1.,0.951056516295154,1.,0.951056516295154,1.,0.951056516295154,
1.,0.951056516295154,1.,0.951056516295154,1.,0.951056516295154,1.,0.951056516295154,
1.,0.951056516295154,1.,0.951056516295154,1.,0.951056516295154,1.,0.951056516295154,
1.,0.951056516295154,1.,0.951056516295154,1.,0.951056516295154,1.,0.951056516295154,
1.,0.951056516295154,1.,0.951056516295154,1.,0.951056516295154,1.,0.951056516295154,
1.,0.951056516295154,1.,0.951056516295154,1.,0.951056516295154,1.,0.951056516295154,
1.,0.951056516295154,1.,0.951056516295154,1.,0.951056516295154,1.,0.951056516295154,
1.,0.951056516295154,1.,0.951056516295154,1.,0.951056516295154,1.,0.951056516295154,
1.,0.951056516295154,1.,0.951056516295154,1.,0.951056516295154,1.,0.951056516295154,
1.,0.951056516295154,1.,0.951056516295154,1.,0.951056516295154,1.,0.951056516295154,
1.,0.951056516295154,1.,0.951056516295154,1.,0.951056516295154,1.,0.951056516295154,
1.,0.951056516295154,1.,0.951056516295154,1.,0.951056516295154,1.,0.951056516295154,
1.,0.951056516295154,1.,0.951056516295154,1.,0.951056516295154,1.,0.951056516295154,
1.,0.951056516295154,1.,0.951056516295154,1.,0.951056516295154,1.,0.951056516295154,
1.,0.951056516295154,1.,0.951056516295154,1.,0.951056516295154,1.,0.951056516295154,
1.,0.951056516295154,1.,0.951056516295154,1.,0.951056516295154,1.,0.951056516295154,
1.,0.951056516295154,1.,0.951056516295154,1.,0.951056516295154,1.,0.951056516295154,
1.,0.951056516295154,1.,0.951056516295154,1.,0.951056516295154,1.,0.951056516295154,
1.,0.951056516295154,1.,0.951056516295154,1.,0.951056516295154,1.,0.951056516295154,
1.,0.951056516295154,1.,0.951056516295154,1.,0.951056516295154,1.,0.951056516295154,
1.,0.951056516295154,1.,0.951056516295154,1.,0.951056516295154,1.)))
REPRESENTATION_ITEM('')
SURFACE()
);
#3196=(
BOUNDED_SURFACE()
B_SPLINE_SURFACE(1,2,((#285828,#285829,#285830,#285831,#285832,#285833,
#285834,#285835,#285836,#285837,#285838,#285839,#285840,#285841,#285842,
#285843,#285844,#285845,#285846,#285847,#285848,#285849,#285850,#285851,
#285852,#285853,#285854,#285855,#285856,#285857,#285858,#285859,#285860,
#285861,#285862,#285863,#285864,#285865,#285866,#285867,#285868,#285869,
#285870,#285871,#285872,#285873,#285874,#285875,#285876,#285877,#285878,
#285879,#285880,#285881,#285882,#285883,#285884,#285885,#285886,#285887,
#285888,#285889,#285890,#285891,#285892,#285893,#285894,#285895,#285896,
#285897,#285898,#285899,#285900,#285901,#285902,#285903,#285904,#285905,
#285906,#285907,#285908,#285909,#285910,#285911,#285912,#285913,#285914,
#285915,#285916,#285917,#285918,#285919,#285920,#285921,#285922,#285923,
#285924,#285925,#285926,#285927,#285928,#285929,#285930,#285931,#285932,
#285933,#285934,#285935,#285936,#285937,#285938,#285939,#285940,#285941,
#285942,#285943,#285944,#285945,#285946,#285947,#285948,#285949,#285950,
#285951,#285952,#285953,#285954,#285955,#285956,#285957,#285958,#285959,
#285960,#285961,#285962,#285963,#285964,#285965,#285966,#285967,#285968,
#285969,#285970,#285971,#285972,#285973,#285974,#285975,#285976,#285977,
#285978,#285979,#285980,#285981,#285982,#285983,#285984,#285985,#285986,
#285987,#285988,#285989,#285990,#285991,#285992,#285993,#285994,#285995,
#285996,#285997,#285998,#285999,#286000,#286001,#286002,#286003,#286004,
#286005,#286006,#286007,#286008,#286009,#286010,#286011,#286012,#286013,
#286014,#286015,#286016,#286017,#286018,#286019,#286020,#286021,#286022,
#286023,#286024,#286025,#286026,#286027,#286028,#286029,#286030,#286031,
#286032,#286033,#286034,#286035,#286036,#286037,#286038,#286039,#286040,
#286041,#286042,#286043,#286044,#286045,#286046,#286047,#286048,#286049,
#286050,#286051,#286052,#286053,#286054,#286055,#286056,#286057,#286058,
#286059,#286060,#286061,#286062,#286063,#286064,#286065,#286066,#286067,
#286068,#286069,#286070,#286071,#286072,#286073,#286074,#286075,#286076,
#286077,#286078,#286079,#286080,#286081,#286082,#286083,#286084,#286085,
#286086,#286087,#286088,#286089,#286090,#286091,#286092,#286093,#286094,
#286095,#286096,#286097,#286098,#286099,#286100,#286101,#286102,#286103,
#286104,#286105,#286106,#286107,#286108,#286109,#286110,#286111,#286112,
#286113,#286114,#286115,#286116,#286117,#286118,#286119,#286120,#286121,
#286122,#286123,#286124,#286125,#286126,#286127,#286128,#286129,#286130,
#286131,#286132,#286133,#286134,#286135,#286136,#286137,#286138,#286139,
#286140,#286141,#286142,#286143,#286144,#286145,#286146,#286147,#286148,
#286149,#286150,#286151,#286152,#286153,#286154,#286155,#286156,#286157,
#286158,#286159,#286160,#286161,#286162,#286163,#286164,#286165,#286166,
#286167,#286168,#286169,#286170,#286171,#286172,#286173,#286174,#286175,
#286176,#286177,#286178,#286179,#286180,#286181,#286182,#286183,#286184,
#286185,#286186,#286187,#286188,#286189,#286190,#286191,#286192,#286193,
#286194,#286195,#286196,#286197,#286198,#286199,#286200,#286201,#286202,
#286203,#286204,#286205,#286206,#286207,#286208,#286209,#286210,#286211,
#286212,#286213,#286214,#286215,#286216,#286217,#286218,#286219,#286220,
#286221,#286222,#286223,#286224,#286225,#286226,#286227,#286228,#286229,
#286230,#286231,#286232,#286233,#286234,#286235,#286236,#286237,#286238,
#286239,#286240,#286241,#286242,#286243,#286244,#286245,#286246,#286247,
#286248,#286249,#286250,#286251,#286252,#286253,#286254,#286255,#286256,
#286257,#286258,#286259,#286260,#286261,#286262,#286263,#286264,#286265,
#286266,#286267,#286268,#286269,#286270,#286271,#286272,#286273,#286274,
#286275,#286276,#286277,#286278,#286279,#286280,#286281,#286282,#286283,
#286284,#286285,#286286,#286287,#286288,#286289,#286290,#286291,#286292,
#286293,#286294,#286295,#286296,#286297,#286298,#286299,#286300,#286301,
#286302,#286303,#286304,#286305,#286306,#286307,#286308,#286309,#286310,
#286311,#286312,#286313,#286314,#286315,#286316,#286317,#286318,#286319,
#286320,#286321,#286322,#286323,#286324,#286325,#286326,#286327,#286328,
#286329,#286330,#286331,#286332,#286333,#286334,#286335,#286336,#286337,
#286338,#286339,#286340,#286341,#286342,#286343,#286344,#286345,#286346,
#286347,#286348,#286349,#286350,#286351,#286352,#286353,#286354,#286355,
#286356,#286357,#286358,#286359,#286360,#286361,#286362,#286363,#286364,
#286365,#286366,#286367,#286368,#286369,#286370,#286371,#286372,#286373,
#286374,#286375,#286376,#286377,#286378,#286379,#286380,#286381,#286382,
#286383,#286384,#286385,#286386,#286387,#286388,#286389,#286390,#286391,
#286392,#286393,#286394,#286395,#286396,#286397,#286398,#286399,#286400,
#286401,#286402,#286403,#286404,#286405,#286406,#286407,#286408,#286409,
#286410,#286411,#286412,#286413,#286414,#286415,#286416,#286417,#286418,
#286419,#286420,#286421,#286422,#286423,#286424,#286425,#286426,#286427,
#286428,#286429,#286430,#286431,#286432,#286433,#286434,#286435,#286436,
#286437,#286438,#286439,#286440,#286441,#286442,#286443,#286444,#286445,
#286446,#286447,#286448,#286449,#286450,#286451,#286452,#286453,#286454,
#286455,#286456,#286457,#286458,#286459,#286460,#286461,#286462,#286463,
#286464,#286465,#286466,#286467,#286468,#286469,#286470,#286471,#286472,
#286473,#286474,#286475,#286476,#286477,#286478,#286479,#286480,#286481,
#286482,#286483,#286484,#286485,#286486,#286487,#286488,#286489,#286490,
#286491,#286492,#286493,#286494,#286495,#286496,#286497,#286498,#286499,
#286500,#286501,#286502,#286503,#286504,#286505,#286506,#286507,#286508,
#286509,#286510,#286511,#286512,#286513,#286514,#286515,#286516,#286517,
#286518,#286519,#286520,#286521,#286522,#286523,#286524,#286525,#286526,
#286527,#286528,#286529,#286530,#286531,#286532,#286533,#286534,#286535,
#286536,#286537,#286538,#286539,#286540,#286541,#286542,#286543,#286544,
#286545,#286546,#286547,#286548,#286549,#286550,#286551,#286552,#286553,
#286554,#286555,#286556,#286557,#286558,#286559,#286560,#286561,#286562,
#286563,#286564,#286565,#286566,#286567,#286568,#286569,#286570,#286571,
#286572,#286573,#286574,#286575,#286576,#286577,#286578,#286579,#286580,
#286581,#286582,#286583,#286584,#286585,#286586,#286587,#286588,#286589,
#286590,#286591,#286592,#286593,#286594,#286595,#286596,#286597,#286598,
#286599,#286600,#286601,#286602,#286603,#286604,#286605,#286606,#286607,
#286608,#286609,#286610,#286611,#286612,#286613,#286614,#286615,#286616,
#286617,#286618,#286619,#286620,#286621,#286622,#286623,#286624,#286625,
#286626,#286627,#286628,#286629,#286630,#286631,#286632,#286633,#286634,
#286635,#286636,#286637,#286638,#286639,#286640,#286641,#286642,#286643,
#286644,#286645,#286646,#286647,#286648,#286649,#286650,#286651,#286652,
#286653,#286654,#286655,#286656,#286657,#286658,#286659,#286660,#286661,
#286662,#286663,#286664,#286665,#286666,#286667,#286668,#286669,#286670,
#286671,#286672,#286673,#286674,#286675,#286676,#286677,#286678,#286679,
#286680,#286681,#286682,#286683,#286684,#286685,#286686,#286687,#286688,
#286689,#286690,#286691,#286692,#286693,#286694,#286695,#286696,#286697,
#286698,#286699,#286700,#286701,#286702,#286703,#286704,#286705,#286706,
#286707,#286708,#286709,#286710,#286711,#286712,#286713,#286714,#286715,
#286716,#286717,#286718,#286719,#286720,#286721,#286722,#286723,#286724,
#286725,#286726,#286727,#286728,#286729,#286730,#286731,#286732,#286733,
#286734,#286735,#286736,#286737,#286738,#286739,#286740,#286741,#286742,
#286743,#286744,#286745,#286746,#286747,#286748,#286749,#286750,#286751,
#286752,#286753,#286754,#286755,#286756,#286757,#286758,#286759,#286760,
#286761,#286762,#286763,#286764,#286765,#286766,#286767,#286768,#286769,
#286770,#286771,#286772,#286773,#286774,#286775,#286776,#286777,#286778,
#286779,#286780,#286781,#286782,#286783,#286784,#286785,#286786,#286787,
#286788,#286789,#286790,#286791,#286792,#286793,#286794,#286795,#286796,
#286797,#286798,#286799,#286800,#286801,#286802,#286803,#286804,#286805,
#286806,#286807,#286808,#286809,#286810,#286811,#286812,#286813,#286814,
#286815,#286816,#286817,#286818,#286819,#286820,#286821,#286822,#286823,
#286824,#286825,#286826,#286827,#286828,#286829,#286830,#286831,#286832,
#286833,#286834,#286835,#286836,#286837,#286838,#286839,#286840,#286841,
#286842,#286843,#286844,#286845,#286846,#286847,#286848,#286849,#286850,
#286851,#286852,#286853,#286854,#286855,#286856,#286857,#286858,#286859,
#286860,#286861,#286862,#286863,#286864),(#286865,#286866,#286867,#286868,
#286869,#286870,#286871,#286872,#286873,#286874,#286875,#286876,#286877,
#286878,#286879,#286880,#286881,#286882,#286883,#286884,#286885,#286886,
#286887,#286888,#286889,#286890,#286891,#286892,#286893,#286894,#286895,
#286896,#286897,#286898,#286899,#286900,#286901,#286902,#286903,#286904,
#286905,#286906,#286907,#286908,#286909,#286910,#286911,#286912,#286913,
#286914,#286915,#286916,#286917,#286918,#286919,#286920,#286921,#286922,
#286923,#286924,#286925,#286926,#286927,#286928,#286929,#286930,#286931,
#286932,#286933,#286934,#286935,#286936,#286937,#286938,#286939,#286940,
#286941,#286942,#286943,#286944,#286945,#286946,#286947,#286948,#286949,
#286950,#286951,#286952,#286953,#286954,#286955,#286956,#286957,#286958,
#286959,#286960,#286961,#286962,#286963,#286964,#286965,#286966,#286967,
#286968,#286969,#286970,#286971,#286972,#286973,#286974,#286975,#286976,
#286977,#286978,#286979,#286980,#286981,#286982,#286983,#286984,#286985,
#286986,#286987,#286988,#286989,#286990,#286991,#286992,#286993,#286994,
#286995,#286996,#286997,#286998,#286999,#287000,#287001,#287002,#287003,
#287004,#287005,#287006,#287007,#287008,#287009,#287010,#287011,#287012,
#287013,#287014,#287015,#287016,#287017,#287018,#287019,#287020,#287021,
#287022,#287023,#287024,#287025,#287026,#287027,#287028,#287029,#287030,
#287031,#287032,#287033,#287034,#287035,#287036,#287037,#287038,#287039,
#287040,#287041,#287042,#287043,#287044,#287045,#287046,#287047,#287048,
#287049,#287050,#287051,#287052,#287053,#287054,#287055,#287056,#287057,
#287058,#287059,#287060,#287061,#287062,#287063,#287064,#287065,#287066,
#287067,#287068,#287069,#287070,#287071,#287072,#287073,#287074,#287075,
#287076,#287077,#287078,#287079,#287080,#287081,#287082,#287083,#287084,
#287085,#287086,#287087,#287088,#287089,#287090,#287091,#287092,#287093,
#287094,#287095,#287096,#287097,#287098,#287099,#287100,#287101,#287102,
#287103,#287104,#287105,#287106,#287107,#287108,#287109,#287110,#287111,
#287112,#287113,#287114,#287115,#287116,#287117,#287118,#287119,#287120,
#287121,#287122,#287123,#287124,#287125,#287126,#287127,#287128,#287129,
#287130,#287131,#287132,#287133,#287134,#287135,#287136,#287137,#287138,
#287139,#287140,#287141,#287142,#287143,#287144,#287145,#287146,#287147,
#287148,#287149,#287150,#287151,#287152,#287153,#287154,#287155,#287156,
#287157,#287158,#287159,#287160,#287161,#287162,#287163,#287164,#287165,
#287166,#287167,#287168,#287169,#287170,#287171,#287172,#287173,#287174,
#287175,#287176,#287177,#287178,#287179,#287180,#287181,#287182,#287183,
#287184,#287185,#287186,#287187,#287188,#287189,#287190,#287191,#287192,
#287193,#287194,#287195,#287196,#287197,#287198,#287199,#287200,#287201,
#287202,#287203,#287204,#287205,#287206,#287207,#287208,#287209,#287210,
#287211,#287212,#287213,#287214,#287215,#287216,#287217,#287218,#287219,
#287220,#287221,#287222,#287223,#287224,#287225,#287226,#287227,#287228,
#287229,#287230,#287231,#287232,#287233,#287234,#287235,#287236,#287237,
#287238,#287239,#287240,#287241,#287242,#287243,#287244,#287245,#287246,
#287247,#287248,#287249,#287250,#287251,#287252,#287253,#287254,#287255,
#287256,#287257,#287258,#287259,#287260,#287261,#287262,#287263,#287264,
#287265,#287266,#287267,#287268,#287269,#287270,#287271,#287272,#287273,
#287274,#287275,#287276,#287277,#287278,#287279,#287280,#287281,#287282,
#287283,#287284,#287285,#287286,#287287,#287288,#287289,#287290,#287291,
#287292,#287293,#287294,#287295,#287296,#287297,#287298,#287299,#287300,
#287301,#287302,#287303,#287304,#287305,#287306,#287307,#287308,#287309,
#287310,#287311,#287312,#287313,#287314,#287315,#287316,#287317,#287318,
#287319,#287320,#287321,#287322,#287323,#287324,#287325,#287326,#287327,
#287328,#287329,#287330,#287331,#287332,#287333,#287334,#287335,#287336,
#287337,#287338,#287339,#287340,#287341,#287342,#287343,#287344,#287345,
#287346,#287347,#287348,#287349,#287350,#287351,#287352,#287353,#287354,
#287355,#287356,#287357,#287358,#287359,#287360,#287361,#287362,#287363,
#287364,#287365,#287366,#287367,#287368,#287369,#287370,#287371,#287372,
#287373,#287374,#287375,#287376,#287377,#287378,#287379,#287380,#287381,
#287382,#287383,#287384,#287385,#287386,#287387,#287388,#287389,#287390,
#287391,#287392,#287393,#287394,#287395,#287396,#287397,#287398,#287399,
#287400,#287401,#287402,#287403,#287404,#287405,#287406,#287407,#287408,
#287409,#287410,#287411,#287412,#287413,#287414,#287415,#287416,#287417,
#287418,#287419,#287420,#287421,#287422,#287423,#287424,#287425,#287426,
#287427,#287428,#287429,#287430,#287431,#287432,#287433,#287434,#287435,
#287436,#287437,#287438,#287439,#287440,#287441,#287442,#287443,#287444,
#287445,#287446,#287447,#287448,#287449,#287450,#287451,#287452,#287453,
#287454,#287455,#287456,#287457,#287458,#287459,#287460,#287461,#287462,
#287463,#287464,#287465,#287466,#287467,#287468,#287469,#287470,#287471,
#287472,#287473,#287474,#287475,#287476,#287477,#287478,#287479,#287480,
#287481,#287482,#287483,#287484,#287485,#287486,#287487,#287488,#287489,
#287490,#287491,#287492,#287493,#287494,#287495,#287496,#287497,#287498,
#287499,#287500,#287501,#287502,#287503,#287504,#287505,#287506,#287507,
#287508,#287509,#287510,#287511,#287512,#287513,#287514,#287515,#287516,
#287517,#287518,#287519,#287520,#287521,#287522,#287523,#287524,#287525,
#287526,#287527,#287528,#287529,#287530,#287531,#287532,#287533,#287534,
#287535,#287536,#287537,#287538,#287539,#287540,#287541,#287542,#287543,
#287544,#287545,#287546,#287547,#287548,#287549,#287550,#287551,#287552,
#287553,#287554,#287555,#287556,#287557,#287558,#287559,#287560,#287561,
#287562,#287563,#287564,#287565,#287566,#287567,#287568,#287569,#287570,
#287571,#287572,#287573,#287574,#287575,#287576,#287577,#287578,#287579,
#287580,#287581,#287582,#287583,#287584,#287585,#287586,#287587,#287588,
#287589,#287590,#287591,#287592,#287593,#287594,#287595,#287596,#287597,
#287598,#287599,#287600,#287601,#287602,#287603,#287604,#287605,#287606,
#287607,#287608,#287609,#287610,#287611,#287612,#287613,#287614,#287615,
#287616,#287617,#287618,#287619,#287620,#287621,#287622,#287623,#287624,
#287625,#287626,#287627,#287628,#287629,#287630,#287631,#287632,#287633,
#287634,#287635,#287636,#287637,#287638,#287639,#287640,#287641,#287642,
#287643,#287644,#287645,#287646,#287647,#287648,#287649,#287650,#287651,
#287652,#287653,#287654,#287655,#287656,#287657,#287658,#287659,#287660,
#287661,#287662,#287663,#287664,#287665,#287666,#287667,#287668,#287669,
#287670,#287671,#287672,#287673,#287674,#287675,#287676,#287677,#287678,
#287679,#287680,#287681,#287682,#287683,#287684,#287685,#287686,#287687,
#287688,#287689,#287690,#287691,#287692,#287693,#287694,#287695,#287696,
#287697,#287698,#287699,#287700,#287701,#287702,#287703,#287704,#287705,
#287706,#287707,#287708,#287709,#287710,#287711,#287712,#287713,#287714,
#287715,#287716,#287717,#287718,#287719,#287720,#287721,#287722,#287723,
#287724,#287725,#287726,#287727,#287728,#287729,#287730,#287731,#287732,
#287733,#287734,#287735,#287736,#287737,#287738,#287739,#287740,#287741,
#287742,#287743,#287744,#287745,#287746,#287747,#287748,#287749,#287750,
#287751,#287752,#287753,#287754,#287755,#287756,#287757,#287758,#287759,
#287760,#287761,#287762,#287763,#287764,#287765,#287766,#287767,#287768,
#287769,#287770,#287771,#287772,#287773,#287774,#287775,#287776,#287777,
#287778,#287779,#287780,#287781,#287782,#287783,#287784,#287785,#287786,
#287787,#287788,#287789,#287790,#287791,#287792,#287793,#287794,#287795,
#287796,#287797,#287798,#287799,#287800,#287801,#287802,#287803,#287804,
#287805,#287806,#287807,#287808,#287809,#287810,#287811,#287812,#287813,
#287814,#287815,#287816,#287817,#287818,#287819,#287820,#287821,#287822,
#287823,#287824,#287825,#287826,#287827,#287828,#287829,#287830,#287831,
#287832,#287833,#287834,#287835,#287836,#287837,#287838,#287839,#287840,
#287841,#287842,#287843,#287844,#287845,#287846,#287847,#287848,#287849,
#287850,#287851,#287852,#287853,#287854,#287855,#287856,#287857,#287858,
#287859,#287860,#287861,#287862,#287863,#287864,#287865,#287866,#287867,
#287868,#287869,#287870,#287871,#287872,#287873,#287874,#287875,#287876,
#287877,#287878,#287879,#287880,#287881,#287882,#287883,#287884,#287885,
#287886,#287887,#287888,#287889,#287890,#287891,#287892,#287893,#287894,
#287895,#287896,#287897,#287898,#287899,#287900,#287901)),.UNSPECIFIED.,
 .F.,.F.,.F.)
B_SPLINE_SURFACE_WITH_KNOTS((2,2),(3,2,2,2,2,2,2,2,2,2,2,2,2,2,2,2,2,2,
2,2,2,2,2,2,2,2,2,2,2,2,2,2,2,2,2,2,2,2,2,2,2,2,2,2,2,2,2,2,2,2,2,2,2,2,
2,2,2,2,2,2,2,2,2,2,2,2,2,2,2,2,2,2,2,2,2,2,2,2,2,2,2,2,2,2,2,2,2,2,2,2,
2,2,2,2,2,2,2,2,2,2,2,2,2,2,2,2,2,2,2,2,2,2,2,2,2,2,2,2,2,2,2,2,2,2,2,2,
2,2,2,2,2,2,2,2,2,2,2,2,2,2,2,2,2,2,2,2,2,2,2,2,2,2,2,2,2,2,2,2,2,2,2,2,
2,2,2,2,2,2,2,2,2,2,2,2,2,2,2,2,2,2,2,2,2,2,2,2,2,2,2,2,2,2,2,2,2,2,2,2,
2,2,2,2,2,2,2,2,2,2,2,2,2,2,2,2,2,2,2,2,2,2,2,2,2,2,2,2,2,2,2,2,2,2,2,2,
2,2,2,2,2,2,2,2,2,2,2,2,2,2,2,2,2,2,2,2,2,2,2,2,2,2,2,2,2,2,2,2,2,2,2,2,
2,2,2,2,2,2,2,2,2,2,2,2,2,2,2,2,2,2,2,2,2,2,2,2,2,2,2,2,2,2,2,2,2,2,2,2,
2,2,2,2,2,2,2,2,2,2,2,2,2,2,2,2,2,2,2,2,2,2,2,2,2,2,2,2,2,2,2,2,2,2,2,2,
2,2,2,2,2,2,2,2,2,2,2,2,2,2,2,2,2,2,2,2,2,2,2,2,2,2,2,2,2,2,2,2,2,2,2,2,
2,2,2,2,2,2,2,2,2,2,2,2,2,2,2,2,2,2,2,2,2,2,2,2,2,2,2,2,2,2,2,2,2,2,2,2,
2,2,2,2,2,2,2,2,2,2,2,2,2,2,2,2,2,2,2,2,2,2,2,2,2,2,2,2,2,2,2,2,2,2,2,2,
2,2,2,2,2,2,2,2,2,2,2,2,2,2,2,2,2,2,2,2,2,2,2,2,2,2,2,2,2,2,2,2,2,2,2,2,
2,2,2,2,2,2,2,2,2,2,2,2,2,2,2,2,2,2,2,2,2,2,2,2,2,2,2,2,2,2,2,2,3),(0.,
1.),(0.,0.00192307692307692,0.00384615384615385,0.00576923076923077,0.00769230769230769,
0.00961538461538462,0.0115384615384615,0.0134615384615385,0.0153846153846154,
0.0173076923076923,0.0192307692307692,0.0211538461538462,0.0230769230769231,
0.025,0.0269230769230769,0.0288461538461538,0.0307692307692308,0.0326923076923077,
0.0346153846153846,0.0365384615384615,0.0384615384615385,0.0403846153846154,
0.0423076923076923,0.0442307692307692,0.0461538461538462,0.0480769230769231,
0.05,0.0519230769230769,0.0538461538461538,0.0557692307692308,0.0576923076923077,
0.0596153846153846,0.0615384615384615,0.0634615384615385,0.0653846153846154,
0.0673076923076923,0.0692307692307692,0.0711538461538462,0.0730769230769231,
0.075,0.0769230769230769,0.0788461538461538,0.0807692307692308,0.0826923076923077,
0.0846153846153846,0.0865384615384615,0.0884615384615385,0.0903846153846154,
0.0923076923076923,0.0942307692307692,0.0961538461538462,0.0980769230769231,
0.1,0.101923076923077,0.103846153846154,0.105769230769231,0.107692307692308,
0.109615384615385,0.111538461538462,0.113461538461538,0.115384615384615,
0.117307692307692,0.119230769230769,0.121153846153846,0.123076923076923,
0.125,0.126923076923077,0.128846153846154,0.130769230769231,0.132692307692308,
0.134615384615385,0.136538461538462,0.138461538461538,0.140384615384615,
0.142307692307692,0.144230769230769,0.146153846153846,0.148076923076923,
0.15,0.151923076923077,0.153846153846154,0.155769230769231,0.157692307692308,
0.159615384615385,0.161538461538462,0.163461538461538,0.165384615384615,
0.167307692307692,0.169230769230769,0.171153846153846,0.173076923076923,
0.175,0.176923076923077,0.178846153846154,0.180769230769231,0.182692307692308,
0.184615384615385,0.186538461538462,0.188461538461538,0.190384615384615,
0.192307692307692,0.194230769230769,0.196153846153846,0.198076923076923,
0.2,0.201923076923077,0.203846153846154,0.205769230769231,0.207692307692308,
0.209615384615385,0.211538461538462,0.213461538461538,0.215384615384615,
0.217307692307692,0.219230769230769,0.221153846153846,0.223076923076923,
0.225,0.226923076923077,0.228846153846154,0.230769230769231,0.232692307692308,
0.234615384615385,0.236538461538462,0.238461538461538,0.240384615384615,
0.242307692307692,0.244230769230769,0.246153846153846,0.248076923076923,
0.25,0.251923076923077,0.253846153846154,0.255769230769231,0.257692307692308,
0.259615384615385,0.261538461538462,0.263461538461538,0.265384615384615,
0.267307692307692,0.269230769230769,0.271153846153846,0.273076923076923,
0.275,0.276923076923077,0.278846153846154,0.280769230769231,0.282692307692308,
0.284615384615385,0.286538461538462,0.288461538461538,0.290384615384615,
0.292307692307692,0.294230769230769,0.296153846153846,0.298076923076923,
0.3,0.301923076923077,0.303846153846154,0.305769230769231,0.307692307692308,
0.309615384615385,0.311538461538462,0.313461538461538,0.315384615384615,
0.317307692307692,0.319230769230769,0.321153846153846,0.323076923076923,
0.325,0.326923076923077,0.328846153846154,0.330769230769231,0.332692307692308,
0.334615384615385,0.336538461538462,0.338461538461538,0.340384615384615,
0.342307692307692,0.344230769230769,0.346153846153846,0.348076923076923,
0.35,0.351923076923077,0.353846153846154,0.355769230769231,0.357692307692308,
0.359615384615385,0.361538461538462,0.363461538461538,0.365384615384615,
0.367307692307692,0.369230769230769,0.371153846153846,0.373076923076923,
0.375,0.376923076923077,0.378846153846154,0.380769230769231,0.382692307692308,
0.384615384615385,0.386538461538462,0.388461538461538,0.390384615384615,
0.392307692307692,0.394230769230769,0.396153846153846,0.398076923076923,
0.4,0.401923076923077,0.403846153846154,0.405769230769231,0.407692307692308,
0.409615384615385,0.411538461538462,0.413461538461538,0.415384615384615,
0.417307692307692,0.419230769230769,0.421153846153846,0.423076923076923,
0.425,0.426923076923077,0.428846153846154,0.430769230769231,0.432692307692308,
0.434615384615385,0.436538461538462,0.438461538461538,0.440384615384615,
0.442307692307692,0.444230769230769,0.446153846153846,0.448076923076923,
0.45,0.451923076923077,0.453846153846154,0.455769230769231,0.457692307692308,
0.459615384615385,0.461538461538462,0.463461538461538,0.465384615384615,
0.467307692307692,0.469230769230769,0.471153846153846,0.473076923076923,
0.475,0.476923076923077,0.478846153846154,0.480769230769231,0.482692307692308,
0.484615384615385,0.486538461538462,0.488461538461538,0.490384615384615,
0.492307692307692,0.494230769230769,0.496153846153846,0.498076923076923,
0.5,0.501923076923077,0.503846153846154,0.505769230769231,0.507692307692308,
0.509615384615385,0.511538461538461,0.513461538461538,0.515384615384615,
0.517307692307692,0.519230769230769,0.521153846153846,0.523076923076923,
0.525,0.526923076923077,0.528846153846154,0.530769230769231,0.532692307692308,
0.534615384615385,0.536538461538462,0.538461538461538,0.540384615384615,
0.542307692307692,0.544230769230769,0.546153846153846,0.548076923076923,
0.55,0.551923076923077,0.553846153846154,0.555769230769231,0.557692307692308,
0.559615384615385,0.561538461538462,0.563461538461538,0.565384615384615,
0.567307692307692,0.569230769230769,0.571153846153846,0.573076923076923,
0.575,0.576923076923077,0.578846153846154,0.580769230769231,0.582692307692308,
0.584615384615385,0.586538461538462,0.588461538461538,0.590384615384615,
0.592307692307692,0.594230769230769,0.596153846153846,0.598076923076923,
0.6,0.601923076923077,0.603846153846154,0.605769230769231,0.607692307692308,
0.609615384615385,0.611538461538462,0.613461538461539,0.615384615384615,
0.617307692307692,0.619230769230769,0.621153846153846,0.623076923076923,
0.625,0.626923076923077,0.628846153846154,0.630769230769231,0.632692307692308,
0.634615384615385,0.636538461538461,0.638461538461538,0.640384615384615,
0.642307692307692,0.644230769230769,0.646153846153846,0.648076923076923,
0.65,0.651923076923077,0.653846153846154,0.655769230769231,0.657692307692308,
0.659615384615385,0.661538461538462,0.663461538461538,0.665384615384615,
0.667307692307692,0.669230769230769,0.671153846153846,0.673076923076923,
0.675,0.676923076923077,0.678846153846154,0.680769230769231,0.682692307692308,
0.684615384615385,0.686538461538462,0.688461538461538,0.690384615384615,
0.692307692307692,0.694230769230769,0.696153846153846,0.698076923076923,
0.7,0.701923076923077,0.703846153846154,0.705769230769231,0.707692307692308,
0.709615384615385,0.711538461538462,0.713461538461538,0.715384615384615,
0.717307692307692,0.719230769230769,0.721153846153846,0.723076923076923,
0.725,0.726923076923077,0.728846153846154,0.730769230769231,0.732692307692308,
0.734615384615385,0.736538461538462,0.738461538461539,0.740384615384615,
0.742307692307692,0.744230769230769,0.746153846153846,0.748076923076923,
0.75,0.751923076923077,0.753846153846154,0.755769230769231,0.757692307692308,
0.759615384615385,0.761538461538461,0.763461538461538,0.765384615384615,
0.767307692307692,0.769230769230769,0.771153846153846,0.773076923076923,
0.775,0.776923076923077,0.778846153846154,0.780769230769231,0.782692307692308,
0.784615384615385,0.786538461538462,0.788461538461538,0.790384615384615,
0.792307692307692,0.794230769230769,0.796153846153846,0.798076923076923,
0.8,0.801923076923077,0.803846153846154,0.805769230769231,0.807692307692308,
0.809615384615385,0.811538461538462,0.813461538461538,0.815384615384615,
0.817307692307692,0.819230769230769,0.821153846153846,0.823076923076923,
0.825,0.826923076923077,0.828846153846154,0.830769230769231,0.832692307692308,
0.834615384615385,0.836538461538462,0.838461538461538,0.840384615384615,
0.842307692307692,0.844230769230769,0.846153846153846,0.848076923076923,
0.85,0.851923076923077,0.853846153846154,0.855769230769231,0.857692307692308,
0.859615384615385,0.861538461538462,0.863461538461539,0.865384615384615,
0.867307692307692,0.869230769230769,0.871153846153846,0.873076923076923,
0.875,0.876923076923077,0.878846153846154,0.880769230769231,0.882692307692308,
0.884615384615385,0.886538461538461,0.888461538461538,0.890384615384615,
0.892307692307692,0.894230769230769,0.896153846153846,0.898076923076923,
0.9,0.901923076923077,0.903846153846154,0.905769230769231,0.907692307692308,
0.909615384615385,0.911538461538462,0.913461538461538,0.915384615384615,
0.917307692307692,0.919230769230769,0.921153846153846,0.923076923076923,
0.925,0.926923076923077,0.928846153846154,0.930769230769231,0.932692307692308,
0.934615384615385,0.936538461538462,0.938461538461538,0.940384615384615,
0.942307692307692,0.944230769230769,0.946153846153846,0.948076923076923,
0.95,0.951923076923077,0.953846153846154,0.955769230769231,0.957692307692308,
0.959615384615385,0.961538461538462,0.963461538461538,0.965384615384615,
0.967307692307692,0.969230769230769,0.971153846153846,0.973076923076923,
0.975,0.976923076923077,0.978846153846154,0.980769230769231,0.982692307692308,
0.984615384615385,0.986538461538462,0.988461538461539,0.990384615384615,
0.992307692307692,0.994230769230769,0.996153846153846),.UNSPECIFIED.)
GEOMETRIC_REPRESENTATION_ITEM()
RATIONAL_B_SPLINE_SURFACE(((1.,0.951056516295154,1.,0.951056516295154,1.,
0.951056516295154,1.,0.951056516295154,1.,0.951056516295154,1.,0.951056516295154,
1.,0.951056516295154,1.,0.951056516295154,1.,0.951056516295154,1.,0.951056516295154,
1.,0.951056516295154,1.,0.951056516295154,1.,0.951056516295154,1.,0.951056516295154,
1.,0.951056516295154,1.,0.951056516295154,1.,0.951056516295154,1.,0.951056516295154,
1.,0.951056516295154,1.,0.951056516295154,1.,0.951056516295154,1.,0.951056516295154,
1.,0.951056516295154,1.,0.951056516295154,1.,0.951056516295154,1.,0.951056516295154,
1.,0.951056516295154,1.,0.951056516295154,1.,0.951056516295154,1.,0.951056516295154,
1.,0.951056516295154,1.,0.951056516295154,1.,0.951056516295154,1.,0.951056516295154,
1.,0.951056516295154,1.,0.951056516295154,1.,0.951056516295154,1.,0.951056516295154,
1.,0.951056516295154,1.,0.951056516295154,1.,0.951056516295154,1.,0.951056516295154,
1.,0.951056516295154,1.,0.951056516295154,1.,0.951056516295154,1.,0.951056516295154,
1.,0.951056516295154,1.,0.951056516295154,1.,0.951056516295154,1.,0.951056516295154,
1.,0.951056516295154,1.,0.951056516295154,1.,0.951056516295154,1.,0.951056516295154,
1.,0.951056516295154,1.,0.951056516295154,1.,0.951056516295154,1.,0.951056516295154,
1.,0.951056516295154,1.,0.951056516295154,1.,0.951056516295154,1.,0.951056516295154,
1.,0.951056516295154,1.,0.951056516295154,1.,0.951056516295154,1.,0.951056516295154,
1.,0.951056516295154,1.,0.951056516295154,1.,0.951056516295154,1.,0.951056516295154,
1.,0.951056516295154,1.,0.951056516295154,1.,0.951056516295154,1.,0.951056516295154,
1.,0.951056516295154,1.,0.951056516295154,1.,0.951056516295154,1.,0.951056516295154,
1.,0.951056516295154,1.,0.951056516295154,1.,0.951056516295154,1.,0.951056516295154,
1.,0.951056516295154,1.,0.951056516295154,1.,0.951056516295154,1.,0.951056516295154,
1.,0.951056516295154,1.,0.951056516295154,1.,0.951056516295154,1.,0.951056516295154,
1.,0.951056516295154,1.,0.951056516295154,1.,0.951056516295154,1.,0.951056516295154,
1.,0.951056516295154,1.,0.951056516295154,1.,0.951056516295154,1.,0.951056516295154,
1.,0.951056516295154,1.,0.951056516295154,1.,0.951056516295154,1.,0.951056516295154,
1.,0.951056516295154,1.,0.951056516295154,1.,0.951056516295154,1.,0.951056516295154,
1.,0.951056516295154,1.,0.951056516295154,1.,0.951056516295154,1.,0.951056516295154,
1.,0.951056516295154,1.,0.951056516295154,1.,0.951056516295154,1.,0.951056516295154,
1.,0.951056516295154,1.,0.951056516295154,1.,0.951056516295154,1.,0.951056516295154,
1.,0.951056516295154,1.,0.951056516295154,1.,0.951056516295154,1.,0.951056516295154,
1.,0.951056516295154,1.,0.951056516295154,1.,0.951056516295154,1.,0.951056516295154,
1.,0.951056516295154,1.,0.951056516295154,1.,0.951056516295154,1.,0.951056516295154,
1.,0.951056516295154,1.,0.951056516295154,1.,0.951056516295154,1.,0.951056516295154,
1.,0.951056516295154,1.,0.951056516295154,1.,0.951056516295154,1.,0.951056516295154,
1.,0.951056516295154,1.,0.951056516295154,1.,0.951056516295154,1.,0.951056516295154,
1.,0.951056516295154,1.,0.951056516295154,1.,0.951056516295154,1.,0.951056516295154,
1.,0.951056516295154,1.,0.951056516295154,1.,0.951056516295154,1.,0.951056516295154,
1.,0.951056516295154,1.,0.951056516295154,1.,0.951056516295154,1.,0.951056516295154,
1.,0.951056516295154,1.,0.951056516295154,1.,0.951056516295154,1.,0.951056516295154,
1.,0.951056516295154,1.,0.951056516295154,1.,0.951056516295154,1.,0.951056516295154,
1.,0.951056516295154,1.,0.951056516295154,1.,0.951056516295154,1.,0.951056516295154,
1.,0.951056516295154,1.,0.951056516295154,1.,0.951056516295154,1.,0.951056516295154,
1.,0.951056516295154,1.,0.951056516295154,1.,0.951056516295154,1.,0.951056516295154,
1.,0.951056516295154,1.,0.951056516295154,1.,0.951056516295154,1.,0.951056516295154,
1.,0.951056516295154,1.,0.951056516295154,1.,0.951056516295154,1.,0.951056516295154,
1.,0.951056516295154,1.,0.951056516295154,1.,0.951056516295154,1.,0.951056516295154,
1.,0.951056516295154,1.,0.951056516295154,1.,0.951056516295154,1.,0.951056516295154,
1.,0.951056516295154,1.,0.951056516295154,1.,0.951056516295154,1.,0.951056516295154,
1.,0.951056516295154,1.,0.951056516295154,1.,0.951056516295154,1.,0.951056516295154,
1.,0.951056516295154,1.,0.951056516295154,1.,0.951056516295154,1.,0.951056516295154,
1.,0.951056516295154,1.,0.951056516295154,1.,0.951056516295154,1.,0.951056516295154,
1.,0.951056516295154,1.,0.951056516295154,1.,0.951056516295154,1.,0.951056516295154,
1.,0.951056516295154,1.,0.951056516295154,1.,0.951056516295154,1.,0.951056516295154,
1.,0.951056516295154,1.,0.951056516295154,1.,0.951056516295154,1.,0.951056516295154,
1.,0.951056516295154,1.,0.951056516295154,1.,0.951056516295154,1.,0.951056516295154,
1.,0.951056516295154,1.,0.951056516295154,1.,0.951056516295154,1.,0.951056516295154,
1.,0.951056516295154,1.,0.951056516295154,1.,0.951056516295154,1.,0.951056516295154,
1.,0.951056516295154,1.,0.951056516295154,1.,0.951056516295154,1.,0.951056516295154,
1.,0.951056516295154,1.,0.951056516295154,1.,0.951056516295154,1.,0.951056516295154,
1.,0.951056516295154,1.,0.951056516295154,1.,0.951056516295154,1.,0.951056516295154,
1.,0.951056516295154,1.,0.951056516295154,1.,0.951056516295154,1.,0.951056516295154,
1.,0.951056516295154,1.,0.951056516295154,1.,0.951056516295154,1.,0.951056516295154,
1.,0.951056516295154,1.,0.951056516295154,1.,0.951056516295154,1.,0.951056516295154,
1.,0.951056516295154,1.,0.951056516295154,1.,0.951056516295154,1.,0.951056516295154,
1.,0.951056516295154,1.,0.951056516295154,1.,0.951056516295154,1.,0.951056516295154,
1.,0.951056516295154,1.,0.951056516295154,1.,0.951056516295154,1.,0.951056516295154,
1.,0.951056516295154,1.,0.951056516295154,1.,0.951056516295154,1.,0.951056516295154,
1.,0.951056516295154,1.,0.951056516295154,1.,0.951056516295154,1.,0.951056516295154,
1.,0.951056516295154,1.,0.951056516295154,1.,0.951056516295154,1.,0.951056516295154,
1.,0.951056516295154,1.,0.951056516295154,1.,0.951056516295154,1.,0.951056516295154,
1.,0.951056516295154,1.,0.951056516295154,1.,0.951056516295154,1.,0.951056516295154,
1.,0.951056516295154,1.,0.951056516295154,1.,0.951056516295154,1.,0.951056516295154,
1.,0.951056516295154,1.,0.951056516295154,1.,0.951056516295154,1.,0.951056516295154,
1.,0.951056516295154,1.,0.951056516295154,1.,0.951056516295154,1.,0.951056516295154,
1.,0.951056516295154,1.,0.951056516295154,1.,0.951056516295154,1.,0.951056516295154,
1.,0.951056516295154,1.,0.951056516295154,1.,0.951056516295154,1.,0.951056516295154,
1.,0.951056516295154,1.,0.951056516295154,1.,0.951056516295154,1.,0.951056516295154,
1.,0.951056516295154,1.,0.951056516295154,1.,0.951056516295154,1.,0.951056516295154,
1.,0.951056516295154,1.,0.951056516295154,1.,0.951056516295154,1.,0.951056516295154,
1.,0.951056516295154,1.,0.951056516295154,1.,0.951056516295154,1.,0.951056516295154,
1.,0.951056516295154,1.,0.951056516295154,1.,0.951056516295154,1.,0.951056516295154,
1.,0.951056516295154,1.,0.951056516295154,1.,0.951056516295154,1.,0.951056516295154,
1.,0.951056516295154,1.,0.951056516295154,1.,0.951056516295154,1.,0.951056516295154,
1.,0.951056516295154,1.,0.951056516295154,1.,0.951056516295154,1.,0.951056516295154,
1.,0.951056516295154,1.,0.951056516295154,1.,0.951056516295154,1.,0.951056516295154,
1.,0.951056516295154,1.,0.951056516295154,1.,0.951056516295154,1.,0.951056516295154,
1.,0.951056516295154,1.,0.951056516295154,1.,0.951056516295154,1.,0.951056516295154,
1.,0.951056516295154,1.,0.951056516295154,1.,0.951056516295154,1.,0.951056516295154,
1.,0.951056516295154,1.,0.951056516295154,1.,0.951056516295154,1.,0.951056516295154,
1.,0.951056516295154,1.,0.951056516295154,1.,0.951056516295154,1.,0.951056516295154,
1.,0.951056516295154,1.,0.951056516295154,1.,0.951056516295154,1.,0.951056516295154,
1.,0.951056516295154,1.,0.951056516295154,1.,0.951056516295154,1.,0.951056516295154,
1.,0.951056516295154,1.,0.951056516295154,1.,0.951056516295154,1.,0.951056516295154,
1.,0.951056516295154,1.,0.951056516295154,1.,0.951056516295154,1.,0.951056516295154,
1.,0.951056516295154,1.,0.951056516295154,1.,0.951056516295154,1.,0.951056516295154,
1.,0.951056516295154,1.,0.951056516295154,1.,0.951056516295154,1.,0.951056516295154,
1.,0.951056516295154,1.,0.951056516295154,1.,0.951056516295154,1.,0.951056516295154,
1.,0.951056516295154,1.,0.951056516295154,1.,0.951056516295154,1.,0.951056516295154,
1.,0.951056516295154,1.,0.951056516295154,1.,0.951056516295154,1.,0.951056516295154,
1.,0.951056516295154,1.,0.951056516295154,1.,0.951056516295154,1.,0.951056516295154,
1.,0.951056516295154,1.,0.951056516295154,1.,0.951056516295154,1.,0.951056516295154,
1.,0.951056516295154,1.,0.951056516295154,1.,0.951056516295154,1.,0.951056516295154,
1.,0.951056516295154,1.,0.951056516295154,1.,0.951056516295154,1.,0.951056516295154,
1.,0.951056516295154,1.,0.951056516295154,1.,0.951056516295154,1.,0.951056516295154,
1.,0.951056516295154,1.,0.951056516295154,1.,0.951056516295154,1.,0.951056516295154,
1.,0.951056516295154,1.,0.951056516295154,1.,0.951056516295154,1.,0.951056516295154,
1.,0.951056516295154,1.,0.951056516295154,1.,0.951056516295154,1.,0.951056516295154,
1.,0.951056516295154,1.,0.951056516295154,1.,0.951056516295154,1.,0.951056516295154,
1.,0.951056516295154,1.,0.951056516295154,1.,0.951056516295154,1.,0.951056516295154,
1.,0.951056516295154,1.,0.951056516295154,1.,0.951056516295154,1.,0.951056516295154,
1.,0.951056516295154,1.,0.951056516295154,1.,0.951056516295154,1.,0.951056516295154,
1.,0.951056516295154,1.,0.951056516295154,1.,0.951056516295154,1.,0.951056516295154,
1.,0.951056516295154,1.,0.951056516295154,1.,0.951056516295154,1.,0.951056516295154,
1.,0.951056516295154,1.,0.951056516295154,1.,0.951056516295154,1.,0.951056516295154,
1.,0.951056516295154,1.,0.951056516295154,1.,0.951056516295154,1.,0.951056516295154,
1.,0.951056516295154,1.,0.951056516295154,1.,0.951056516295154,1.,0.951056516295154,
1.,0.951056516295154,1.,0.951056516295154,1.,0.951056516295154,1.,0.951056516295154,
1.,0.951056516295154,1.,0.951056516295154,1.,0.951056516295154,1.,0.951056516295154,
1.,0.951056516295154,1.,0.951056516295154,1.,0.951056516295154,1.,0.951056516295154,
1.,0.951056516295154,1.,0.951056516295154,1.,0.951056516295154,1.,0.951056516295154,
1.,0.951056516295154,1.,0.951056516295154,1.,0.951056516295154,1.,0.951056516295154,
1.,0.951056516295154,1.,0.951056516295154,1.,0.951056516295154,1.,0.951056516295154,
1.,0.951056516295154,1.,0.951056516295154,1.,0.951056516295154,1.,0.951056516295154,
1.,0.951056516295154,1.,0.951056516295154,1.,0.951056516295154,1.,0.951056516295154,
1.,0.951056516295154,1.,0.951056516295154,1.,0.951056516295154,1.,0.951056516295154,
1.,0.951056516295154,1.,0.951056516295154,1.,0.951056516295154,1.,0.951056516295154,
1.,0.951056516295154,1.,0.951056516295154,1.,0.951056516295154,1.,0.951056516295154,
1.,0.951056516295154,1.,0.951056516295154,1.,0.951056516295154,1.,0.951056516295154,
1.,0.951056516295154,1.,0.951056516295154,1.,0.951056516295154,1.,0.951056516295154,
1.),(1.,0.951056516295154,1.,0.951056516295154,1.,0.951056516295154,1.,
0.951056516295154,1.,0.951056516295154,1.,0.951056516295154,1.,0.951056516295154,
1.,0.951056516295154,1.,0.951056516295154,1.,0.951056516295154,1.,0.951056516295154,
1.,0.951056516295154,1.,0.951056516295154,1.,0.951056516295154,1.,0.951056516295154,
1.,0.951056516295154,1.,0.951056516295154,1.,0.951056516295154,1.,0.951056516295154,
1.,0.951056516295154,1.,0.951056516295154,1.,0.951056516295154,1.,0.951056516295154,
1.,0.951056516295154,1.,0.951056516295154,1.,0.951056516295154,1.,0.951056516295154,
1.,0.951056516295154,1.,0.951056516295154,1.,0.951056516295154,1.,0.951056516295154,
1.,0.951056516295154,1.,0.951056516295154,1.,0.951056516295154,1.,0.951056516295154,
1.,0.951056516295154,1.,0.951056516295154,1.,0.951056516295154,1.,0.951056516295154,
1.,0.951056516295154,1.,0.951056516295154,1.,0.951056516295154,1.,0.951056516295154,
1.,0.951056516295154,1.,0.951056516295154,1.,0.951056516295154,1.,0.951056516295154,
1.,0.951056516295154,1.,0.951056516295154,1.,0.951056516295154,1.,0.951056516295154,
1.,0.951056516295154,1.,0.951056516295154,1.,0.951056516295154,1.,0.951056516295154,
1.,0.951056516295154,1.,0.951056516295154,1.,0.951056516295154,1.,0.951056516295154,
1.,0.951056516295154,1.,0.951056516295154,1.,0.951056516295154,1.,0.951056516295154,
1.,0.951056516295154,1.,0.951056516295154,1.,0.951056516295154,1.,0.951056516295154,
1.,0.951056516295154,1.,0.951056516295154,1.,0.951056516295154,1.,0.951056516295154,
1.,0.951056516295154,1.,0.951056516295154,1.,0.951056516295154,1.,0.951056516295154,
1.,0.951056516295154,1.,0.951056516295154,1.,0.951056516295154,1.,0.951056516295154,
1.,0.951056516295154,1.,0.951056516295154,1.,0.951056516295154,1.,0.951056516295154,
1.,0.951056516295154,1.,0.951056516295154,1.,0.951056516295154,1.,0.951056516295154,
1.,0.951056516295154,1.,0.951056516295154,1.,0.951056516295154,1.,0.951056516295154,
1.,0.951056516295154,1.,0.951056516295154,1.,0.951056516295154,1.,0.951056516295154,
1.,0.951056516295154,1.,0.951056516295154,1.,0.951056516295154,1.,0.951056516295154,
1.,0.951056516295154,1.,0.951056516295154,1.,0.951056516295154,1.,0.951056516295154,
1.,0.951056516295154,1.,0.951056516295154,1.,0.951056516295154,1.,0.951056516295154,
1.,0.951056516295154,1.,0.951056516295154,1.,0.951056516295154,1.,0.951056516295154,
1.,0.951056516295154,1.,0.951056516295154,1.,0.951056516295154,1.,0.951056516295154,
1.,0.951056516295154,1.,0.951056516295154,1.,0.951056516295154,1.,0.951056516295154,
1.,0.951056516295154,1.,0.951056516295154,1.,0.951056516295154,1.,0.951056516295154,
1.,0.951056516295154,1.,0.951056516295154,1.,0.951056516295154,1.,0.951056516295154,
1.,0.951056516295154,1.,0.951056516295154,1.,0.951056516295154,1.,0.951056516295154,
1.,0.951056516295154,1.,0.951056516295154,1.,0.951056516295154,1.,0.951056516295154,
1.,0.951056516295154,1.,0.951056516295154,1.,0.951056516295154,1.,0.951056516295154,
1.,0.951056516295154,1.,0.951056516295154,1.,0.951056516295154,1.,0.951056516295154,
1.,0.951056516295154,1.,0.951056516295154,1.,0.951056516295154,1.,0.951056516295154,
1.,0.951056516295154,1.,0.951056516295154,1.,0.951056516295154,1.,0.951056516295154,
1.,0.951056516295154,1.,0.951056516295154,1.,0.951056516295154,1.,0.951056516295154,
1.,0.951056516295154,1.,0.951056516295154,1.,0.951056516295154,1.,0.951056516295154,
1.,0.951056516295154,1.,0.951056516295154,1.,0.951056516295154,1.,0.951056516295154,
1.,0.951056516295154,1.,0.951056516295154,1.,0.951056516295154,1.,0.951056516295154,
1.,0.951056516295154,1.,0.951056516295154,1.,0.951056516295154,1.,0.951056516295154,
1.,0.951056516295154,1.,0.951056516295154,1.,0.951056516295154,1.,0.951056516295154,
1.,0.951056516295154,1.,0.951056516295154,1.,0.951056516295154,1.,0.951056516295154,
1.,0.951056516295154,1.,0.951056516295154,1.,0.951056516295154,1.,0.951056516295154,
1.,0.951056516295154,1.,0.951056516295154,1.,0.951056516295154,1.,0.951056516295154,
1.,0.951056516295154,1.,0.951056516295154,1.,0.951056516295154,1.,0.951056516295154,
1.,0.951056516295154,1.,0.951056516295154,1.,0.951056516295154,1.,0.951056516295154,
1.,0.951056516295154,1.,0.951056516295154,1.,0.951056516295154,1.,0.951056516295154,
1.,0.951056516295154,1.,0.951056516295154,1.,0.951056516295154,1.,0.951056516295154,
1.,0.951056516295154,1.,0.951056516295154,1.,0.951056516295154,1.,0.951056516295154,
1.,0.951056516295154,1.,0.951056516295154,1.,0.951056516295154,1.,0.951056516295154,
1.,0.951056516295154,1.,0.951056516295154,1.,0.951056516295154,1.,0.951056516295154,
1.,0.951056516295154,1.,0.951056516295154,1.,0.951056516295154,1.,0.951056516295154,
1.,0.951056516295154,1.,0.951056516295154,1.,0.951056516295154,1.,0.951056516295154,
1.,0.951056516295154,1.,0.951056516295154,1.,0.951056516295154,1.,0.951056516295154,
1.,0.951056516295154,1.,0.951056516295154,1.,0.951056516295154,1.,0.951056516295154,
1.,0.951056516295154,1.,0.951056516295154,1.,0.951056516295154,1.,0.951056516295154,
1.,0.951056516295154,1.,0.951056516295154,1.,0.951056516295154,1.,0.951056516295154,
1.,0.951056516295154,1.,0.951056516295154,1.,0.951056516295154,1.,0.951056516295154,
1.,0.951056516295154,1.,0.951056516295154,1.,0.951056516295154,1.,0.951056516295154,
1.,0.951056516295154,1.,0.951056516295154,1.,0.951056516295154,1.,0.951056516295154,
1.,0.951056516295154,1.,0.951056516295154,1.,0.951056516295154,1.,0.951056516295154,
1.,0.951056516295154,1.,0.951056516295154,1.,0.951056516295154,1.,0.951056516295154,
1.,0.951056516295154,1.,0.951056516295154,1.,0.951056516295154,1.,0.951056516295154,
1.,0.951056516295154,1.,0.951056516295154,1.,0.951056516295154,1.,0.951056516295154,
1.,0.951056516295154,1.,0.951056516295154,1.,0.951056516295154,1.,0.951056516295154,
1.,0.951056516295154,1.,0.951056516295154,1.,0.951056516295154,1.,0.951056516295154,
1.,0.951056516295154,1.,0.951056516295154,1.,0.951056516295154,1.,0.951056516295154,
1.,0.951056516295154,1.,0.951056516295154,1.,0.951056516295154,1.,0.951056516295154,
1.,0.951056516295154,1.,0.951056516295154,1.,0.951056516295154,1.,0.951056516295154,
1.,0.951056516295154,1.,0.951056516295154,1.,0.951056516295154,1.,0.951056516295154,
1.,0.951056516295154,1.,0.951056516295154,1.,0.951056516295154,1.,0.951056516295154,
1.,0.951056516295154,1.,0.951056516295154,1.,0.951056516295154,1.,0.951056516295154,
1.,0.951056516295154,1.,0.951056516295154,1.,0.951056516295154,1.,0.951056516295154,
1.,0.951056516295154,1.,0.951056516295154,1.,0.951056516295154,1.,0.951056516295154,
1.,0.951056516295154,1.,0.951056516295154,1.,0.951056516295154,1.,0.951056516295154,
1.,0.951056516295154,1.,0.951056516295154,1.,0.951056516295154,1.,0.951056516295154,
1.,0.951056516295154,1.,0.951056516295154,1.,0.951056516295154,1.,0.951056516295154,
1.,0.951056516295154,1.,0.951056516295154,1.,0.951056516295154,1.,0.951056516295154,
1.,0.951056516295154,1.,0.951056516295154,1.,0.951056516295154,1.,0.951056516295154,
1.,0.951056516295154,1.,0.951056516295154,1.,0.951056516295154,1.,0.951056516295154,
1.,0.951056516295154,1.,0.951056516295154,1.,0.951056516295154,1.,0.951056516295154,
1.,0.951056516295154,1.,0.951056516295154,1.,0.951056516295154,1.,0.951056516295154,
1.,0.951056516295154,1.,0.951056516295154,1.,0.951056516295154,1.,0.951056516295154,
1.,0.951056516295154,1.,0.951056516295154,1.,0.951056516295154,1.,0.951056516295154,
1.,0.951056516295154,1.,0.951056516295154,1.,0.951056516295154,1.,0.951056516295154,
1.,0.951056516295154,1.,0.951056516295154,1.,0.951056516295154,1.,0.951056516295154,
1.,0.951056516295154,1.,0.951056516295154,1.,0.951056516295154,1.,0.951056516295154,
1.,0.951056516295154,1.,0.951056516295154,1.,0.951056516295154,1.,0.951056516295154,
1.,0.951056516295154,1.,0.951056516295154,1.,0.951056516295154,1.,0.951056516295154,
1.,0.951056516295154,1.,0.951056516295154,1.,0.951056516295154,1.,0.951056516295154,
1.,0.951056516295154,1.,0.951056516295154,1.,0.951056516295154,1.,0.951056516295154,
1.,0.951056516295154,1.,0.951056516295154,1.,0.951056516295154,1.,0.951056516295154,
1.,0.951056516295154,1.,0.951056516295154,1.,0.951056516295154,1.,0.951056516295154,
1.,0.951056516295154,1.,0.951056516295154,1.,0.951056516295154,1.,0.951056516295154,
1.,0.951056516295154,1.,0.951056516295154,1.,0.951056516295154,1.,0.951056516295154,
1.,0.951056516295154,1.,0.951056516295154,1.,0.951056516295154,1.,0.951056516295154,
1.,0.951056516295154,1.,0.951056516295154,1.,0.951056516295154,1.,0.951056516295154,
1.,0.951056516295154,1.,0.951056516295154,1.,0.951056516295154,1.,0.951056516295154,
1.,0.951056516295154,1.,0.951056516295154,1.,0.951056516295154,1.,0.951056516295154,
1.,0.951056516295154,1.,0.951056516295154,1.,0.951056516295154,1.,0.951056516295154,
1.,0.951056516295154,1.,0.951056516295154,1.,0.951056516295154,1.,0.951056516295154,
1.,0.951056516295154,1.,0.951056516295154,1.,0.951056516295154,1.,0.951056516295154,
1.,0.951056516295154,1.,0.951056516295154,1.,0.951056516295154,1.,0.951056516295154,
1.,0.951056516295154,1.,0.951056516295154,1.,0.951056516295154,1.,0.951056516295154,
1.,0.951056516295154,1.,0.951056516295154,1.,0.951056516295154,1.,0.951056516295154,
1.,0.951056516295154,1.,0.951056516295154,1.,0.951056516295154,1.,0.951056516295154,
1.,0.951056516295154,1.,0.951056516295154,1.,0.951056516295154,1.,0.951056516295154,
1.,0.951056516295154,1.,0.951056516295154,1.,0.951056516295154,1.,0.951056516295154,
1.,0.951056516295154,1.,0.951056516295154,1.,0.951056516295154,1.,0.951056516295154,
1.,0.951056516295154,1.,0.951056516295154,1.,0.951056516295154,1.,0.951056516295154,
1.,0.951056516295154,1.,0.951056516295154,1.,0.951056516295154,1.,0.951056516295154,
1.,0.951056516295154,1.,0.951056516295154,1.,0.951056516295154,1.,0.951056516295154,
1.,0.951056516295154,1.,0.951056516295154,1.,0.951056516295154,1.,0.951056516295154,
1.,0.951056516295154,1.,0.951056516295154,1.,0.951056516295154,1.,0.951056516295154,
1.,0.951056516295154,1.,0.951056516295154,1.,0.951056516295154,1.,0.951056516295154,
1.,0.951056516295154,1.,0.951056516295154,1.,0.951056516295154,1.,0.951056516295154,
1.,0.951056516295154,1.,0.951056516295154,1.,0.951056516295154,1.,0.951056516295154,
1.,0.951056516295154,1.,0.951056516295154,1.,0.951056516295154,1.,0.951056516295154,
1.,0.951056516295154,1.,0.951056516295154,1.,0.951056516295154,1.,0.951056516295154,
1.,0.951056516295154,1.,0.951056516295154,1.,0.951056516295154,1.,0.951056516295154,
1.,0.951056516295154,1.,0.951056516295154,1.,0.951056516295154,1.,0.951056516295154,
1.,0.951056516295154,1.,0.951056516295154,1.,0.951056516295154,1.,0.951056516295154,
1.,0.951056516295154,1.,0.951056516295154,1.,0.951056516295154,1.,0.951056516295154,
1.,0.951056516295154,1.,0.951056516295154,1.,0.951056516295154,1.,0.951056516295154,
1.,0.951056516295154,1.,0.951056516295154,1.,0.951056516295154,1.,0.951056516295154,
1.,0.951056516295154,1.,0.951056516295154,1.,0.951056516295154,1.,0.951056516295154,
1.,0.951056516295154,1.,0.951056516295154,1.,0.951056516295154,1.)))
REPRESENTATION_ITEM('')
SURFACE()
);
#3197=(
BOUNDED_SURFACE()
B_SPLINE_SURFACE(1,2,((#287932,#287933,#287934,#287935,#287936,#287937,
#287938,#287939,#287940,#287941,#287942,#287943,#287944,#287945,#287946,
#287947,#287948,#287949,#287950,#287951,#287952,#287953,#287954,#287955,
#287956,#287957,#287958,#287959,#287960,#287961,#287962,#287963,#287964,
#287965,#287966,#287967,#287968,#287969,#287970,#287971,#287972,#287973,
#287974,#287975,#287976,#287977,#287978,#287979,#287980,#287981,#287982,
#287983,#287984,#287985,#287986,#287987,#287988,#287989,#287990,#287991,
#287992,#287993,#287994,#287995,#287996,#287997,#287998,#287999,#288000,
#288001,#288002,#288003,#288004,#288005,#288006,#288007,#288008,#288009,
#288010,#288011,#288012,#288013,#288014,#288015,#288016,#288017,#288018,
#288019,#288020,#288021,#288022,#288023,#288024,#288025,#288026,#288027,
#288028,#288029,#288030,#288031,#288032,#288033,#288034,#288035,#288036,
#288037,#288038,#288039,#288040,#288041,#288042,#288043,#288044,#288045,
#288046,#288047,#288048,#288049,#288050,#288051,#288052,#288053,#288054,
#288055,#288056,#288057,#288058,#288059,#288060,#288061,#288062,#288063,
#288064,#288065,#288066,#288067,#288068,#288069,#288070,#288071,#288072,
#288073,#288074,#288075,#288076,#288077,#288078,#288079,#288080,#288081,
#288082,#288083,#288084,#288085,#288086,#288087,#288088,#288089,#288090,
#288091,#288092,#288093,#288094,#288095,#288096,#288097,#288098,#288099,
#288100,#288101,#288102,#288103,#288104,#288105,#288106,#288107,#288108,
#288109,#288110,#288111,#288112,#288113,#288114,#288115,#288116,#288117,
#288118,#288119,#288120,#288121,#288122,#288123,#288124,#288125,#288126,
#288127,#288128,#288129,#288130,#288131,#288132,#288133,#288134,#288135,
#288136,#288137,#288138,#288139,#288140,#288141,#288142,#288143,#288144,
#288145,#288146,#288147,#288148,#288149,#288150,#288151,#288152,#288153,
#288154,#288155,#288156,#288157,#288158,#288159,#288160,#288161,#288162,
#288163,#288164,#288165,#288166,#288167,#288168,#288169,#288170,#288171,
#288172,#288173,#288174,#288175,#288176,#288177,#288178,#288179,#288180,
#288181,#288182,#288183,#288184,#288185,#288186,#288187,#288188,#288189,
#288190,#288191,#288192,#288193,#288194,#288195,#288196,#288197,#288198,
#288199,#288200,#288201,#288202,#288203,#288204,#288205,#288206,#288207,
#288208,#288209,#288210,#288211,#288212,#288213,#288214,#288215,#288216,
#288217,#288218,#288219,#288220,#288221,#288222,#288223,#288224,#288225,
#288226,#288227,#288228,#288229,#288230,#288231,#288232,#288233,#288234,
#288235,#288236,#288237,#288238,#288239,#288240,#288241,#288242,#288243,
#288244,#288245,#288246,#288247,#288248,#288249,#288250,#288251,#288252,
#288253,#288254,#288255,#288256,#288257,#288258,#288259,#288260,#288261,
#288262,#288263,#288264,#288265,#288266,#288267,#288268,#288269,#288270,
#288271,#288272,#288273,#288274,#288275,#288276,#288277,#288278,#288279,
#288280,#288281,#288282,#288283,#288284,#288285,#288286,#288287,#288288,
#288289,#288290,#288291,#288292,#288293,#288294,#288295,#288296,#288297,
#288298,#288299,#288300,#288301,#288302,#288303,#288304,#288305,#288306,
#288307,#288308,#288309,#288310,#288311,#288312,#288313,#288314,#288315,
#288316,#288317,#288318,#288319,#288320,#288321,#288322,#288323,#288324,
#288325,#288326,#288327,#288328,#288329,#288330,#288331,#288332,#288333,
#288334,#288335,#288336,#288337,#288338,#288339,#288340,#288341,#288342,
#288343,#288344,#288345,#288346,#288347,#288348,#288349,#288350,#288351,
#288352,#288353,#288354,#288355,#288356,#288357,#288358,#288359,#288360,
#288361,#288362,#288363,#288364,#288365,#288366,#288367,#288368,#288369,
#288370,#288371,#288372,#288373,#288374,#288375,#288376,#288377,#288378,
#288379,#288380,#288381,#288382,#288383,#288384,#288385,#288386,#288387,
#288388,#288389,#288390,#288391,#288392,#288393,#288394,#288395,#288396,
#288397,#288398,#288399,#288400,#288401,#288402,#288403,#288404,#288405,
#288406,#288407,#288408,#288409,#288410,#288411,#288412,#288413,#288414,
#288415,#288416,#288417,#288418,#288419,#288420,#288421,#288422,#288423,
#288424,#288425,#288426,#288427,#288428,#288429,#288430,#288431,#288432,
#288433,#288434,#288435,#288436,#288437,#288438,#288439,#288440,#288441,
#288442,#288443,#288444,#288445,#288446,#288447,#288448,#288449,#288450,
#288451,#288452,#288453,#288454,#288455,#288456,#288457,#288458,#288459,
#288460,#288461,#288462,#288463,#288464,#288465,#288466,#288467,#288468,
#288469,#288470,#288471,#288472,#288473,#288474,#288475,#288476,#288477,
#288478,#288479,#288480,#288481,#288482,#288483,#288484,#288485,#288486,
#288487,#288488,#288489,#288490,#288491,#288492,#288493,#288494,#288495,
#288496,#288497,#288498,#288499,#288500,#288501,#288502,#288503,#288504,
#288505,#288506,#288507,#288508,#288509,#288510,#288511,#288512,#288513,
#288514,#288515,#288516,#288517,#288518,#288519,#288520,#288521,#288522,
#288523,#288524,#288525,#288526,#288527,#288528,#288529,#288530,#288531,
#288532,#288533,#288534,#288535,#288536,#288537,#288538,#288539,#288540,
#288541,#288542,#288543,#288544,#288545,#288546,#288547,#288548,#288549,
#288550,#288551,#288552,#288553,#288554,#288555,#288556,#288557,#288558,
#288559,#288560,#288561,#288562,#288563,#288564,#288565,#288566,#288567,
#288568,#288569,#288570,#288571,#288572,#288573,#288574,#288575,#288576,
#288577,#288578,#288579,#288580,#288581,#288582,#288583,#288584,#288585,
#288586,#288587,#288588,#288589,#288590,#288591,#288592,#288593,#288594,
#288595,#288596,#288597,#288598,#288599,#288600,#288601,#288602,#288603,
#288604,#288605,#288606,#288607,#288608,#288609,#288610,#288611,#288612,
#288613,#288614,#288615,#288616,#288617,#288618,#288619,#288620,#288621,
#288622,#288623,#288624,#288625,#288626,#288627,#288628,#288629,#288630,
#288631,#288632,#288633,#288634,#288635,#288636,#288637,#288638,#288639,
#288640,#288641,#288642,#288643,#288644,#288645,#288646,#288647,#288648,
#288649,#288650,#288651,#288652,#288653,#288654,#288655,#288656,#288657,
#288658,#288659,#288660,#288661,#288662,#288663,#288664,#288665,#288666,
#288667,#288668,#288669,#288670,#288671,#288672,#288673,#288674,#288675,
#288676,#288677,#288678,#288679,#288680,#288681,#288682,#288683,#288684,
#288685,#288686,#288687,#288688,#288689,#288690,#288691,#288692,#288693,
#288694,#288695,#288696,#288697,#288698,#288699,#288700,#288701,#288702,
#288703,#288704,#288705,#288706,#288707,#288708,#288709,#288710,#288711,
#288712,#288713,#288714,#288715,#288716,#288717,#288718,#288719,#288720,
#288721,#288722,#288723,#288724,#288725,#288726,#288727,#288728,#288729,
#288730,#288731,#288732,#288733,#288734,#288735,#288736,#288737,#288738,
#288739,#288740,#288741,#288742,#288743,#288744,#288745,#288746,#288747,
#288748,#288749,#288750,#288751,#288752,#288753,#288754,#288755,#288756,
#288757,#288758,#288759,#288760,#288761,#288762,#288763,#288764,#288765,
#288766,#288767,#288768,#288769,#288770,#288771,#288772,#288773,#288774,
#288775,#288776,#288777,#288778,#288779,#288780,#288781,#288782,#288783,
#288784,#288785,#288786,#288787,#288788,#288789,#288790,#288791,#288792,
#288793,#288794,#288795,#288796,#288797,#288798,#288799,#288800,#288801,
#288802,#288803,#288804,#288805,#288806,#288807,#288808,#288809,#288810,
#288811,#288812,#288813,#288814,#288815,#288816,#288817,#288818,#288819,
#288820,#288821,#288822,#288823,#288824,#288825,#288826,#288827,#288828,
#288829,#288830,#288831,#288832,#288833,#288834,#288835,#288836,#288837,
#288838,#288839,#288840,#288841,#288842,#288843,#288844,#288845,#288846,
#288847,#288848,#288849,#288850,#288851,#288852,#288853,#288854,#288855,
#288856,#288857,#288858,#288859,#288860,#288861,#288862,#288863,#288864,
#288865,#288866,#288867,#288868,#288869,#288870,#288871,#288872,#288873,
#288874,#288875,#288876,#288877,#288878,#288879,#288880,#288881,#288882,
#288883,#288884,#288885,#288886,#288887,#288888,#288889,#288890,#288891,
#288892,#288893,#288894,#288895,#288896,#288897,#288898,#288899,#288900,
#288901,#288902,#288903,#288904,#288905,#288906,#288907,#288908,#288909,
#288910,#288911,#288912,#288913,#288914,#288915,#288916,#288917,#288918,
#288919,#288920,#288921,#288922,#288923,#288924,#288925,#288926,#288927,
#288928,#288929,#288930,#288931,#288932,#288933,#288934,#288935,#288936,
#288937,#288938,#288939,#288940,#288941,#288942,#288943,#288944,#288945,
#288946,#288947,#288948,#288949,#288950,#288951,#288952,#288953,#288954,
#288955,#288956,#288957,#288958,#288959,#288960,#288961,#288962,#288963,
#288964,#288965,#288966,#288967,#288968),(#288969,#288970,#288971,#288972,
#288973,#288974,#288975,#288976,#288977,#288978,#288979,#288980,#288981,
#288982,#288983,#288984,#288985,#288986,#288987,#288988,#288989,#288990,
#288991,#288992,#288993,#288994,#288995,#288996,#288997,#288998,#288999,
#289000,#289001,#289002,#289003,#289004,#289005,#289006,#289007,#289008,
#289009,#289010,#289011,#289012,#289013,#289014,#289015,#289016,#289017,
#289018,#289019,#289020,#289021,#289022,#289023,#289024,#289025,#289026,
#289027,#289028,#289029,#289030,#289031,#289032,#289033,#289034,#289035,
#289036,#289037,#289038,#289039,#289040,#289041,#289042,#289043,#289044,
#289045,#289046,#289047,#289048,#289049,#289050,#289051,#289052,#289053,
#289054,#289055,#289056,#289057,#289058,#289059,#289060,#289061,#289062,
#289063,#289064,#289065,#289066,#289067,#289068,#289069,#289070,#289071,
#289072,#289073,#289074,#289075,#289076,#289077,#289078,#289079,#289080,
#289081,#289082,#289083,#289084,#289085,#289086,#289087,#289088,#289089,
#289090,#289091,#289092,#289093,#289094,#289095,#289096,#289097,#289098,
#289099,#289100,#289101,#289102,#289103,#289104,#289105,#289106,#289107,
#289108,#289109,#289110,#289111,#289112,#289113,#289114,#289115,#289116,
#289117,#289118,#289119,#289120,#289121,#289122,#289123,#289124,#289125,
#289126,#289127,#289128,#289129,#289130,#289131,#289132,#289133,#289134,
#289135,#289136,#289137,#289138,#289139,#289140,#289141,#289142,#289143,
#289144,#289145,#289146,#289147,#289148,#289149,#289150,#289151,#289152,
#289153,#289154,#289155,#289156,#289157,#289158,#289159,#289160,#289161,
#289162,#289163,#289164,#289165,#289166,#289167,#289168,#289169,#289170,
#289171,#289172,#289173,#289174,#289175,#289176,#289177,#289178,#289179,
#289180,#289181,#289182,#289183,#289184,#289185,#289186,#289187,#289188,
#289189,#289190,#289191,#289192,#289193,#289194,#289195,#289196,#289197,
#289198,#289199,#289200,#289201,#289202,#289203,#289204,#289205,#289206,
#289207,#289208,#289209,#289210,#289211,#289212,#289213,#289214,#289215,
#289216,#289217,#289218,#289219,#289220,#289221,#289222,#289223,#289224,
#289225,#289226,#289227,#289228,#289229,#289230,#289231,#289232,#289233,
#289234,#289235,#289236,#289237,#289238,#289239,#289240,#289241,#289242,
#289243,#289244,#289245,#289246,#289247,#289248,#289249,#289250,#289251,
#289252,#289253,#289254,#289255,#289256,#289257,#289258,#289259,#289260,
#289261,#289262,#289263,#289264,#289265,#289266,#289267,#289268,#289269,
#289270,#289271,#289272,#289273,#289274,#289275,#289276,#289277,#289278,
#289279,#289280,#289281,#289282,#289283,#289284,#289285,#289286,#289287,
#289288,#289289,#289290,#289291,#289292,#289293,#289294,#289295,#289296,
#289297,#289298,#289299,#289300,#289301,#289302,#289303,#289304,#289305,
#289306,#289307,#289308,#289309,#289310,#289311,#289312,#289313,#289314,
#289315,#289316,#289317,#289318,#289319,#289320,#289321,#289322,#289323,
#289324,#289325,#289326,#289327,#289328,#289329,#289330,#289331,#289332,
#289333,#289334,#289335,#289336,#289337,#289338,#289339,#289340,#289341,
#289342,#289343,#289344,#289345,#289346,#289347,#289348,#289349,#289350,
#289351,#289352,#289353,#289354,#289355,#289356,#289357,#289358,#289359,
#289360,#289361,#289362,#289363,#289364,#289365,#289366,#289367,#289368,
#289369,#289370,#289371,#289372,#289373,#289374,#289375,#289376,#289377,
#289378,#289379,#289380,#289381,#289382,#289383,#289384,#289385,#289386,
#289387,#289388,#289389,#289390,#289391,#289392,#289393,#289394,#289395,
#289396,#289397,#289398,#289399,#289400,#289401,#289402,#289403,#289404,
#289405,#289406,#289407,#289408,#289409,#289410,#289411,#289412,#289413,
#289414,#289415,#289416,#289417,#289418,#289419,#289420,#289421,#289422,
#289423,#289424,#289425,#289426,#289427,#289428,#289429,#289430,#289431,
#289432,#289433,#289434,#289435,#289436,#289437,#289438,#289439,#289440,
#289441,#289442,#289443,#289444,#289445,#289446,#289447,#289448,#289449,
#289450,#289451,#289452,#289453,#289454,#289455,#289456,#289457,#289458,
#289459,#289460,#289461,#289462,#289463,#289464,#289465,#289466,#289467,
#289468,#289469,#289470,#289471,#289472,#289473,#289474,#289475,#289476,
#289477,#289478,#289479,#289480,#289481,#289482,#289483,#289484,#289485,
#289486,#289487,#289488,#289489,#289490,#289491,#289492,#289493,#289494,
#289495,#289496,#289497,#289498,#289499,#289500,#289501,#289502,#289503,
#289504,#289505,#289506,#289507,#289508,#289509,#289510,#289511,#289512,
#289513,#289514,#289515,#289516,#289517,#289518,#289519,#289520,#289521,
#289522,#289523,#289524,#289525,#289526,#289527,#289528,#289529,#289530,
#289531,#289532,#289533,#289534,#289535,#289536,#289537,#289538,#289539,
#289540,#289541,#289542,#289543,#289544,#289545,#289546,#289547,#289548,
#289549,#289550,#289551,#289552,#289553,#289554,#289555,#289556,#289557,
#289558,#289559,#289560,#289561,#289562,#289563,#289564,#289565,#289566,
#289567,#289568,#289569,#289570,#289571,#289572,#289573,#289574,#289575,
#289576,#289577,#289578,#289579,#289580,#289581,#289582,#289583,#289584,
#289585,#289586,#289587,#289588,#289589,#289590,#289591,#289592,#289593,
#289594,#289595,#289596,#289597,#289598,#289599,#289600,#289601,#289602,
#289603,#289604,#289605,#289606,#289607,#289608,#289609,#289610,#289611,
#289612,#289613,#289614,#289615,#289616,#289617,#289618,#289619,#289620,
#289621,#289622,#289623,#289624,#289625,#289626,#289627,#289628,#289629,
#289630,#289631,#289632,#289633,#289634,#289635,#289636,#289637,#289638,
#289639,#289640,#289641,#289642,#289643,#289644,#289645,#289646,#289647,
#289648,#289649,#289650,#289651,#289652,#289653,#289654,#289655,#289656,
#289657,#289658,#289659,#289660,#289661,#289662,#289663,#289664,#289665,
#289666,#289667,#289668,#289669,#289670,#289671,#289672,#289673,#289674,
#289675,#289676,#289677,#289678,#289679,#289680,#289681,#289682,#289683,
#289684,#289685,#289686,#289687,#289688,#289689,#289690,#289691,#289692,
#289693,#289694,#289695,#289696,#289697,#289698,#289699,#289700,#289701,
#289702,#289703,#289704,#289705,#289706,#289707,#289708,#289709,#289710,
#289711,#289712,#289713,#289714,#289715,#289716,#289717,#289718,#289719,
#289720,#289721,#289722,#289723,#289724,#289725,#289726,#289727,#289728,
#289729,#289730,#289731,#289732,#289733,#289734,#289735,#289736,#289737,
#289738,#289739,#289740,#289741,#289742,#289743,#289744,#289745,#289746,
#289747,#289748,#289749,#289750,#289751,#289752,#289753,#289754,#289755,
#289756,#289757,#289758,#289759,#289760,#289761,#289762,#289763,#289764,
#289765,#289766,#289767,#289768,#289769,#289770,#289771,#289772,#289773,
#289774,#289775,#289776,#289777,#289778,#289779,#289780,#289781,#289782,
#289783,#289784,#289785,#289786,#289787,#289788,#289789,#289790,#289791,
#289792,#289793,#289794,#289795,#289796,#289797,#289798,#289799,#289800,
#289801,#289802,#289803,#289804,#289805,#289806,#289807,#289808,#289809,
#289810,#289811,#289812,#289813,#289814,#289815,#289816,#289817,#289818,
#289819,#289820,#289821,#289822,#289823,#289824,#289825,#289826,#289827,
#289828,#289829,#289830,#289831,#289832,#289833,#289834,#289835,#289836,
#289837,#289838,#289839,#289840,#289841,#289842,#289843,#289844,#289845,
#289846,#289847,#289848,#289849,#289850,#289851,#289852,#289853,#289854,
#289855,#289856,#289857,#289858,#289859,#289860,#289861,#289862,#289863,
#289864,#289865,#289866,#289867,#289868,#289869,#289870,#289871,#289872,
#289873,#289874,#289875,#289876,#289877,#289878,#289879,#289880,#289881,
#289882,#289883,#289884,#289885,#289886,#289887,#289888,#289889,#289890,
#289891,#289892,#289893,#289894,#289895,#289896,#289897,#289898,#289899,
#289900,#289901,#289902,#289903,#289904,#289905,#289906,#289907,#289908,
#289909,#289910,#289911,#289912,#289913,#289914,#289915,#289916,#289917,
#289918,#289919,#289920,#289921,#289922,#289923,#289924,#289925,#289926,
#289927,#289928,#289929,#289930,#289931,#289932,#289933,#289934,#289935,
#289936,#289937,#289938,#289939,#289940,#289941,#289942,#289943,#289944,
#289945,#289946,#289947,#289948,#289949,#289950,#289951,#289952,#289953,
#289954,#289955,#289956,#289957,#289958,#289959,#289960,#289961,#289962,
#289963,#289964,#289965,#289966,#289967,#289968,#289969,#289970,#289971,
#289972,#289973,#289974,#289975,#289976,#289977,#289978,#289979,#289980,
#289981,#289982,#289983,#289984,#289985,#289986,#289987,#289988,#289989,
#289990,#289991,#289992,#289993,#289994,#289995,#289996,#289997,#289998,
#289999,#290000,#290001,#290002,#290003,#290004,#290005)),.UNSPECIFIED.,
 .F.,.F.,.F.)
B_SPLINE_SURFACE_WITH_KNOTS((2,2),(3,2,2,2,2,2,2,2,2,2,2,2,2,2,2,2,2,2,
2,2,2,2,2,2,2,2,2,2,2,2,2,2,2,2,2,2,2,2,2,2,2,2,2,2,2,2,2,2,2,2,2,2,2,2,
2,2,2,2,2,2,2,2,2,2,2,2,2,2,2,2,2,2,2,2,2,2,2,2,2,2,2,2,2,2,2,2,2,2,2,2,
2,2,2,2,2,2,2,2,2,2,2,2,2,2,2,2,2,2,2,2,2,2,2,2,2,2,2,2,2,2,2,2,2,2,2,2,
2,2,2,2,2,2,2,2,2,2,2,2,2,2,2,2,2,2,2,2,2,2,2,2,2,2,2,2,2,2,2,2,2,2,2,2,
2,2,2,2,2,2,2,2,2,2,2,2,2,2,2,2,2,2,2,2,2,2,2,2,2,2,2,2,2,2,2,2,2,2,2,2,
2,2,2,2,2,2,2,2,2,2,2,2,2,2,2,2,2,2,2,2,2,2,2,2,2,2,2,2,2,2,2,2,2,2,2,2,
2,2,2,2,2,2,2,2,2,2,2,2,2,2,2,2,2,2,2,2,2,2,2,2,2,2,2,2,2,2,2,2,2,2,2,2,
2,2,2,2,2,2,2,2,2,2,2,2,2,2,2,2,2,2,2,2,2,2,2,2,2,2,2,2,2,2,2,2,2,2,2,2,
2,2,2,2,2,2,2,2,2,2,2,2,2,2,2,2,2,2,2,2,2,2,2,2,2,2,2,2,2,2,2,2,2,2,2,2,
2,2,2,2,2,2,2,2,2,2,2,2,2,2,2,2,2,2,2,2,2,2,2,2,2,2,2,2,2,2,2,2,2,2,2,2,
2,2,2,2,2,2,2,2,2,2,2,2,2,2,2,2,2,2,2,2,2,2,2,2,2,2,2,2,2,2,2,2,2,2,2,2,
2,2,2,2,2,2,2,2,2,2,2,2,2,2,2,2,2,2,2,2,2,2,2,2,2,2,2,2,2,2,2,2,2,2,2,2,
2,2,2,2,2,2,2,2,2,2,2,2,2,2,2,2,2,2,2,2,2,2,2,2,2,2,2,2,2,2,2,2,2,2,2,2,
2,2,2,2,2,2,2,2,2,2,2,2,2,2,2,2,2,2,2,2,2,2,2,2,2,2,2,2,2,2,2,2,3),(0.,
1.),(0.,0.00192307692307692,0.00384615384615385,0.00576923076923077,0.00769230769230769,
0.00961538461538462,0.0115384615384615,0.0134615384615385,0.0153846153846154,
0.0173076923076923,0.0192307692307692,0.0211538461538462,0.0230769230769231,
0.025,0.0269230769230769,0.0288461538461538,0.0307692307692308,0.0326923076923077,
0.0346153846153846,0.0365384615384615,0.0384615384615385,0.0403846153846154,
0.0423076923076923,0.0442307692307692,0.0461538461538462,0.0480769230769231,
0.05,0.0519230769230769,0.0538461538461538,0.0557692307692308,0.0576923076923077,
0.0596153846153846,0.0615384615384615,0.0634615384615385,0.0653846153846154,
0.0673076923076923,0.0692307692307692,0.0711538461538462,0.0730769230769231,
0.075,0.0769230769230769,0.0788461538461538,0.0807692307692308,0.0826923076923077,
0.0846153846153846,0.0865384615384615,0.0884615384615385,0.0903846153846154,
0.0923076923076923,0.0942307692307692,0.0961538461538462,0.0980769230769231,
0.1,0.101923076923077,0.103846153846154,0.105769230769231,0.107692307692308,
0.109615384615385,0.111538461538462,0.113461538461538,0.115384615384615,
0.117307692307692,0.119230769230769,0.121153846153846,0.123076923076923,
0.125,0.126923076923077,0.128846153846154,0.130769230769231,0.132692307692308,
0.134615384615385,0.136538461538462,0.138461538461538,0.140384615384615,
0.142307692307692,0.144230769230769,0.146153846153846,0.148076923076923,
0.15,0.151923076923077,0.153846153846154,0.155769230769231,0.157692307692308,
0.159615384615385,0.161538461538462,0.163461538461538,0.165384615384615,
0.167307692307692,0.169230769230769,0.171153846153846,0.173076923076923,
0.175,0.176923076923077,0.178846153846154,0.180769230769231,0.182692307692308,
0.184615384615385,0.186538461538462,0.188461538461538,0.190384615384615,
0.192307692307692,0.194230769230769,0.196153846153846,0.198076923076923,
0.2,0.201923076923077,0.203846153846154,0.205769230769231,0.207692307692308,
0.209615384615385,0.211538461538462,0.213461538461538,0.215384615384615,
0.217307692307692,0.219230769230769,0.221153846153846,0.223076923076923,
0.225,0.226923076923077,0.228846153846154,0.230769230769231,0.232692307692308,
0.234615384615385,0.236538461538462,0.238461538461538,0.240384615384615,
0.242307692307692,0.244230769230769,0.246153846153846,0.248076923076923,
0.25,0.251923076923077,0.253846153846154,0.255769230769231,0.257692307692308,
0.259615384615385,0.261538461538462,0.263461538461538,0.265384615384615,
0.267307692307692,0.269230769230769,0.271153846153846,0.273076923076923,
0.275,0.276923076923077,0.278846153846154,0.280769230769231,0.282692307692308,
0.284615384615385,0.286538461538462,0.288461538461538,0.290384615384615,
0.292307692307692,0.294230769230769,0.296153846153846,0.298076923076923,
0.3,0.301923076923077,0.303846153846154,0.305769230769231,0.307692307692308,
0.309615384615385,0.311538461538462,0.313461538461538,0.315384615384615,
0.317307692307692,0.319230769230769,0.321153846153846,0.323076923076923,
0.325,0.326923076923077,0.328846153846154,0.330769230769231,0.332692307692308,
0.334615384615385,0.336538461538462,0.338461538461538,0.340384615384615,
0.342307692307692,0.344230769230769,0.346153846153846,0.348076923076923,
0.35,0.351923076923077,0.353846153846154,0.355769230769231,0.357692307692308,
0.359615384615385,0.361538461538462,0.363461538461538,0.365384615384615,
0.367307692307692,0.369230769230769,0.371153846153846,0.373076923076923,
0.375,0.376923076923077,0.378846153846154,0.380769230769231,0.382692307692308,
0.384615384615385,0.386538461538462,0.388461538461538,0.390384615384615,
0.392307692307692,0.394230769230769,0.396153846153846,0.398076923076923,
0.4,0.401923076923077,0.403846153846154,0.405769230769231,0.407692307692308,
0.409615384615385,0.411538461538462,0.413461538461538,0.415384615384615,
0.417307692307692,0.419230769230769,0.421153846153846,0.423076923076923,
0.425,0.426923076923077,0.428846153846154,0.430769230769231,0.432692307692308,
0.434615384615385,0.436538461538462,0.438461538461538,0.440384615384615,
0.442307692307692,0.444230769230769,0.446153846153846,0.448076923076923,
0.45,0.451923076923077,0.453846153846154,0.455769230769231,0.457692307692308,
0.459615384615385,0.461538461538462,0.463461538461538,0.465384615384615,
0.467307692307692,0.469230769230769,0.471153846153846,0.473076923076923,
0.475,0.476923076923077,0.478846153846154,0.480769230769231,0.482692307692308,
0.484615384615385,0.486538461538462,0.488461538461538,0.490384615384615,
0.492307692307692,0.494230769230769,0.496153846153846,0.498076923076923,
0.5,0.501923076923077,0.503846153846154,0.505769230769231,0.507692307692308,
0.509615384615385,0.511538461538461,0.513461538461538,0.515384615384615,
0.517307692307692,0.519230769230769,0.521153846153846,0.523076923076923,
0.525,0.526923076923077,0.528846153846154,0.530769230769231,0.532692307692308,
0.534615384615385,0.536538461538462,0.538461538461538,0.540384615384615,
0.542307692307692,0.544230769230769,0.546153846153846,0.548076923076923,
0.55,0.551923076923077,0.553846153846154,0.555769230769231,0.557692307692308,
0.559615384615385,0.561538461538462,0.563461538461538,0.565384615384615,
0.567307692307692,0.569230769230769,0.571153846153846,0.573076923076923,
0.575,0.576923076923077,0.578846153846154,0.580769230769231,0.582692307692308,
0.584615384615385,0.586538461538462,0.588461538461538,0.590384615384615,
0.592307692307692,0.594230769230769,0.596153846153846,0.598076923076923,
0.6,0.601923076923077,0.603846153846154,0.605769230769231,0.607692307692308,
0.609615384615385,0.611538461538462,0.613461538461539,0.615384615384615,
0.617307692307692,0.619230769230769,0.621153846153846,0.623076923076923,
0.625,0.626923076923077,0.628846153846154,0.630769230769231,0.632692307692308,
0.634615384615385,0.636538461538461,0.638461538461538,0.640384615384615,
0.642307692307692,0.644230769230769,0.646153846153846,0.648076923076923,
0.65,0.651923076923077,0.653846153846154,0.655769230769231,0.657692307692308,
0.659615384615385,0.661538461538462,0.663461538461538,0.665384615384615,
0.667307692307692,0.669230769230769,0.671153846153846,0.673076923076923,
0.675,0.676923076923077,0.678846153846154,0.680769230769231,0.682692307692308,
0.684615384615385,0.686538461538462,0.688461538461538,0.690384615384615,
0.692307692307692,0.694230769230769,0.696153846153846,0.698076923076923,
0.7,0.701923076923077,0.703846153846154,0.705769230769231,0.707692307692308,
0.709615384615385,0.711538461538462,0.713461538461538,0.715384615384615,
0.717307692307692,0.719230769230769,0.721153846153846,0.723076923076923,
0.725,0.726923076923077,0.728846153846154,0.730769230769231,0.732692307692308,
0.734615384615385,0.736538461538462,0.738461538461539,0.740384615384615,
0.742307692307692,0.744230769230769,0.746153846153846,0.748076923076923,
0.75,0.751923076923077,0.753846153846154,0.755769230769231,0.757692307692308,
0.759615384615385,0.761538461538461,0.763461538461538,0.765384615384615,
0.767307692307692,0.769230769230769,0.771153846153846,0.773076923076923,
0.775,0.776923076923077,0.778846153846154,0.780769230769231,0.782692307692308,
0.784615384615385,0.786538461538462,0.788461538461538,0.790384615384615,
0.792307692307692,0.794230769230769,0.796153846153846,0.798076923076923,
0.8,0.801923076923077,0.803846153846154,0.805769230769231,0.807692307692308,
0.809615384615385,0.811538461538462,0.813461538461538,0.815384615384615,
0.817307692307692,0.819230769230769,0.821153846153846,0.823076923076923,
0.825,0.826923076923077,0.828846153846154,0.830769230769231,0.832692307692308,
0.834615384615385,0.836538461538462,0.838461538461538,0.840384615384615,
0.842307692307692,0.844230769230769,0.846153846153846,0.848076923076923,
0.85,0.851923076923077,0.853846153846154,0.855769230769231,0.857692307692308,
0.859615384615385,0.861538461538462,0.863461538461539,0.865384615384615,
0.867307692307692,0.869230769230769,0.871153846153846,0.873076923076923,
0.875,0.876923076923077,0.878846153846154,0.880769230769231,0.882692307692308,
0.884615384615385,0.886538461538461,0.888461538461538,0.890384615384615,
0.892307692307692,0.894230769230769,0.896153846153846,0.898076923076923,
0.9,0.901923076923077,0.903846153846154,0.905769230769231,0.907692307692308,
0.909615384615385,0.911538461538462,0.913461538461538,0.915384615384615,
0.917307692307692,0.919230769230769,0.921153846153846,0.923076923076923,
0.925,0.926923076923077,0.928846153846154,0.930769230769231,0.932692307692308,
0.934615384615385,0.936538461538462,0.938461538461538,0.940384615384615,
0.942307692307692,0.944230769230769,0.946153846153846,0.948076923076923,
0.95,0.951923076923077,0.953846153846154,0.955769230769231,0.957692307692308,
0.959615384615385,0.961538461538462,0.963461538461538,0.965384615384615,
0.967307692307692,0.969230769230769,0.971153846153846,0.973076923076923,
0.975,0.976923076923077,0.978846153846154,0.980769230769231,0.982692307692308,
0.984615384615385,0.986538461538462,0.988461538461539,0.990384615384615,
0.992307692307692,0.994230769230769,0.996153846153846),.UNSPECIFIED.)
GEOMETRIC_REPRESENTATION_ITEM()
RATIONAL_B_SPLINE_SURFACE(((1.,0.951056516295154,1.,0.951056516295154,1.,
0.951056516295154,1.,0.951056516295154,1.,0.951056516295154,1.,0.951056516295154,
1.,0.951056516295154,1.,0.951056516295154,1.,0.951056516295154,1.,0.951056516295154,
1.,0.951056516295154,1.,0.951056516295154,1.,0.951056516295154,1.,0.951056516295154,
1.,0.951056516295154,1.,0.951056516295154,1.,0.951056516295154,1.,0.951056516295154,
1.,0.951056516295154,1.,0.951056516295154,1.,0.951056516295154,1.,0.951056516295154,
1.,0.951056516295154,1.,0.951056516295154,1.,0.951056516295154,1.,0.951056516295154,
1.,0.951056516295154,1.,0.951056516295154,1.,0.951056516295154,1.,0.951056516295154,
1.,0.951056516295154,1.,0.951056516295154,1.,0.951056516295154,1.,0.951056516295154,
1.,0.951056516295154,1.,0.951056516295154,1.,0.951056516295154,1.,0.951056516295154,
1.,0.951056516295154,1.,0.951056516295154,1.,0.951056516295154,1.,0.951056516295154,
1.,0.951056516295154,1.,0.951056516295154,1.,0.951056516295154,1.,0.951056516295154,
1.,0.951056516295154,1.,0.951056516295154,1.,0.951056516295154,1.,0.951056516295154,
1.,0.951056516295154,1.,0.951056516295154,1.,0.951056516295154,1.,0.951056516295154,
1.,0.951056516295154,1.,0.951056516295154,1.,0.951056516295154,1.,0.951056516295154,
1.,0.951056516295154,1.,0.951056516295154,1.,0.951056516295154,1.,0.951056516295154,
1.,0.951056516295154,1.,0.951056516295154,1.,0.951056516295154,1.,0.951056516295154,
1.,0.951056516295154,1.,0.951056516295154,1.,0.951056516295154,1.,0.951056516295154,
1.,0.951056516295154,1.,0.951056516295154,1.,0.951056516295154,1.,0.951056516295154,
1.,0.951056516295154,1.,0.951056516295154,1.,0.951056516295154,1.,0.951056516295154,
1.,0.951056516295154,1.,0.951056516295154,1.,0.951056516295154,1.,0.951056516295154,
1.,0.951056516295154,1.,0.951056516295154,1.,0.951056516295154,1.,0.951056516295154,
1.,0.951056516295154,1.,0.951056516295154,1.,0.951056516295154,1.,0.951056516295154,
1.,0.951056516295154,1.,0.951056516295154,1.,0.951056516295154,1.,0.951056516295154,
1.,0.951056516295154,1.,0.951056516295154,1.,0.951056516295154,1.,0.951056516295154,
1.,0.951056516295154,1.,0.951056516295154,1.,0.951056516295154,1.,0.951056516295154,
1.,0.951056516295154,1.,0.951056516295154,1.,0.951056516295154,1.,0.951056516295154,
1.,0.951056516295154,1.,0.951056516295154,1.,0.951056516295154,1.,0.951056516295154,
1.,0.951056516295154,1.,0.951056516295154,1.,0.951056516295154,1.,0.951056516295154,
1.,0.951056516295154,1.,0.951056516295154,1.,0.951056516295154,1.,0.951056516295154,
1.,0.951056516295154,1.,0.951056516295154,1.,0.951056516295154,1.,0.951056516295154,
1.,0.951056516295154,1.,0.951056516295154,1.,0.951056516295154,1.,0.951056516295154,
1.,0.951056516295154,1.,0.951056516295154,1.,0.951056516295154,1.,0.951056516295154,
1.,0.951056516295154,1.,0.951056516295154,1.,0.951056516295154,1.,0.951056516295154,
1.,0.951056516295154,1.,0.951056516295154,1.,0.951056516295154,1.,0.951056516295154,
1.,0.951056516295154,1.,0.951056516295154,1.,0.951056516295154,1.,0.951056516295154,
1.,0.951056516295154,1.,0.951056516295154,1.,0.951056516295154,1.,0.951056516295154,
1.,0.951056516295154,1.,0.951056516295154,1.,0.951056516295154,1.,0.951056516295154,
1.,0.951056516295154,1.,0.951056516295154,1.,0.951056516295154,1.,0.951056516295154,
1.,0.951056516295154,1.,0.951056516295154,1.,0.951056516295154,1.,0.951056516295154,
1.,0.951056516295154,1.,0.951056516295154,1.,0.951056516295154,1.,0.951056516295154,
1.,0.951056516295154,1.,0.951056516295154,1.,0.951056516295154,1.,0.951056516295154,
1.,0.951056516295154,1.,0.951056516295154,1.,0.951056516295154,1.,0.951056516295154,
1.,0.951056516295154,1.,0.951056516295154,1.,0.951056516295154,1.,0.951056516295154,
1.,0.951056516295154,1.,0.951056516295154,1.,0.951056516295154,1.,0.951056516295154,
1.,0.951056516295154,1.,0.951056516295154,1.,0.951056516295154,1.,0.951056516295154,
1.,0.951056516295154,1.,0.951056516295154,1.,0.951056516295154,1.,0.951056516295154,
1.,0.951056516295154,1.,0.951056516295154,1.,0.951056516295154,1.,0.951056516295154,
1.,0.951056516295154,1.,0.951056516295154,1.,0.951056516295154,1.,0.951056516295154,
1.,0.951056516295154,1.,0.951056516295154,1.,0.951056516295154,1.,0.951056516295154,
1.,0.951056516295154,1.,0.951056516295154,1.,0.951056516295154,1.,0.951056516295154,
1.,0.951056516295154,1.,0.951056516295154,1.,0.951056516295154,1.,0.951056516295154,
1.,0.951056516295154,1.,0.951056516295154,1.,0.951056516295154,1.,0.951056516295154,
1.,0.951056516295154,1.,0.951056516295154,1.,0.951056516295154,1.,0.951056516295154,
1.,0.951056516295154,1.,0.951056516295154,1.,0.951056516295154,1.,0.951056516295154,
1.,0.951056516295154,1.,0.951056516295154,1.,0.951056516295154,1.,0.951056516295154,
1.,0.951056516295154,1.,0.951056516295154,1.,0.951056516295154,1.,0.951056516295154,
1.,0.951056516295154,1.,0.951056516295154,1.,0.951056516295154,1.,0.951056516295154,
1.,0.951056516295154,1.,0.951056516295154,1.,0.951056516295154,1.,0.951056516295154,
1.,0.951056516295154,1.,0.951056516295154,1.,0.951056516295154,1.,0.951056516295154,
1.,0.951056516295154,1.,0.951056516295154,1.,0.951056516295154,1.,0.951056516295154,
1.,0.951056516295154,1.,0.951056516295154,1.,0.951056516295154,1.,0.951056516295154,
1.,0.951056516295154,1.,0.951056516295154,1.,0.951056516295154,1.,0.951056516295154,
1.,0.951056516295154,1.,0.951056516295154,1.,0.951056516295154,1.,0.951056516295154,
1.,0.951056516295154,1.,0.951056516295154,1.,0.951056516295154,1.,0.951056516295154,
1.,0.951056516295154,1.,0.951056516295154,1.,0.951056516295154,1.,0.951056516295154,
1.,0.951056516295154,1.,0.951056516295154,1.,0.951056516295154,1.,0.951056516295154,
1.,0.951056516295154,1.,0.951056516295154,1.,0.951056516295154,1.,0.951056516295154,
1.,0.951056516295154,1.,0.951056516295154,1.,0.951056516295154,1.,0.951056516295154,
1.,0.951056516295154,1.,0.951056516295154,1.,0.951056516295154,1.,0.951056516295154,
1.,0.951056516295154,1.,0.951056516295154,1.,0.951056516295154,1.,0.951056516295154,
1.,0.951056516295154,1.,0.951056516295154,1.,0.951056516295154,1.,0.951056516295154,
1.,0.951056516295154,1.,0.951056516295154,1.,0.951056516295154,1.,0.951056516295154,
1.,0.951056516295154,1.,0.951056516295154,1.,0.951056516295154,1.,0.951056516295154,
1.,0.951056516295154,1.,0.951056516295154,1.,0.951056516295154,1.,0.951056516295154,
1.,0.951056516295154,1.,0.951056516295154,1.,0.951056516295154,1.,0.951056516295154,
1.,0.951056516295154,1.,0.951056516295154,1.,0.951056516295154,1.,0.951056516295154,
1.,0.951056516295154,1.,0.951056516295154,1.,0.951056516295154,1.,0.951056516295154,
1.,0.951056516295154,1.,0.951056516295154,1.,0.951056516295154,1.,0.951056516295154,
1.,0.951056516295154,1.,0.951056516295154,1.,0.951056516295154,1.,0.951056516295154,
1.,0.951056516295154,1.,0.951056516295154,1.,0.951056516295154,1.,0.951056516295154,
1.,0.951056516295154,1.,0.951056516295154,1.,0.951056516295154,1.,0.951056516295154,
1.,0.951056516295154,1.,0.951056516295154,1.,0.951056516295154,1.,0.951056516295154,
1.,0.951056516295154,1.,0.951056516295154,1.,0.951056516295154,1.,0.951056516295154,
1.,0.951056516295154,1.,0.951056516295154,1.,0.951056516295154,1.,0.951056516295154,
1.,0.951056516295154,1.,0.951056516295154,1.,0.951056516295154,1.,0.951056516295154,
1.,0.951056516295154,1.,0.951056516295154,1.,0.951056516295154,1.,0.951056516295154,
1.,0.951056516295154,1.,0.951056516295154,1.,0.951056516295154,1.,0.951056516295154,
1.,0.951056516295154,1.,0.951056516295154,1.,0.951056516295154,1.,0.951056516295154,
1.,0.951056516295154,1.,0.951056516295154,1.,0.951056516295154,1.,0.951056516295154,
1.,0.951056516295154,1.,0.951056516295154,1.,0.951056516295154,1.,0.951056516295154,
1.,0.951056516295154,1.,0.951056516295154,1.,0.951056516295154,1.,0.951056516295154,
1.,0.951056516295154,1.,0.951056516295154,1.,0.951056516295154,1.,0.951056516295154,
1.,0.951056516295154,1.,0.951056516295154,1.,0.951056516295154,1.,0.951056516295154,
1.,0.951056516295154,1.,0.951056516295154,1.,0.951056516295154,1.,0.951056516295154,
1.,0.951056516295154,1.,0.951056516295154,1.,0.951056516295154,1.,0.951056516295154,
1.,0.951056516295154,1.,0.951056516295154,1.,0.951056516295154,1.,0.951056516295154,
1.,0.951056516295154,1.,0.951056516295154,1.,0.951056516295154,1.,0.951056516295154,
1.,0.951056516295154,1.,0.951056516295154,1.,0.951056516295154,1.,0.951056516295154,
1.,0.951056516295154,1.,0.951056516295154,1.,0.951056516295154,1.,0.951056516295154,
1.,0.951056516295154,1.,0.951056516295154,1.,0.951056516295154,1.,0.951056516295154,
1.,0.951056516295154,1.,0.951056516295154,1.,0.951056516295154,1.,0.951056516295154,
1.,0.951056516295154,1.,0.951056516295154,1.,0.951056516295154,1.,0.951056516295154,
1.,0.951056516295154,1.,0.951056516295154,1.,0.951056516295154,1.,0.951056516295154,
1.,0.951056516295154,1.,0.951056516295154,1.,0.951056516295154,1.,0.951056516295154,
1.,0.951056516295154,1.,0.951056516295154,1.,0.951056516295154,1.,0.951056516295154,
1.,0.951056516295154,1.,0.951056516295154,1.,0.951056516295154,1.,0.951056516295154,
1.,0.951056516295154,1.,0.951056516295154,1.,0.951056516295154,1.,0.951056516295154,
1.,0.951056516295154,1.,0.951056516295154,1.,0.951056516295154,1.,0.951056516295154,
1.,0.951056516295154,1.,0.951056516295154,1.,0.951056516295154,1.,0.951056516295154,
1.,0.951056516295154,1.,0.951056516295154,1.,0.951056516295154,1.,0.951056516295154,
1.,0.951056516295154,1.,0.951056516295154,1.,0.951056516295154,1.,0.951056516295154,
1.,0.951056516295154,1.,0.951056516295154,1.,0.951056516295154,1.,0.951056516295154,
1.,0.951056516295154,1.,0.951056516295154,1.,0.951056516295154,1.,0.951056516295154,
1.,0.951056516295154,1.,0.951056516295154,1.,0.951056516295154,1.,0.951056516295154,
1.,0.951056516295154,1.,0.951056516295154,1.,0.951056516295154,1.,0.951056516295154,
1.,0.951056516295154,1.,0.951056516295154,1.,0.951056516295154,1.,0.951056516295154,
1.,0.951056516295154,1.,0.951056516295154,1.,0.951056516295154,1.,0.951056516295154,
1.,0.951056516295154,1.,0.951056516295154,1.,0.951056516295154,1.,0.951056516295154,
1.,0.951056516295154,1.,0.951056516295154,1.,0.951056516295154,1.,0.951056516295154,
1.,0.951056516295154,1.,0.951056516295154,1.,0.951056516295154,1.,0.951056516295154,
1.,0.951056516295154,1.,0.951056516295154,1.,0.951056516295154,1.,0.951056516295154,
1.,0.951056516295154,1.,0.951056516295154,1.,0.951056516295154,1.,0.951056516295154,
1.,0.951056516295154,1.,0.951056516295154,1.,0.951056516295154,1.,0.951056516295154,
1.,0.951056516295154,1.,0.951056516295154,1.,0.951056516295154,1.,0.951056516295154,
1.,0.951056516295154,1.,0.951056516295154,1.,0.951056516295154,1.,0.951056516295154,
1.,0.951056516295154,1.,0.951056516295154,1.,0.951056516295154,1.,0.951056516295154,
1.,0.951056516295154,1.,0.951056516295154,1.,0.951056516295154,1.,0.951056516295154,
1.,0.951056516295154,1.,0.951056516295154,1.,0.951056516295154,1.,0.951056516295154,
1.,0.951056516295154,1.,0.951056516295154,1.,0.951056516295154,1.,0.951056516295154,
1.),(1.,0.951056516295154,1.,0.951056516295154,1.,0.951056516295154,1.,
0.951056516295154,1.,0.951056516295154,1.,0.951056516295154,1.,0.951056516295154,
1.,0.951056516295154,1.,0.951056516295154,1.,0.951056516295154,1.,0.951056516295154,
1.,0.951056516295154,1.,0.951056516295154,1.,0.951056516295154,1.,0.951056516295154,
1.,0.951056516295154,1.,0.951056516295154,1.,0.951056516295154,1.,0.951056516295154,
1.,0.951056516295154,1.,0.951056516295154,1.,0.951056516295154,1.,0.951056516295154,
1.,0.951056516295154,1.,0.951056516295154,1.,0.951056516295154,1.,0.951056516295154,
1.,0.951056516295154,1.,0.951056516295154,1.,0.951056516295154,1.,0.951056516295154,
1.,0.951056516295154,1.,0.951056516295154,1.,0.951056516295154,1.,0.951056516295154,
1.,0.951056516295154,1.,0.951056516295154,1.,0.951056516295154,1.,0.951056516295154,
1.,0.951056516295154,1.,0.951056516295154,1.,0.951056516295154,1.,0.951056516295154,
1.,0.951056516295154,1.,0.951056516295154,1.,0.951056516295154,1.,0.951056516295154,
1.,0.951056516295154,1.,0.951056516295154,1.,0.951056516295154,1.,0.951056516295154,
1.,0.951056516295154,1.,0.951056516295154,1.,0.951056516295154,1.,0.951056516295154,
1.,0.951056516295154,1.,0.951056516295154,1.,0.951056516295154,1.,0.951056516295154,
1.,0.951056516295154,1.,0.951056516295154,1.,0.951056516295154,1.,0.951056516295154,
1.,0.951056516295154,1.,0.951056516295154,1.,0.951056516295154,1.,0.951056516295154,
1.,0.951056516295154,1.,0.951056516295154,1.,0.951056516295154,1.,0.951056516295154,
1.,0.951056516295154,1.,0.951056516295154,1.,0.951056516295154,1.,0.951056516295154,
1.,0.951056516295154,1.,0.951056516295154,1.,0.951056516295154,1.,0.951056516295154,
1.,0.951056516295154,1.,0.951056516295154,1.,0.951056516295154,1.,0.951056516295154,
1.,0.951056516295154,1.,0.951056516295154,1.,0.951056516295154,1.,0.951056516295154,
1.,0.951056516295154,1.,0.951056516295154,1.,0.951056516295154,1.,0.951056516295154,
1.,0.951056516295154,1.,0.951056516295154,1.,0.951056516295154,1.,0.951056516295154,
1.,0.951056516295154,1.,0.951056516295154,1.,0.951056516295154,1.,0.951056516295154,
1.,0.951056516295154,1.,0.951056516295154,1.,0.951056516295154,1.,0.951056516295154,
1.,0.951056516295154,1.,0.951056516295154,1.,0.951056516295154,1.,0.951056516295154,
1.,0.951056516295154,1.,0.951056516295154,1.,0.951056516295154,1.,0.951056516295154,
1.,0.951056516295154,1.,0.951056516295154,1.,0.951056516295154,1.,0.951056516295154,
1.,0.951056516295154,1.,0.951056516295154,1.,0.951056516295154,1.,0.951056516295154,
1.,0.951056516295154,1.,0.951056516295154,1.,0.951056516295154,1.,0.951056516295154,
1.,0.951056516295154,1.,0.951056516295154,1.,0.951056516295154,1.,0.951056516295154,
1.,0.951056516295154,1.,0.951056516295154,1.,0.951056516295154,1.,0.951056516295154,
1.,0.951056516295154,1.,0.951056516295154,1.,0.951056516295154,1.,0.951056516295154,
1.,0.951056516295154,1.,0.951056516295154,1.,0.951056516295154,1.,0.951056516295154,
1.,0.951056516295154,1.,0.951056516295154,1.,0.951056516295154,1.,0.951056516295154,
1.,0.951056516295154,1.,0.951056516295154,1.,0.951056516295154,1.,0.951056516295154,
1.,0.951056516295154,1.,0.951056516295154,1.,0.951056516295154,1.,0.951056516295154,
1.,0.951056516295154,1.,0.951056516295154,1.,0.951056516295154,1.,0.951056516295154,
1.,0.951056516295154,1.,0.951056516295154,1.,0.951056516295154,1.,0.951056516295154,
1.,0.951056516295154,1.,0.951056516295154,1.,0.951056516295154,1.,0.951056516295154,
1.,0.951056516295154,1.,0.951056516295154,1.,0.951056516295154,1.,0.951056516295154,
1.,0.951056516295154,1.,0.951056516295154,1.,0.951056516295154,1.,0.951056516295154,
1.,0.951056516295154,1.,0.951056516295154,1.,0.951056516295154,1.,0.951056516295154,
1.,0.951056516295154,1.,0.951056516295154,1.,0.951056516295154,1.,0.951056516295154,
1.,0.951056516295154,1.,0.951056516295154,1.,0.951056516295154,1.,0.951056516295154,
1.,0.951056516295154,1.,0.951056516295154,1.,0.951056516295154,1.,0.951056516295154,
1.,0.951056516295154,1.,0.951056516295154,1.,0.951056516295154,1.,0.951056516295154,
1.,0.951056516295154,1.,0.951056516295154,1.,0.951056516295154,1.,0.951056516295154,
1.,0.951056516295154,1.,0.951056516295154,1.,0.951056516295154,1.,0.951056516295154,
1.,0.951056516295154,1.,0.951056516295154,1.,0.951056516295154,1.,0.951056516295154,
1.,0.951056516295154,1.,0.951056516295154,1.,0.951056516295154,1.,0.951056516295154,
1.,0.951056516295154,1.,0.951056516295154,1.,0.951056516295154,1.,0.951056516295154,
1.,0.951056516295154,1.,0.951056516295154,1.,0.951056516295154,1.,0.951056516295154,
1.,0.951056516295154,1.,0.951056516295154,1.,0.951056516295154,1.,0.951056516295154,
1.,0.951056516295154,1.,0.951056516295154,1.,0.951056516295154,1.,0.951056516295154,
1.,0.951056516295154,1.,0.951056516295154,1.,0.951056516295154,1.,0.951056516295154,
1.,0.951056516295154,1.,0.951056516295154,1.,0.951056516295154,1.,0.951056516295154,
1.,0.951056516295154,1.,0.951056516295154,1.,0.951056516295154,1.,0.951056516295154,
1.,0.951056516295154,1.,0.951056516295154,1.,0.951056516295154,1.,0.951056516295154,
1.,0.951056516295154,1.,0.951056516295154,1.,0.951056516295154,1.,0.951056516295154,
1.,0.951056516295154,1.,0.951056516295154,1.,0.951056516295154,1.,0.951056516295154,
1.,0.951056516295154,1.,0.951056516295154,1.,0.951056516295154,1.,0.951056516295154,
1.,0.951056516295154,1.,0.951056516295154,1.,0.951056516295154,1.,0.951056516295154,
1.,0.951056516295154,1.,0.951056516295154,1.,0.951056516295154,1.,0.951056516295154,
1.,0.951056516295154,1.,0.951056516295154,1.,0.951056516295154,1.,0.951056516295154,
1.,0.951056516295154,1.,0.951056516295154,1.,0.951056516295154,1.,0.951056516295154,
1.,0.951056516295154,1.,0.951056516295154,1.,0.951056516295154,1.,0.951056516295154,
1.,0.951056516295154,1.,0.951056516295154,1.,0.951056516295154,1.,0.951056516295154,
1.,0.951056516295154,1.,0.951056516295154,1.,0.951056516295154,1.,0.951056516295154,
1.,0.951056516295154,1.,0.951056516295154,1.,0.951056516295154,1.,0.951056516295154,
1.,0.951056516295154,1.,0.951056516295154,1.,0.951056516295154,1.,0.951056516295154,
1.,0.951056516295154,1.,0.951056516295154,1.,0.951056516295154,1.,0.951056516295154,
1.,0.951056516295154,1.,0.951056516295154,1.,0.951056516295154,1.,0.951056516295154,
1.,0.951056516295154,1.,0.951056516295154,1.,0.951056516295154,1.,0.951056516295154,
1.,0.951056516295154,1.,0.951056516295154,1.,0.951056516295154,1.,0.951056516295154,
1.,0.951056516295154,1.,0.951056516295154,1.,0.951056516295154,1.,0.951056516295154,
1.,0.951056516295154,1.,0.951056516295154,1.,0.951056516295154,1.,0.951056516295154,
1.,0.951056516295154,1.,0.951056516295154,1.,0.951056516295154,1.,0.951056516295154,
1.,0.951056516295154,1.,0.951056516295154,1.,0.951056516295154,1.,0.951056516295154,
1.,0.951056516295154,1.,0.951056516295154,1.,0.951056516295154,1.,0.951056516295154,
1.,0.951056516295154,1.,0.951056516295154,1.,0.951056516295154,1.,0.951056516295154,
1.,0.951056516295154,1.,0.951056516295154,1.,0.951056516295154,1.,0.951056516295154,
1.,0.951056516295154,1.,0.951056516295154,1.,0.951056516295154,1.,0.951056516295154,
1.,0.951056516295154,1.,0.951056516295154,1.,0.951056516295154,1.,0.951056516295154,
1.,0.951056516295154,1.,0.951056516295154,1.,0.951056516295154,1.,0.951056516295154,
1.,0.951056516295154,1.,0.951056516295154,1.,0.951056516295154,1.,0.951056516295154,
1.,0.951056516295154,1.,0.951056516295154,1.,0.951056516295154,1.,0.951056516295154,
1.,0.951056516295154,1.,0.951056516295154,1.,0.951056516295154,1.,0.951056516295154,
1.,0.951056516295154,1.,0.951056516295154,1.,0.951056516295154,1.,0.951056516295154,
1.,0.951056516295154,1.,0.951056516295154,1.,0.951056516295154,1.,0.951056516295154,
1.,0.951056516295154,1.,0.951056516295154,1.,0.951056516295154,1.,0.951056516295154,
1.,0.951056516295154,1.,0.951056516295154,1.,0.951056516295154,1.,0.951056516295154,
1.,0.951056516295154,1.,0.951056516295154,1.,0.951056516295154,1.,0.951056516295154,
1.,0.951056516295154,1.,0.951056516295154,1.,0.951056516295154,1.,0.951056516295154,
1.,0.951056516295154,1.,0.951056516295154,1.,0.951056516295154,1.,0.951056516295154,
1.,0.951056516295154,1.,0.951056516295154,1.,0.951056516295154,1.,0.951056516295154,
1.,0.951056516295154,1.,0.951056516295154,1.,0.951056516295154,1.,0.951056516295154,
1.,0.951056516295154,1.,0.951056516295154,1.,0.951056516295154,1.,0.951056516295154,
1.,0.951056516295154,1.,0.951056516295154,1.,0.951056516295154,1.,0.951056516295154,
1.,0.951056516295154,1.,0.951056516295154,1.,0.951056516295154,1.,0.951056516295154,
1.,0.951056516295154,1.,0.951056516295154,1.,0.951056516295154,1.,0.951056516295154,
1.,0.951056516295154,1.,0.951056516295154,1.,0.951056516295154,1.,0.951056516295154,
1.,0.951056516295154,1.,0.951056516295154,1.,0.951056516295154,1.,0.951056516295154,
1.,0.951056516295154,1.,0.951056516295154,1.,0.951056516295154,1.,0.951056516295154,
1.,0.951056516295154,1.,0.951056516295154,1.,0.951056516295154,1.,0.951056516295154,
1.,0.951056516295154,1.,0.951056516295154,1.,0.951056516295154,1.,0.951056516295154,
1.,0.951056516295154,1.,0.951056516295154,1.,0.951056516295154,1.,0.951056516295154,
1.,0.951056516295154,1.,0.951056516295154,1.,0.951056516295154,1.,0.951056516295154,
1.,0.951056516295154,1.,0.951056516295154,1.,0.951056516295154,1.,0.951056516295154,
1.,0.951056516295154,1.,0.951056516295154,1.,0.951056516295154,1.,0.951056516295154,
1.,0.951056516295154,1.,0.951056516295154,1.,0.951056516295154,1.,0.951056516295154,
1.,0.951056516295154,1.,0.951056516295154,1.,0.951056516295154,1.,0.951056516295154,
1.,0.951056516295154,1.,0.951056516295154,1.,0.951056516295154,1.,0.951056516295154,
1.,0.951056516295154,1.,0.951056516295154,1.,0.951056516295154,1.,0.951056516295154,
1.,0.951056516295154,1.,0.951056516295154,1.,0.951056516295154,1.,0.951056516295154,
1.,0.951056516295154,1.,0.951056516295154,1.,0.951056516295154,1.,0.951056516295154,
1.,0.951056516295154,1.,0.951056516295154,1.,0.951056516295154,1.,0.951056516295154,
1.,0.951056516295154,1.,0.951056516295154,1.,0.951056516295154,1.,0.951056516295154,
1.,0.951056516295154,1.,0.951056516295154,1.,0.951056516295154,1.,0.951056516295154,
1.,0.951056516295154,1.,0.951056516295154,1.,0.951056516295154,1.,0.951056516295154,
1.,0.951056516295154,1.,0.951056516295154,1.,0.951056516295154,1.,0.951056516295154,
1.,0.951056516295154,1.,0.951056516295154,1.,0.951056516295154,1.,0.951056516295154,
1.,0.951056516295154,1.,0.951056516295154,1.,0.951056516295154,1.,0.951056516295154,
1.,0.951056516295154,1.,0.951056516295154,1.,0.951056516295154,1.,0.951056516295154,
1.,0.951056516295154,1.,0.951056516295154,1.,0.951056516295154,1.,0.951056516295154,
1.,0.951056516295154,1.,0.951056516295154,1.,0.951056516295154,1.,0.951056516295154,
1.,0.951056516295154,1.,0.951056516295154,1.,0.951056516295154,1.,0.951056516295154,
1.,0.951056516295154,1.,0.951056516295154,1.,0.951056516295154,1.,0.951056516295154,
1.,0.951056516295154,1.,0.951056516295154,1.,0.951056516295154,1.)))
REPRESENTATION_ITEM('')
SURFACE()
);
#3198=(
BOUNDED_SURFACE()
B_SPLINE_SURFACE(1,2,((#294054,#294055,#294056,#294057,#294058,#294059,
#294060,#294061,#294062,#294063,#294064,#294065,#294066,#294067,#294068,
#294069,#294070,#294071,#294072,#294073,#294074,#294075,#294076,#294077,
#294078,#294079,#294080,#294081,#294082,#294083,#294084,#294085,#294086,
#294087,#294088,#294089,#294090,#294091,#294092,#294093,#294094,#294095,
#294096,#294097,#294098,#294099,#294100,#294101,#294102,#294103,#294104,
#294105,#294106,#294107,#294108,#294109,#294110,#294111,#294112,#294113,
#294114,#294115,#294116,#294117,#294118,#294119,#294120,#294121,#294122,
#294123,#294124,#294125,#294126,#294127,#294128,#294129,#294130,#294131,
#294132,#294133,#294134,#294135,#294136,#294137,#294138,#294139,#294140,
#294141,#294142,#294143,#294144,#294145,#294146,#294147,#294148,#294149,
#294150,#294151,#294152,#294153,#294154,#294155,#294156,#294157,#294158,
#294159,#294160,#294161,#294162,#294163,#294164,#294165,#294166,#294167,
#294168,#294169,#294170,#294171,#294172,#294173,#294174,#294175,#294176,
#294177,#294178,#294179,#294180,#294181,#294182,#294183,#294184,#294185,
#294186,#294187,#294188,#294189,#294190,#294191,#294192,#294193,#294194,
#294195,#294196,#294197,#294198,#294199,#294200,#294201,#294202,#294203,
#294204,#294205,#294206,#294207,#294208,#294209,#294210,#294211,#294212,
#294213,#294214,#294215,#294216,#294217,#294218,#294219,#294220,#294221,
#294222,#294223,#294224,#294225,#294226,#294227,#294228,#294229,#294230,
#294231,#294232,#294233,#294234,#294235,#294236,#294237,#294238,#294239,
#294240,#294241,#294242,#294243,#294244,#294245,#294246,#294247,#294248,
#294249,#294250,#294251,#294252,#294253,#294254,#294255,#294256,#294257,
#294258,#294259,#294260,#294261,#294262,#294263,#294264,#294265,#294266,
#294267,#294268,#294269,#294270,#294271,#294272,#294273,#294274,#294275,
#294276,#294277,#294278,#294279,#294280,#294281,#294282,#294283,#294284,
#294285,#294286,#294287,#294288,#294289,#294290,#294291,#294292,#294293,
#294294,#294295,#294296,#294297,#294298,#294299,#294300,#294301,#294302,
#294303,#294304,#294305,#294306,#294307,#294308,#294309,#294310,#294311,
#294312,#294313,#294314,#294315,#294316,#294317,#294318,#294319,#294320,
#294321,#294322,#294323,#294324,#294325,#294326,#294327,#294328,#294329,
#294330,#294331,#294332,#294333,#294334,#294335,#294336,#294337,#294338,
#294339,#294340,#294341,#294342,#294343,#294344,#294345,#294346,#294347,
#294348,#294349,#294350,#294351,#294352,#294353,#294354,#294355,#294356,
#294357,#294358,#294359,#294360,#294361,#294362,#294363,#294364,#294365,
#294366,#294367,#294368,#294369,#294370,#294371,#294372,#294373,#294374,
#294375,#294376,#294377,#294378,#294379,#294380,#294381,#294382,#294383,
#294384,#294385,#294386,#294387,#294388,#294389,#294390,#294391,#294392,
#294393,#294394,#294395,#294396,#294397,#294398,#294399,#294400,#294401,
#294402,#294403,#294404,#294405,#294406,#294407,#294408,#294409,#294410,
#294411,#294412,#294413,#294414,#294415,#294416,#294417,#294418,#294419,
#294420,#294421,#294422,#294423,#294424,#294425,#294426,#294427,#294428,
#294429,#294430,#294431,#294432,#294433,#294434,#294435,#294436,#294437,
#294438,#294439,#294440,#294441,#294442,#294443,#294444,#294445,#294446,
#294447,#294448,#294449,#294450,#294451,#294452,#294453,#294454,#294455,
#294456,#294457,#294458,#294459,#294460,#294461,#294462,#294463,#294464,
#294465,#294466,#294467,#294468,#294469,#294470,#294471,#294472,#294473,
#294474,#294475,#294476,#294477,#294478,#294479,#294480,#294481,#294482,
#294483,#294484,#294485,#294486,#294487,#294488,#294489,#294490,#294491,
#294492,#294493,#294494,#294495,#294496,#294497,#294498,#294499,#294500,
#294501,#294502,#294503,#294504,#294505,#294506,#294507,#294508,#294509,
#294510,#294511,#294512,#294513,#294514,#294515,#294516,#294517,#294518,
#294519,#294520,#294521,#294522,#294523,#294524,#294525,#294526,#294527,
#294528,#294529,#294530,#294531,#294532,#294533,#294534,#294535,#294536,
#294537,#294538,#294539,#294540,#294541,#294542,#294543,#294544,#294545,
#294546,#294547,#294548,#294549,#294550,#294551,#294552,#294553,#294554,
#294555,#294556,#294557,#294558,#294559,#294560,#294561,#294562,#294563,
#294564,#294565,#294566,#294567,#294568,#294569,#294570,#294571,#294572,
#294573,#294574,#294575,#294576,#294577,#294578,#294579,#294580,#294581,
#294582,#294583,#294584,#294585,#294586,#294587,#294588,#294589,#294590,
#294591,#294592,#294593,#294594,#294595,#294596,#294597,#294598,#294599,
#294600,#294601,#294602,#294603,#294604,#294605,#294606,#294607,#294608,
#294609,#294610,#294611,#294612,#294613,#294614,#294615,#294616,#294617,
#294618,#294619,#294620,#294621,#294622,#294623,#294624,#294625,#294626,
#294627,#294628,#294629,#294630,#294631,#294632,#294633,#294634,#294635,
#294636,#294637,#294638,#294639,#294640,#294641,#294642,#294643,#294644,
#294645,#294646,#294647,#294648,#294649,#294650,#294651,#294652,#294653,
#294654,#294655,#294656,#294657,#294658,#294659,#294660,#294661,#294662,
#294663,#294664,#294665,#294666,#294667,#294668,#294669,#294670,#294671,
#294672,#294673,#294674,#294675,#294676,#294677,#294678,#294679,#294680,
#294681,#294682,#294683,#294684,#294685,#294686,#294687,#294688,#294689,
#294690,#294691,#294692,#294693,#294694,#294695,#294696,#294697,#294698,
#294699,#294700,#294701,#294702,#294703,#294704,#294705,#294706,#294707,
#294708,#294709,#294710,#294711,#294712,#294713,#294714,#294715,#294716,
#294717,#294718,#294719,#294720,#294721,#294722,#294723,#294724,#294725,
#294726,#294727,#294728,#294729,#294730,#294731,#294732,#294733,#294734,
#294735,#294736,#294737,#294738,#294739,#294740,#294741,#294742,#294743,
#294744,#294745,#294746,#294747,#294748,#294749,#294750,#294751,#294752,
#294753,#294754,#294755,#294756,#294757,#294758,#294759,#294760,#294761,
#294762,#294763,#294764,#294765,#294766,#294767,#294768,#294769,#294770,
#294771,#294772,#294773,#294774,#294775,#294776,#294777,#294778,#294779,
#294780,#294781,#294782,#294783,#294784,#294785,#294786,#294787,#294788,
#294789,#294790,#294791,#294792,#294793,#294794,#294795,#294796,#294797,
#294798,#294799,#294800,#294801,#294802,#294803,#294804,#294805,#294806,
#294807,#294808,#294809,#294810,#294811,#294812,#294813,#294814,#294815,
#294816,#294817,#294818,#294819,#294820,#294821,#294822,#294823,#294824,
#294825,#294826,#294827,#294828,#294829,#294830,#294831,#294832,#294833,
#294834,#294835,#294836,#294837,#294838,#294839,#294840,#294841,#294842,
#294843,#294844,#294845,#294846,#294847,#294848,#294849,#294850,#294851,
#294852,#294853,#294854,#294855,#294856,#294857,#294858,#294859,#294860,
#294861,#294862,#294863,#294864,#294865,#294866,#294867,#294868,#294869,
#294870,#294871,#294872,#294873,#294874,#294875,#294876,#294877,#294878,
#294879,#294880,#294881,#294882,#294883,#294884,#294885,#294886,#294887,
#294888,#294889,#294890,#294891,#294892,#294893,#294894,#294895,#294896,
#294897,#294898,#294899,#294900,#294901,#294902,#294903,#294904,#294905,
#294906,#294907,#294908,#294909,#294910,#294911,#294912,#294913,#294914,
#294915,#294916,#294917,#294918,#294919,#294920,#294921,#294922,#294923,
#294924,#294925,#294926,#294927,#294928,#294929,#294930,#294931,#294932,
#294933,#294934,#294935,#294936,#294937,#294938,#294939,#294940,#294941,
#294942,#294943,#294944,#294945,#294946,#294947,#294948,#294949,#294950,
#294951,#294952,#294953,#294954,#294955,#294956,#294957,#294958,#294959,
#294960,#294961,#294962,#294963,#294964,#294965,#294966,#294967,#294968,
#294969,#294970,#294971,#294972,#294973,#294974,#294975,#294976,#294977,
#294978,#294979,#294980,#294981,#294982,#294983,#294984,#294985,#294986,
#294987,#294988,#294989,#294990,#294991,#294992,#294993,#294994,#294995,
#294996,#294997,#294998,#294999,#295000,#295001,#295002,#295003,#295004,
#295005,#295006,#295007,#295008,#295009,#295010,#295011,#295012,#295013,
#295014,#295015,#295016,#295017,#295018,#295019,#295020,#295021,#295022,
#295023,#295024,#295025,#295026,#295027,#295028,#295029,#295030,#295031,
#295032,#295033,#295034,#295035,#295036,#295037,#295038,#295039,#295040,
#295041,#295042,#295043,#295044,#295045,#295046,#295047,#295048,#295049,
#295050,#295051,#295052,#295053,#295054,#295055,#295056,#295057,#295058,
#295059,#295060,#295061,#295062,#295063,#295064,#295065,#295066,#295067,
#295068,#295069,#295070,#295071,#295072,#295073,#295074,#295075,#295076,
#295077,#295078,#295079,#295080,#295081,#295082,#295083,#295084,#295085,
#295086,#295087,#295088,#295089,#295090),(#295091,#295092,#295093,#295094,
#295095,#295096,#295097,#295098,#295099,#295100,#295101,#295102,#295103,
#295104,#295105,#295106,#295107,#295108,#295109,#295110,#295111,#295112,
#295113,#295114,#295115,#295116,#295117,#295118,#295119,#295120,#295121,
#295122,#295123,#295124,#295125,#295126,#295127,#295128,#295129,#295130,
#295131,#295132,#295133,#295134,#295135,#295136,#295137,#295138,#295139,
#295140,#295141,#295142,#295143,#295144,#295145,#295146,#295147,#295148,
#295149,#295150,#295151,#295152,#295153,#295154,#295155,#295156,#295157,
#295158,#295159,#295160,#295161,#295162,#295163,#295164,#295165,#295166,
#295167,#295168,#295169,#295170,#295171,#295172,#295173,#295174,#295175,
#295176,#295177,#295178,#295179,#295180,#295181,#295182,#295183,#295184,
#295185,#295186,#295187,#295188,#295189,#295190,#295191,#295192,#295193,
#295194,#295195,#295196,#295197,#295198,#295199,#295200,#295201,#295202,
#295203,#295204,#295205,#295206,#295207,#295208,#295209,#295210,#295211,
#295212,#295213,#295214,#295215,#295216,#295217,#295218,#295219,#295220,
#295221,#295222,#295223,#295224,#295225,#295226,#295227,#295228,#295229,
#295230,#295231,#295232,#295233,#295234,#295235,#295236,#295237,#295238,
#295239,#295240,#295241,#295242,#295243,#295244,#295245,#295246,#295247,
#295248,#295249,#295250,#295251,#295252,#295253,#295254,#295255,#295256,
#295257,#295258,#295259,#295260,#295261,#295262,#295263,#295264,#295265,
#295266,#295267,#295268,#295269,#295270,#295271,#295272,#295273,#295274,
#295275,#295276,#295277,#295278,#295279,#295280,#295281,#295282,#295283,
#295284,#295285,#295286,#295287,#295288,#295289,#295290,#295291,#295292,
#295293,#295294,#295295,#295296,#295297,#295298,#295299,#295300,#295301,
#295302,#295303,#295304,#295305,#295306,#295307,#295308,#295309,#295310,
#295311,#295312,#295313,#295314,#295315,#295316,#295317,#295318,#295319,
#295320,#295321,#295322,#295323,#295324,#295325,#295326,#295327,#295328,
#295329,#295330,#295331,#295332,#295333,#295334,#295335,#295336,#295337,
#295338,#295339,#295340,#295341,#295342,#295343,#295344,#295345,#295346,
#295347,#295348,#295349,#295350,#295351,#295352,#295353,#295354,#295355,
#295356,#295357,#295358,#295359,#295360,#295361,#295362,#295363,#295364,
#295365,#295366,#295367,#295368,#295369,#295370,#295371,#295372,#295373,
#295374,#295375,#295376,#295377,#295378,#295379,#295380,#295381,#295382,
#295383,#295384,#295385,#295386,#295387,#295388,#295389,#295390,#295391,
#295392,#295393,#295394,#295395,#295396,#295397,#295398,#295399,#295400,
#295401,#295402,#295403,#295404,#295405,#295406,#295407,#295408,#295409,
#295410,#295411,#295412,#295413,#295414,#295415,#295416,#295417,#295418,
#295419,#295420,#295421,#295422,#295423,#295424,#295425,#295426,#295427,
#295428,#295429,#295430,#295431,#295432,#295433,#295434,#295435,#295436,
#295437,#295438,#295439,#295440,#295441,#295442,#295443,#295444,#295445,
#295446,#295447,#295448,#295449,#295450,#295451,#295452,#295453,#295454,
#295455,#295456,#295457,#295458,#295459,#295460,#295461,#295462,#295463,
#295464,#295465,#295466,#295467,#295468,#295469,#295470,#295471,#295472,
#295473,#295474,#295475,#295476,#295477,#295478,#295479,#295480,#295481,
#295482,#295483,#295484,#295485,#295486,#295487,#295488,#295489,#295490,
#295491,#295492,#295493,#295494,#295495,#295496,#295497,#295498,#295499,
#295500,#295501,#295502,#295503,#295504,#295505,#295506,#295507,#295508,
#295509,#295510,#295511,#295512,#295513,#295514,#295515,#295516,#295517,
#295518,#295519,#295520,#295521,#295522,#295523,#295524,#295525,#295526,
#295527,#295528,#295529,#295530,#295531,#295532,#295533,#295534,#295535,
#295536,#295537,#295538,#295539,#295540,#295541,#295542,#295543,#295544,
#295545,#295546,#295547,#295548,#295549,#295550,#295551,#295552,#295553,
#295554,#295555,#295556,#295557,#295558,#295559,#295560,#295561,#295562,
#295563,#295564,#295565,#295566,#295567,#295568,#295569,#295570,#295571,
#295572,#295573,#295574,#295575,#295576,#295577,#295578,#295579,#295580,
#295581,#295582,#295583,#295584,#295585,#295586,#295587,#295588,#295589,
#295590,#295591,#295592,#295593,#295594,#295595,#295596,#295597,#295598,
#295599,#295600,#295601,#295602,#295603,#295604,#295605,#295606,#295607,
#295608,#295609,#295610,#295611,#295612,#295613,#295614,#295615,#295616,
#295617,#295618,#295619,#295620,#295621,#295622,#295623,#295624,#295625,
#295626,#295627,#295628,#295629,#295630,#295631,#295632,#295633,#295634,
#295635,#295636,#295637,#295638,#295639,#295640,#295641,#295642,#295643,
#295644,#295645,#295646,#295647,#295648,#295649,#295650,#295651,#295652,
#295653,#295654,#295655,#295656,#295657,#295658,#295659,#295660,#295661,
#295662,#295663,#295664,#295665,#295666,#295667,#295668,#295669,#295670,
#295671,#295672,#295673,#295674,#295675,#295676,#295677,#295678,#295679,
#295680,#295681,#295682,#295683,#295684,#295685,#295686,#295687,#295688,
#295689,#295690,#295691,#295692,#295693,#295694,#295695,#295696,#295697,
#295698,#295699,#295700,#295701,#295702,#295703,#295704,#295705,#295706,
#295707,#295708,#295709,#295710,#295711,#295712,#295713,#295714,#295715,
#295716,#295717,#295718,#295719,#295720,#295721,#295722,#295723,#295724,
#295725,#295726,#295727,#295728,#295729,#295730,#295731,#295732,#295733,
#295734,#295735,#295736,#295737,#295738,#295739,#295740,#295741,#295742,
#295743,#295744,#295745,#295746,#295747,#295748,#295749,#295750,#295751,
#295752,#295753,#295754,#295755,#295756,#295757,#295758,#295759,#295760,
#295761,#295762,#295763,#295764,#295765,#295766,#295767,#295768,#295769,
#295770,#295771,#295772,#295773,#295774,#295775,#295776,#295777,#295778,
#295779,#295780,#295781,#295782,#295783,#295784,#295785,#295786,#295787,
#295788,#295789,#295790,#295791,#295792,#295793,#295794,#295795,#295796,
#295797,#295798,#295799,#295800,#295801,#295802,#295803,#295804,#295805,
#295806,#295807,#295808,#295809,#295810,#295811,#295812,#295813,#295814,
#295815,#295816,#295817,#295818,#295819,#295820,#295821,#295822,#295823,
#295824,#295825,#295826,#295827,#295828,#295829,#295830,#295831,#295832,
#295833,#295834,#295835,#295836,#295837,#295838,#295839,#295840,#295841,
#295842,#295843,#295844,#295845,#295846,#295847,#295848,#295849,#295850,
#295851,#295852,#295853,#295854,#295855,#295856,#295857,#295858,#295859,
#295860,#295861,#295862,#295863,#295864,#295865,#295866,#295867,#295868,
#295869,#295870,#295871,#295872,#295873,#295874,#295875,#295876,#295877,
#295878,#295879,#295880,#295881,#295882,#295883,#295884,#295885,#295886,
#295887,#295888,#295889,#295890,#295891,#295892,#295893,#295894,#295895,
#295896,#295897,#295898,#295899,#295900,#295901,#295902,#295903,#295904,
#295905,#295906,#295907,#295908,#295909,#295910,#295911,#295912,#295913,
#295914,#295915,#295916,#295917,#295918,#295919,#295920,#295921,#295922,
#295923,#295924,#295925,#295926,#295927,#295928,#295929,#295930,#295931,
#295932,#295933,#295934,#295935,#295936,#295937,#295938,#295939,#295940,
#295941,#295942,#295943,#295944,#295945,#295946,#295947,#295948,#295949,
#295950,#295951,#295952,#295953,#295954,#295955,#295956,#295957,#295958,
#295959,#295960,#295961,#295962,#295963,#295964,#295965,#295966,#295967,
#295968,#295969,#295970,#295971,#295972,#295973,#295974,#295975,#295976,
#295977,#295978,#295979,#295980,#295981,#295982,#295983,#295984,#295985,
#295986,#295987,#295988,#295989,#295990,#295991,#295992,#295993,#295994,
#295995,#295996,#295997,#295998,#295999,#296000,#296001,#296002,#296003,
#296004,#296005,#296006,#296007,#296008,#296009,#296010,#296011,#296012,
#296013,#296014,#296015,#296016,#296017,#296018,#296019,#296020,#296021,
#296022,#296023,#296024,#296025,#296026,#296027,#296028,#296029,#296030,
#296031,#296032,#296033,#296034,#296035,#296036,#296037,#296038,#296039,
#296040,#296041,#296042,#296043,#296044,#296045,#296046,#296047,#296048,
#296049,#296050,#296051,#296052,#296053,#296054,#296055,#296056,#296057,
#296058,#296059,#296060,#296061,#296062,#296063,#296064,#296065,#296066,
#296067,#296068,#296069,#296070,#296071,#296072,#296073,#296074,#296075,
#296076,#296077,#296078,#296079,#296080,#296081,#296082,#296083,#296084,
#296085,#296086,#296087,#296088,#296089,#296090,#296091,#296092,#296093,
#296094,#296095,#296096,#296097,#296098,#296099,#296100,#296101,#296102,
#296103,#296104,#296105,#296106,#296107,#296108,#296109,#296110,#296111,
#296112,#296113,#296114,#296115,#296116,#296117,#296118,#296119,#296120,
#296121,#296122,#296123,#296124,#296125,#296126,#296127)),.UNSPECIFIED.,
 .F.,.F.,.F.)
B_SPLINE_SURFACE_WITH_KNOTS((2,2),(3,2,2,2,2,2,2,2,2,2,2,2,2,2,2,2,2,2,
2,2,2,2,2,2,2,2,2,2,2,2,2,2,2,2,2,2,2,2,2,2,2,2,2,2,2,2,2,2,2,2,2,2,2,2,
2,2,2,2,2,2,2,2,2,2,2,2,2,2,2,2,2,2,2,2,2,2,2,2,2,2,2,2,2,2,2,2,2,2,2,2,
2,2,2,2,2,2,2,2,2,2,2,2,2,2,2,2,2,2,2,2,2,2,2,2,2,2,2,2,2,2,2,2,2,2,2,2,
2,2,2,2,2,2,2,2,2,2,2,2,2,2,2,2,2,2,2,2,2,2,2,2,2,2,2,2,2,2,2,2,2,2,2,2,
2,2,2,2,2,2,2,2,2,2,2,2,2,2,2,2,2,2,2,2,2,2,2,2,2,2,2,2,2,2,2,2,2,2,2,2,
2,2,2,2,2,2,2,2,2,2,2,2,2,2,2,2,2,2,2,2,2,2,2,2,2,2,2,2,2,2,2,2,2,2,2,2,
2,2,2,2,2,2,2,2,2,2,2,2,2,2,2,2,2,2,2,2,2,2,2,2,2,2,2,2,2,2,2,2,2,2,2,2,
2,2,2,2,2,2,2,2,2,2,2,2,2,2,2,2,2,2,2,2,2,2,2,2,2,2,2,2,2,2,2,2,2,2,2,2,
2,2,2,2,2,2,2,2,2,2,2,2,2,2,2,2,2,2,2,2,2,2,2,2,2,2,2,2,2,2,2,2,2,2,2,2,
2,2,2,2,2,2,2,2,2,2,2,2,2,2,2,2,2,2,2,2,2,2,2,2,2,2,2,2,2,2,2,2,2,2,2,2,
2,2,2,2,2,2,2,2,2,2,2,2,2,2,2,2,2,2,2,2,2,2,2,2,2,2,2,2,2,2,2,2,2,2,2,2,
2,2,2,2,2,2,2,2,2,2,2,2,2,2,2,2,2,2,2,2,2,2,2,2,2,2,2,2,2,2,2,2,2,2,2,2,
2,2,2,2,2,2,2,2,2,2,2,2,2,2,2,2,2,2,2,2,2,2,2,2,2,2,2,2,2,2,2,2,2,2,2,2,
2,2,2,2,2,2,2,2,2,2,2,2,2,2,2,2,2,2,2,2,2,2,2,2,2,2,2,2,2,2,2,2,3),(0.,
1.),(0.,0.00192307692307692,0.00384615384615385,0.00576923076923077,0.00769230769230769,
0.00961538461538462,0.0115384615384615,0.0134615384615385,0.0153846153846154,
0.0173076923076923,0.0192307692307692,0.0211538461538462,0.0230769230769231,
0.025,0.0269230769230769,0.0288461538461538,0.0307692307692308,0.0326923076923077,
0.0346153846153846,0.0365384615384615,0.0384615384615385,0.0403846153846154,
0.0423076923076923,0.0442307692307692,0.0461538461538462,0.0480769230769231,
0.05,0.0519230769230769,0.0538461538461538,0.0557692307692308,0.0576923076923077,
0.0596153846153846,0.0615384615384615,0.0634615384615385,0.0653846153846154,
0.0673076923076923,0.0692307692307692,0.0711538461538462,0.0730769230769231,
0.075,0.0769230769230769,0.0788461538461538,0.0807692307692308,0.0826923076923077,
0.0846153846153846,0.0865384615384615,0.0884615384615385,0.0903846153846154,
0.0923076923076923,0.0942307692307692,0.0961538461538462,0.0980769230769231,
0.1,0.101923076923077,0.103846153846154,0.105769230769231,0.107692307692308,
0.109615384615385,0.111538461538462,0.113461538461538,0.115384615384615,
0.117307692307692,0.119230769230769,0.121153846153846,0.123076923076923,
0.125,0.126923076923077,0.128846153846154,0.130769230769231,0.132692307692308,
0.134615384615385,0.136538461538462,0.138461538461538,0.140384615384615,
0.142307692307692,0.144230769230769,0.146153846153846,0.148076923076923,
0.15,0.151923076923077,0.153846153846154,0.155769230769231,0.157692307692308,
0.159615384615385,0.161538461538462,0.163461538461538,0.165384615384615,
0.167307692307692,0.169230769230769,0.171153846153846,0.173076923076923,
0.175,0.176923076923077,0.178846153846154,0.180769230769231,0.182692307692308,
0.184615384615385,0.186538461538462,0.188461538461538,0.190384615384615,
0.192307692307692,0.194230769230769,0.196153846153846,0.198076923076923,
0.2,0.201923076923077,0.203846153846154,0.205769230769231,0.207692307692308,
0.209615384615385,0.211538461538462,0.213461538461538,0.215384615384615,
0.217307692307692,0.219230769230769,0.221153846153846,0.223076923076923,
0.225,0.226923076923077,0.228846153846154,0.230769230769231,0.232692307692308,
0.234615384615385,0.236538461538462,0.238461538461538,0.240384615384615,
0.242307692307692,0.244230769230769,0.246153846153846,0.248076923076923,
0.25,0.251923076923077,0.253846153846154,0.255769230769231,0.257692307692308,
0.259615384615385,0.261538461538462,0.263461538461538,0.265384615384615,
0.267307692307692,0.269230769230769,0.271153846153846,0.273076923076923,
0.275,0.276923076923077,0.278846153846154,0.280769230769231,0.282692307692308,
0.284615384615385,0.286538461538462,0.288461538461538,0.290384615384615,
0.292307692307692,0.294230769230769,0.296153846153846,0.298076923076923,
0.3,0.301923076923077,0.303846153846154,0.305769230769231,0.307692307692308,
0.309615384615385,0.311538461538462,0.313461538461538,0.315384615384615,
0.317307692307692,0.319230769230769,0.321153846153846,0.323076923076923,
0.325,0.326923076923077,0.328846153846154,0.330769230769231,0.332692307692308,
0.334615384615385,0.336538461538462,0.338461538461538,0.340384615384615,
0.342307692307692,0.344230769230769,0.346153846153846,0.348076923076923,
0.35,0.351923076923077,0.353846153846154,0.355769230769231,0.357692307692308,
0.359615384615385,0.361538461538462,0.363461538461538,0.365384615384615,
0.367307692307692,0.369230769230769,0.371153846153846,0.373076923076923,
0.375,0.376923076923077,0.378846153846154,0.380769230769231,0.382692307692308,
0.384615384615385,0.386538461538462,0.388461538461538,0.390384615384615,
0.392307692307692,0.394230769230769,0.396153846153846,0.398076923076923,
0.4,0.401923076923077,0.403846153846154,0.405769230769231,0.407692307692308,
0.409615384615385,0.411538461538462,0.413461538461538,0.415384615384615,
0.417307692307692,0.419230769230769,0.421153846153846,0.423076923076923,
0.425,0.426923076923077,0.428846153846154,0.430769230769231,0.432692307692308,
0.434615384615385,0.436538461538462,0.438461538461538,0.440384615384615,
0.442307692307692,0.444230769230769,0.446153846153846,0.448076923076923,
0.45,0.451923076923077,0.453846153846154,0.455769230769231,0.457692307692308,
0.459615384615385,0.461538461538462,0.463461538461538,0.465384615384615,
0.467307692307692,0.469230769230769,0.471153846153846,0.473076923076923,
0.475,0.476923076923077,0.478846153846154,0.480769230769231,0.482692307692308,
0.484615384615385,0.486538461538462,0.488461538461538,0.490384615384615,
0.492307692307692,0.494230769230769,0.496153846153846,0.498076923076923,
0.5,0.501923076923077,0.503846153846154,0.505769230769231,0.507692307692308,
0.509615384615385,0.511538461538461,0.513461538461538,0.515384615384615,
0.517307692307692,0.519230769230769,0.521153846153846,0.523076923076923,
0.525,0.526923076923077,0.528846153846154,0.530769230769231,0.532692307692308,
0.534615384615385,0.536538461538462,0.538461538461538,0.540384615384615,
0.542307692307692,0.544230769230769,0.546153846153846,0.548076923076923,
0.55,0.551923076923077,0.553846153846154,0.555769230769231,0.557692307692308,
0.559615384615385,0.561538461538462,0.563461538461538,0.565384615384615,
0.567307692307692,0.569230769230769,0.571153846153846,0.573076923076923,
0.575,0.576923076923077,0.578846153846154,0.580769230769231,0.582692307692308,
0.584615384615385,0.586538461538462,0.588461538461538,0.590384615384615,
0.592307692307692,0.594230769230769,0.596153846153846,0.598076923076923,
0.6,0.601923076923077,0.603846153846154,0.605769230769231,0.607692307692308,
0.609615384615385,0.611538461538462,0.613461538461539,0.615384615384615,
0.617307692307692,0.619230769230769,0.621153846153846,0.623076923076923,
0.625,0.626923076923077,0.628846153846154,0.630769230769231,0.632692307692308,
0.634615384615385,0.636538461538461,0.638461538461538,0.640384615384615,
0.642307692307692,0.644230769230769,0.646153846153846,0.648076923076923,
0.65,0.651923076923077,0.653846153846154,0.655769230769231,0.657692307692308,
0.659615384615385,0.661538461538462,0.663461538461538,0.665384615384615,
0.667307692307692,0.669230769230769,0.671153846153846,0.673076923076923,
0.675,0.676923076923077,0.678846153846154,0.680769230769231,0.682692307692308,
0.684615384615385,0.686538461538462,0.688461538461538,0.690384615384615,
0.692307692307692,0.694230769230769,0.696153846153846,0.698076923076923,
0.7,0.701923076923077,0.703846153846154,0.705769230769231,0.707692307692308,
0.709615384615385,0.711538461538462,0.713461538461538,0.715384615384615,
0.717307692307692,0.719230769230769,0.721153846153846,0.723076923076923,
0.725,0.726923076923077,0.728846153846154,0.730769230769231,0.732692307692308,
0.734615384615385,0.736538461538462,0.738461538461539,0.740384615384615,
0.742307692307692,0.744230769230769,0.746153846153846,0.748076923076923,
0.75,0.751923076923077,0.753846153846154,0.755769230769231,0.757692307692308,
0.759615384615385,0.761538461538461,0.763461538461538,0.765384615384615,
0.767307692307692,0.769230769230769,0.771153846153846,0.773076923076923,
0.775,0.776923076923077,0.778846153846154,0.780769230769231,0.782692307692308,
0.784615384615385,0.786538461538462,0.788461538461538,0.790384615384615,
0.792307692307692,0.794230769230769,0.796153846153846,0.798076923076923,
0.8,0.801923076923077,0.803846153846154,0.805769230769231,0.807692307692308,
0.809615384615385,0.811538461538462,0.813461538461538,0.815384615384615,
0.817307692307692,0.819230769230769,0.821153846153846,0.823076923076923,
0.825,0.826923076923077,0.828846153846154,0.830769230769231,0.832692307692308,
0.834615384615385,0.836538461538462,0.838461538461538,0.840384615384615,
0.842307692307692,0.844230769230769,0.846153846153846,0.848076923076923,
0.85,0.851923076923077,0.853846153846154,0.855769230769231,0.857692307692308,
0.859615384615385,0.861538461538462,0.863461538461539,0.865384615384615,
0.867307692307692,0.869230769230769,0.871153846153846,0.873076923076923,
0.875,0.876923076923077,0.878846153846154,0.880769230769231,0.882692307692308,
0.884615384615385,0.886538461538461,0.888461538461538,0.890384615384615,
0.892307692307692,0.894230769230769,0.896153846153846,0.898076923076923,
0.9,0.901923076923077,0.903846153846154,0.905769230769231,0.907692307692308,
0.909615384615385,0.911538461538462,0.913461538461538,0.915384615384615,
0.917307692307692,0.919230769230769,0.921153846153846,0.923076923076923,
0.925,0.926923076923077,0.928846153846154,0.930769230769231,0.932692307692308,
0.934615384615385,0.936538461538462,0.938461538461538,0.940384615384615,
0.942307692307692,0.944230769230769,0.946153846153846,0.948076923076923,
0.95,0.951923076923077,0.953846153846154,0.955769230769231,0.957692307692308,
0.959615384615385,0.961538461538462,0.963461538461538,0.965384615384615,
0.967307692307692,0.969230769230769,0.971153846153846,0.973076923076923,
0.975,0.976923076923077,0.978846153846154,0.980769230769231,0.982692307692308,
0.984615384615385,0.986538461538462,0.988461538461539,0.990384615384615,
0.992307692307692,0.994230769230769,0.996153846153846),.UNSPECIFIED.)
GEOMETRIC_REPRESENTATION_ITEM()
RATIONAL_B_SPLINE_SURFACE(((1.,0.951056516295154,1.,0.951056516295154,1.,
0.951056516295154,1.,0.951056516295154,1.,0.951056516295154,1.,0.951056516295154,
1.,0.951056516295154,1.,0.951056516295154,1.,0.951056516295154,1.,0.951056516295154,
1.,0.951056516295154,1.,0.951056516295154,1.,0.951056516295154,1.,0.951056516295154,
1.,0.951056516295154,1.,0.951056516295154,1.,0.951056516295154,1.,0.951056516295154,
1.,0.951056516295154,1.,0.951056516295154,1.,0.951056516295154,1.,0.951056516295154,
1.,0.951056516295154,1.,0.951056516295154,1.,0.951056516295154,1.,0.951056516295154,
1.,0.951056516295154,1.,0.951056516295154,1.,0.951056516295154,1.,0.951056516295154,
1.,0.951056516295154,1.,0.951056516295154,1.,0.951056516295154,1.,0.951056516295154,
1.,0.951056516295154,1.,0.951056516295154,1.,0.951056516295154,1.,0.951056516295154,
1.,0.951056516295154,1.,0.951056516295154,1.,0.951056516295154,1.,0.951056516295154,
1.,0.951056516295154,1.,0.951056516295154,1.,0.951056516295154,1.,0.951056516295154,
1.,0.951056516295154,1.,0.951056516295154,1.,0.951056516295154,1.,0.951056516295154,
1.,0.951056516295154,1.,0.951056516295154,1.,0.951056516295154,1.,0.951056516295154,
1.,0.951056516295154,1.,0.951056516295154,1.,0.951056516295154,1.,0.951056516295154,
1.,0.951056516295154,1.,0.951056516295154,1.,0.951056516295154,1.,0.951056516295154,
1.,0.951056516295154,1.,0.951056516295154,1.,0.951056516295154,1.,0.951056516295154,
1.,0.951056516295154,1.,0.951056516295154,1.,0.951056516295154,1.,0.951056516295154,
1.,0.951056516295154,1.,0.951056516295154,1.,0.951056516295154,1.,0.951056516295154,
1.,0.951056516295154,1.,0.951056516295154,1.,0.951056516295154,1.,0.951056516295154,
1.,0.951056516295154,1.,0.951056516295154,1.,0.951056516295154,1.,0.951056516295154,
1.,0.951056516295154,1.,0.951056516295154,1.,0.951056516295154,1.,0.951056516295154,
1.,0.951056516295154,1.,0.951056516295154,1.,0.951056516295154,1.,0.951056516295154,
1.,0.951056516295154,1.,0.951056516295154,1.,0.951056516295154,1.,0.951056516295154,
1.,0.951056516295154,1.,0.951056516295154,1.,0.951056516295154,1.,0.951056516295154,
1.,0.951056516295154,1.,0.951056516295154,1.,0.951056516295154,1.,0.951056516295154,
1.,0.951056516295154,1.,0.951056516295154,1.,0.951056516295154,1.,0.951056516295154,
1.,0.951056516295154,1.,0.951056516295154,1.,0.951056516295154,1.,0.951056516295154,
1.,0.951056516295154,1.,0.951056516295154,1.,0.951056516295154,1.,0.951056516295154,
1.,0.951056516295154,1.,0.951056516295154,1.,0.951056516295154,1.,0.951056516295154,
1.,0.951056516295154,1.,0.951056516295154,1.,0.951056516295154,1.,0.951056516295154,
1.,0.951056516295154,1.,0.951056516295154,1.,0.951056516295154,1.,0.951056516295154,
1.,0.951056516295154,1.,0.951056516295154,1.,0.951056516295154,1.,0.951056516295154,
1.,0.951056516295154,1.,0.951056516295154,1.,0.951056516295154,1.,0.951056516295154,
1.,0.951056516295154,1.,0.951056516295154,1.,0.951056516295154,1.,0.951056516295154,
1.,0.951056516295154,1.,0.951056516295154,1.,0.951056516295154,1.,0.951056516295154,
1.,0.951056516295154,1.,0.951056516295154,1.,0.951056516295154,1.,0.951056516295154,
1.,0.951056516295154,1.,0.951056516295154,1.,0.951056516295154,1.,0.951056516295154,
1.,0.951056516295154,1.,0.951056516295154,1.,0.951056516295154,1.,0.951056516295154,
1.,0.951056516295154,1.,0.951056516295154,1.,0.951056516295154,1.,0.951056516295154,
1.,0.951056516295154,1.,0.951056516295154,1.,0.951056516295154,1.,0.951056516295154,
1.,0.951056516295154,1.,0.951056516295154,1.,0.951056516295154,1.,0.951056516295154,
1.,0.951056516295154,1.,0.951056516295154,1.,0.951056516295154,1.,0.951056516295154,
1.,0.951056516295154,1.,0.951056516295154,1.,0.951056516295154,1.,0.951056516295154,
1.,0.951056516295154,1.,0.951056516295154,1.,0.951056516295154,1.,0.951056516295154,
1.,0.951056516295154,1.,0.951056516295154,1.,0.951056516295154,1.,0.951056516295154,
1.,0.951056516295154,1.,0.951056516295154,1.,0.951056516295154,1.,0.951056516295154,
1.,0.951056516295154,1.,0.951056516295154,1.,0.951056516295154,1.,0.951056516295154,
1.,0.951056516295154,1.,0.951056516295154,1.,0.951056516295154,1.,0.951056516295154,
1.,0.951056516295154,1.,0.951056516295154,1.,0.951056516295154,1.,0.951056516295154,
1.,0.951056516295154,1.,0.951056516295154,1.,0.951056516295154,1.,0.951056516295154,
1.,0.951056516295154,1.,0.951056516295154,1.,0.951056516295154,1.,0.951056516295154,
1.,0.951056516295154,1.,0.951056516295154,1.,0.951056516295154,1.,0.951056516295154,
1.,0.951056516295154,1.,0.951056516295154,1.,0.951056516295154,1.,0.951056516295154,
1.,0.951056516295154,1.,0.951056516295154,1.,0.951056516295154,1.,0.951056516295154,
1.,0.951056516295154,1.,0.951056516295154,1.,0.951056516295154,1.,0.951056516295154,
1.,0.951056516295154,1.,0.951056516295154,1.,0.951056516295154,1.,0.951056516295154,
1.,0.951056516295154,1.,0.951056516295154,1.,0.951056516295154,1.,0.951056516295154,
1.,0.951056516295154,1.,0.951056516295154,1.,0.951056516295154,1.,0.951056516295154,
1.,0.951056516295154,1.,0.951056516295154,1.,0.951056516295154,1.,0.951056516295154,
1.,0.951056516295154,1.,0.951056516295154,1.,0.951056516295154,1.,0.951056516295154,
1.,0.951056516295154,1.,0.951056516295154,1.,0.951056516295154,1.,0.951056516295154,
1.,0.951056516295154,1.,0.951056516295154,1.,0.951056516295154,1.,0.951056516295154,
1.,0.951056516295154,1.,0.951056516295154,1.,0.951056516295154,1.,0.951056516295154,
1.,0.951056516295154,1.,0.951056516295154,1.,0.951056516295154,1.,0.951056516295154,
1.,0.951056516295154,1.,0.951056516295154,1.,0.951056516295154,1.,0.951056516295154,
1.,0.951056516295154,1.,0.951056516295154,1.,0.951056516295154,1.,0.951056516295154,
1.,0.951056516295154,1.,0.951056516295154,1.,0.951056516295154,1.,0.951056516295154,
1.,0.951056516295154,1.,0.951056516295154,1.,0.951056516295154,1.,0.951056516295154,
1.,0.951056516295154,1.,0.951056516295154,1.,0.951056516295154,1.,0.951056516295154,
1.,0.951056516295154,1.,0.951056516295154,1.,0.951056516295154,1.,0.951056516295154,
1.,0.951056516295154,1.,0.951056516295154,1.,0.951056516295154,1.,0.951056516295154,
1.,0.951056516295154,1.,0.951056516295154,1.,0.951056516295154,1.,0.951056516295154,
1.,0.951056516295154,1.,0.951056516295154,1.,0.951056516295154,1.,0.951056516295154,
1.,0.951056516295154,1.,0.951056516295154,1.,0.951056516295154,1.,0.951056516295154,
1.,0.951056516295154,1.,0.951056516295154,1.,0.951056516295154,1.,0.951056516295154,
1.,0.951056516295154,1.,0.951056516295154,1.,0.951056516295154,1.,0.951056516295154,
1.,0.951056516295154,1.,0.951056516295154,1.,0.951056516295154,1.,0.951056516295154,
1.,0.951056516295154,1.,0.951056516295154,1.,0.951056516295154,1.,0.951056516295154,
1.,0.951056516295154,1.,0.951056516295154,1.,0.951056516295154,1.,0.951056516295154,
1.,0.951056516295154,1.,0.951056516295154,1.,0.951056516295154,1.,0.951056516295154,
1.,0.951056516295154,1.,0.951056516295154,1.,0.951056516295154,1.,0.951056516295154,
1.,0.951056516295154,1.,0.951056516295154,1.,0.951056516295154,1.,0.951056516295154,
1.,0.951056516295154,1.,0.951056516295154,1.,0.951056516295154,1.,0.951056516295154,
1.,0.951056516295154,1.,0.951056516295154,1.,0.951056516295154,1.,0.951056516295154,
1.,0.951056516295154,1.,0.951056516295154,1.,0.951056516295154,1.,0.951056516295154,
1.,0.951056516295154,1.,0.951056516295154,1.,0.951056516295154,1.,0.951056516295154,
1.,0.951056516295154,1.,0.951056516295154,1.,0.951056516295154,1.,0.951056516295154,
1.,0.951056516295154,1.,0.951056516295154,1.,0.951056516295154,1.,0.951056516295154,
1.,0.951056516295154,1.,0.951056516295154,1.,0.951056516295154,1.,0.951056516295154,
1.,0.951056516295154,1.,0.951056516295154,1.,0.951056516295154,1.,0.951056516295154,
1.,0.951056516295154,1.,0.951056516295154,1.,0.951056516295154,1.,0.951056516295154,
1.,0.951056516295154,1.,0.951056516295154,1.,0.951056516295154,1.,0.951056516295154,
1.,0.951056516295154,1.,0.951056516295154,1.,0.951056516295154,1.,0.951056516295154,
1.,0.951056516295154,1.,0.951056516295154,1.,0.951056516295154,1.,0.951056516295154,
1.,0.951056516295154,1.,0.951056516295154,1.,0.951056516295154,1.,0.951056516295154,
1.,0.951056516295154,1.,0.951056516295154,1.,0.951056516295154,1.,0.951056516295154,
1.,0.951056516295154,1.,0.951056516295154,1.,0.951056516295154,1.,0.951056516295154,
1.,0.951056516295154,1.,0.951056516295154,1.,0.951056516295154,1.,0.951056516295154,
1.,0.951056516295154,1.,0.951056516295154,1.,0.951056516295154,1.,0.951056516295154,
1.,0.951056516295154,1.,0.951056516295154,1.,0.951056516295154,1.,0.951056516295154,
1.,0.951056516295154,1.,0.951056516295154,1.,0.951056516295154,1.,0.951056516295154,
1.,0.951056516295154,1.,0.951056516295154,1.,0.951056516295154,1.,0.951056516295154,
1.,0.951056516295154,1.,0.951056516295154,1.,0.951056516295154,1.,0.951056516295154,
1.,0.951056516295154,1.,0.951056516295154,1.,0.951056516295154,1.,0.951056516295154,
1.,0.951056516295154,1.,0.951056516295154,1.,0.951056516295154,1.,0.951056516295154,
1.,0.951056516295154,1.,0.951056516295154,1.,0.951056516295154,1.,0.951056516295154,
1.,0.951056516295154,1.,0.951056516295154,1.,0.951056516295154,1.,0.951056516295154,
1.,0.951056516295154,1.,0.951056516295154,1.,0.951056516295154,1.,0.951056516295154,
1.,0.951056516295154,1.,0.951056516295154,1.,0.951056516295154,1.,0.951056516295154,
1.,0.951056516295154,1.,0.951056516295154,1.,0.951056516295154,1.,0.951056516295154,
1.,0.951056516295154,1.,0.951056516295154,1.,0.951056516295154,1.,0.951056516295154,
1.,0.951056516295154,1.,0.951056516295154,1.,0.951056516295154,1.,0.951056516295154,
1.,0.951056516295154,1.,0.951056516295154,1.,0.951056516295154,1.,0.951056516295154,
1.,0.951056516295154,1.,0.951056516295154,1.,0.951056516295154,1.,0.951056516295154,
1.,0.951056516295154,1.,0.951056516295154,1.,0.951056516295154,1.,0.951056516295154,
1.,0.951056516295154,1.,0.951056516295154,1.,0.951056516295154,1.,0.951056516295154,
1.,0.951056516295154,1.,0.951056516295154,1.,0.951056516295154,1.,0.951056516295154,
1.,0.951056516295154,1.,0.951056516295154,1.,0.951056516295154,1.,0.951056516295154,
1.,0.951056516295154,1.,0.951056516295154,1.,0.951056516295154,1.,0.951056516295154,
1.,0.951056516295154,1.,0.951056516295154,1.,0.951056516295154,1.,0.951056516295154,
1.,0.951056516295154,1.,0.951056516295154,1.,0.951056516295154,1.,0.951056516295154,
1.,0.951056516295154,1.,0.951056516295154,1.,0.951056516295154,1.,0.951056516295154,
1.,0.951056516295154,1.,0.951056516295154,1.,0.951056516295154,1.,0.951056516295154,
1.,0.951056516295154,1.,0.951056516295154,1.,0.951056516295154,1.,0.951056516295154,
1.,0.951056516295154,1.,0.951056516295154,1.,0.951056516295154,1.,0.951056516295154,
1.,0.951056516295154,1.,0.951056516295154,1.,0.951056516295154,1.,0.951056516295154,
1.,0.951056516295154,1.,0.951056516295154,1.,0.951056516295154,1.,0.951056516295154,
1.,0.951056516295154,1.,0.951056516295154,1.,0.951056516295154,1.,0.951056516295154,
1.,0.951056516295154,1.,0.951056516295154,1.,0.951056516295154,1.,0.951056516295154,
1.),(1.,0.951056516295154,1.,0.951056516295154,1.,0.951056516295154,1.,
0.951056516295154,1.,0.951056516295154,1.,0.951056516295154,1.,0.951056516295154,
1.,0.951056516295154,1.,0.951056516295154,1.,0.951056516295154,1.,0.951056516295154,
1.,0.951056516295154,1.,0.951056516295154,1.,0.951056516295154,1.,0.951056516295154,
1.,0.951056516295154,1.,0.951056516295154,1.,0.951056516295154,1.,0.951056516295154,
1.,0.951056516295154,1.,0.951056516295154,1.,0.951056516295154,1.,0.951056516295154,
1.,0.951056516295154,1.,0.951056516295154,1.,0.951056516295154,1.,0.951056516295154,
1.,0.951056516295154,1.,0.951056516295154,1.,0.951056516295154,1.,0.951056516295154,
1.,0.951056516295154,1.,0.951056516295154,1.,0.951056516295154,1.,0.951056516295154,
1.,0.951056516295154,1.,0.951056516295154,1.,0.951056516295154,1.,0.951056516295154,
1.,0.951056516295154,1.,0.951056516295154,1.,0.951056516295154,1.,0.951056516295154,
1.,0.951056516295154,1.,0.951056516295154,1.,0.951056516295154,1.,0.951056516295154,
1.,0.951056516295154,1.,0.951056516295154,1.,0.951056516295154,1.,0.951056516295154,
1.,0.951056516295154,1.,0.951056516295154,1.,0.951056516295154,1.,0.951056516295154,
1.,0.951056516295154,1.,0.951056516295154,1.,0.951056516295154,1.,0.951056516295154,
1.,0.951056516295154,1.,0.951056516295154,1.,0.951056516295154,1.,0.951056516295154,
1.,0.951056516295154,1.,0.951056516295154,1.,0.951056516295154,1.,0.951056516295154,
1.,0.951056516295154,1.,0.951056516295154,1.,0.951056516295154,1.,0.951056516295154,
1.,0.951056516295154,1.,0.951056516295154,1.,0.951056516295154,1.,0.951056516295154,
1.,0.951056516295154,1.,0.951056516295154,1.,0.951056516295154,1.,0.951056516295154,
1.,0.951056516295154,1.,0.951056516295154,1.,0.951056516295154,1.,0.951056516295154,
1.,0.951056516295154,1.,0.951056516295154,1.,0.951056516295154,1.,0.951056516295154,
1.,0.951056516295154,1.,0.951056516295154,1.,0.951056516295154,1.,0.951056516295154,
1.,0.951056516295154,1.,0.951056516295154,1.,0.951056516295154,1.,0.951056516295154,
1.,0.951056516295154,1.,0.951056516295154,1.,0.951056516295154,1.,0.951056516295154,
1.,0.951056516295154,1.,0.951056516295154,1.,0.951056516295154,1.,0.951056516295154,
1.,0.951056516295154,1.,0.951056516295154,1.,0.951056516295154,1.,0.951056516295154,
1.,0.951056516295154,1.,0.951056516295154,1.,0.951056516295154,1.,0.951056516295154,
1.,0.951056516295154,1.,0.951056516295154,1.,0.951056516295154,1.,0.951056516295154,
1.,0.951056516295154,1.,0.951056516295154,1.,0.951056516295154,1.,0.951056516295154,
1.,0.951056516295154,1.,0.951056516295154,1.,0.951056516295154,1.,0.951056516295154,
1.,0.951056516295154,1.,0.951056516295154,1.,0.951056516295154,1.,0.951056516295154,
1.,0.951056516295154,1.,0.951056516295154,1.,0.951056516295154,1.,0.951056516295154,
1.,0.951056516295154,1.,0.951056516295154,1.,0.951056516295154,1.,0.951056516295154,
1.,0.951056516295154,1.,0.951056516295154,1.,0.951056516295154,1.,0.951056516295154,
1.,0.951056516295154,1.,0.951056516295154,1.,0.951056516295154,1.,0.951056516295154,
1.,0.951056516295154,1.,0.951056516295154,1.,0.951056516295154,1.,0.951056516295154,
1.,0.951056516295154,1.,0.951056516295154,1.,0.951056516295154,1.,0.951056516295154,
1.,0.951056516295154,1.,0.951056516295154,1.,0.951056516295154,1.,0.951056516295154,
1.,0.951056516295154,1.,0.951056516295154,1.,0.951056516295154,1.,0.951056516295154,
1.,0.951056516295154,1.,0.951056516295154,1.,0.951056516295154,1.,0.951056516295154,
1.,0.951056516295154,1.,0.951056516295154,1.,0.951056516295154,1.,0.951056516295154,
1.,0.951056516295154,1.,0.951056516295154,1.,0.951056516295154,1.,0.951056516295154,
1.,0.951056516295154,1.,0.951056516295154,1.,0.951056516295154,1.,0.951056516295154,
1.,0.951056516295154,1.,0.951056516295154,1.,0.951056516295154,1.,0.951056516295154,
1.,0.951056516295154,1.,0.951056516295154,1.,0.951056516295154,1.,0.951056516295154,
1.,0.951056516295154,1.,0.951056516295154,1.,0.951056516295154,1.,0.951056516295154,
1.,0.951056516295154,1.,0.951056516295154,1.,0.951056516295154,1.,0.951056516295154,
1.,0.951056516295154,1.,0.951056516295154,1.,0.951056516295154,1.,0.951056516295154,
1.,0.951056516295154,1.,0.951056516295154,1.,0.951056516295154,1.,0.951056516295154,
1.,0.951056516295154,1.,0.951056516295154,1.,0.951056516295154,1.,0.951056516295154,
1.,0.951056516295154,1.,0.951056516295154,1.,0.951056516295154,1.,0.951056516295154,
1.,0.951056516295154,1.,0.951056516295154,1.,0.951056516295154,1.,0.951056516295154,
1.,0.951056516295154,1.,0.951056516295154,1.,0.951056516295154,1.,0.951056516295154,
1.,0.951056516295154,1.,0.951056516295154,1.,0.951056516295154,1.,0.951056516295154,
1.,0.951056516295154,1.,0.951056516295154,1.,0.951056516295154,1.,0.951056516295154,
1.,0.951056516295154,1.,0.951056516295154,1.,0.951056516295154,1.,0.951056516295154,
1.,0.951056516295154,1.,0.951056516295154,1.,0.951056516295154,1.,0.951056516295154,
1.,0.951056516295154,1.,0.951056516295154,1.,0.951056516295154,1.,0.951056516295154,
1.,0.951056516295154,1.,0.951056516295154,1.,0.951056516295154,1.,0.951056516295154,
1.,0.951056516295154,1.,0.951056516295154,1.,0.951056516295154,1.,0.951056516295154,
1.,0.951056516295154,1.,0.951056516295154,1.,0.951056516295154,1.,0.951056516295154,
1.,0.951056516295154,1.,0.951056516295154,1.,0.951056516295154,1.,0.951056516295154,
1.,0.951056516295154,1.,0.951056516295154,1.,0.951056516295154,1.,0.951056516295154,
1.,0.951056516295154,1.,0.951056516295154,1.,0.951056516295154,1.,0.951056516295154,
1.,0.951056516295154,1.,0.951056516295154,1.,0.951056516295154,1.,0.951056516295154,
1.,0.951056516295154,1.,0.951056516295154,1.,0.951056516295154,1.,0.951056516295154,
1.,0.951056516295154,1.,0.951056516295154,1.,0.951056516295154,1.,0.951056516295154,
1.,0.951056516295154,1.,0.951056516295154,1.,0.951056516295154,1.,0.951056516295154,
1.,0.951056516295154,1.,0.951056516295154,1.,0.951056516295154,1.,0.951056516295154,
1.,0.951056516295154,1.,0.951056516295154,1.,0.951056516295154,1.,0.951056516295154,
1.,0.951056516295154,1.,0.951056516295154,1.,0.951056516295154,1.,0.951056516295154,
1.,0.951056516295154,1.,0.951056516295154,1.,0.951056516295154,1.,0.951056516295154,
1.,0.951056516295154,1.,0.951056516295154,1.,0.951056516295154,1.,0.951056516295154,
1.,0.951056516295154,1.,0.951056516295154,1.,0.951056516295154,1.,0.951056516295154,
1.,0.951056516295154,1.,0.951056516295154,1.,0.951056516295154,1.,0.951056516295154,
1.,0.951056516295154,1.,0.951056516295154,1.,0.951056516295154,1.,0.951056516295154,
1.,0.951056516295154,1.,0.951056516295154,1.,0.951056516295154,1.,0.951056516295154,
1.,0.951056516295154,1.,0.951056516295154,1.,0.951056516295154,1.,0.951056516295154,
1.,0.951056516295154,1.,0.951056516295154,1.,0.951056516295154,1.,0.951056516295154,
1.,0.951056516295154,1.,0.951056516295154,1.,0.951056516295154,1.,0.951056516295154,
1.,0.951056516295154,1.,0.951056516295154,1.,0.951056516295154,1.,0.951056516295154,
1.,0.951056516295154,1.,0.951056516295154,1.,0.951056516295154,1.,0.951056516295154,
1.,0.951056516295154,1.,0.951056516295154,1.,0.951056516295154,1.,0.951056516295154,
1.,0.951056516295154,1.,0.951056516295154,1.,0.951056516295154,1.,0.951056516295154,
1.,0.951056516295154,1.,0.951056516295154,1.,0.951056516295154,1.,0.951056516295154,
1.,0.951056516295154,1.,0.951056516295154,1.,0.951056516295154,1.,0.951056516295154,
1.,0.951056516295154,1.,0.951056516295154,1.,0.951056516295154,1.,0.951056516295154,
1.,0.951056516295154,1.,0.951056516295154,1.,0.951056516295154,1.,0.951056516295154,
1.,0.951056516295154,1.,0.951056516295154,1.,0.951056516295154,1.,0.951056516295154,
1.,0.951056516295154,1.,0.951056516295154,1.,0.951056516295154,1.,0.951056516295154,
1.,0.951056516295154,1.,0.951056516295154,1.,0.951056516295154,1.,0.951056516295154,
1.,0.951056516295154,1.,0.951056516295154,1.,0.951056516295154,1.,0.951056516295154,
1.,0.951056516295154,1.,0.951056516295154,1.,0.951056516295154,1.,0.951056516295154,
1.,0.951056516295154,1.,0.951056516295154,1.,0.951056516295154,1.,0.951056516295154,
1.,0.951056516295154,1.,0.951056516295154,1.,0.951056516295154,1.,0.951056516295154,
1.,0.951056516295154,1.,0.951056516295154,1.,0.951056516295154,1.,0.951056516295154,
1.,0.951056516295154,1.,0.951056516295154,1.,0.951056516295154,1.,0.951056516295154,
1.,0.951056516295154,1.,0.951056516295154,1.,0.951056516295154,1.,0.951056516295154,
1.,0.951056516295154,1.,0.951056516295154,1.,0.951056516295154,1.,0.951056516295154,
1.,0.951056516295154,1.,0.951056516295154,1.,0.951056516295154,1.,0.951056516295154,
1.,0.951056516295154,1.,0.951056516295154,1.,0.951056516295154,1.,0.951056516295154,
1.,0.951056516295154,1.,0.951056516295154,1.,0.951056516295154,1.,0.951056516295154,
1.,0.951056516295154,1.,0.951056516295154,1.,0.951056516295154,1.,0.951056516295154,
1.,0.951056516295154,1.,0.951056516295154,1.,0.951056516295154,1.,0.951056516295154,
1.,0.951056516295154,1.,0.951056516295154,1.,0.951056516295154,1.,0.951056516295154,
1.,0.951056516295154,1.,0.951056516295154,1.,0.951056516295154,1.,0.951056516295154,
1.,0.951056516295154,1.,0.951056516295154,1.,0.951056516295154,1.,0.951056516295154,
1.,0.951056516295154,1.,0.951056516295154,1.,0.951056516295154,1.,0.951056516295154,
1.,0.951056516295154,1.,0.951056516295154,1.,0.951056516295154,1.,0.951056516295154,
1.,0.951056516295154,1.,0.951056516295154,1.,0.951056516295154,1.,0.951056516295154,
1.,0.951056516295154,1.,0.951056516295154,1.,0.951056516295154,1.,0.951056516295154,
1.,0.951056516295154,1.,0.951056516295154,1.,0.951056516295154,1.,0.951056516295154,
1.,0.951056516295154,1.,0.951056516295154,1.,0.951056516295154,1.,0.951056516295154,
1.,0.951056516295154,1.,0.951056516295154,1.,0.951056516295154,1.,0.951056516295154,
1.,0.951056516295154,1.,0.951056516295154,1.,0.951056516295154,1.,0.951056516295154,
1.,0.951056516295154,1.,0.951056516295154,1.,0.951056516295154,1.,0.951056516295154,
1.,0.951056516295154,1.,0.951056516295154,1.,0.951056516295154,1.,0.951056516295154,
1.,0.951056516295154,1.,0.951056516295154,1.,0.951056516295154,1.,0.951056516295154,
1.,0.951056516295154,1.,0.951056516295154,1.,0.951056516295154,1.,0.951056516295154,
1.,0.951056516295154,1.,0.951056516295154,1.,0.951056516295154,1.,0.951056516295154,
1.,0.951056516295154,1.,0.951056516295154,1.,0.951056516295154,1.,0.951056516295154,
1.,0.951056516295154,1.,0.951056516295154,1.,0.951056516295154,1.,0.951056516295154,
1.,0.951056516295154,1.,0.951056516295154,1.,0.951056516295154,1.,0.951056516295154,
1.,0.951056516295154,1.,0.951056516295154,1.,0.951056516295154,1.,0.951056516295154,
1.,0.951056516295154,1.,0.951056516295154,1.,0.951056516295154,1.,0.951056516295154,
1.,0.951056516295154,1.,0.951056516295154,1.,0.951056516295154,1.,0.951056516295154,
1.,0.951056516295154,1.,0.951056516295154,1.,0.951056516295154,1.,0.951056516295154,
1.,0.951056516295154,1.,0.951056516295154,1.,0.951056516295154,1.,0.951056516295154,
1.,0.951056516295154,1.,0.951056516295154,1.,0.951056516295154,1.)))
REPRESENTATION_ITEM('')
SURFACE()
);
#3199=(
BOUNDED_SURFACE()
B_SPLINE_SURFACE(1,2,((#296159,#296160,#296161,#296162,#296163,#296164,
#296165,#296166,#296167,#296168,#296169,#296170,#296171,#296172,#296173,
#296174,#296175,#296176,#296177,#296178,#296179,#296180,#296181,#296182,
#296183,#296184,#296185,#296186,#296187,#296188,#296189,#296190,#296191,
#296192,#296193,#296194,#296195,#296196,#296197,#296198,#296199,#296200,
#296201,#296202,#296203,#296204,#296205,#296206,#296207,#296208,#296209,
#296210,#296211,#296212,#296213,#296214,#296215,#296216,#296217,#296218,
#296219,#296220,#296221,#296222,#296223,#296224,#296225,#296226,#296227,
#296228,#296229,#296230,#296231,#296232,#296233,#296234,#296235,#296236,
#296237,#296238,#296239,#296240,#296241,#296242,#296243,#296244,#296245,
#296246,#296247,#296248,#296249,#296250,#296251,#296252,#296253,#296254,
#296255,#296256,#296257,#296258,#296259,#296260,#296261,#296262,#296263,
#296264,#296265,#296266,#296267,#296268,#296269,#296270,#296271,#296272,
#296273,#296274,#296275,#296276,#296277,#296278,#296279,#296280,#296281,
#296282,#296283,#296284,#296285,#296286,#296287,#296288,#296289,#296290,
#296291,#296292,#296293,#296294,#296295,#296296,#296297,#296298,#296299,
#296300,#296301,#296302,#296303,#296304,#296305,#296306,#296307,#296308,
#296309,#296310,#296311,#296312,#296313,#296314,#296315,#296316,#296317,
#296318,#296319,#296320,#296321,#296322,#296323,#296324,#296325,#296326,
#296327,#296328,#296329,#296330,#296331,#296332,#296333,#296334,#296335,
#296336,#296337,#296338,#296339,#296340,#296341,#296342,#296343,#296344,
#296345,#296346,#296347,#296348,#296349,#296350,#296351,#296352,#296353,
#296354,#296355,#296356,#296357,#296358,#296359,#296360,#296361,#296362,
#296363,#296364,#296365,#296366,#296367,#296368,#296369,#296370,#296371,
#296372,#296373,#296374,#296375,#296376,#296377,#296378,#296379,#296380,
#296381,#296382,#296383,#296384,#296385,#296386,#296387,#296388,#296389,
#296390,#296391,#296392,#296393,#296394,#296395,#296396,#296397,#296398,
#296399,#296400,#296401,#296402,#296403,#296404,#296405,#296406,#296407,
#296408,#296409,#296410,#296411,#296412,#296413,#296414,#296415,#296416,
#296417,#296418,#296419,#296420,#296421,#296422,#296423,#296424,#296425,
#296426,#296427,#296428,#296429,#296430,#296431,#296432,#296433,#296434,
#296435,#296436,#296437,#296438,#296439,#296440,#296441,#296442,#296443,
#296444,#296445,#296446,#296447,#296448,#296449,#296450,#296451,#296452,
#296453,#296454,#296455,#296456,#296457,#296458,#296459,#296460,#296461,
#296462,#296463,#296464,#296465,#296466,#296467,#296468,#296469,#296470,
#296471,#296472,#296473,#296474,#296475,#296476,#296477,#296478,#296479,
#296480,#296481,#296482,#296483,#296484,#296485,#296486,#296487,#296488,
#296489,#296490,#296491,#296492,#296493,#296494,#296495,#296496,#296497,
#296498,#296499,#296500,#296501,#296502,#296503,#296504,#296505,#296506,
#296507,#296508,#296509,#296510,#296511,#296512,#296513,#296514,#296515,
#296516,#296517,#296518,#296519,#296520,#296521,#296522,#296523,#296524,
#296525,#296526,#296527,#296528,#296529,#296530,#296531,#296532,#296533,
#296534,#296535,#296536,#296537,#296538,#296539,#296540,#296541,#296542,
#296543,#296544,#296545,#296546,#296547,#296548,#296549,#296550,#296551,
#296552,#296553,#296554,#296555,#296556,#296557,#296558,#296559,#296560,
#296561,#296562,#296563,#296564,#296565,#296566,#296567,#296568,#296569,
#296570,#296571,#296572,#296573,#296574,#296575,#296576,#296577,#296578,
#296579,#296580,#296581,#296582,#296583,#296584,#296585,#296586,#296587,
#296588,#296589,#296590,#296591,#296592,#296593,#296594,#296595,#296596,
#296597,#296598,#296599,#296600,#296601,#296602,#296603,#296604,#296605,
#296606,#296607,#296608,#296609,#296610,#296611,#296612,#296613,#296614,
#296615,#296616,#296617,#296618,#296619,#296620,#296621,#296622,#296623,
#296624,#296625,#296626,#296627,#296628,#296629,#296630,#296631,#296632,
#296633,#296634,#296635,#296636,#296637,#296638,#296639,#296640,#296641,
#296642,#296643,#296644,#296645,#296646,#296647,#296648,#296649,#296650,
#296651,#296652,#296653,#296654,#296655,#296656,#296657,#296658,#296659,
#296660,#296661,#296662,#296663,#296664,#296665,#296666,#296667,#296668,
#296669,#296670,#296671,#296672,#296673,#296674,#296675,#296676,#296677,
#296678,#296679,#296680,#296681,#296682,#296683,#296684,#296685,#296686,
#296687,#296688,#296689,#296690,#296691,#296692,#296693,#296694,#296695,
#296696,#296697,#296698,#296699,#296700,#296701,#296702,#296703,#296704,
#296705,#296706,#296707,#296708,#296709,#296710,#296711,#296712,#296713,
#296714,#296715,#296716,#296717,#296718,#296719,#296720,#296721,#296722,
#296723,#296724,#296725,#296726,#296727,#296728,#296729,#296730,#296731,
#296732,#296733,#296734,#296735,#296736,#296737,#296738,#296739,#296740,
#296741,#296742,#296743,#296744,#296745,#296746,#296747,#296748,#296749,
#296750,#296751,#296752,#296753,#296754,#296755,#296756,#296757,#296758,
#296759,#296760,#296761,#296762,#296763,#296764,#296765,#296766,#296767,
#296768,#296769,#296770,#296771,#296772,#296773,#296774,#296775,#296776,
#296777,#296778,#296779,#296780,#296781,#296782,#296783,#296784,#296785,
#296786,#296787,#296788,#296789,#296790,#296791,#296792,#296793,#296794,
#296795,#296796,#296797,#296798,#296799,#296800,#296801,#296802,#296803,
#296804,#296805,#296806,#296807,#296808,#296809,#296810,#296811,#296812,
#296813,#296814,#296815,#296816,#296817,#296818,#296819,#296820,#296821,
#296822,#296823,#296824,#296825,#296826,#296827,#296828,#296829,#296830,
#296831,#296832,#296833,#296834,#296835,#296836,#296837,#296838,#296839,
#296840,#296841,#296842,#296843,#296844,#296845,#296846,#296847,#296848,
#296849,#296850,#296851,#296852,#296853,#296854,#296855,#296856,#296857,
#296858,#296859,#296860,#296861,#296862,#296863,#296864,#296865,#296866,
#296867,#296868,#296869,#296870,#296871,#296872,#296873,#296874,#296875,
#296876,#296877,#296878,#296879,#296880,#296881,#296882,#296883,#296884,
#296885,#296886,#296887,#296888,#296889,#296890,#296891,#296892,#296893,
#296894,#296895,#296896,#296897,#296898,#296899,#296900,#296901,#296902,
#296903,#296904,#296905,#296906,#296907,#296908,#296909,#296910,#296911,
#296912,#296913,#296914,#296915,#296916,#296917,#296918,#296919,#296920,
#296921,#296922,#296923,#296924,#296925,#296926,#296927,#296928,#296929,
#296930,#296931,#296932,#296933,#296934,#296935,#296936,#296937,#296938,
#296939,#296940,#296941,#296942,#296943,#296944,#296945,#296946,#296947,
#296948,#296949,#296950,#296951,#296952,#296953,#296954,#296955,#296956,
#296957,#296958,#296959,#296960,#296961,#296962,#296963,#296964,#296965,
#296966,#296967,#296968,#296969,#296970,#296971,#296972,#296973,#296974,
#296975,#296976,#296977,#296978,#296979,#296980,#296981,#296982,#296983,
#296984,#296985,#296986,#296987,#296988,#296989,#296990,#296991,#296992,
#296993,#296994,#296995,#296996,#296997,#296998,#296999,#297000,#297001,
#297002,#297003,#297004,#297005,#297006,#297007,#297008,#297009,#297010,
#297011,#297012,#297013,#297014,#297015,#297016,#297017,#297018,#297019,
#297020,#297021,#297022,#297023,#297024,#297025,#297026,#297027,#297028,
#297029,#297030,#297031,#297032,#297033,#297034,#297035,#297036,#297037,
#297038,#297039,#297040,#297041,#297042,#297043,#297044,#297045,#297046,
#297047,#297048,#297049,#297050,#297051,#297052,#297053,#297054,#297055,
#297056,#297057,#297058,#297059,#297060,#297061,#297062,#297063,#297064,
#297065,#297066,#297067,#297068,#297069,#297070,#297071,#297072,#297073,
#297074,#297075,#297076,#297077,#297078,#297079,#297080,#297081,#297082,
#297083,#297084,#297085,#297086,#297087,#297088,#297089,#297090,#297091,
#297092,#297093,#297094,#297095,#297096,#297097,#297098,#297099,#297100,
#297101,#297102,#297103,#297104,#297105,#297106,#297107,#297108,#297109,
#297110,#297111,#297112,#297113,#297114,#297115,#297116,#297117,#297118,
#297119,#297120,#297121,#297122,#297123,#297124,#297125,#297126,#297127,
#297128,#297129,#297130,#297131,#297132,#297133,#297134,#297135,#297136,
#297137,#297138,#297139,#297140,#297141,#297142,#297143,#297144,#297145,
#297146,#297147,#297148,#297149,#297150,#297151,#297152,#297153,#297154,
#297155,#297156,#297157,#297158,#297159,#297160,#297161,#297162,#297163,
#297164,#297165,#297166,#297167,#297168,#297169,#297170,#297171,#297172,
#297173,#297174,#297175,#297176,#297177,#297178,#297179,#297180,#297181,
#297182,#297183,#297184,#297185,#297186,#297187,#297188,#297189,#297190,
#297191,#297192,#297193,#297194,#297195),(#297196,#297197,#297198,#297199,
#297200,#297201,#297202,#297203,#297204,#297205,#297206,#297207,#297208,
#297209,#297210,#297211,#297212,#297213,#297214,#297215,#297216,#297217,
#297218,#297219,#297220,#297221,#297222,#297223,#297224,#297225,#297226,
#297227,#297228,#297229,#297230,#297231,#297232,#297233,#297234,#297235,
#297236,#297237,#297238,#297239,#297240,#297241,#297242,#297243,#297244,
#297245,#297246,#297247,#297248,#297249,#297250,#297251,#297252,#297253,
#297254,#297255,#297256,#297257,#297258,#297259,#297260,#297261,#297262,
#297263,#297264,#297265,#297266,#297267,#297268,#297269,#297270,#297271,
#297272,#297273,#297274,#297275,#297276,#297277,#297278,#297279,#297280,
#297281,#297282,#297283,#297284,#297285,#297286,#297287,#297288,#297289,
#297290,#297291,#297292,#297293,#297294,#297295,#297296,#297297,#297298,
#297299,#297300,#297301,#297302,#297303,#297304,#297305,#297306,#297307,
#297308,#297309,#297310,#297311,#297312,#297313,#297314,#297315,#297316,
#297317,#297318,#297319,#297320,#297321,#297322,#297323,#297324,#297325,
#297326,#297327,#297328,#297329,#297330,#297331,#297332,#297333,#297334,
#297335,#297336,#297337,#297338,#297339,#297340,#297341,#297342,#297343,
#297344,#297345,#297346,#297347,#297348,#297349,#297350,#297351,#297352,
#297353,#297354,#297355,#297356,#297357,#297358,#297359,#297360,#297361,
#297362,#297363,#297364,#297365,#297366,#297367,#297368,#297369,#297370,
#297371,#297372,#297373,#297374,#297375,#297376,#297377,#297378,#297379,
#297380,#297381,#297382,#297383,#297384,#297385,#297386,#297387,#297388,
#297389,#297390,#297391,#297392,#297393,#297394,#297395,#297396,#297397,
#297398,#297399,#297400,#297401,#297402,#297403,#297404,#297405,#297406,
#297407,#297408,#297409,#297410,#297411,#297412,#297413,#297414,#297415,
#297416,#297417,#297418,#297419,#297420,#297421,#297422,#297423,#297424,
#297425,#297426,#297427,#297428,#297429,#297430,#297431,#297432,#297433,
#297434,#297435,#297436,#297437,#297438,#297439,#297440,#297441,#297442,
#297443,#297444,#297445,#297446,#297447,#297448,#297449,#297450,#297451,
#297452,#297453,#297454,#297455,#297456,#297457,#297458,#297459,#297460,
#297461,#297462,#297463,#297464,#297465,#297466,#297467,#297468,#297469,
#297470,#297471,#297472,#297473,#297474,#297475,#297476,#297477,#297478,
#297479,#297480,#297481,#297482,#297483,#297484,#297485,#297486,#297487,
#297488,#297489,#297490,#297491,#297492,#297493,#297494,#297495,#297496,
#297497,#297498,#297499,#297500,#297501,#297502,#297503,#297504,#297505,
#297506,#297507,#297508,#297509,#297510,#297511,#297512,#297513,#297514,
#297515,#297516,#297517,#297518,#297519,#297520,#297521,#297522,#297523,
#297524,#297525,#297526,#297527,#297528,#297529,#297530,#297531,#297532,
#297533,#297534,#297535,#297536,#297537,#297538,#297539,#297540,#297541,
#297542,#297543,#297544,#297545,#297546,#297547,#297548,#297549,#297550,
#297551,#297552,#297553,#297554,#297555,#297556,#297557,#297558,#297559,
#297560,#297561,#297562,#297563,#297564,#297565,#297566,#297567,#297568,
#297569,#297570,#297571,#297572,#297573,#297574,#297575,#297576,#297577,
#297578,#297579,#297580,#297581,#297582,#297583,#297584,#297585,#297586,
#297587,#297588,#297589,#297590,#297591,#297592,#297593,#297594,#297595,
#297596,#297597,#297598,#297599,#297600,#297601,#297602,#297603,#297604,
#297605,#297606,#297607,#297608,#297609,#297610,#297611,#297612,#297613,
#297614,#297615,#297616,#297617,#297618,#297619,#297620,#297621,#297622,
#297623,#297624,#297625,#297626,#297627,#297628,#297629,#297630,#297631,
#297632,#297633,#297634,#297635,#297636,#297637,#297638,#297639,#297640,
#297641,#297642,#297643,#297644,#297645,#297646,#297647,#297648,#297649,
#297650,#297651,#297652,#297653,#297654,#297655,#297656,#297657,#297658,
#297659,#297660,#297661,#297662,#297663,#297664,#297665,#297666,#297667,
#297668,#297669,#297670,#297671,#297672,#297673,#297674,#297675,#297676,
#297677,#297678,#297679,#297680,#297681,#297682,#297683,#297684,#297685,
#297686,#297687,#297688,#297689,#297690,#297691,#297692,#297693,#297694,
#297695,#297696,#297697,#297698,#297699,#297700,#297701,#297702,#297703,
#297704,#297705,#297706,#297707,#297708,#297709,#297710,#297711,#297712,
#297713,#297714,#297715,#297716,#297717,#297718,#297719,#297720,#297721,
#297722,#297723,#297724,#297725,#297726,#297727,#297728,#297729,#297730,
#297731,#297732,#297733,#297734,#297735,#297736,#297737,#297738,#297739,
#297740,#297741,#297742,#297743,#297744,#297745,#297746,#297747,#297748,
#297749,#297750,#297751,#297752,#297753,#297754,#297755,#297756,#297757,
#297758,#297759,#297760,#297761,#297762,#297763,#297764,#297765,#297766,
#297767,#297768,#297769,#297770,#297771,#297772,#297773,#297774,#297775,
#297776,#297777,#297778,#297779,#297780,#297781,#297782,#297783,#297784,
#297785,#297786,#297787,#297788,#297789,#297790,#297791,#297792,#297793,
#297794,#297795,#297796,#297797,#297798,#297799,#297800,#297801,#297802,
#297803,#297804,#297805,#297806,#297807,#297808,#297809,#297810,#297811,
#297812,#297813,#297814,#297815,#297816,#297817,#297818,#297819,#297820,
#297821,#297822,#297823,#297824,#297825,#297826,#297827,#297828,#297829,
#297830,#297831,#297832,#297833,#297834,#297835,#297836,#297837,#297838,
#297839,#297840,#297841,#297842,#297843,#297844,#297845,#297846,#297847,
#297848,#297849,#297850,#297851,#297852,#297853,#297854,#297855,#297856,
#297857,#297858,#297859,#297860,#297861,#297862,#297863,#297864,#297865,
#297866,#297867,#297868,#297869,#297870,#297871,#297872,#297873,#297874,
#297875,#297876,#297877,#297878,#297879,#297880,#297881,#297882,#297883,
#297884,#297885,#297886,#297887,#297888,#297889,#297890,#297891,#297892,
#297893,#297894,#297895,#297896,#297897,#297898,#297899,#297900,#297901,
#297902,#297903,#297904,#297905,#297906,#297907,#297908,#297909,#297910,
#297911,#297912,#297913,#297914,#297915,#297916,#297917,#297918,#297919,
#297920,#297921,#297922,#297923,#297924,#297925,#297926,#297927,#297928,
#297929,#297930,#297931,#297932,#297933,#297934,#297935,#297936,#297937,
#297938,#297939,#297940,#297941,#297942,#297943,#297944,#297945,#297946,
#297947,#297948,#297949,#297950,#297951,#297952,#297953,#297954,#297955,
#297956,#297957,#297958,#297959,#297960,#297961,#297962,#297963,#297964,
#297965,#297966,#297967,#297968,#297969,#297970,#297971,#297972,#297973,
#297974,#297975,#297976,#297977,#297978,#297979,#297980,#297981,#297982,
#297983,#297984,#297985,#297986,#297987,#297988,#297989,#297990,#297991,
#297992,#297993,#297994,#297995,#297996,#297997,#297998,#297999,#298000,
#298001,#298002,#298003,#298004,#298005,#298006,#298007,#298008,#298009,
#298010,#298011,#298012,#298013,#298014,#298015,#298016,#298017,#298018,
#298019,#298020,#298021,#298022,#298023,#298024,#298025,#298026,#298027,
#298028,#298029,#298030,#298031,#298032,#298033,#298034,#298035,#298036,
#298037,#298038,#298039,#298040,#298041,#298042,#298043,#298044,#298045,
#298046,#298047,#298048,#298049,#298050,#298051,#298052,#298053,#298054,
#298055,#298056,#298057,#298058,#298059,#298060,#298061,#298062,#298063,
#298064,#298065,#298066,#298067,#298068,#298069,#298070,#298071,#298072,
#298073,#298074,#298075,#298076,#298077,#298078,#298079,#298080,#298081,
#298082,#298083,#298084,#298085,#298086,#298087,#298088,#298089,#298090,
#298091,#298092,#298093,#298094,#298095,#298096,#298097,#298098,#298099,
#298100,#298101,#298102,#298103,#298104,#298105,#298106,#298107,#298108,
#298109,#298110,#298111,#298112,#298113,#298114,#298115,#298116,#298117,
#298118,#298119,#298120,#298121,#298122,#298123,#298124,#298125,#298126,
#298127,#298128,#298129,#298130,#298131,#298132,#298133,#298134,#298135,
#298136,#298137,#298138,#298139,#298140,#298141,#298142,#298143,#298144,
#298145,#298146,#298147,#298148,#298149,#298150,#298151,#298152,#298153,
#298154,#298155,#298156,#298157,#298158,#298159,#298160,#298161,#298162,
#298163,#298164,#298165,#298166,#298167,#298168,#298169,#298170,#298171,
#298172,#298173,#298174,#298175,#298176,#298177,#298178,#298179,#298180,
#298181,#298182,#298183,#298184,#298185,#298186,#298187,#298188,#298189,
#298190,#298191,#298192,#298193,#298194,#298195,#298196,#298197,#298198,
#298199,#298200,#298201,#298202,#298203,#298204,#298205,#298206,#298207,
#298208,#298209,#298210,#298211,#298212,#298213,#298214,#298215,#298216,
#298217,#298218,#298219,#298220,#298221,#298222,#298223,#298224,#298225,
#298226,#298227,#298228,#298229,#298230,#298231,#298232)),.UNSPECIFIED.,
 .F.,.F.,.F.)
B_SPLINE_SURFACE_WITH_KNOTS((2,2),(3,2,2,2,2,2,2,2,2,2,2,2,2,2,2,2,2,2,
2,2,2,2,2,2,2,2,2,2,2,2,2,2,2,2,2,2,2,2,2,2,2,2,2,2,2,2,2,2,2,2,2,2,2,2,
2,2,2,2,2,2,2,2,2,2,2,2,2,2,2,2,2,2,2,2,2,2,2,2,2,2,2,2,2,2,2,2,2,2,2,2,
2,2,2,2,2,2,2,2,2,2,2,2,2,2,2,2,2,2,2,2,2,2,2,2,2,2,2,2,2,2,2,2,2,2,2,2,
2,2,2,2,2,2,2,2,2,2,2,2,2,2,2,2,2,2,2,2,2,2,2,2,2,2,2,2,2,2,2,2,2,2,2,2,
2,2,2,2,2,2,2,2,2,2,2,2,2,2,2,2,2,2,2,2,2,2,2,2,2,2,2,2,2,2,2,2,2,2,2,2,
2,2,2,2,2,2,2,2,2,2,2,2,2,2,2,2,2,2,2,2,2,2,2,2,2,2,2,2,2,2,2,2,2,2,2,2,
2,2,2,2,2,2,2,2,2,2,2,2,2,2,2,2,2,2,2,2,2,2,2,2,2,2,2,2,2,2,2,2,2,2,2,2,
2,2,2,2,2,2,2,2,2,2,2,2,2,2,2,2,2,2,2,2,2,2,2,2,2,2,2,2,2,2,2,2,2,2,2,2,
2,2,2,2,2,2,2,2,2,2,2,2,2,2,2,2,2,2,2,2,2,2,2,2,2,2,2,2,2,2,2,2,2,2,2,2,
2,2,2,2,2,2,2,2,2,2,2,2,2,2,2,2,2,2,2,2,2,2,2,2,2,2,2,2,2,2,2,2,2,2,2,2,
2,2,2,2,2,2,2,2,2,2,2,2,2,2,2,2,2,2,2,2,2,2,2,2,2,2,2,2,2,2,2,2,2,2,2,2,
2,2,2,2,2,2,2,2,2,2,2,2,2,2,2,2,2,2,2,2,2,2,2,2,2,2,2,2,2,2,2,2,2,2,2,2,
2,2,2,2,2,2,2,2,2,2,2,2,2,2,2,2,2,2,2,2,2,2,2,2,2,2,2,2,2,2,2,2,2,2,2,2,
2,2,2,2,2,2,2,2,2,2,2,2,2,2,2,2,2,2,2,2,2,2,2,2,2,2,2,2,2,2,2,2,3),(0.,
1.),(0.,0.00192307692307692,0.00384615384615385,0.00576923076923077,0.00769230769230769,
0.00961538461538462,0.0115384615384615,0.0134615384615385,0.0153846153846154,
0.0173076923076923,0.0192307692307692,0.0211538461538462,0.0230769230769231,
0.025,0.0269230769230769,0.0288461538461538,0.0307692307692308,0.0326923076923077,
0.0346153846153846,0.0365384615384615,0.0384615384615385,0.0403846153846154,
0.0423076923076923,0.0442307692307692,0.0461538461538462,0.0480769230769231,
0.05,0.0519230769230769,0.0538461538461538,0.0557692307692308,0.0576923076923077,
0.0596153846153846,0.0615384615384615,0.0634615384615385,0.0653846153846154,
0.0673076923076923,0.0692307692307692,0.0711538461538462,0.0730769230769231,
0.075,0.0769230769230769,0.0788461538461538,0.0807692307692308,0.0826923076923077,
0.0846153846153846,0.0865384615384615,0.0884615384615385,0.0903846153846154,
0.0923076923076923,0.0942307692307692,0.0961538461538462,0.0980769230769231,
0.1,0.101923076923077,0.103846153846154,0.105769230769231,0.107692307692308,
0.109615384615385,0.111538461538462,0.113461538461538,0.115384615384615,
0.117307692307692,0.119230769230769,0.121153846153846,0.123076923076923,
0.125,0.126923076923077,0.128846153846154,0.130769230769231,0.132692307692308,
0.134615384615385,0.136538461538462,0.138461538461538,0.140384615384615,
0.142307692307692,0.144230769230769,0.146153846153846,0.148076923076923,
0.15,0.151923076923077,0.153846153846154,0.155769230769231,0.157692307692308,
0.159615384615385,0.161538461538462,0.163461538461538,0.165384615384615,
0.167307692307692,0.169230769230769,0.171153846153846,0.173076923076923,
0.175,0.176923076923077,0.178846153846154,0.180769230769231,0.182692307692308,
0.184615384615385,0.186538461538462,0.188461538461538,0.190384615384615,
0.192307692307692,0.194230769230769,0.196153846153846,0.198076923076923,
0.2,0.201923076923077,0.203846153846154,0.205769230769231,0.207692307692308,
0.209615384615385,0.211538461538462,0.213461538461538,0.215384615384615,
0.217307692307692,0.219230769230769,0.221153846153846,0.223076923076923,
0.225,0.226923076923077,0.228846153846154,0.230769230769231,0.232692307692308,
0.234615384615385,0.236538461538462,0.238461538461538,0.240384615384615,
0.242307692307692,0.244230769230769,0.246153846153846,0.248076923076923,
0.25,0.251923076923077,0.253846153846154,0.255769230769231,0.257692307692308,
0.259615384615385,0.261538461538462,0.263461538461538,0.265384615384615,
0.267307692307692,0.269230769230769,0.271153846153846,0.273076923076923,
0.275,0.276923076923077,0.278846153846154,0.280769230769231,0.282692307692308,
0.284615384615385,0.286538461538462,0.288461538461538,0.290384615384615,
0.292307692307692,0.294230769230769,0.296153846153846,0.298076923076923,
0.3,0.301923076923077,0.303846153846154,0.305769230769231,0.307692307692308,
0.309615384615385,0.311538461538462,0.313461538461538,0.315384615384615,
0.317307692307692,0.319230769230769,0.321153846153846,0.323076923076923,
0.325,0.326923076923077,0.328846153846154,0.330769230769231,0.332692307692308,
0.334615384615385,0.336538461538462,0.338461538461538,0.340384615384615,
0.342307692307692,0.344230769230769,0.346153846153846,0.348076923076923,
0.35,0.351923076923077,0.353846153846154,0.355769230769231,0.357692307692308,
0.359615384615385,0.361538461538462,0.363461538461538,0.365384615384615,
0.367307692307692,0.369230769230769,0.371153846153846,0.373076923076923,
0.375,0.376923076923077,0.378846153846154,0.380769230769231,0.382692307692308,
0.384615384615385,0.386538461538462,0.388461538461538,0.390384615384615,
0.392307692307692,0.394230769230769,0.396153846153846,0.398076923076923,
0.4,0.401923076923077,0.403846153846154,0.405769230769231,0.407692307692308,
0.409615384615385,0.411538461538462,0.413461538461538,0.415384615384615,
0.417307692307692,0.419230769230769,0.421153846153846,0.423076923076923,
0.425,0.426923076923077,0.428846153846154,0.430769230769231,0.432692307692308,
0.434615384615385,0.436538461538462,0.438461538461538,0.440384615384615,
0.442307692307692,0.444230769230769,0.446153846153846,0.448076923076923,
0.45,0.451923076923077,0.453846153846154,0.455769230769231,0.457692307692308,
0.459615384615385,0.461538461538462,0.463461538461538,0.465384615384615,
0.467307692307692,0.469230769230769,0.471153846153846,0.473076923076923,
0.475,0.476923076923077,0.478846153846154,0.480769230769231,0.482692307692308,
0.484615384615385,0.486538461538462,0.488461538461538,0.490384615384615,
0.492307692307692,0.494230769230769,0.496153846153846,0.498076923076923,
0.5,0.501923076923077,0.503846153846154,0.505769230769231,0.507692307692308,
0.509615384615385,0.511538461538461,0.513461538461538,0.515384615384615,
0.517307692307692,0.519230769230769,0.521153846153846,0.523076923076923,
0.525,0.526923076923077,0.528846153846154,0.530769230769231,0.532692307692308,
0.534615384615385,0.536538461538462,0.538461538461538,0.540384615384615,
0.542307692307692,0.544230769230769,0.546153846153846,0.548076923076923,
0.55,0.551923076923077,0.553846153846154,0.555769230769231,0.557692307692308,
0.559615384615385,0.561538461538462,0.563461538461538,0.565384615384615,
0.567307692307692,0.569230769230769,0.571153846153846,0.573076923076923,
0.575,0.576923076923077,0.578846153846154,0.580769230769231,0.582692307692308,
0.584615384615385,0.586538461538462,0.588461538461538,0.590384615384615,
0.592307692307692,0.594230769230769,0.596153846153846,0.598076923076923,
0.6,0.601923076923077,0.603846153846154,0.605769230769231,0.607692307692308,
0.609615384615385,0.611538461538462,0.613461538461539,0.615384615384615,
0.617307692307692,0.619230769230769,0.621153846153846,0.623076923076923,
0.625,0.626923076923077,0.628846153846154,0.630769230769231,0.632692307692308,
0.634615384615385,0.636538461538461,0.638461538461538,0.640384615384615,
0.642307692307692,0.644230769230769,0.646153846153846,0.648076923076923,
0.65,0.651923076923077,0.653846153846154,0.655769230769231,0.657692307692308,
0.659615384615385,0.661538461538462,0.663461538461538,0.665384615384615,
0.667307692307692,0.669230769230769,0.671153846153846,0.673076923076923,
0.675,0.676923076923077,0.678846153846154,0.680769230769231,0.682692307692308,
0.684615384615385,0.686538461538462,0.688461538461538,0.690384615384615,
0.692307692307692,0.694230769230769,0.696153846153846,0.698076923076923,
0.7,0.701923076923077,0.703846153846154,0.705769230769231,0.707692307692308,
0.709615384615385,0.711538461538462,0.713461538461538,0.715384615384615,
0.717307692307692,0.719230769230769,0.721153846153846,0.723076923076923,
0.725,0.726923076923077,0.728846153846154,0.730769230769231,0.732692307692308,
0.734615384615385,0.736538461538462,0.738461538461539,0.740384615384615,
0.742307692307692,0.744230769230769,0.746153846153846,0.748076923076923,
0.75,0.751923076923077,0.753846153846154,0.755769230769231,0.757692307692308,
0.759615384615385,0.761538461538461,0.763461538461538,0.765384615384615,
0.767307692307692,0.769230769230769,0.771153846153846,0.773076923076923,
0.775,0.776923076923077,0.778846153846154,0.780769230769231,0.782692307692308,
0.784615384615385,0.786538461538462,0.788461538461538,0.790384615384615,
0.792307692307692,0.794230769230769,0.796153846153846,0.798076923076923,
0.8,0.801923076923077,0.803846153846154,0.805769230769231,0.807692307692308,
0.809615384615385,0.811538461538462,0.813461538461538,0.815384615384615,
0.817307692307692,0.819230769230769,0.821153846153846,0.823076923076923,
0.825,0.826923076923077,0.828846153846154,0.830769230769231,0.832692307692308,
0.834615384615385,0.836538461538462,0.838461538461538,0.840384615384615,
0.842307692307692,0.844230769230769,0.846153846153846,0.848076923076923,
0.85,0.851923076923077,0.853846153846154,0.855769230769231,0.857692307692308,
0.859615384615385,0.861538461538462,0.863461538461539,0.865384615384615,
0.867307692307692,0.869230769230769,0.871153846153846,0.873076923076923,
0.875,0.876923076923077,0.878846153846154,0.880769230769231,0.882692307692308,
0.884615384615385,0.886538461538461,0.888461538461538,0.890384615384615,
0.892307692307692,0.894230769230769,0.896153846153846,0.898076923076923,
0.9,0.901923076923077,0.903846153846154,0.905769230769231,0.907692307692308,
0.909615384615385,0.911538461538462,0.913461538461538,0.915384615384615,
0.917307692307692,0.919230769230769,0.921153846153846,0.923076923076923,
0.925,0.926923076923077,0.928846153846154,0.930769230769231,0.932692307692308,
0.934615384615385,0.936538461538462,0.938461538461538,0.940384615384615,
0.942307692307692,0.944230769230769,0.946153846153846,0.948076923076923,
0.95,0.951923076923077,0.953846153846154,0.955769230769231,0.957692307692308,
0.959615384615385,0.961538461538462,0.963461538461538,0.965384615384615,
0.967307692307692,0.969230769230769,0.971153846153846,0.973076923076923,
0.975,0.976923076923077,0.978846153846154,0.980769230769231,0.982692307692308,
0.984615384615385,0.986538461538462,0.988461538461539,0.990384615384615,
0.992307692307692,0.994230769230769,0.996153846153846),.UNSPECIFIED.)
GEOMETRIC_REPRESENTATION_ITEM()
RATIONAL_B_SPLINE_SURFACE(((1.,0.951056516295154,1.,0.951056516295154,1.,
0.951056516295154,1.,0.951056516295154,1.,0.951056516295154,1.,0.951056516295154,
1.,0.951056516295154,1.,0.951056516295154,1.,0.951056516295154,1.,0.951056516295154,
1.,0.951056516295154,1.,0.951056516295154,1.,0.951056516295154,1.,0.951056516295154,
1.,0.951056516295154,1.,0.951056516295154,1.,0.951056516295154,1.,0.951056516295154,
1.,0.951056516295154,1.,0.951056516295154,1.,0.951056516295154,1.,0.951056516295154,
1.,0.951056516295154,1.,0.951056516295154,1.,0.951056516295154,1.,0.951056516295154,
1.,0.951056516295154,1.,0.951056516295154,1.,0.951056516295154,1.,0.951056516295154,
1.,0.951056516295154,1.,0.951056516295154,1.,0.951056516295154,1.,0.951056516295154,
1.,0.951056516295154,1.,0.951056516295154,1.,0.951056516295154,1.,0.951056516295154,
1.,0.951056516295154,1.,0.951056516295154,1.,0.951056516295154,1.,0.951056516295154,
1.,0.951056516295154,1.,0.951056516295154,1.,0.951056516295154,1.,0.951056516295154,
1.,0.951056516295154,1.,0.951056516295154,1.,0.951056516295154,1.,0.951056516295154,
1.,0.951056516295154,1.,0.951056516295154,1.,0.951056516295154,1.,0.951056516295154,
1.,0.951056516295154,1.,0.951056516295154,1.,0.951056516295154,1.,0.951056516295154,
1.,0.951056516295154,1.,0.951056516295154,1.,0.951056516295154,1.,0.951056516295154,
1.,0.951056516295154,1.,0.951056516295154,1.,0.951056516295154,1.,0.951056516295154,
1.,0.951056516295154,1.,0.951056516295154,1.,0.951056516295154,1.,0.951056516295154,
1.,0.951056516295154,1.,0.951056516295154,1.,0.951056516295154,1.,0.951056516295154,
1.,0.951056516295154,1.,0.951056516295154,1.,0.951056516295154,1.,0.951056516295154,
1.,0.951056516295154,1.,0.951056516295154,1.,0.951056516295154,1.,0.951056516295154,
1.,0.951056516295154,1.,0.951056516295154,1.,0.951056516295154,1.,0.951056516295154,
1.,0.951056516295154,1.,0.951056516295154,1.,0.951056516295154,1.,0.951056516295154,
1.,0.951056516295154,1.,0.951056516295154,1.,0.951056516295154,1.,0.951056516295154,
1.,0.951056516295154,1.,0.951056516295154,1.,0.951056516295154,1.,0.951056516295154,
1.,0.951056516295154,1.,0.951056516295154,1.,0.951056516295154,1.,0.951056516295154,
1.,0.951056516295154,1.,0.951056516295154,1.,0.951056516295154,1.,0.951056516295154,
1.,0.951056516295154,1.,0.951056516295154,1.,0.951056516295154,1.,0.951056516295154,
1.,0.951056516295154,1.,0.951056516295154,1.,0.951056516295154,1.,0.951056516295154,
1.,0.951056516295154,1.,0.951056516295154,1.,0.951056516295154,1.,0.951056516295154,
1.,0.951056516295154,1.,0.951056516295154,1.,0.951056516295154,1.,0.951056516295154,
1.,0.951056516295154,1.,0.951056516295154,1.,0.951056516295154,1.,0.951056516295154,
1.,0.951056516295154,1.,0.951056516295154,1.,0.951056516295154,1.,0.951056516295154,
1.,0.951056516295154,1.,0.951056516295154,1.,0.951056516295154,1.,0.951056516295154,
1.,0.951056516295154,1.,0.951056516295154,1.,0.951056516295154,1.,0.951056516295154,
1.,0.951056516295154,1.,0.951056516295154,1.,0.951056516295154,1.,0.951056516295154,
1.,0.951056516295154,1.,0.951056516295154,1.,0.951056516295154,1.,0.951056516295154,
1.,0.951056516295154,1.,0.951056516295154,1.,0.951056516295154,1.,0.951056516295154,
1.,0.951056516295154,1.,0.951056516295154,1.,0.951056516295154,1.,0.951056516295154,
1.,0.951056516295154,1.,0.951056516295154,1.,0.951056516295154,1.,0.951056516295154,
1.,0.951056516295154,1.,0.951056516295154,1.,0.951056516295154,1.,0.951056516295154,
1.,0.951056516295154,1.,0.951056516295154,1.,0.951056516295154,1.,0.951056516295154,
1.,0.951056516295154,1.,0.951056516295154,1.,0.951056516295154,1.,0.951056516295154,
1.,0.951056516295154,1.,0.951056516295154,1.,0.951056516295154,1.,0.951056516295154,
1.,0.951056516295154,1.,0.951056516295154,1.,0.951056516295154,1.,0.951056516295154,
1.,0.951056516295154,1.,0.951056516295154,1.,0.951056516295154,1.,0.951056516295154,
1.,0.951056516295154,1.,0.951056516295154,1.,0.951056516295154,1.,0.951056516295154,
1.,0.951056516295154,1.,0.951056516295154,1.,0.951056516295154,1.,0.951056516295154,
1.,0.951056516295154,1.,0.951056516295154,1.,0.951056516295154,1.,0.951056516295154,
1.,0.951056516295154,1.,0.951056516295154,1.,0.951056516295154,1.,0.951056516295154,
1.,0.951056516295154,1.,0.951056516295154,1.,0.951056516295154,1.,0.951056516295154,
1.,0.951056516295154,1.,0.951056516295154,1.,0.951056516295154,1.,0.951056516295154,
1.,0.951056516295154,1.,0.951056516295154,1.,0.951056516295154,1.,0.951056516295154,
1.,0.951056516295154,1.,0.951056516295154,1.,0.951056516295154,1.,0.951056516295154,
1.,0.951056516295154,1.,0.951056516295154,1.,0.951056516295154,1.,0.951056516295154,
1.,0.951056516295154,1.,0.951056516295154,1.,0.951056516295154,1.,0.951056516295154,
1.,0.951056516295154,1.,0.951056516295154,1.,0.951056516295154,1.,0.951056516295154,
1.,0.951056516295154,1.,0.951056516295154,1.,0.951056516295154,1.,0.951056516295154,
1.,0.951056516295154,1.,0.951056516295154,1.,0.951056516295154,1.,0.951056516295154,
1.,0.951056516295154,1.,0.951056516295154,1.,0.951056516295154,1.,0.951056516295154,
1.,0.951056516295154,1.,0.951056516295154,1.,0.951056516295154,1.,0.951056516295154,
1.,0.951056516295154,1.,0.951056516295154,1.,0.951056516295154,1.,0.951056516295154,
1.,0.951056516295154,1.,0.951056516295154,1.,0.951056516295154,1.,0.951056516295154,
1.,0.951056516295154,1.,0.951056516295154,1.,0.951056516295154,1.,0.951056516295154,
1.,0.951056516295154,1.,0.951056516295154,1.,0.951056516295154,1.,0.951056516295154,
1.,0.951056516295154,1.,0.951056516295154,1.,0.951056516295154,1.,0.951056516295154,
1.,0.951056516295154,1.,0.951056516295154,1.,0.951056516295154,1.,0.951056516295154,
1.,0.951056516295154,1.,0.951056516295154,1.,0.951056516295154,1.,0.951056516295154,
1.,0.951056516295154,1.,0.951056516295154,1.,0.951056516295154,1.,0.951056516295154,
1.,0.951056516295154,1.,0.951056516295154,1.,0.951056516295154,1.,0.951056516295154,
1.,0.951056516295154,1.,0.951056516295154,1.,0.951056516295154,1.,0.951056516295154,
1.,0.951056516295154,1.,0.951056516295154,1.,0.951056516295154,1.,0.951056516295154,
1.,0.951056516295154,1.,0.951056516295154,1.,0.951056516295154,1.,0.951056516295154,
1.,0.951056516295154,1.,0.951056516295154,1.,0.951056516295154,1.,0.951056516295154,
1.,0.951056516295154,1.,0.951056516295154,1.,0.951056516295154,1.,0.951056516295154,
1.,0.951056516295154,1.,0.951056516295154,1.,0.951056516295154,1.,0.951056516295154,
1.,0.951056516295154,1.,0.951056516295154,1.,0.951056516295154,1.,0.951056516295154,
1.,0.951056516295154,1.,0.951056516295154,1.,0.951056516295154,1.,0.951056516295154,
1.,0.951056516295154,1.,0.951056516295154,1.,0.951056516295154,1.,0.951056516295154,
1.,0.951056516295154,1.,0.951056516295154,1.,0.951056516295154,1.,0.951056516295154,
1.,0.951056516295154,1.,0.951056516295154,1.,0.951056516295154,1.,0.951056516295154,
1.,0.951056516295154,1.,0.951056516295154,1.,0.951056516295154,1.,0.951056516295154,
1.,0.951056516295154,1.,0.951056516295154,1.,0.951056516295154,1.,0.951056516295154,
1.,0.951056516295154,1.,0.951056516295154,1.,0.951056516295154,1.,0.951056516295154,
1.,0.951056516295154,1.,0.951056516295154,1.,0.951056516295154,1.,0.951056516295154,
1.,0.951056516295154,1.,0.951056516295154,1.,0.951056516295154,1.,0.951056516295154,
1.,0.951056516295154,1.,0.951056516295154,1.,0.951056516295154,1.,0.951056516295154,
1.,0.951056516295154,1.,0.951056516295154,1.,0.951056516295154,1.,0.951056516295154,
1.,0.951056516295154,1.,0.951056516295154,1.,0.951056516295154,1.,0.951056516295154,
1.,0.951056516295154,1.,0.951056516295154,1.,0.951056516295154,1.,0.951056516295154,
1.,0.951056516295154,1.,0.951056516295154,1.,0.951056516295154,1.,0.951056516295154,
1.,0.951056516295154,1.,0.951056516295154,1.,0.951056516295154,1.,0.951056516295154,
1.,0.951056516295154,1.,0.951056516295154,1.,0.951056516295154,1.,0.951056516295154,
1.,0.951056516295154,1.,0.951056516295154,1.,0.951056516295154,1.,0.951056516295154,
1.,0.951056516295154,1.,0.951056516295154,1.,0.951056516295154,1.,0.951056516295154,
1.,0.951056516295154,1.,0.951056516295154,1.,0.951056516295154,1.,0.951056516295154,
1.,0.951056516295154,1.,0.951056516295154,1.,0.951056516295154,1.,0.951056516295154,
1.,0.951056516295154,1.,0.951056516295154,1.,0.951056516295154,1.,0.951056516295154,
1.,0.951056516295154,1.,0.951056516295154,1.,0.951056516295154,1.,0.951056516295154,
1.,0.951056516295154,1.,0.951056516295154,1.,0.951056516295154,1.,0.951056516295154,
1.,0.951056516295154,1.,0.951056516295154,1.,0.951056516295154,1.,0.951056516295154,
1.,0.951056516295154,1.,0.951056516295154,1.,0.951056516295154,1.,0.951056516295154,
1.,0.951056516295154,1.,0.951056516295154,1.,0.951056516295154,1.,0.951056516295154,
1.,0.951056516295154,1.,0.951056516295154,1.,0.951056516295154,1.,0.951056516295154,
1.,0.951056516295154,1.,0.951056516295154,1.,0.951056516295154,1.,0.951056516295154,
1.,0.951056516295154,1.,0.951056516295154,1.,0.951056516295154,1.,0.951056516295154,
1.,0.951056516295154,1.,0.951056516295154,1.,0.951056516295154,1.,0.951056516295154,
1.,0.951056516295154,1.,0.951056516295154,1.,0.951056516295154,1.,0.951056516295154,
1.,0.951056516295154,1.,0.951056516295154,1.,0.951056516295154,1.,0.951056516295154,
1.,0.951056516295154,1.,0.951056516295154,1.,0.951056516295154,1.,0.951056516295154,
1.,0.951056516295154,1.,0.951056516295154,1.,0.951056516295154,1.,0.951056516295154,
1.,0.951056516295154,1.,0.951056516295154,1.,0.951056516295154,1.,0.951056516295154,
1.,0.951056516295154,1.,0.951056516295154,1.,0.951056516295154,1.,0.951056516295154,
1.,0.951056516295154,1.,0.951056516295154,1.,0.951056516295154,1.,0.951056516295154,
1.,0.951056516295154,1.,0.951056516295154,1.,0.951056516295154,1.,0.951056516295154,
1.,0.951056516295154,1.,0.951056516295154,1.,0.951056516295154,1.,0.951056516295154,
1.,0.951056516295154,1.,0.951056516295154,1.,0.951056516295154,1.,0.951056516295154,
1.,0.951056516295154,1.,0.951056516295154,1.,0.951056516295154,1.,0.951056516295154,
1.,0.951056516295154,1.,0.951056516295154,1.,0.951056516295154,1.,0.951056516295154,
1.,0.951056516295154,1.,0.951056516295154,1.,0.951056516295154,1.,0.951056516295154,
1.,0.951056516295154,1.,0.951056516295154,1.,0.951056516295154,1.,0.951056516295154,
1.,0.951056516295154,1.,0.951056516295154,1.,0.951056516295154,1.,0.951056516295154,
1.,0.951056516295154,1.,0.951056516295154,1.,0.951056516295154,1.,0.951056516295154,
1.,0.951056516295154,1.,0.951056516295154,1.,0.951056516295154,1.,0.951056516295154,
1.,0.951056516295154,1.,0.951056516295154,1.,0.951056516295154,1.,0.951056516295154,
1.,0.951056516295154,1.,0.951056516295154,1.,0.951056516295154,1.,0.951056516295154,
1.,0.951056516295154,1.,0.951056516295154,1.,0.951056516295154,1.,0.951056516295154,
1.,0.951056516295154,1.,0.951056516295154,1.,0.951056516295154,1.,0.951056516295154,
1.,0.951056516295154,1.,0.951056516295154,1.,0.951056516295154,1.,0.951056516295154,
1.,0.951056516295154,1.,0.951056516295154,1.,0.951056516295154,1.,0.951056516295154,
1.),(1.,0.951056516295154,1.,0.951056516295154,1.,0.951056516295154,1.,
0.951056516295154,1.,0.951056516295154,1.,0.951056516295154,1.,0.951056516295154,
1.,0.951056516295154,1.,0.951056516295154,1.,0.951056516295154,1.,0.951056516295154,
1.,0.951056516295154,1.,0.951056516295154,1.,0.951056516295154,1.,0.951056516295154,
1.,0.951056516295154,1.,0.951056516295154,1.,0.951056516295154,1.,0.951056516295154,
1.,0.951056516295154,1.,0.951056516295154,1.,0.951056516295154,1.,0.951056516295154,
1.,0.951056516295154,1.,0.951056516295154,1.,0.951056516295154,1.,0.951056516295154,
1.,0.951056516295154,1.,0.951056516295154,1.,0.951056516295154,1.,0.951056516295154,
1.,0.951056516295154,1.,0.951056516295154,1.,0.951056516295154,1.,0.951056516295154,
1.,0.951056516295154,1.,0.951056516295154,1.,0.951056516295154,1.,0.951056516295154,
1.,0.951056516295154,1.,0.951056516295154,1.,0.951056516295154,1.,0.951056516295154,
1.,0.951056516295154,1.,0.951056516295154,1.,0.951056516295154,1.,0.951056516295154,
1.,0.951056516295154,1.,0.951056516295154,1.,0.951056516295154,1.,0.951056516295154,
1.,0.951056516295154,1.,0.951056516295154,1.,0.951056516295154,1.,0.951056516295154,
1.,0.951056516295154,1.,0.951056516295154,1.,0.951056516295154,1.,0.951056516295154,
1.,0.951056516295154,1.,0.951056516295154,1.,0.951056516295154,1.,0.951056516295154,
1.,0.951056516295154,1.,0.951056516295154,1.,0.951056516295154,1.,0.951056516295154,
1.,0.951056516295154,1.,0.951056516295154,1.,0.951056516295154,1.,0.951056516295154,
1.,0.951056516295154,1.,0.951056516295154,1.,0.951056516295154,1.,0.951056516295154,
1.,0.951056516295154,1.,0.951056516295154,1.,0.951056516295154,1.,0.951056516295154,
1.,0.951056516295154,1.,0.951056516295154,1.,0.951056516295154,1.,0.951056516295154,
1.,0.951056516295154,1.,0.951056516295154,1.,0.951056516295154,1.,0.951056516295154,
1.,0.951056516295154,1.,0.951056516295154,1.,0.951056516295154,1.,0.951056516295154,
1.,0.951056516295154,1.,0.951056516295154,1.,0.951056516295154,1.,0.951056516295154,
1.,0.951056516295154,1.,0.951056516295154,1.,0.951056516295154,1.,0.951056516295154,
1.,0.951056516295154,1.,0.951056516295154,1.,0.951056516295154,1.,0.951056516295154,
1.,0.951056516295154,1.,0.951056516295154,1.,0.951056516295154,1.,0.951056516295154,
1.,0.951056516295154,1.,0.951056516295154,1.,0.951056516295154,1.,0.951056516295154,
1.,0.951056516295154,1.,0.951056516295154,1.,0.951056516295154,1.,0.951056516295154,
1.,0.951056516295154,1.,0.951056516295154,1.,0.951056516295154,1.,0.951056516295154,
1.,0.951056516295154,1.,0.951056516295154,1.,0.951056516295154,1.,0.951056516295154,
1.,0.951056516295154,1.,0.951056516295154,1.,0.951056516295154,1.,0.951056516295154,
1.,0.951056516295154,1.,0.951056516295154,1.,0.951056516295154,1.,0.951056516295154,
1.,0.951056516295154,1.,0.951056516295154,1.,0.951056516295154,1.,0.951056516295154,
1.,0.951056516295154,1.,0.951056516295154,1.,0.951056516295154,1.,0.951056516295154,
1.,0.951056516295154,1.,0.951056516295154,1.,0.951056516295154,1.,0.951056516295154,
1.,0.951056516295154,1.,0.951056516295154,1.,0.951056516295154,1.,0.951056516295154,
1.,0.951056516295154,1.,0.951056516295154,1.,0.951056516295154,1.,0.951056516295154,
1.,0.951056516295154,1.,0.951056516295154,1.,0.951056516295154,1.,0.951056516295154,
1.,0.951056516295154,1.,0.951056516295154,1.,0.951056516295154,1.,0.951056516295154,
1.,0.951056516295154,1.,0.951056516295154,1.,0.951056516295154,1.,0.951056516295154,
1.,0.951056516295154,1.,0.951056516295154,1.,0.951056516295154,1.,0.951056516295154,
1.,0.951056516295154,1.,0.951056516295154,1.,0.951056516295154,1.,0.951056516295154,
1.,0.951056516295154,1.,0.951056516295154,1.,0.951056516295154,1.,0.951056516295154,
1.,0.951056516295154,1.,0.951056516295154,1.,0.951056516295154,1.,0.951056516295154,
1.,0.951056516295154,1.,0.951056516295154,1.,0.951056516295154,1.,0.951056516295154,
1.,0.951056516295154,1.,0.951056516295154,1.,0.951056516295154,1.,0.951056516295154,
1.,0.951056516295154,1.,0.951056516295154,1.,0.951056516295154,1.,0.951056516295154,
1.,0.951056516295154,1.,0.951056516295154,1.,0.951056516295154,1.,0.951056516295154,
1.,0.951056516295154,1.,0.951056516295154,1.,0.951056516295154,1.,0.951056516295154,
1.,0.951056516295154,1.,0.951056516295154,1.,0.951056516295154,1.,0.951056516295154,
1.,0.951056516295154,1.,0.951056516295154,1.,0.951056516295154,1.,0.951056516295154,
1.,0.951056516295154,1.,0.951056516295154,1.,0.951056516295154,1.,0.951056516295154,
1.,0.951056516295154,1.,0.951056516295154,1.,0.951056516295154,1.,0.951056516295154,
1.,0.951056516295154,1.,0.951056516295154,1.,0.951056516295154,1.,0.951056516295154,
1.,0.951056516295154,1.,0.951056516295154,1.,0.951056516295154,1.,0.951056516295154,
1.,0.951056516295154,1.,0.951056516295154,1.,0.951056516295154,1.,0.951056516295154,
1.,0.951056516295154,1.,0.951056516295154,1.,0.951056516295154,1.,0.951056516295154,
1.,0.951056516295154,1.,0.951056516295154,1.,0.951056516295154,1.,0.951056516295154,
1.,0.951056516295154,1.,0.951056516295154,1.,0.951056516295154,1.,0.951056516295154,
1.,0.951056516295154,1.,0.951056516295154,1.,0.951056516295154,1.,0.951056516295154,
1.,0.951056516295154,1.,0.951056516295154,1.,0.951056516295154,1.,0.951056516295154,
1.,0.951056516295154,1.,0.951056516295154,1.,0.951056516295154,1.,0.951056516295154,
1.,0.951056516295154,1.,0.951056516295154,1.,0.951056516295154,1.,0.951056516295154,
1.,0.951056516295154,1.,0.951056516295154,1.,0.951056516295154,1.,0.951056516295154,
1.,0.951056516295154,1.,0.951056516295154,1.,0.951056516295154,1.,0.951056516295154,
1.,0.951056516295154,1.,0.951056516295154,1.,0.951056516295154,1.,0.951056516295154,
1.,0.951056516295154,1.,0.951056516295154,1.,0.951056516295154,1.,0.951056516295154,
1.,0.951056516295154,1.,0.951056516295154,1.,0.951056516295154,1.,0.951056516295154,
1.,0.951056516295154,1.,0.951056516295154,1.,0.951056516295154,1.,0.951056516295154,
1.,0.951056516295154,1.,0.951056516295154,1.,0.951056516295154,1.,0.951056516295154,
1.,0.951056516295154,1.,0.951056516295154,1.,0.951056516295154,1.,0.951056516295154,
1.,0.951056516295154,1.,0.951056516295154,1.,0.951056516295154,1.,0.951056516295154,
1.,0.951056516295154,1.,0.951056516295154,1.,0.951056516295154,1.,0.951056516295154,
1.,0.951056516295154,1.,0.951056516295154,1.,0.951056516295154,1.,0.951056516295154,
1.,0.951056516295154,1.,0.951056516295154,1.,0.951056516295154,1.,0.951056516295154,
1.,0.951056516295154,1.,0.951056516295154,1.,0.951056516295154,1.,0.951056516295154,
1.,0.951056516295154,1.,0.951056516295154,1.,0.951056516295154,1.,0.951056516295154,
1.,0.951056516295154,1.,0.951056516295154,1.,0.951056516295154,1.,0.951056516295154,
1.,0.951056516295154,1.,0.951056516295154,1.,0.951056516295154,1.,0.951056516295154,
1.,0.951056516295154,1.,0.951056516295154,1.,0.951056516295154,1.,0.951056516295154,
1.,0.951056516295154,1.,0.951056516295154,1.,0.951056516295154,1.,0.951056516295154,
1.,0.951056516295154,1.,0.951056516295154,1.,0.951056516295154,1.,0.951056516295154,
1.,0.951056516295154,1.,0.951056516295154,1.,0.951056516295154,1.,0.951056516295154,
1.,0.951056516295154,1.,0.951056516295154,1.,0.951056516295154,1.,0.951056516295154,
1.,0.951056516295154,1.,0.951056516295154,1.,0.951056516295154,1.,0.951056516295154,
1.,0.951056516295154,1.,0.951056516295154,1.,0.951056516295154,1.,0.951056516295154,
1.,0.951056516295154,1.,0.951056516295154,1.,0.951056516295154,1.,0.951056516295154,
1.,0.951056516295154,1.,0.951056516295154,1.,0.951056516295154,1.,0.951056516295154,
1.,0.951056516295154,1.,0.951056516295154,1.,0.951056516295154,1.,0.951056516295154,
1.,0.951056516295154,1.,0.951056516295154,1.,0.951056516295154,1.,0.951056516295154,
1.,0.951056516295154,1.,0.951056516295154,1.,0.951056516295154,1.,0.951056516295154,
1.,0.951056516295154,1.,0.951056516295154,1.,0.951056516295154,1.,0.951056516295154,
1.,0.951056516295154,1.,0.951056516295154,1.,0.951056516295154,1.,0.951056516295154,
1.,0.951056516295154,1.,0.951056516295154,1.,0.951056516295154,1.,0.951056516295154,
1.,0.951056516295154,1.,0.951056516295154,1.,0.951056516295154,1.,0.951056516295154,
1.,0.951056516295154,1.,0.951056516295154,1.,0.951056516295154,1.,0.951056516295154,
1.,0.951056516295154,1.,0.951056516295154,1.,0.951056516295154,1.,0.951056516295154,
1.,0.951056516295154,1.,0.951056516295154,1.,0.951056516295154,1.,0.951056516295154,
1.,0.951056516295154,1.,0.951056516295154,1.,0.951056516295154,1.,0.951056516295154,
1.,0.951056516295154,1.,0.951056516295154,1.,0.951056516295154,1.,0.951056516295154,
1.,0.951056516295154,1.,0.951056516295154,1.,0.951056516295154,1.,0.951056516295154,
1.,0.951056516295154,1.,0.951056516295154,1.,0.951056516295154,1.,0.951056516295154,
1.,0.951056516295154,1.,0.951056516295154,1.,0.951056516295154,1.,0.951056516295154,
1.,0.951056516295154,1.,0.951056516295154,1.,0.951056516295154,1.,0.951056516295154,
1.,0.951056516295154,1.,0.951056516295154,1.,0.951056516295154,1.,0.951056516295154,
1.,0.951056516295154,1.,0.951056516295154,1.,0.951056516295154,1.,0.951056516295154,
1.,0.951056516295154,1.,0.951056516295154,1.,0.951056516295154,1.,0.951056516295154,
1.,0.951056516295154,1.,0.951056516295154,1.,0.951056516295154,1.,0.951056516295154,
1.,0.951056516295154,1.,0.951056516295154,1.,0.951056516295154,1.,0.951056516295154,
1.,0.951056516295154,1.,0.951056516295154,1.,0.951056516295154,1.,0.951056516295154,
1.,0.951056516295154,1.,0.951056516295154,1.,0.951056516295154,1.,0.951056516295154,
1.,0.951056516295154,1.,0.951056516295154,1.,0.951056516295154,1.,0.951056516295154,
1.,0.951056516295154,1.,0.951056516295154,1.,0.951056516295154,1.,0.951056516295154,
1.,0.951056516295154,1.,0.951056516295154,1.,0.951056516295154,1.,0.951056516295154,
1.,0.951056516295154,1.,0.951056516295154,1.,0.951056516295154,1.,0.951056516295154,
1.,0.951056516295154,1.,0.951056516295154,1.,0.951056516295154,1.,0.951056516295154,
1.,0.951056516295154,1.,0.951056516295154,1.,0.951056516295154,1.,0.951056516295154,
1.,0.951056516295154,1.,0.951056516295154,1.,0.951056516295154,1.,0.951056516295154,
1.,0.951056516295154,1.,0.951056516295154,1.,0.951056516295154,1.,0.951056516295154,
1.,0.951056516295154,1.,0.951056516295154,1.,0.951056516295154,1.,0.951056516295154,
1.,0.951056516295154,1.,0.951056516295154,1.,0.951056516295154,1.,0.951056516295154,
1.,0.951056516295154,1.,0.951056516295154,1.,0.951056516295154,1.,0.951056516295154,
1.,0.951056516295154,1.,0.951056516295154,1.,0.951056516295154,1.,0.951056516295154,
1.,0.951056516295154,1.,0.951056516295154,1.,0.951056516295154,1.,0.951056516295154,
1.,0.951056516295154,1.,0.951056516295154,1.,0.951056516295154,1.,0.951056516295154,
1.,0.951056516295154,1.,0.951056516295154,1.,0.951056516295154,1.,0.951056516295154,
1.,0.951056516295154,1.,0.951056516295154,1.,0.951056516295154,1.,0.951056516295154,
1.,0.951056516295154,1.,0.951056516295154,1.,0.951056516295154,1.,0.951056516295154,
1.,0.951056516295154,1.,0.951056516295154,1.,0.951056516295154,1.)))
REPRESENTATION_ITEM('')
SURFACE()
);
#3200=(
BOUNDED_SURFACE()
B_SPLINE_SURFACE(1,2,((#298462,#298463,#298464,#298465,#298466,#298467,
#298468,#298469,#298470,#298471,#298472,#298473,#298474,#298475,#298476,
#298477,#298478,#298479,#298480,#298481,#298482,#298483,#298484,#298485,
#298486,#298487,#298488,#298489,#298490,#298491,#298492,#298493,#298494,
#298495,#298496,#298497,#298498,#298499,#298500,#298501,#298502,#298503,
#298504,#298505,#298506,#298507,#298508,#298509,#298510,#298511,#298512,
#298513,#298514,#298515,#298516,#298517,#298518,#298519,#298520,#298521,
#298522,#298523,#298524,#298525,#298526,#298527,#298528,#298529,#298530,
#298531,#298532,#298533,#298534,#298535,#298536,#298537,#298538,#298539,
#298540,#298541,#298542,#298543,#298544,#298545,#298546,#298547,#298548,
#298549,#298550,#298551,#298552,#298553,#298554,#298555,#298556,#298557,
#298558,#298559,#298560,#298561,#298562,#298563,#298564,#298565,#298566,
#298567,#298568,#298569,#298570,#298571,#298572,#298573,#298574,#298575,
#298576,#298577,#298578,#298579,#298580,#298581,#298582,#298583,#298584,
#298585,#298586,#298587,#298588,#298589,#298590,#298591,#298592,#298593,
#298594,#298595,#298596,#298597,#298598,#298599,#298600,#298601,#298602,
#298603,#298604,#298605,#298606,#298607,#298608,#298609,#298610,#298611,
#298612,#298613,#298614,#298615,#298616,#298617,#298618,#298619,#298620,
#298621,#298622,#298623,#298624,#298625,#298626,#298627,#298628,#298629,
#298630,#298631,#298632,#298633,#298634,#298635,#298636,#298637,#298638,
#298639,#298640,#298641,#298642,#298643,#298644,#298645,#298646,#298647,
#298648,#298649,#298650,#298651,#298652,#298653,#298654,#298655,#298656,
#298657,#298658,#298659,#298660,#298661,#298662,#298663,#298664,#298665,
#298666,#298667,#298668,#298669,#298670,#298671,#298672,#298673,#298674,
#298675,#298676,#298677,#298678,#298679,#298680,#298681,#298682,#298683,
#298684,#298685,#298686,#298687,#298688,#298689,#298690,#298691,#298692,
#298693,#298694,#298695,#298696,#298697,#298698,#298699,#298700,#298701,
#298702,#298703,#298704,#298705,#298706,#298707,#298708,#298709,#298710,
#298711,#298712,#298713,#298714,#298715,#298716,#298717,#298718,#298719,
#298720,#298721,#298722,#298723,#298724,#298725,#298726,#298727,#298728,
#298729,#298730,#298731,#298732,#298733,#298734,#298735,#298736,#298737,
#298738,#298739,#298740,#298741,#298742,#298743,#298744,#298745,#298746,
#298747,#298748,#298749,#298750,#298751,#298752,#298753,#298754,#298755,
#298756,#298757,#298758,#298759,#298760,#298761,#298762,#298763,#298764,
#298765,#298766,#298767,#298768,#298769,#298770,#298771,#298772,#298773,
#298774,#298775,#298776,#298777,#298778,#298779,#298780,#298781,#298782,
#298783,#298784,#298785,#298786,#298787,#298788,#298789,#298790,#298791,
#298792,#298793,#298794,#298795,#298796,#298797,#298798,#298799,#298800,
#298801,#298802,#298803,#298804,#298805,#298806,#298807,#298808,#298809,
#298810,#298811,#298812,#298813,#298814,#298815,#298816,#298817,#298818,
#298819,#298820,#298821,#298822,#298823,#298824,#298825,#298826,#298827,
#298828,#298829,#298830,#298831,#298832,#298833,#298834,#298835,#298836,
#298837,#298838,#298839,#298840,#298841,#298842,#298843,#298844,#298845,
#298846,#298847,#298848,#298849,#298850,#298851,#298852,#298853,#298854,
#298855,#298856,#298857,#298858,#298859,#298860,#298861,#298862,#298863,
#298864,#298865,#298866,#298867,#298868,#298869,#298870,#298871,#298872,
#298873,#298874,#298875,#298876,#298877,#298878,#298879,#298880,#298881,
#298882,#298883,#298884,#298885,#298886,#298887,#298888,#298889,#298890,
#298891,#298892,#298893,#298894,#298895,#298896,#298897,#298898,#298899,
#298900,#298901,#298902,#298903,#298904,#298905,#298906,#298907,#298908,
#298909,#298910,#298911,#298912,#298913,#298914,#298915,#298916,#298917,
#298918,#298919,#298920,#298921,#298922,#298923,#298924,#298925,#298926,
#298927,#298928,#298929,#298930,#298931,#298932,#298933,#298934,#298935,
#298936,#298937,#298938,#298939,#298940,#298941,#298942,#298943,#298944,
#298945,#298946,#298947,#298948,#298949,#298950,#298951,#298952,#298953,
#298954,#298955,#298956,#298957,#298958,#298959,#298960,#298961,#298962,
#298963,#298964,#298965,#298966,#298967,#298968,#298969,#298970,#298971,
#298972,#298973,#298974,#298975,#298976,#298977,#298978,#298979,#298980,
#298981,#298982,#298983,#298984,#298985,#298986,#298987,#298988,#298989,
#298990,#298991,#298992,#298993,#298994,#298995,#298996,#298997,#298998,
#298999,#299000,#299001,#299002,#299003,#299004,#299005,#299006,#299007,
#299008,#299009,#299010,#299011,#299012,#299013,#299014,#299015,#299016,
#299017,#299018,#299019,#299020,#299021,#299022,#299023,#299024,#299025,
#299026,#299027,#299028,#299029,#299030,#299031,#299032,#299033,#299034,
#299035,#299036,#299037,#299038,#299039,#299040,#299041,#299042,#299043,
#299044,#299045,#299046,#299047,#299048,#299049,#299050,#299051,#299052,
#299053,#299054,#299055,#299056,#299057,#299058,#299059,#299060,#299061,
#299062,#299063,#299064,#299065,#299066,#299067,#299068,#299069,#299070,
#299071,#299072,#299073,#299074,#299075,#299076,#299077,#299078,#299079,
#299080,#299081,#299082,#299083,#299084,#299085,#299086,#299087,#299088,
#299089,#299090,#299091,#299092,#299093,#299094,#299095,#299096,#299097,
#299098,#299099,#299100,#299101,#299102,#299103,#299104,#299105,#299106,
#299107,#299108,#299109,#299110,#299111,#299112,#299113,#299114,#299115,
#299116,#299117,#299118,#299119,#299120,#299121,#299122,#299123,#299124,
#299125,#299126,#299127,#299128,#299129,#299130,#299131,#299132,#299133,
#299134,#299135,#299136,#299137,#299138,#299139,#299140,#299141,#299142,
#299143,#299144,#299145,#299146,#299147,#299148,#299149,#299150,#299151,
#299152,#299153,#299154,#299155,#299156,#299157,#299158,#299159,#299160,
#299161,#299162,#299163,#299164,#299165,#299166,#299167,#299168,#299169,
#299170,#299171,#299172,#299173,#299174,#299175,#299176,#299177,#299178,
#299179,#299180,#299181,#299182,#299183,#299184,#299185,#299186,#299187,
#299188,#299189,#299190,#299191,#299192,#299193,#299194,#299195,#299196,
#299197,#299198,#299199,#299200,#299201,#299202,#299203,#299204,#299205,
#299206,#299207,#299208,#299209,#299210,#299211,#299212,#299213,#299214,
#299215,#299216,#299217,#299218,#299219,#299220,#299221,#299222,#299223,
#299224,#299225,#299226,#299227,#299228,#299229,#299230,#299231,#299232,
#299233,#299234,#299235,#299236,#299237,#299238,#299239,#299240,#299241,
#299242,#299243,#299244,#299245,#299246,#299247,#299248,#299249,#299250,
#299251,#299252,#299253,#299254,#299255,#299256,#299257,#299258,#299259,
#299260,#299261,#299262,#299263,#299264,#299265,#299266,#299267,#299268,
#299269,#299270,#299271,#299272,#299273,#299274,#299275,#299276,#299277,
#299278,#299279,#299280,#299281,#299282,#299283,#299284,#299285,#299286,
#299287,#299288,#299289,#299290,#299291,#299292,#299293,#299294,#299295,
#299296,#299297,#299298,#299299,#299300,#299301,#299302,#299303,#299304,
#299305,#299306,#299307,#299308,#299309,#299310,#299311,#299312,#299313,
#299314,#299315,#299316,#299317,#299318,#299319,#299320,#299321,#299322,
#299323,#299324,#299325,#299326,#299327,#299328,#299329,#299330,#299331,
#299332,#299333,#299334,#299335,#299336,#299337,#299338,#299339,#299340,
#299341,#299342,#299343,#299344,#299345,#299346,#299347,#299348,#299349,
#299350,#299351,#299352,#299353,#299354,#299355,#299356,#299357,#299358,
#299359,#299360,#299361,#299362,#299363,#299364,#299365,#299366,#299367,
#299368,#299369,#299370,#299371,#299372,#299373,#299374,#299375,#299376,
#299377,#299378,#299379,#299380,#299381,#299382,#299383,#299384,#299385,
#299386,#299387,#299388,#299389,#299390,#299391,#299392,#299393,#299394,
#299395,#299396,#299397,#299398,#299399,#299400,#299401,#299402,#299403,
#299404,#299405,#299406,#299407,#299408,#299409,#299410,#299411,#299412,
#299413,#299414,#299415,#299416,#299417,#299418,#299419,#299420,#299421,
#299422,#299423,#299424,#299425,#299426,#299427,#299428,#299429,#299430,
#299431,#299432,#299433,#299434,#299435,#299436,#299437,#299438,#299439,
#299440,#299441,#299442,#299443,#299444,#299445,#299446,#299447,#299448,
#299449,#299450,#299451,#299452,#299453,#299454,#299455,#299456,#299457,
#299458,#299459,#299460,#299461,#299462,#299463,#299464,#299465,#299466,
#299467,#299468,#299469,#299470,#299471,#299472,#299473,#299474,#299475,
#299476,#299477,#299478,#299479,#299480,#299481,#299482,#299483,#299484,
#299485,#299486,#299487,#299488,#299489,#299490,#299491,#299492,#299493,
#299494,#299495,#299496,#299497,#299498),(#299499,#299500,#299501,#299502,
#299503,#299504,#299505,#299506,#299507,#299508,#299509,#299510,#299511,
#299512,#299513,#299514,#299515,#299516,#299517,#299518,#299519,#299520,
#299521,#299522,#299523,#299524,#299525,#299526,#299527,#299528,#299529,
#299530,#299531,#299532,#299533,#299534,#299535,#299536,#299537,#299538,
#299539,#299540,#299541,#299542,#299543,#299544,#299545,#299546,#299547,
#299548,#299549,#299550,#299551,#299552,#299553,#299554,#299555,#299556,
#299557,#299558,#299559,#299560,#299561,#299562,#299563,#299564,#299565,
#299566,#299567,#299568,#299569,#299570,#299571,#299572,#299573,#299574,
#299575,#299576,#299577,#299578,#299579,#299580,#299581,#299582,#299583,
#299584,#299585,#299586,#299587,#299588,#299589,#299590,#299591,#299592,
#299593,#299594,#299595,#299596,#299597,#299598,#299599,#299600,#299601,
#299602,#299603,#299604,#299605,#299606,#299607,#299608,#299609,#299610,
#299611,#299612,#299613,#299614,#299615,#299616,#299617,#299618,#299619,
#299620,#299621,#299622,#299623,#299624,#299625,#299626,#299627,#299628,
#299629,#299630,#299631,#299632,#299633,#299634,#299635,#299636,#299637,
#299638,#299639,#299640,#299641,#299642,#299643,#299644,#299645,#299646,
#299647,#299648,#299649,#299650,#299651,#299652,#299653,#299654,#299655,
#299656,#299657,#299658,#299659,#299660,#299661,#299662,#299663,#299664,
#299665,#299666,#299667,#299668,#299669,#299670,#299671,#299672,#299673,
#299674,#299675,#299676,#299677,#299678,#299679,#299680,#299681,#299682,
#299683,#299684,#299685,#299686,#299687,#299688,#299689,#299690,#299691,
#299692,#299693,#299694,#299695,#299696,#299697,#299698,#299699,#299700,
#299701,#299702,#299703,#299704,#299705,#299706,#299707,#299708,#299709,
#299710,#299711,#299712,#299713,#299714,#299715,#299716,#299717,#299718,
#299719,#299720,#299721,#299722,#299723,#299724,#299725,#299726,#299727,
#299728,#299729,#299730,#299731,#299732,#299733,#299734,#299735,#299736,
#299737,#299738,#299739,#299740,#299741,#299742,#299743,#299744,#299745,
#299746,#299747,#299748,#299749,#299750,#299751,#299752,#299753,#299754,
#299755,#299756,#299757,#299758,#299759,#299760,#299761,#299762,#299763,
#299764,#299765,#299766,#299767,#299768,#299769,#299770,#299771,#299772,
#299773,#299774,#299775,#299776,#299777,#299778,#299779,#299780,#299781,
#299782,#299783,#299784,#299785,#299786,#299787,#299788,#299789,#299790,
#299791,#299792,#299793,#299794,#299795,#299796,#299797,#299798,#299799,
#299800,#299801,#299802,#299803,#299804,#299805,#299806,#299807,#299808,
#299809,#299810,#299811,#299812,#299813,#299814,#299815,#299816,#299817,
#299818,#299819,#299820,#299821,#299822,#299823,#299824,#299825,#299826,
#299827,#299828,#299829,#299830,#299831,#299832,#299833,#299834,#299835,
#299836,#299837,#299838,#299839,#299840,#299841,#299842,#299843,#299844,
#299845,#299846,#299847,#299848,#299849,#299850,#299851,#299852,#299853,
#299854,#299855,#299856,#299857,#299858,#299859,#299860,#299861,#299862,
#299863,#299864,#299865,#299866,#299867,#299868,#299869,#299870,#299871,
#299872,#299873,#299874,#299875,#299876,#299877,#299878,#299879,#299880,
#299881,#299882,#299883,#299884,#299885,#299886,#299887,#299888,#299889,
#299890,#299891,#299892,#299893,#299894,#299895,#299896,#299897,#299898,
#299899,#299900,#299901,#299902,#299903,#299904,#299905,#299906,#299907,
#299908,#299909,#299910,#299911,#299912,#299913,#299914,#299915,#299916,
#299917,#299918,#299919,#299920,#299921,#299922,#299923,#299924,#299925,
#299926,#299927,#299928,#299929,#299930,#299931,#299932,#299933,#299934,
#299935,#299936,#299937,#299938,#299939,#299940,#299941,#299942,#299943,
#299944,#299945,#299946,#299947,#299948,#299949,#299950,#299951,#299952,
#299953,#299954,#299955,#299956,#299957,#299958,#299959,#299960,#299961,
#299962,#299963,#299964,#299965,#299966,#299967,#299968,#299969,#299970,
#299971,#299972,#299973,#299974,#299975,#299976,#299977,#299978,#299979,
#299980,#299981,#299982,#299983,#299984,#299985,#299986,#299987,#299988,
#299989,#299990,#299991,#299992,#299993,#299994,#299995,#299996,#299997,
#299998,#299999,#300000,#300001,#300002,#300003,#300004,#300005,#300006,
#300007,#300008,#300009,#300010,#300011,#300012,#300013,#300014,#300015,
#300016,#300017,#300018,#300019,#300020,#300021,#300022,#300023,#300024,
#300025,#300026,#300027,#300028,#300029,#300030,#300031,#300032,#300033,
#300034,#300035,#300036,#300037,#300038,#300039,#300040,#300041,#300042,
#300043,#300044,#300045,#300046,#300047,#300048,#300049,#300050,#300051,
#300052,#300053,#300054,#300055,#300056,#300057,#300058,#300059,#300060,
#300061,#300062,#300063,#300064,#300065,#300066,#300067,#300068,#300069,
#300070,#300071,#300072,#300073,#300074,#300075,#300076,#300077,#300078,
#300079,#300080,#300081,#300082,#300083,#300084,#300085,#300086,#300087,
#300088,#300089,#300090,#300091,#300092,#300093,#300094,#300095,#300096,
#300097,#300098,#300099,#300100,#300101,#300102,#300103,#300104,#300105,
#300106,#300107,#300108,#300109,#300110,#300111,#300112,#300113,#300114,
#300115,#300116,#300117,#300118,#300119,#300120,#300121,#300122,#300123,
#300124,#300125,#300126,#300127,#300128,#300129,#300130,#300131,#300132,
#300133,#300134,#300135,#300136,#300137,#300138,#300139,#300140,#300141,
#300142,#300143,#300144,#300145,#300146,#300147,#300148,#300149,#300150,
#300151,#300152,#300153,#300154,#300155,#300156,#300157,#300158,#300159,
#300160,#300161,#300162,#300163,#300164,#300165,#300166,#300167,#300168,
#300169,#300170,#300171,#300172,#300173,#300174,#300175,#300176,#300177,
#300178,#300179,#300180,#300181,#300182,#300183,#300184,#300185,#300186,
#300187,#300188,#300189,#300190,#300191,#300192,#300193,#300194,#300195,
#300196,#300197,#300198,#300199,#300200,#300201,#300202,#300203,#300204,
#300205,#300206,#300207,#300208,#300209,#300210,#300211,#300212,#300213,
#300214,#300215,#300216,#300217,#300218,#300219,#300220,#300221,#300222,
#300223,#300224,#300225,#300226,#300227,#300228,#300229,#300230,#300231,
#300232,#300233,#300234,#300235,#300236,#300237,#300238,#300239,#300240,
#300241,#300242,#300243,#300244,#300245,#300246,#300247,#300248,#300249,
#300250,#300251,#300252,#300253,#300254,#300255,#300256,#300257,#300258,
#300259,#300260,#300261,#300262,#300263,#300264,#300265,#300266,#300267,
#300268,#300269,#300270,#300271,#300272,#300273,#300274,#300275,#300276,
#300277,#300278,#300279,#300280,#300281,#300282,#300283,#300284,#300285,
#300286,#300287,#300288,#300289,#300290,#300291,#300292,#300293,#300294,
#300295,#300296,#300297,#300298,#300299,#300300,#300301,#300302,#300303,
#300304,#300305,#300306,#300307,#300308,#300309,#300310,#300311,#300312,
#300313,#300314,#300315,#300316,#300317,#300318,#300319,#300320,#300321,
#300322,#300323,#300324,#300325,#300326,#300327,#300328,#300329,#300330,
#300331,#300332,#300333,#300334,#300335,#300336,#300337,#300338,#300339,
#300340,#300341,#300342,#300343,#300344,#300345,#300346,#300347,#300348,
#300349,#300350,#300351,#300352,#300353,#300354,#300355,#300356,#300357,
#300358,#300359,#300360,#300361,#300362,#300363,#300364,#300365,#300366,
#300367,#300368,#300369,#300370,#300371,#300372,#300373,#300374,#300375,
#300376,#300377,#300378,#300379,#300380,#300381,#300382,#300383,#300384,
#300385,#300386,#300387,#300388,#300389,#300390,#300391,#300392,#300393,
#300394,#300395,#300396,#300397,#300398,#300399,#300400,#300401,#300402,
#300403,#300404,#300405,#300406,#300407,#300408,#300409,#300410,#300411,
#300412,#300413,#300414,#300415,#300416,#300417,#300418,#300419,#300420,
#300421,#300422,#300423,#300424,#300425,#300426,#300427,#300428,#300429,
#300430,#300431,#300432,#300433,#300434,#300435,#300436,#300437,#300438,
#300439,#300440,#300441,#300442,#300443,#300444,#300445,#300446,#300447,
#300448,#300449,#300450,#300451,#300452,#300453,#300454,#300455,#300456,
#300457,#300458,#300459,#300460,#300461,#300462,#300463,#300464,#300465,
#300466,#300467,#300468,#300469,#300470,#300471,#300472,#300473,#300474,
#300475,#300476,#300477,#300478,#300479,#300480,#300481,#300482,#300483,
#300484,#300485,#300486,#300487,#300488,#300489,#300490,#300491,#300492,
#300493,#300494,#300495,#300496,#300497,#300498,#300499,#300500,#300501,
#300502,#300503,#300504,#300505,#300506,#300507,#300508,#300509,#300510,
#300511,#300512,#300513,#300514,#300515,#300516,#300517,#300518,#300519,
#300520,#300521,#300522,#300523,#300524,#300525,#300526,#300527,#300528,
#300529,#300530,#300531,#300532,#300533,#300534,#300535)),.UNSPECIFIED.,
 .F.,.F.,.F.)
B_SPLINE_SURFACE_WITH_KNOTS((2,2),(3,2,2,2,2,2,2,2,2,2,2,2,2,2,2,2,2,2,
2,2,2,2,2,2,2,2,2,2,2,2,2,2,2,2,2,2,2,2,2,2,2,2,2,2,2,2,2,2,2,2,2,2,2,2,
2,2,2,2,2,2,2,2,2,2,2,2,2,2,2,2,2,2,2,2,2,2,2,2,2,2,2,2,2,2,2,2,2,2,2,2,
2,2,2,2,2,2,2,2,2,2,2,2,2,2,2,2,2,2,2,2,2,2,2,2,2,2,2,2,2,2,2,2,2,2,2,2,
2,2,2,2,2,2,2,2,2,2,2,2,2,2,2,2,2,2,2,2,2,2,2,2,2,2,2,2,2,2,2,2,2,2,2,2,
2,2,2,2,2,2,2,2,2,2,2,2,2,2,2,2,2,2,2,2,2,2,2,2,2,2,2,2,2,2,2,2,2,2,2,2,
2,2,2,2,2,2,2,2,2,2,2,2,2,2,2,2,2,2,2,2,2,2,2,2,2,2,2,2,2,2,2,2,2,2,2,2,
2,2,2,2,2,2,2,2,2,2,2,2,2,2,2,2,2,2,2,2,2,2,2,2,2,2,2,2,2,2,2,2,2,2,2,2,
2,2,2,2,2,2,2,2,2,2,2,2,2,2,2,2,2,2,2,2,2,2,2,2,2,2,2,2,2,2,2,2,2,2,2,2,
2,2,2,2,2,2,2,2,2,2,2,2,2,2,2,2,2,2,2,2,2,2,2,2,2,2,2,2,2,2,2,2,2,2,2,2,
2,2,2,2,2,2,2,2,2,2,2,2,2,2,2,2,2,2,2,2,2,2,2,2,2,2,2,2,2,2,2,2,2,2,2,2,
2,2,2,2,2,2,2,2,2,2,2,2,2,2,2,2,2,2,2,2,2,2,2,2,2,2,2,2,2,2,2,2,2,2,2,2,
2,2,2,2,2,2,2,2,2,2,2,2,2,2,2,2,2,2,2,2,2,2,2,2,2,2,2,2,2,2,2,2,2,2,2,2,
2,2,2,2,2,2,2,2,2,2,2,2,2,2,2,2,2,2,2,2,2,2,2,2,2,2,2,2,2,2,2,2,2,2,2,2,
2,2,2,2,2,2,2,2,2,2,2,2,2,2,2,2,2,2,2,2,2,2,2,2,2,2,2,2,2,2,2,2,3),(0.,
1.),(0.,0.00192307692307692,0.00384615384615385,0.00576923076923077,0.00769230769230769,
0.00961538461538462,0.0115384615384615,0.0134615384615385,0.0153846153846154,
0.0173076923076923,0.0192307692307692,0.0211538461538462,0.0230769230769231,
0.025,0.0269230769230769,0.0288461538461538,0.0307692307692308,0.0326923076923077,
0.0346153846153846,0.0365384615384615,0.0384615384615385,0.0403846153846154,
0.0423076923076923,0.0442307692307692,0.0461538461538462,0.0480769230769231,
0.05,0.0519230769230769,0.0538461538461538,0.0557692307692308,0.0576923076923077,
0.0596153846153846,0.0615384615384615,0.0634615384615385,0.0653846153846154,
0.0673076923076923,0.0692307692307692,0.0711538461538462,0.0730769230769231,
0.075,0.0769230769230769,0.0788461538461538,0.0807692307692308,0.0826923076923077,
0.0846153846153846,0.0865384615384615,0.0884615384615385,0.0903846153846154,
0.0923076923076923,0.0942307692307692,0.0961538461538462,0.0980769230769231,
0.1,0.101923076923077,0.103846153846154,0.105769230769231,0.107692307692308,
0.109615384615385,0.111538461538462,0.113461538461538,0.115384615384615,
0.117307692307692,0.119230769230769,0.121153846153846,0.123076923076923,
0.125,0.126923076923077,0.128846153846154,0.130769230769231,0.132692307692308,
0.134615384615385,0.136538461538462,0.138461538461538,0.140384615384615,
0.142307692307692,0.144230769230769,0.146153846153846,0.148076923076923,
0.15,0.151923076923077,0.153846153846154,0.155769230769231,0.157692307692308,
0.159615384615385,0.161538461538462,0.163461538461538,0.165384615384615,
0.167307692307692,0.169230769230769,0.171153846153846,0.173076923076923,
0.175,0.176923076923077,0.178846153846154,0.180769230769231,0.182692307692308,
0.184615384615385,0.186538461538462,0.188461538461538,0.190384615384615,
0.192307692307692,0.194230769230769,0.196153846153846,0.198076923076923,
0.2,0.201923076923077,0.203846153846154,0.205769230769231,0.207692307692308,
0.209615384615385,0.211538461538462,0.213461538461538,0.215384615384615,
0.217307692307692,0.219230769230769,0.221153846153846,0.223076923076923,
0.225,0.226923076923077,0.228846153846154,0.230769230769231,0.232692307692308,
0.234615384615385,0.236538461538462,0.238461538461538,0.240384615384615,
0.242307692307692,0.244230769230769,0.246153846153846,0.248076923076923,
0.25,0.251923076923077,0.253846153846154,0.255769230769231,0.257692307692308,
0.259615384615385,0.261538461538462,0.263461538461538,0.265384615384615,
0.267307692307692,0.269230769230769,0.271153846153846,0.273076923076923,
0.275,0.276923076923077,0.278846153846154,0.280769230769231,0.282692307692308,
0.284615384615385,0.286538461538462,0.288461538461538,0.290384615384615,
0.292307692307692,0.294230769230769,0.296153846153846,0.298076923076923,
0.3,0.301923076923077,0.303846153846154,0.305769230769231,0.307692307692308,
0.309615384615385,0.311538461538462,0.313461538461538,0.315384615384615,
0.317307692307692,0.319230769230769,0.321153846153846,0.323076923076923,
0.325,0.326923076923077,0.328846153846154,0.330769230769231,0.332692307692308,
0.334615384615385,0.336538461538462,0.338461538461538,0.340384615384615,
0.342307692307692,0.344230769230769,0.346153846153846,0.348076923076923,
0.35,0.351923076923077,0.353846153846154,0.355769230769231,0.357692307692308,
0.359615384615385,0.361538461538462,0.363461538461538,0.365384615384615,
0.367307692307692,0.369230769230769,0.371153846153846,0.373076923076923,
0.375,0.376923076923077,0.378846153846154,0.380769230769231,0.382692307692308,
0.384615384615385,0.386538461538462,0.388461538461538,0.390384615384615,
0.392307692307692,0.394230769230769,0.396153846153846,0.398076923076923,
0.4,0.401923076923077,0.403846153846154,0.405769230769231,0.407692307692308,
0.409615384615385,0.411538461538462,0.413461538461538,0.415384615384615,
0.417307692307692,0.419230769230769,0.421153846153846,0.423076923076923,
0.425,0.426923076923077,0.428846153846154,0.430769230769231,0.432692307692308,
0.434615384615385,0.436538461538462,0.438461538461538,0.440384615384615,
0.442307692307692,0.444230769230769,0.446153846153846,0.448076923076923,
0.45,0.451923076923077,0.453846153846154,0.455769230769231,0.457692307692308,
0.459615384615385,0.461538461538462,0.463461538461538,0.465384615384615,
0.467307692307692,0.469230769230769,0.471153846153846,0.473076923076923,
0.475,0.476923076923077,0.478846153846154,0.480769230769231,0.482692307692308,
0.484615384615385,0.486538461538462,0.488461538461538,0.490384615384615,
0.492307692307692,0.494230769230769,0.496153846153846,0.498076923076923,
0.5,0.501923076923077,0.503846153846154,0.505769230769231,0.507692307692308,
0.509615384615385,0.511538461538461,0.513461538461538,0.515384615384615,
0.517307692307692,0.519230769230769,0.521153846153846,0.523076923076923,
0.525,0.526923076923077,0.528846153846154,0.530769230769231,0.532692307692308,
0.534615384615385,0.536538461538462,0.538461538461538,0.540384615384615,
0.542307692307692,0.544230769230769,0.546153846153846,0.548076923076923,
0.55,0.551923076923077,0.553846153846154,0.555769230769231,0.557692307692308,
0.559615384615385,0.561538461538462,0.563461538461538,0.565384615384615,
0.567307692307692,0.569230769230769,0.571153846153846,0.573076923076923,
0.575,0.576923076923077,0.578846153846154,0.580769230769231,0.582692307692308,
0.584615384615385,0.586538461538462,0.588461538461538,0.590384615384615,
0.592307692307692,0.594230769230769,0.596153846153846,0.598076923076923,
0.6,0.601923076923077,0.603846153846154,0.605769230769231,0.607692307692308,
0.609615384615385,0.611538461538462,0.613461538461539,0.615384615384615,
0.617307692307692,0.619230769230769,0.621153846153846,0.623076923076923,
0.625,0.626923076923077,0.628846153846154,0.630769230769231,0.632692307692308,
0.634615384615385,0.636538461538461,0.638461538461538,0.640384615384615,
0.642307692307692,0.644230769230769,0.646153846153846,0.648076923076923,
0.65,0.651923076923077,0.653846153846154,0.655769230769231,0.657692307692308,
0.659615384615385,0.661538461538462,0.663461538461538,0.665384615384615,
0.667307692307692,0.669230769230769,0.671153846153846,0.673076923076923,
0.675,0.676923076923077,0.678846153846154,0.680769230769231,0.682692307692308,
0.684615384615385,0.686538461538462,0.688461538461538,0.690384615384615,
0.692307692307692,0.694230769230769,0.696153846153846,0.698076923076923,
0.7,0.701923076923077,0.703846153846154,0.705769230769231,0.707692307692308,
0.709615384615385,0.711538461538462,0.713461538461538,0.715384615384615,
0.717307692307692,0.719230769230769,0.721153846153846,0.723076923076923,
0.725,0.726923076923077,0.728846153846154,0.730769230769231,0.732692307692308,
0.734615384615385,0.736538461538462,0.738461538461539,0.740384615384615,
0.742307692307692,0.744230769230769,0.746153846153846,0.748076923076923,
0.75,0.751923076923077,0.753846153846154,0.755769230769231,0.757692307692308,
0.759615384615385,0.761538461538461,0.763461538461538,0.765384615384615,
0.767307692307692,0.769230769230769,0.771153846153846,0.773076923076923,
0.775,0.776923076923077,0.778846153846154,0.780769230769231,0.782692307692308,
0.784615384615385,0.786538461538462,0.788461538461538,0.790384615384615,
0.792307692307692,0.794230769230769,0.796153846153846,0.798076923076923,
0.8,0.801923076923077,0.803846153846154,0.805769230769231,0.807692307692308,
0.809615384615385,0.811538461538462,0.813461538461538,0.815384615384615,
0.817307692307692,0.819230769230769,0.821153846153846,0.823076923076923,
0.825,0.826923076923077,0.828846153846154,0.830769230769231,0.832692307692308,
0.834615384615385,0.836538461538462,0.838461538461538,0.840384615384615,
0.842307692307692,0.844230769230769,0.846153846153846,0.848076923076923,
0.85,0.851923076923077,0.853846153846154,0.855769230769231,0.857692307692308,
0.859615384615385,0.861538461538462,0.863461538461539,0.865384615384615,
0.867307692307692,0.869230769230769,0.871153846153846,0.873076923076923,
0.875,0.876923076923077,0.878846153846154,0.880769230769231,0.882692307692308,
0.884615384615385,0.886538461538461,0.888461538461538,0.890384615384615,
0.892307692307692,0.894230769230769,0.896153846153846,0.898076923076923,
0.9,0.901923076923077,0.903846153846154,0.905769230769231,0.907692307692308,
0.909615384615385,0.911538461538462,0.913461538461538,0.915384615384615,
0.917307692307692,0.919230769230769,0.921153846153846,0.923076923076923,
0.925,0.926923076923077,0.928846153846154,0.930769230769231,0.932692307692308,
0.934615384615385,0.936538461538462,0.938461538461538,0.940384615384615,
0.942307692307692,0.944230769230769,0.946153846153846,0.948076923076923,
0.95,0.951923076923077,0.953846153846154,0.955769230769231,0.957692307692308,
0.959615384615385,0.961538461538462,0.963461538461538,0.965384615384615,
0.967307692307692,0.969230769230769,0.971153846153846,0.973076923076923,
0.975,0.976923076923077,0.978846153846154,0.980769230769231,0.982692307692308,
0.984615384615385,0.986538461538462,0.988461538461539,0.990384615384615,
0.992307692307692,0.994230769230769,0.996153846153846),.UNSPECIFIED.)
GEOMETRIC_REPRESENTATION_ITEM()
RATIONAL_B_SPLINE_SURFACE(((1.,0.951056516295154,1.,0.951056516295154,1.,
0.951056516295154,1.,0.951056516295154,1.,0.951056516295154,1.,0.951056516295154,
1.,0.951056516295154,1.,0.951056516295154,1.,0.951056516295154,1.,0.951056516295154,
1.,0.951056516295154,1.,0.951056516295154,1.,0.951056516295154,1.,0.951056516295154,
1.,0.951056516295154,1.,0.951056516295154,1.,0.951056516295154,1.,0.951056516295154,
1.,0.951056516295154,1.,0.951056516295154,1.,0.951056516295154,1.,0.951056516295154,
1.,0.951056516295154,1.,0.951056516295154,1.,0.951056516295154,1.,0.951056516295154,
1.,0.951056516295154,1.,0.951056516295154,1.,0.951056516295154,1.,0.951056516295154,
1.,0.951056516295154,1.,0.951056516295154,1.,0.951056516295154,1.,0.951056516295154,
1.,0.951056516295154,1.,0.951056516295154,1.,0.951056516295154,1.,0.951056516295154,
1.,0.951056516295154,1.,0.951056516295154,1.,0.951056516295154,1.,0.951056516295154,
1.,0.951056516295154,1.,0.951056516295154,1.,0.951056516295154,1.,0.951056516295154,
1.,0.951056516295154,1.,0.951056516295154,1.,0.951056516295154,1.,0.951056516295154,
1.,0.951056516295154,1.,0.951056516295154,1.,0.951056516295154,1.,0.951056516295154,
1.,0.951056516295154,1.,0.951056516295154,1.,0.951056516295154,1.,0.951056516295154,
1.,0.951056516295154,1.,0.951056516295154,1.,0.951056516295154,1.,0.951056516295154,
1.,0.951056516295154,1.,0.951056516295154,1.,0.951056516295154,1.,0.951056516295154,
1.,0.951056516295154,1.,0.951056516295154,1.,0.951056516295154,1.,0.951056516295154,
1.,0.951056516295154,1.,0.951056516295154,1.,0.951056516295154,1.,0.951056516295154,
1.,0.951056516295154,1.,0.951056516295154,1.,0.951056516295154,1.,0.951056516295154,
1.,0.951056516295154,1.,0.951056516295154,1.,0.951056516295154,1.,0.951056516295154,
1.,0.951056516295154,1.,0.951056516295154,1.,0.951056516295154,1.,0.951056516295154,
1.,0.951056516295154,1.,0.951056516295154,1.,0.951056516295154,1.,0.951056516295154,
1.,0.951056516295154,1.,0.951056516295154,1.,0.951056516295154,1.,0.951056516295154,
1.,0.951056516295154,1.,0.951056516295154,1.,0.951056516295154,1.,0.951056516295154,
1.,0.951056516295154,1.,0.951056516295154,1.,0.951056516295154,1.,0.951056516295154,
1.,0.951056516295154,1.,0.951056516295154,1.,0.951056516295154,1.,0.951056516295154,
1.,0.951056516295154,1.,0.951056516295154,1.,0.951056516295154,1.,0.951056516295154,
1.,0.951056516295154,1.,0.951056516295154,1.,0.951056516295154,1.,0.951056516295154,
1.,0.951056516295154,1.,0.951056516295154,1.,0.951056516295154,1.,0.951056516295154,
1.,0.951056516295154,1.,0.951056516295154,1.,0.951056516295154,1.,0.951056516295154,
1.,0.951056516295154,1.,0.951056516295154,1.,0.951056516295154,1.,0.951056516295154,
1.,0.951056516295154,1.,0.951056516295154,1.,0.951056516295154,1.,0.951056516295154,
1.,0.951056516295154,1.,0.951056516295154,1.,0.951056516295154,1.,0.951056516295154,
1.,0.951056516295154,1.,0.951056516295154,1.,0.951056516295154,1.,0.951056516295154,
1.,0.951056516295154,1.,0.951056516295154,1.,0.951056516295154,1.,0.951056516295154,
1.,0.951056516295154,1.,0.951056516295154,1.,0.951056516295154,1.,0.951056516295154,
1.,0.951056516295154,1.,0.951056516295154,1.,0.951056516295154,1.,0.951056516295154,
1.,0.951056516295154,1.,0.951056516295154,1.,0.951056516295154,1.,0.951056516295154,
1.,0.951056516295154,1.,0.951056516295154,1.,0.951056516295154,1.,0.951056516295154,
1.,0.951056516295154,1.,0.951056516295154,1.,0.951056516295154,1.,0.951056516295154,
1.,0.951056516295154,1.,0.951056516295154,1.,0.951056516295154,1.,0.951056516295154,
1.,0.951056516295154,1.,0.951056516295154,1.,0.951056516295154,1.,0.951056516295154,
1.,0.951056516295154,1.,0.951056516295154,1.,0.951056516295154,1.,0.951056516295154,
1.,0.951056516295154,1.,0.951056516295154,1.,0.951056516295154,1.,0.951056516295154,
1.,0.951056516295154,1.,0.951056516295154,1.,0.951056516295154,1.,0.951056516295154,
1.,0.951056516295154,1.,0.951056516295154,1.,0.951056516295154,1.,0.951056516295154,
1.,0.951056516295154,1.,0.951056516295154,1.,0.951056516295154,1.,0.951056516295154,
1.,0.951056516295154,1.,0.951056516295154,1.,0.951056516295154,1.,0.951056516295154,
1.,0.951056516295154,1.,0.951056516295154,1.,0.951056516295154,1.,0.951056516295154,
1.,0.951056516295154,1.,0.951056516295154,1.,0.951056516295154,1.,0.951056516295154,
1.,0.951056516295154,1.,0.951056516295154,1.,0.951056516295154,1.,0.951056516295154,
1.,0.951056516295154,1.,0.951056516295154,1.,0.951056516295154,1.,0.951056516295154,
1.,0.951056516295154,1.,0.951056516295154,1.,0.951056516295154,1.,0.951056516295154,
1.,0.951056516295154,1.,0.951056516295154,1.,0.951056516295154,1.,0.951056516295154,
1.,0.951056516295154,1.,0.951056516295154,1.,0.951056516295154,1.,0.951056516295154,
1.,0.951056516295154,1.,0.951056516295154,1.,0.951056516295154,1.,0.951056516295154,
1.,0.951056516295154,1.,0.951056516295154,1.,0.951056516295154,1.,0.951056516295154,
1.,0.951056516295154,1.,0.951056516295154,1.,0.951056516295154,1.,0.951056516295154,
1.,0.951056516295154,1.,0.951056516295154,1.,0.951056516295154,1.,0.951056516295154,
1.,0.951056516295154,1.,0.951056516295154,1.,0.951056516295154,1.,0.951056516295154,
1.,0.951056516295154,1.,0.951056516295154,1.,0.951056516295154,1.,0.951056516295154,
1.,0.951056516295154,1.,0.951056516295154,1.,0.951056516295154,1.,0.951056516295154,
1.,0.951056516295154,1.,0.951056516295154,1.,0.951056516295154,1.,0.951056516295154,
1.,0.951056516295154,1.,0.951056516295154,1.,0.951056516295154,1.,0.951056516295154,
1.,0.951056516295154,1.,0.951056516295154,1.,0.951056516295154,1.,0.951056516295154,
1.,0.951056516295154,1.,0.951056516295154,1.,0.951056516295154,1.,0.951056516295154,
1.,0.951056516295154,1.,0.951056516295154,1.,0.951056516295154,1.,0.951056516295154,
1.,0.951056516295154,1.,0.951056516295154,1.,0.951056516295154,1.,0.951056516295154,
1.,0.951056516295154,1.,0.951056516295154,1.,0.951056516295154,1.,0.951056516295154,
1.,0.951056516295154,1.,0.951056516295154,1.,0.951056516295154,1.,0.951056516295154,
1.,0.951056516295154,1.,0.951056516295154,1.,0.951056516295154,1.,0.951056516295154,
1.,0.951056516295154,1.,0.951056516295154,1.,0.951056516295154,1.,0.951056516295154,
1.,0.951056516295154,1.,0.951056516295154,1.,0.951056516295154,1.,0.951056516295154,
1.,0.951056516295154,1.,0.951056516295154,1.,0.951056516295154,1.,0.951056516295154,
1.,0.951056516295154,1.,0.951056516295154,1.,0.951056516295154,1.,0.951056516295154,
1.,0.951056516295154,1.,0.951056516295154,1.,0.951056516295154,1.,0.951056516295154,
1.,0.951056516295154,1.,0.951056516295154,1.,0.951056516295154,1.,0.951056516295154,
1.,0.951056516295154,1.,0.951056516295154,1.,0.951056516295154,1.,0.951056516295154,
1.,0.951056516295154,1.,0.951056516295154,1.,0.951056516295154,1.,0.951056516295154,
1.,0.951056516295154,1.,0.951056516295154,1.,0.951056516295154,1.,0.951056516295154,
1.,0.951056516295154,1.,0.951056516295154,1.,0.951056516295154,1.,0.951056516295154,
1.,0.951056516295154,1.,0.951056516295154,1.,0.951056516295154,1.,0.951056516295154,
1.,0.951056516295154,1.,0.951056516295154,1.,0.951056516295154,1.,0.951056516295154,
1.,0.951056516295154,1.,0.951056516295154,1.,0.951056516295154,1.,0.951056516295154,
1.,0.951056516295154,1.,0.951056516295154,1.,0.951056516295154,1.,0.951056516295154,
1.,0.951056516295154,1.,0.951056516295154,1.,0.951056516295154,1.,0.951056516295154,
1.,0.951056516295154,1.,0.951056516295154,1.,0.951056516295154,1.,0.951056516295154,
1.,0.951056516295154,1.,0.951056516295154,1.,0.951056516295154,1.,0.951056516295154,
1.,0.951056516295154,1.,0.951056516295154,1.,0.951056516295154,1.,0.951056516295154,
1.,0.951056516295154,1.,0.951056516295154,1.,0.951056516295154,1.,0.951056516295154,
1.,0.951056516295154,1.,0.951056516295154,1.,0.951056516295154,1.,0.951056516295154,
1.,0.951056516295154,1.,0.951056516295154,1.,0.951056516295154,1.,0.951056516295154,
1.,0.951056516295154,1.,0.951056516295154,1.,0.951056516295154,1.,0.951056516295154,
1.,0.951056516295154,1.,0.951056516295154,1.,0.951056516295154,1.,0.951056516295154,
1.,0.951056516295154,1.,0.951056516295154,1.,0.951056516295154,1.,0.951056516295154,
1.,0.951056516295154,1.,0.951056516295154,1.,0.951056516295154,1.,0.951056516295154,
1.,0.951056516295154,1.,0.951056516295154,1.,0.951056516295154,1.,0.951056516295154,
1.,0.951056516295154,1.,0.951056516295154,1.,0.951056516295154,1.,0.951056516295154,
1.,0.951056516295154,1.,0.951056516295154,1.,0.951056516295154,1.,0.951056516295154,
1.,0.951056516295154,1.,0.951056516295154,1.,0.951056516295154,1.,0.951056516295154,
1.,0.951056516295154,1.,0.951056516295154,1.,0.951056516295154,1.,0.951056516295154,
1.,0.951056516295154,1.,0.951056516295154,1.,0.951056516295154,1.,0.951056516295154,
1.,0.951056516295154,1.,0.951056516295154,1.,0.951056516295154,1.,0.951056516295154,
1.,0.951056516295154,1.,0.951056516295154,1.,0.951056516295154,1.,0.951056516295154,
1.,0.951056516295154,1.,0.951056516295154,1.,0.951056516295154,1.,0.951056516295154,
1.,0.951056516295154,1.,0.951056516295154,1.,0.951056516295154,1.,0.951056516295154,
1.,0.951056516295154,1.,0.951056516295154,1.,0.951056516295154,1.,0.951056516295154,
1.,0.951056516295154,1.,0.951056516295154,1.,0.951056516295154,1.,0.951056516295154,
1.,0.951056516295154,1.,0.951056516295154,1.,0.951056516295154,1.,0.951056516295154,
1.,0.951056516295154,1.,0.951056516295154,1.,0.951056516295154,1.,0.951056516295154,
1.,0.951056516295154,1.,0.951056516295154,1.,0.951056516295154,1.,0.951056516295154,
1.,0.951056516295154,1.,0.951056516295154,1.,0.951056516295154,1.,0.951056516295154,
1.,0.951056516295154,1.,0.951056516295154,1.,0.951056516295154,1.,0.951056516295154,
1.,0.951056516295154,1.,0.951056516295154,1.,0.951056516295154,1.,0.951056516295154,
1.,0.951056516295154,1.,0.951056516295154,1.,0.951056516295154,1.,0.951056516295154,
1.,0.951056516295154,1.,0.951056516295154,1.,0.951056516295154,1.,0.951056516295154,
1.,0.951056516295154,1.,0.951056516295154,1.,0.951056516295154,1.,0.951056516295154,
1.,0.951056516295154,1.,0.951056516295154,1.,0.951056516295154,1.,0.951056516295154,
1.,0.951056516295154,1.,0.951056516295154,1.,0.951056516295154,1.,0.951056516295154,
1.,0.951056516295154,1.,0.951056516295154,1.,0.951056516295154,1.,0.951056516295154,
1.,0.951056516295154,1.,0.951056516295154,1.,0.951056516295154,1.,0.951056516295154,
1.,0.951056516295154,1.,0.951056516295154,1.,0.951056516295154,1.,0.951056516295154,
1.,0.951056516295154,1.,0.951056516295154,1.,0.951056516295154,1.,0.951056516295154,
1.,0.951056516295154,1.,0.951056516295154,1.,0.951056516295154,1.,0.951056516295154,
1.,0.951056516295154,1.,0.951056516295154,1.,0.951056516295154,1.,0.951056516295154,
1.,0.951056516295154,1.,0.951056516295154,1.,0.951056516295154,1.,0.951056516295154,
1.,0.951056516295154,1.,0.951056516295154,1.,0.951056516295154,1.,0.951056516295154,
1.,0.951056516295154,1.,0.951056516295154,1.,0.951056516295154,1.,0.951056516295154,
1.,0.951056516295154,1.,0.951056516295154,1.,0.951056516295154,1.,0.951056516295154,
1.),(1.,0.951056516295154,1.,0.951056516295154,1.,0.951056516295154,1.,
0.951056516295154,1.,0.951056516295154,1.,0.951056516295154,1.,0.951056516295154,
1.,0.951056516295154,1.,0.951056516295154,1.,0.951056516295154,1.,0.951056516295154,
1.,0.951056516295154,1.,0.951056516295154,1.,0.951056516295154,1.,0.951056516295154,
1.,0.951056516295154,1.,0.951056516295154,1.,0.951056516295154,1.,0.951056516295154,
1.,0.951056516295154,1.,0.951056516295154,1.,0.951056516295154,1.,0.951056516295154,
1.,0.951056516295154,1.,0.951056516295154,1.,0.951056516295154,1.,0.951056516295154,
1.,0.951056516295154,1.,0.951056516295154,1.,0.951056516295154,1.,0.951056516295154,
1.,0.951056516295154,1.,0.951056516295154,1.,0.951056516295154,1.,0.951056516295154,
1.,0.951056516295154,1.,0.951056516295154,1.,0.951056516295154,1.,0.951056516295154,
1.,0.951056516295154,1.,0.951056516295154,1.,0.951056516295154,1.,0.951056516295154,
1.,0.951056516295154,1.,0.951056516295154,1.,0.951056516295154,1.,0.951056516295154,
1.,0.951056516295154,1.,0.951056516295154,1.,0.951056516295154,1.,0.951056516295154,
1.,0.951056516295154,1.,0.951056516295154,1.,0.951056516295154,1.,0.951056516295154,
1.,0.951056516295154,1.,0.951056516295154,1.,0.951056516295154,1.,0.951056516295154,
1.,0.951056516295154,1.,0.951056516295154,1.,0.951056516295154,1.,0.951056516295154,
1.,0.951056516295154,1.,0.951056516295154,1.,0.951056516295154,1.,0.951056516295154,
1.,0.951056516295154,1.,0.951056516295154,1.,0.951056516295154,1.,0.951056516295154,
1.,0.951056516295154,1.,0.951056516295154,1.,0.951056516295154,1.,0.951056516295154,
1.,0.951056516295154,1.,0.951056516295154,1.,0.951056516295154,1.,0.951056516295154,
1.,0.951056516295154,1.,0.951056516295154,1.,0.951056516295154,1.,0.951056516295154,
1.,0.951056516295154,1.,0.951056516295154,1.,0.951056516295154,1.,0.951056516295154,
1.,0.951056516295154,1.,0.951056516295154,1.,0.951056516295154,1.,0.951056516295154,
1.,0.951056516295154,1.,0.951056516295154,1.,0.951056516295154,1.,0.951056516295154,
1.,0.951056516295154,1.,0.951056516295154,1.,0.951056516295154,1.,0.951056516295154,
1.,0.951056516295154,1.,0.951056516295154,1.,0.951056516295154,1.,0.951056516295154,
1.,0.951056516295154,1.,0.951056516295154,1.,0.951056516295154,1.,0.951056516295154,
1.,0.951056516295154,1.,0.951056516295154,1.,0.951056516295154,1.,0.951056516295154,
1.,0.951056516295154,1.,0.951056516295154,1.,0.951056516295154,1.,0.951056516295154,
1.,0.951056516295154,1.,0.951056516295154,1.,0.951056516295154,1.,0.951056516295154,
1.,0.951056516295154,1.,0.951056516295154,1.,0.951056516295154,1.,0.951056516295154,
1.,0.951056516295154,1.,0.951056516295154,1.,0.951056516295154,1.,0.951056516295154,
1.,0.951056516295154,1.,0.951056516295154,1.,0.951056516295154,1.,0.951056516295154,
1.,0.951056516295154,1.,0.951056516295154,1.,0.951056516295154,1.,0.951056516295154,
1.,0.951056516295154,1.,0.951056516295154,1.,0.951056516295154,1.,0.951056516295154,
1.,0.951056516295154,1.,0.951056516295154,1.,0.951056516295154,1.,0.951056516295154,
1.,0.951056516295154,1.,0.951056516295154,1.,0.951056516295154,1.,0.951056516295154,
1.,0.951056516295154,1.,0.951056516295154,1.,0.951056516295154,1.,0.951056516295154,
1.,0.951056516295154,1.,0.951056516295154,1.,0.951056516295154,1.,0.951056516295154,
1.,0.951056516295154,1.,0.951056516295154,1.,0.951056516295154,1.,0.951056516295154,
1.,0.951056516295154,1.,0.951056516295154,1.,0.951056516295154,1.,0.951056516295154,
1.,0.951056516295154,1.,0.951056516295154,1.,0.951056516295154,1.,0.951056516295154,
1.,0.951056516295154,1.,0.951056516295154,1.,0.951056516295154,1.,0.951056516295154,
1.,0.951056516295154,1.,0.951056516295154,1.,0.951056516295154,1.,0.951056516295154,
1.,0.951056516295154,1.,0.951056516295154,1.,0.951056516295154,1.,0.951056516295154,
1.,0.951056516295154,1.,0.951056516295154,1.,0.951056516295154,1.,0.951056516295154,
1.,0.951056516295154,1.,0.951056516295154,1.,0.951056516295154,1.,0.951056516295154,
1.,0.951056516295154,1.,0.951056516295154,1.,0.951056516295154,1.,0.951056516295154,
1.,0.951056516295154,1.,0.951056516295154,1.,0.951056516295154,1.,0.951056516295154,
1.,0.951056516295154,1.,0.951056516295154,1.,0.951056516295154,1.,0.951056516295154,
1.,0.951056516295154,1.,0.951056516295154,1.,0.951056516295154,1.,0.951056516295154,
1.,0.951056516295154,1.,0.951056516295154,1.,0.951056516295154,1.,0.951056516295154,
1.,0.951056516295154,1.,0.951056516295154,1.,0.951056516295154,1.,0.951056516295154,
1.,0.951056516295154,1.,0.951056516295154,1.,0.951056516295154,1.,0.951056516295154,
1.,0.951056516295154,1.,0.951056516295154,1.,0.951056516295154,1.,0.951056516295154,
1.,0.951056516295154,1.,0.951056516295154,1.,0.951056516295154,1.,0.951056516295154,
1.,0.951056516295154,1.,0.951056516295154,1.,0.951056516295154,1.,0.951056516295154,
1.,0.951056516295154,1.,0.951056516295154,1.,0.951056516295154,1.,0.951056516295154,
1.,0.951056516295154,1.,0.951056516295154,1.,0.951056516295154,1.,0.951056516295154,
1.,0.951056516295154,1.,0.951056516295154,1.,0.951056516295154,1.,0.951056516295154,
1.,0.951056516295154,1.,0.951056516295154,1.,0.951056516295154,1.,0.951056516295154,
1.,0.951056516295154,1.,0.951056516295154,1.,0.951056516295154,1.,0.951056516295154,
1.,0.951056516295154,1.,0.951056516295154,1.,0.951056516295154,1.,0.951056516295154,
1.,0.951056516295154,1.,0.951056516295154,1.,0.951056516295154,1.,0.951056516295154,
1.,0.951056516295154,1.,0.951056516295154,1.,0.951056516295154,1.,0.951056516295154,
1.,0.951056516295154,1.,0.951056516295154,1.,0.951056516295154,1.,0.951056516295154,
1.,0.951056516295154,1.,0.951056516295154,1.,0.951056516295154,1.,0.951056516295154,
1.,0.951056516295154,1.,0.951056516295154,1.,0.951056516295154,1.,0.951056516295154,
1.,0.951056516295154,1.,0.951056516295154,1.,0.951056516295154,1.,0.951056516295154,
1.,0.951056516295154,1.,0.951056516295154,1.,0.951056516295154,1.,0.951056516295154,
1.,0.951056516295154,1.,0.951056516295154,1.,0.951056516295154,1.,0.951056516295154,
1.,0.951056516295154,1.,0.951056516295154,1.,0.951056516295154,1.,0.951056516295154,
1.,0.951056516295154,1.,0.951056516295154,1.,0.951056516295154,1.,0.951056516295154,
1.,0.951056516295154,1.,0.951056516295154,1.,0.951056516295154,1.,0.951056516295154,
1.,0.951056516295154,1.,0.951056516295154,1.,0.951056516295154,1.,0.951056516295154,
1.,0.951056516295154,1.,0.951056516295154,1.,0.951056516295154,1.,0.951056516295154,
1.,0.951056516295154,1.,0.951056516295154,1.,0.951056516295154,1.,0.951056516295154,
1.,0.951056516295154,1.,0.951056516295154,1.,0.951056516295154,1.,0.951056516295154,
1.,0.951056516295154,1.,0.951056516295154,1.,0.951056516295154,1.,0.951056516295154,
1.,0.951056516295154,1.,0.951056516295154,1.,0.951056516295154,1.,0.951056516295154,
1.,0.951056516295154,1.,0.951056516295154,1.,0.951056516295154,1.,0.951056516295154,
1.,0.951056516295154,1.,0.951056516295154,1.,0.951056516295154,1.,0.951056516295154,
1.,0.951056516295154,1.,0.951056516295154,1.,0.951056516295154,1.,0.951056516295154,
1.,0.951056516295154,1.,0.951056516295154,1.,0.951056516295154,1.,0.951056516295154,
1.,0.951056516295154,1.,0.951056516295154,1.,0.951056516295154,1.,0.951056516295154,
1.,0.951056516295154,1.,0.951056516295154,1.,0.951056516295154,1.,0.951056516295154,
1.,0.951056516295154,1.,0.951056516295154,1.,0.951056516295154,1.,0.951056516295154,
1.,0.951056516295154,1.,0.951056516295154,1.,0.951056516295154,1.,0.951056516295154,
1.,0.951056516295154,1.,0.951056516295154,1.,0.951056516295154,1.,0.951056516295154,
1.,0.951056516295154,1.,0.951056516295154,1.,0.951056516295154,1.,0.951056516295154,
1.,0.951056516295154,1.,0.951056516295154,1.,0.951056516295154,1.,0.951056516295154,
1.,0.951056516295154,1.,0.951056516295154,1.,0.951056516295154,1.,0.951056516295154,
1.,0.951056516295154,1.,0.951056516295154,1.,0.951056516295154,1.,0.951056516295154,
1.,0.951056516295154,1.,0.951056516295154,1.,0.951056516295154,1.,0.951056516295154,
1.,0.951056516295154,1.,0.951056516295154,1.,0.951056516295154,1.,0.951056516295154,
1.,0.951056516295154,1.,0.951056516295154,1.,0.951056516295154,1.,0.951056516295154,
1.,0.951056516295154,1.,0.951056516295154,1.,0.951056516295154,1.,0.951056516295154,
1.,0.951056516295154,1.,0.951056516295154,1.,0.951056516295154,1.,0.951056516295154,
1.,0.951056516295154,1.,0.951056516295154,1.,0.951056516295154,1.,0.951056516295154,
1.,0.951056516295154,1.,0.951056516295154,1.,0.951056516295154,1.,0.951056516295154,
1.,0.951056516295154,1.,0.951056516295154,1.,0.951056516295154,1.,0.951056516295154,
1.,0.951056516295154,1.,0.951056516295154,1.,0.951056516295154,1.,0.951056516295154,
1.,0.951056516295154,1.,0.951056516295154,1.,0.951056516295154,1.,0.951056516295154,
1.,0.951056516295154,1.,0.951056516295154,1.,0.951056516295154,1.,0.951056516295154,
1.,0.951056516295154,1.,0.951056516295154,1.,0.951056516295154,1.,0.951056516295154,
1.,0.951056516295154,1.,0.951056516295154,1.,0.951056516295154,1.,0.951056516295154,
1.,0.951056516295154,1.,0.951056516295154,1.,0.951056516295154,1.,0.951056516295154,
1.,0.951056516295154,1.,0.951056516295154,1.,0.951056516295154,1.,0.951056516295154,
1.,0.951056516295154,1.,0.951056516295154,1.,0.951056516295154,1.,0.951056516295154,
1.,0.951056516295154,1.,0.951056516295154,1.,0.951056516295154,1.,0.951056516295154,
1.,0.951056516295154,1.,0.951056516295154,1.,0.951056516295154,1.,0.951056516295154,
1.,0.951056516295154,1.,0.951056516295154,1.,0.951056516295154,1.,0.951056516295154,
1.,0.951056516295154,1.,0.951056516295154,1.,0.951056516295154,1.,0.951056516295154,
1.,0.951056516295154,1.,0.951056516295154,1.,0.951056516295154,1.,0.951056516295154,
1.,0.951056516295154,1.,0.951056516295154,1.,0.951056516295154,1.,0.951056516295154,
1.,0.951056516295154,1.,0.951056516295154,1.,0.951056516295154,1.,0.951056516295154,
1.,0.951056516295154,1.,0.951056516295154,1.,0.951056516295154,1.,0.951056516295154,
1.,0.951056516295154,1.,0.951056516295154,1.,0.951056516295154,1.,0.951056516295154,
1.,0.951056516295154,1.,0.951056516295154,1.,0.951056516295154,1.,0.951056516295154,
1.,0.951056516295154,1.,0.951056516295154,1.,0.951056516295154,1.,0.951056516295154,
1.,0.951056516295154,1.,0.951056516295154,1.,0.951056516295154,1.,0.951056516295154,
1.,0.951056516295154,1.,0.951056516295154,1.,0.951056516295154,1.,0.951056516295154,
1.,0.951056516295154,1.,0.951056516295154,1.,0.951056516295154,1.,0.951056516295154,
1.,0.951056516295154,1.,0.951056516295154,1.,0.951056516295154,1.,0.951056516295154,
1.,0.951056516295154,1.,0.951056516295154,1.,0.951056516295154,1.,0.951056516295154,
1.,0.951056516295154,1.,0.951056516295154,1.,0.951056516295154,1.,0.951056516295154,
1.,0.951056516295154,1.,0.951056516295154,1.,0.951056516295154,1.,0.951056516295154,
1.,0.951056516295154,1.,0.951056516295154,1.,0.951056516295154,1.,0.951056516295154,
1.,0.951056516295154,1.,0.951056516295154,1.,0.951056516295154,1.,0.951056516295154,
1.,0.951056516295154,1.,0.951056516295154,1.,0.951056516295154,1.)))
REPRESENTATION_ITEM('')
SURFACE()
);
#3201=(
BOUNDED_SURFACE()
B_SPLINE_SURFACE(1,2,((#300541,#300542,#300543,#300544,#300545,#300546,
#300547,#300548,#300549,#300550,#300551,#300552,#300553,#300554,#300555,
#300556,#300557,#300558,#300559,#300560,#300561,#300562,#300563,#300564,
#300565,#300566,#300567,#300568,#300569,#300570,#300571,#300572,#300573,
#300574,#300575,#300576,#300577,#300578,#300579,#300580,#300581,#300582,
#300583,#300584,#300585,#300586,#300587,#300588,#300589,#300590,#300591,
#300592,#300593,#300594,#300595,#300596,#300597,#300598,#300599,#300600,
#300601,#300602,#300603,#300604,#300605,#300606,#300607,#300608,#300609,
#300610,#300611,#300612,#300613,#300614,#300615,#300616,#300617,#300618,
#300619,#300620,#300621,#300622,#300623,#300624,#300625,#300626,#300627,
#300628,#300629,#300630,#300631,#300632,#300633,#300634,#300635,#300636,
#300637,#300638,#300639,#300640,#300641,#300642,#300643,#300644,#300645,
#300646,#300647,#300648,#300649,#300650,#300651,#300652,#300653,#300654,
#300655,#300656,#300657,#300658,#300659,#300660,#300661,#300662,#300663,
#300664,#300665,#300666,#300667,#300668,#300669,#300670,#300671,#300672,
#300673,#300674,#300675,#300676,#300677,#300678,#300679,#300680,#300681,
#300682,#300683,#300684,#300685,#300686,#300687,#300688,#300689,#300690,
#300691,#300692,#300693,#300694,#300695,#300696,#300697,#300698,#300699,
#300700,#300701,#300702,#300703,#300704,#300705,#300706,#300707,#300708,
#300709,#300710,#300711,#300712,#300713,#300714,#300715,#300716,#300717,
#300718,#300719,#300720,#300721,#300722,#300723,#300724,#300725,#300726,
#300727,#300728,#300729,#300730,#300731,#300732,#300733,#300734,#300735,
#300736,#300737,#300738,#300739,#300740,#300741,#300742,#300743,#300744,
#300745,#300746,#300747,#300748,#300749,#300750,#300751,#300752,#300753,
#300754,#300755,#300756,#300757,#300758,#300759,#300760,#300761,#300762,
#300763,#300764,#300765,#300766,#300767,#300768,#300769,#300770,#300771,
#300772,#300773,#300774,#300775,#300776,#300777,#300778,#300779,#300780,
#300781,#300782,#300783,#300784,#300785,#300786,#300787,#300788,#300789,
#300790,#300791,#300792,#300793,#300794,#300795,#300796,#300797,#300798,
#300799,#300800,#300801,#300802,#300803,#300804,#300805,#300806,#300807,
#300808,#300809,#300810,#300811,#300812,#300813,#300814,#300815,#300816,
#300817,#300818,#300819,#300820,#300821,#300822,#300823,#300824,#300825,
#300826,#300827,#300828,#300829,#300830,#300831,#300832,#300833,#300834,
#300835,#300836,#300837,#300838,#300839,#300840,#300841,#300842,#300843,
#300844,#300845,#300846,#300847,#300848,#300849,#300850,#300851,#300852,
#300853,#300854,#300855,#300856,#300857,#300858,#300859,#300860,#300861,
#300862,#300863,#300864,#300865,#300866,#300867,#300868,#300869,#300870,
#300871,#300872,#300873,#300874,#300875,#300876,#300877,#300878,#300879,
#300880,#300881,#300882,#300883,#300884,#300885,#300886,#300887,#300888,
#300889,#300890,#300891,#300892,#300893,#300894,#300895,#300896,#300897,
#300898,#300899,#300900,#300901,#300902,#300903,#300904,#300905,#300906,
#300907,#300908,#300909,#300910,#300911,#300912,#300913,#300914,#300915,
#300916,#300917,#300918,#300919,#300920,#300921,#300922,#300923,#300924,
#300925,#300926,#300927,#300928,#300929,#300930,#300931,#300932,#300933,
#300934,#300935,#300936,#300937,#300938,#300939,#300940,#300941,#300942,
#300943,#300944,#300945,#300946,#300947,#300948,#300949,#300950,#300951,
#300952,#300953,#300954,#300955,#300956,#300957,#300958,#300959,#300960,
#300961,#300962,#300963,#300964,#300965,#300966,#300967,#300968,#300969,
#300970,#300971,#300972,#300973,#300974,#300975,#300976,#300977,#300978,
#300979,#300980,#300981,#300982,#300983,#300984,#300985,#300986,#300987,
#300988,#300989,#300990,#300991,#300992,#300993,#300994,#300995,#300996,
#300997,#300998,#300999,#301000,#301001,#301002,#301003,#301004,#301005,
#301006,#301007,#301008,#301009,#301010,#301011,#301012,#301013,#301014,
#301015,#301016,#301017,#301018,#301019,#301020,#301021,#301022,#301023,
#301024,#301025,#301026,#301027,#301028,#301029,#301030,#301031,#301032,
#301033,#301034,#301035,#301036,#301037,#301038,#301039,#301040,#301041,
#301042,#301043,#301044,#301045,#301046,#301047,#301048,#301049,#301050,
#301051,#301052,#301053,#301054,#301055,#301056,#301057,#301058,#301059,
#301060,#301061,#301062,#301063,#301064,#301065,#301066,#301067,#301068,
#301069,#301070,#301071,#301072,#301073,#301074,#301075,#301076,#301077,
#301078,#301079,#301080,#301081,#301082,#301083,#301084,#301085,#301086,
#301087,#301088,#301089,#301090,#301091,#301092,#301093,#301094,#301095,
#301096,#301097,#301098,#301099,#301100,#301101,#301102,#301103,#301104,
#301105,#301106,#301107,#301108,#301109,#301110,#301111,#301112,#301113,
#301114,#301115,#301116,#301117,#301118,#301119,#301120,#301121,#301122,
#301123,#301124,#301125,#301126,#301127,#301128,#301129,#301130,#301131,
#301132,#301133,#301134,#301135,#301136,#301137,#301138,#301139,#301140,
#301141,#301142,#301143,#301144,#301145,#301146,#301147,#301148,#301149,
#301150,#301151,#301152,#301153,#301154,#301155,#301156,#301157,#301158,
#301159,#301160,#301161,#301162,#301163,#301164,#301165,#301166,#301167,
#301168,#301169,#301170,#301171,#301172,#301173,#301174,#301175,#301176,
#301177,#301178,#301179,#301180,#301181,#301182,#301183,#301184,#301185,
#301186,#301187,#301188,#301189,#301190,#301191,#301192,#301193,#301194,
#301195,#301196,#301197,#301198,#301199,#301200,#301201,#301202,#301203,
#301204,#301205,#301206,#301207,#301208,#301209,#301210,#301211,#301212,
#301213,#301214,#301215,#301216,#301217,#301218,#301219,#301220,#301221,
#301222,#301223,#301224,#301225,#301226,#301227,#301228,#301229,#301230,
#301231,#301232,#301233,#301234,#301235,#301236,#301237,#301238,#301239,
#301240,#301241,#301242,#301243,#301244,#301245,#301246,#301247,#301248,
#301249,#301250,#301251,#301252,#301253,#301254,#301255,#301256,#301257,
#301258,#301259,#301260,#301261,#301262,#301263,#301264,#301265,#301266,
#301267,#301268,#301269,#301270,#301271,#301272,#301273,#301274,#301275,
#301276,#301277,#301278,#301279,#301280,#301281,#301282,#301283,#301284,
#301285,#301286,#301287,#301288,#301289,#301290,#301291,#301292,#301293,
#301294,#301295,#301296,#301297,#301298,#301299,#301300,#301301,#301302,
#301303,#301304,#301305,#301306,#301307,#301308,#301309,#301310,#301311,
#301312,#301313,#301314,#301315,#301316,#301317,#301318,#301319,#301320,
#301321,#301322,#301323,#301324,#301325,#301326,#301327,#301328,#301329,
#301330,#301331,#301332,#301333,#301334,#301335,#301336,#301337,#301338,
#301339,#301340,#301341,#301342,#301343,#301344,#301345,#301346,#301347,
#301348,#301349,#301350,#301351,#301352,#301353,#301354,#301355,#301356,
#301357,#301358,#301359,#301360,#301361,#301362,#301363,#301364,#301365,
#301366,#301367,#301368,#301369,#301370,#301371,#301372,#301373,#301374,
#301375,#301376,#301377,#301378,#301379,#301380,#301381,#301382,#301383,
#301384,#301385,#301386,#301387,#301388,#301389,#301390,#301391,#301392,
#301393,#301394,#301395,#301396,#301397,#301398,#301399,#301400,#301401,
#301402,#301403,#301404,#301405,#301406,#301407,#301408,#301409,#301410,
#301411,#301412,#301413,#301414,#301415,#301416,#301417,#301418,#301419,
#301420,#301421,#301422,#301423,#301424,#301425,#301426,#301427,#301428,
#301429,#301430,#301431,#301432,#301433,#301434,#301435,#301436,#301437,
#301438,#301439,#301440,#301441,#301442,#301443,#301444,#301445,#301446,
#301447,#301448,#301449,#301450,#301451,#301452,#301453,#301454,#301455,
#301456,#301457,#301458,#301459,#301460,#301461,#301462,#301463,#301464,
#301465,#301466,#301467,#301468,#301469,#301470,#301471,#301472,#301473,
#301474,#301475,#301476,#301477,#301478,#301479,#301480,#301481,#301482,
#301483,#301484,#301485,#301486,#301487,#301488,#301489,#301490,#301491,
#301492,#301493,#301494,#301495,#301496,#301497,#301498,#301499,#301500,
#301501,#301502,#301503,#301504,#301505,#301506,#301507,#301508,#301509,
#301510,#301511,#301512,#301513,#301514,#301515,#301516,#301517,#301518,
#301519,#301520,#301521,#301522,#301523,#301524,#301525,#301526,#301527,
#301528,#301529,#301530,#301531,#301532,#301533,#301534,#301535,#301536,
#301537,#301538,#301539,#301540,#301541,#301542,#301543,#301544,#301545,
#301546,#301547,#301548,#301549,#301550,#301551,#301552,#301553,#301554,
#301555,#301556,#301557,#301558,#301559,#301560,#301561,#301562,#301563,
#301564,#301565,#301566,#301567,#301568,#301569,#301570,#301571,#301572,
#301573,#301574,#301575,#301576,#301577),(#301578,#301579,#301580,#301581,
#301582,#301583,#301584,#301585,#301586,#301587,#301588,#301589,#301590,
#301591,#301592,#301593,#301594,#301595,#301596,#301597,#301598,#301599,
#301600,#301601,#301602,#301603,#301604,#301605,#301606,#301607,#301608,
#301609,#301610,#301611,#301612,#301613,#301614,#301615,#301616,#301617,
#301618,#301619,#301620,#301621,#301622,#301623,#301624,#301625,#301626,
#301627,#301628,#301629,#301630,#301631,#301632,#301633,#301634,#301635,
#301636,#301637,#301638,#301639,#301640,#301641,#301642,#301643,#301644,
#301645,#301646,#301647,#301648,#301649,#301650,#301651,#301652,#301653,
#301654,#301655,#301656,#301657,#301658,#301659,#301660,#301661,#301662,
#301663,#301664,#301665,#301666,#301667,#301668,#301669,#301670,#301671,
#301672,#301673,#301674,#301675,#301676,#301677,#301678,#301679,#301680,
#301681,#301682,#301683,#301684,#301685,#301686,#301687,#301688,#301689,
#301690,#301691,#301692,#301693,#301694,#301695,#301696,#301697,#301698,
#301699,#301700,#301701,#301702,#301703,#301704,#301705,#301706,#301707,
#301708,#301709,#301710,#301711,#301712,#301713,#301714,#301715,#301716,
#301717,#301718,#301719,#301720,#301721,#301722,#301723,#301724,#301725,
#301726,#301727,#301728,#301729,#301730,#301731,#301732,#301733,#301734,
#301735,#301736,#301737,#301738,#301739,#301740,#301741,#301742,#301743,
#301744,#301745,#301746,#301747,#301748,#301749,#301750,#301751,#301752,
#301753,#301754,#301755,#301756,#301757,#301758,#301759,#301760,#301761,
#301762,#301763,#301764,#301765,#301766,#301767,#301768,#301769,#301770,
#301771,#301772,#301773,#301774,#301775,#301776,#301777,#301778,#301779,
#301780,#301781,#301782,#301783,#301784,#301785,#301786,#301787,#301788,
#301789,#301790,#301791,#301792,#301793,#301794,#301795,#301796,#301797,
#301798,#301799,#301800,#301801,#301802,#301803,#301804,#301805,#301806,
#301807,#301808,#301809,#301810,#301811,#301812,#301813,#301814,#301815,
#301816,#301817,#301818,#301819,#301820,#301821,#301822,#301823,#301824,
#301825,#301826,#301827,#301828,#301829,#301830,#301831,#301832,#301833,
#301834,#301835,#301836,#301837,#301838,#301839,#301840,#301841,#301842,
#301843,#301844,#301845,#301846,#301847,#301848,#301849,#301850,#301851,
#301852,#301853,#301854,#301855,#301856,#301857,#301858,#301859,#301860,
#301861,#301862,#301863,#301864,#301865,#301866,#301867,#301868,#301869,
#301870,#301871,#301872,#301873,#301874,#301875,#301876,#301877,#301878,
#301879,#301880,#301881,#301882,#301883,#301884,#301885,#301886,#301887,
#301888,#301889,#301890,#301891,#301892,#301893,#301894,#301895,#301896,
#301897,#301898,#301899,#301900,#301901,#301902,#301903,#301904,#301905,
#301906,#301907,#301908,#301909,#301910,#301911,#301912,#301913,#301914,
#301915,#301916,#301917,#301918,#301919,#301920,#301921,#301922,#301923,
#301924,#301925,#301926,#301927,#301928,#301929,#301930,#301931,#301932,
#301933,#301934,#301935,#301936,#301937,#301938,#301939,#301940,#301941,
#301942,#301943,#301944,#301945,#301946,#301947,#301948,#301949,#301950,
#301951,#301952,#301953,#301954,#301955,#301956,#301957,#301958,#301959,
#301960,#301961,#301962,#301963,#301964,#301965,#301966,#301967,#301968,
#301969,#301970,#301971,#301972,#301973,#301974,#301975,#301976,#301977,
#301978,#301979,#301980,#301981,#301982,#301983,#301984,#301985,#301986,
#301987,#301988,#301989,#301990,#301991,#301992,#301993,#301994,#301995,
#301996,#301997,#301998,#301999,#302000,#302001,#302002,#302003,#302004,
#302005,#302006,#302007,#302008,#302009,#302010,#302011,#302012,#302013,
#302014,#302015,#302016,#302017,#302018,#302019,#302020,#302021,#302022,
#302023,#302024,#302025,#302026,#302027,#302028,#302029,#302030,#302031,
#302032,#302033,#302034,#302035,#302036,#302037,#302038,#302039,#302040,
#302041,#302042,#302043,#302044,#302045,#302046,#302047,#302048,#302049,
#302050,#302051,#302052,#302053,#302054,#302055,#302056,#302057,#302058,
#302059,#302060,#302061,#302062,#302063,#302064,#302065,#302066,#302067,
#302068,#302069,#302070,#302071,#302072,#302073,#302074,#302075,#302076,
#302077,#302078,#302079,#302080,#302081,#302082,#302083,#302084,#302085,
#302086,#302087,#302088,#302089,#302090,#302091,#302092,#302093,#302094,
#302095,#302096,#302097,#302098,#302099,#302100,#302101,#302102,#302103,
#302104,#302105,#302106,#302107,#302108,#302109,#302110,#302111,#302112,
#302113,#302114,#302115,#302116,#302117,#302118,#302119,#302120,#302121,
#302122,#302123,#302124,#302125,#302126,#302127,#302128,#302129,#302130,
#302131,#302132,#302133,#302134,#302135,#302136,#302137,#302138,#302139,
#302140,#302141,#302142,#302143,#302144,#302145,#302146,#302147,#302148,
#302149,#302150,#302151,#302152,#302153,#302154,#302155,#302156,#302157,
#302158,#302159,#302160,#302161,#302162,#302163,#302164,#302165,#302166,
#302167,#302168,#302169,#302170,#302171,#302172,#302173,#302174,#302175,
#302176,#302177,#302178,#302179,#302180,#302181,#302182,#302183,#302184,
#302185,#302186,#302187,#302188,#302189,#302190,#302191,#302192,#302193,
#302194,#302195,#302196,#302197,#302198,#302199,#302200,#302201,#302202,
#302203,#302204,#302205,#302206,#302207,#302208,#302209,#302210,#302211,
#302212,#302213,#302214,#302215,#302216,#302217,#302218,#302219,#302220,
#302221,#302222,#302223,#302224,#302225,#302226,#302227,#302228,#302229,
#302230,#302231,#302232,#302233,#302234,#302235,#302236,#302237,#302238,
#302239,#302240,#302241,#302242,#302243,#302244,#302245,#302246,#302247,
#302248,#302249,#302250,#302251,#302252,#302253,#302254,#302255,#302256,
#302257,#302258,#302259,#302260,#302261,#302262,#302263,#302264,#302265,
#302266,#302267,#302268,#302269,#302270,#302271,#302272,#302273,#302274,
#302275,#302276,#302277,#302278,#302279,#302280,#302281,#302282,#302283,
#302284,#302285,#302286,#302287,#302288,#302289,#302290,#302291,#302292,
#302293,#302294,#302295,#302296,#302297,#302298,#302299,#302300,#302301,
#302302,#302303,#302304,#302305,#302306,#302307,#302308,#302309,#302310,
#302311,#302312,#302313,#302314,#302315,#302316,#302317,#302318,#302319,
#302320,#302321,#302322,#302323,#302324,#302325,#302326,#302327,#302328,
#302329,#302330,#302331,#302332,#302333,#302334,#302335,#302336,#302337,
#302338,#302339,#302340,#302341,#302342,#302343,#302344,#302345,#302346,
#302347,#302348,#302349,#302350,#302351,#302352,#302353,#302354,#302355,
#302356,#302357,#302358,#302359,#302360,#302361,#302362,#302363,#302364,
#302365,#302366,#302367,#302368,#302369,#302370,#302371,#302372,#302373,
#302374,#302375,#302376,#302377,#302378,#302379,#302380,#302381,#302382,
#302383,#302384,#302385,#302386,#302387,#302388,#302389,#302390,#302391,
#302392,#302393,#302394,#302395,#302396,#302397,#302398,#302399,#302400,
#302401,#302402,#302403,#302404,#302405,#302406,#302407,#302408,#302409,
#302410,#302411,#302412,#302413,#302414,#302415,#302416,#302417,#302418,
#302419,#302420,#302421,#302422,#302423,#302424,#302425,#302426,#302427,
#302428,#302429,#302430,#302431,#302432,#302433,#302434,#302435,#302436,
#302437,#302438,#302439,#302440,#302441,#302442,#302443,#302444,#302445,
#302446,#302447,#302448,#302449,#302450,#302451,#302452,#302453,#302454,
#302455,#302456,#302457,#302458,#302459,#302460,#302461,#302462,#302463,
#302464,#302465,#302466,#302467,#302468,#302469,#302470,#302471,#302472,
#302473,#302474,#302475,#302476,#302477,#302478,#302479,#302480,#302481,
#302482,#302483,#302484,#302485,#302486,#302487,#302488,#302489,#302490,
#302491,#302492,#302493,#302494,#302495,#302496,#302497,#302498,#302499,
#302500,#302501,#302502,#302503,#302504,#302505,#302506,#302507,#302508,
#302509,#302510,#302511,#302512,#302513,#302514,#302515,#302516,#302517,
#302518,#302519,#302520,#302521,#302522,#302523,#302524,#302525,#302526,
#302527,#302528,#302529,#302530,#302531,#302532,#302533,#302534,#302535,
#302536,#302537,#302538,#302539,#302540,#302541,#302542,#302543,#302544,
#302545,#302546,#302547,#302548,#302549,#302550,#302551,#302552,#302553,
#302554,#302555,#302556,#302557,#302558,#302559,#302560,#302561,#302562,
#302563,#302564,#302565,#302566,#302567,#302568,#302569,#302570,#302571,
#302572,#302573,#302574,#302575,#302576,#302577,#302578,#302579,#302580,
#302581,#302582,#302583,#302584,#302585,#302586,#302587,#302588,#302589,
#302590,#302591,#302592,#302593,#302594,#302595,#302596,#302597,#302598,
#302599,#302600,#302601,#302602,#302603,#302604,#302605,#302606,#302607,
#302608,#302609,#302610,#302611,#302612,#302613,#302614)),.UNSPECIFIED.,
 .F.,.F.,.F.)
B_SPLINE_SURFACE_WITH_KNOTS((2,2),(3,2,2,2,2,2,2,2,2,2,2,2,2,2,2,2,2,2,
2,2,2,2,2,2,2,2,2,2,2,2,2,2,2,2,2,2,2,2,2,2,2,2,2,2,2,2,2,2,2,2,2,2,2,2,
2,2,2,2,2,2,2,2,2,2,2,2,2,2,2,2,2,2,2,2,2,2,2,2,2,2,2,2,2,2,2,2,2,2,2,2,
2,2,2,2,2,2,2,2,2,2,2,2,2,2,2,2,2,2,2,2,2,2,2,2,2,2,2,2,2,2,2,2,2,2,2,2,
2,2,2,2,2,2,2,2,2,2,2,2,2,2,2,2,2,2,2,2,2,2,2,2,2,2,2,2,2,2,2,2,2,2,2,2,
2,2,2,2,2,2,2,2,2,2,2,2,2,2,2,2,2,2,2,2,2,2,2,2,2,2,2,2,2,2,2,2,2,2,2,2,
2,2,2,2,2,2,2,2,2,2,2,2,2,2,2,2,2,2,2,2,2,2,2,2,2,2,2,2,2,2,2,2,2,2,2,2,
2,2,2,2,2,2,2,2,2,2,2,2,2,2,2,2,2,2,2,2,2,2,2,2,2,2,2,2,2,2,2,2,2,2,2,2,
2,2,2,2,2,2,2,2,2,2,2,2,2,2,2,2,2,2,2,2,2,2,2,2,2,2,2,2,2,2,2,2,2,2,2,2,
2,2,2,2,2,2,2,2,2,2,2,2,2,2,2,2,2,2,2,2,2,2,2,2,2,2,2,2,2,2,2,2,2,2,2,2,
2,2,2,2,2,2,2,2,2,2,2,2,2,2,2,2,2,2,2,2,2,2,2,2,2,2,2,2,2,2,2,2,2,2,2,2,
2,2,2,2,2,2,2,2,2,2,2,2,2,2,2,2,2,2,2,2,2,2,2,2,2,2,2,2,2,2,2,2,2,2,2,2,
2,2,2,2,2,2,2,2,2,2,2,2,2,2,2,2,2,2,2,2,2,2,2,2,2,2,2,2,2,2,2,2,2,2,2,2,
2,2,2,2,2,2,2,2,2,2,2,2,2,2,2,2,2,2,2,2,2,2,2,2,2,2,2,2,2,2,2,2,2,2,2,2,
2,2,2,2,2,2,2,2,2,2,2,2,2,2,2,2,2,2,2,2,2,2,2,2,2,2,2,2,2,2,2,2,3),(0.,
1.),(0.,0.00192307692307692,0.00384615384615385,0.00576923076923077,0.00769230769230769,
0.00961538461538462,0.0115384615384615,0.0134615384615385,0.0153846153846154,
0.0173076923076923,0.0192307692307692,0.0211538461538462,0.0230769230769231,
0.025,0.0269230769230769,0.0288461538461538,0.0307692307692308,0.0326923076923077,
0.0346153846153846,0.0365384615384615,0.0384615384615385,0.0403846153846154,
0.0423076923076923,0.0442307692307692,0.0461538461538462,0.0480769230769231,
0.05,0.0519230769230769,0.0538461538461538,0.0557692307692308,0.0576923076923077,
0.0596153846153846,0.0615384615384615,0.0634615384615385,0.0653846153846154,
0.0673076923076923,0.0692307692307692,0.0711538461538462,0.0730769230769231,
0.075,0.0769230769230769,0.0788461538461538,0.0807692307692308,0.0826923076923077,
0.0846153846153846,0.0865384615384615,0.0884615384615385,0.0903846153846154,
0.0923076923076923,0.0942307692307692,0.0961538461538462,0.0980769230769231,
0.1,0.101923076923077,0.103846153846154,0.105769230769231,0.107692307692308,
0.109615384615385,0.111538461538462,0.113461538461538,0.115384615384615,
0.117307692307692,0.119230769230769,0.121153846153846,0.123076923076923,
0.125,0.126923076923077,0.128846153846154,0.130769230769231,0.132692307692308,
0.134615384615385,0.136538461538462,0.138461538461538,0.140384615384615,
0.142307692307692,0.144230769230769,0.146153846153846,0.148076923076923,
0.15,0.151923076923077,0.153846153846154,0.155769230769231,0.157692307692308,
0.159615384615385,0.161538461538462,0.163461538461538,0.165384615384615,
0.167307692307692,0.169230769230769,0.171153846153846,0.173076923076923,
0.175,0.176923076923077,0.178846153846154,0.180769230769231,0.182692307692308,
0.184615384615385,0.186538461538462,0.188461538461538,0.190384615384615,
0.192307692307692,0.194230769230769,0.196153846153846,0.198076923076923,
0.2,0.201923076923077,0.203846153846154,0.205769230769231,0.207692307692308,
0.209615384615385,0.211538461538462,0.213461538461538,0.215384615384615,
0.217307692307692,0.219230769230769,0.221153846153846,0.223076923076923,
0.225,0.226923076923077,0.228846153846154,0.230769230769231,0.232692307692308,
0.234615384615385,0.236538461538462,0.238461538461538,0.240384615384615,
0.242307692307692,0.244230769230769,0.246153846153846,0.248076923076923,
0.25,0.251923076923077,0.253846153846154,0.255769230769231,0.257692307692308,
0.259615384615385,0.261538461538462,0.263461538461538,0.265384615384615,
0.267307692307692,0.269230769230769,0.271153846153846,0.273076923076923,
0.275,0.276923076923077,0.278846153846154,0.280769230769231,0.282692307692308,
0.284615384615385,0.286538461538462,0.288461538461538,0.290384615384615,
0.292307692307692,0.294230769230769,0.296153846153846,0.298076923076923,
0.3,0.301923076923077,0.303846153846154,0.305769230769231,0.307692307692308,
0.309615384615385,0.311538461538462,0.313461538461538,0.315384615384615,
0.317307692307692,0.319230769230769,0.321153846153846,0.323076923076923,
0.325,0.326923076923077,0.328846153846154,0.330769230769231,0.332692307692308,
0.334615384615385,0.336538461538462,0.338461538461538,0.340384615384615,
0.342307692307692,0.344230769230769,0.346153846153846,0.348076923076923,
0.35,0.351923076923077,0.353846153846154,0.355769230769231,0.357692307692308,
0.359615384615385,0.361538461538462,0.363461538461538,0.365384615384615,
0.367307692307692,0.369230769230769,0.371153846153846,0.373076923076923,
0.375,0.376923076923077,0.378846153846154,0.380769230769231,0.382692307692308,
0.384615384615385,0.386538461538462,0.388461538461538,0.390384615384615,
0.392307692307692,0.394230769230769,0.396153846153846,0.398076923076923,
0.4,0.401923076923077,0.403846153846154,0.405769230769231,0.407692307692308,
0.409615384615385,0.411538461538462,0.413461538461538,0.415384615384615,
0.417307692307692,0.419230769230769,0.421153846153846,0.423076923076923,
0.425,0.426923076923077,0.428846153846154,0.430769230769231,0.432692307692308,
0.434615384615385,0.436538461538462,0.438461538461538,0.440384615384615,
0.442307692307692,0.444230769230769,0.446153846153846,0.448076923076923,
0.45,0.451923076923077,0.453846153846154,0.455769230769231,0.457692307692308,
0.459615384615385,0.461538461538462,0.463461538461538,0.465384615384615,
0.467307692307692,0.469230769230769,0.471153846153846,0.473076923076923,
0.475,0.476923076923077,0.478846153846154,0.480769230769231,0.482692307692308,
0.484615384615385,0.486538461538462,0.488461538461538,0.490384615384615,
0.492307692307692,0.494230769230769,0.496153846153846,0.498076923076923,
0.5,0.501923076923077,0.503846153846154,0.505769230769231,0.507692307692308,
0.509615384615385,0.511538461538461,0.513461538461538,0.515384615384615,
0.517307692307692,0.519230769230769,0.521153846153846,0.523076923076923,
0.525,0.526923076923077,0.528846153846154,0.530769230769231,0.532692307692308,
0.534615384615385,0.536538461538462,0.538461538461538,0.540384615384615,
0.542307692307692,0.544230769230769,0.546153846153846,0.548076923076923,
0.55,0.551923076923077,0.553846153846154,0.555769230769231,0.557692307692308,
0.559615384615385,0.561538461538462,0.563461538461538,0.565384615384615,
0.567307692307692,0.569230769230769,0.571153846153846,0.573076923076923,
0.575,0.576923076923077,0.578846153846154,0.580769230769231,0.582692307692308,
0.584615384615385,0.586538461538462,0.588461538461538,0.590384615384615,
0.592307692307692,0.594230769230769,0.596153846153846,0.598076923076923,
0.6,0.601923076923077,0.603846153846154,0.605769230769231,0.607692307692308,
0.609615384615385,0.611538461538462,0.613461538461539,0.615384615384615,
0.617307692307692,0.619230769230769,0.621153846153846,0.623076923076923,
0.625,0.626923076923077,0.628846153846154,0.630769230769231,0.632692307692308,
0.634615384615385,0.636538461538461,0.638461538461538,0.640384615384615,
0.642307692307692,0.644230769230769,0.646153846153846,0.648076923076923,
0.65,0.651923076923077,0.653846153846154,0.655769230769231,0.657692307692308,
0.659615384615385,0.661538461538462,0.663461538461538,0.665384615384615,
0.667307692307692,0.669230769230769,0.671153846153846,0.673076923076923,
0.675,0.676923076923077,0.678846153846154,0.680769230769231,0.682692307692308,
0.684615384615385,0.686538461538462,0.688461538461538,0.690384615384615,
0.692307692307692,0.694230769230769,0.696153846153846,0.698076923076923,
0.7,0.701923076923077,0.703846153846154,0.705769230769231,0.707692307692308,
0.709615384615385,0.711538461538462,0.713461538461538,0.715384615384615,
0.717307692307692,0.719230769230769,0.721153846153846,0.723076923076923,
0.725,0.726923076923077,0.728846153846154,0.730769230769231,0.732692307692308,
0.734615384615385,0.736538461538462,0.738461538461539,0.740384615384615,
0.742307692307692,0.744230769230769,0.746153846153846,0.748076923076923,
0.75,0.751923076923077,0.753846153846154,0.755769230769231,0.757692307692308,
0.759615384615385,0.761538461538461,0.763461538461538,0.765384615384615,
0.767307692307692,0.769230769230769,0.771153846153846,0.773076923076923,
0.775,0.776923076923077,0.778846153846154,0.780769230769231,0.782692307692308,
0.784615384615385,0.786538461538462,0.788461538461538,0.790384615384615,
0.792307692307692,0.794230769230769,0.796153846153846,0.798076923076923,
0.8,0.801923076923077,0.803846153846154,0.805769230769231,0.807692307692308,
0.809615384615385,0.811538461538462,0.813461538461538,0.815384615384615,
0.817307692307692,0.819230769230769,0.821153846153846,0.823076923076923,
0.825,0.826923076923077,0.828846153846154,0.830769230769231,0.832692307692308,
0.834615384615385,0.836538461538462,0.838461538461538,0.840384615384615,
0.842307692307692,0.844230769230769,0.846153846153846,0.848076923076923,
0.85,0.851923076923077,0.853846153846154,0.855769230769231,0.857692307692308,
0.859615384615385,0.861538461538462,0.863461538461539,0.865384615384615,
0.867307692307692,0.869230769230769,0.871153846153846,0.873076923076923,
0.875,0.876923076923077,0.878846153846154,0.880769230769231,0.882692307692308,
0.884615384615385,0.886538461538461,0.888461538461538,0.890384615384615,
0.892307692307692,0.894230769230769,0.896153846153846,0.898076923076923,
0.9,0.901923076923077,0.903846153846154,0.905769230769231,0.907692307692308,
0.909615384615385,0.911538461538462,0.913461538461538,0.915384615384615,
0.917307692307692,0.919230769230769,0.921153846153846,0.923076923076923,
0.925,0.926923076923077,0.928846153846154,0.930769230769231,0.932692307692308,
0.934615384615385,0.936538461538462,0.938461538461538,0.940384615384615,
0.942307692307692,0.944230769230769,0.946153846153846,0.948076923076923,
0.95,0.951923076923077,0.953846153846154,0.955769230769231,0.957692307692308,
0.959615384615385,0.961538461538462,0.963461538461538,0.965384615384615,
0.967307692307692,0.969230769230769,0.971153846153846,0.973076923076923,
0.975,0.976923076923077,0.978846153846154,0.980769230769231,0.982692307692308,
0.984615384615385,0.986538461538462,0.988461538461539,0.990384615384615,
0.992307692307692,0.994230769230769,0.996153846153846),.UNSPECIFIED.)
GEOMETRIC_REPRESENTATION_ITEM()
RATIONAL_B_SPLINE_SURFACE(((1.,0.951056516295154,1.,0.951056516295154,1.,
0.951056516295154,1.,0.951056516295154,1.,0.951056516295154,1.,0.951056516295154,
1.,0.951056516295154,1.,0.951056516295154,1.,0.951056516295154,1.,0.951056516295154,
1.,0.951056516295154,1.,0.951056516295154,1.,0.951056516295154,1.,0.951056516295154,
1.,0.951056516295154,1.,0.951056516295154,1.,0.951056516295154,1.,0.951056516295154,
1.,0.951056516295154,1.,0.951056516295154,1.,0.951056516295154,1.,0.951056516295154,
1.,0.951056516295154,1.,0.951056516295154,1.,0.951056516295154,1.,0.951056516295154,
1.,0.951056516295154,1.,0.951056516295154,1.,0.951056516295154,1.,0.951056516295154,
1.,0.951056516295154,1.,0.951056516295154,1.,0.951056516295154,1.,0.951056516295154,
1.,0.951056516295154,1.,0.951056516295154,1.,0.951056516295154,1.,0.951056516295154,
1.,0.951056516295154,1.,0.951056516295154,1.,0.951056516295154,1.,0.951056516295154,
1.,0.951056516295154,1.,0.951056516295154,1.,0.951056516295154,1.,0.951056516295154,
1.,0.951056516295154,1.,0.951056516295154,1.,0.951056516295154,1.,0.951056516295154,
1.,0.951056516295154,1.,0.951056516295154,1.,0.951056516295154,1.,0.951056516295154,
1.,0.951056516295154,1.,0.951056516295154,1.,0.951056516295154,1.,0.951056516295154,
1.,0.951056516295154,1.,0.951056516295154,1.,0.951056516295154,1.,0.951056516295154,
1.,0.951056516295154,1.,0.951056516295154,1.,0.951056516295154,1.,0.951056516295154,
1.,0.951056516295154,1.,0.951056516295154,1.,0.951056516295154,1.,0.951056516295154,
1.,0.951056516295154,1.,0.951056516295154,1.,0.951056516295154,1.,0.951056516295154,
1.,0.951056516295154,1.,0.951056516295154,1.,0.951056516295154,1.,0.951056516295154,
1.,0.951056516295154,1.,0.951056516295154,1.,0.951056516295154,1.,0.951056516295154,
1.,0.951056516295154,1.,0.951056516295154,1.,0.951056516295154,1.,0.951056516295154,
1.,0.951056516295154,1.,0.951056516295154,1.,0.951056516295154,1.,0.951056516295154,
1.,0.951056516295154,1.,0.951056516295154,1.,0.951056516295154,1.,0.951056516295154,
1.,0.951056516295154,1.,0.951056516295154,1.,0.951056516295154,1.,0.951056516295154,
1.,0.951056516295154,1.,0.951056516295154,1.,0.951056516295154,1.,0.951056516295154,
1.,0.951056516295154,1.,0.951056516295154,1.,0.951056516295154,1.,0.951056516295154,
1.,0.951056516295154,1.,0.951056516295154,1.,0.951056516295154,1.,0.951056516295154,
1.,0.951056516295154,1.,0.951056516295154,1.,0.951056516295154,1.,0.951056516295154,
1.,0.951056516295154,1.,0.951056516295154,1.,0.951056516295154,1.,0.951056516295154,
1.,0.951056516295154,1.,0.951056516295154,1.,0.951056516295154,1.,0.951056516295154,
1.,0.951056516295154,1.,0.951056516295154,1.,0.951056516295154,1.,0.951056516295154,
1.,0.951056516295154,1.,0.951056516295154,1.,0.951056516295154,1.,0.951056516295154,
1.,0.951056516295154,1.,0.951056516295154,1.,0.951056516295154,1.,0.951056516295154,
1.,0.951056516295154,1.,0.951056516295154,1.,0.951056516295154,1.,0.951056516295154,
1.,0.951056516295154,1.,0.951056516295154,1.,0.951056516295154,1.,0.951056516295154,
1.,0.951056516295154,1.,0.951056516295154,1.,0.951056516295154,1.,0.951056516295154,
1.,0.951056516295154,1.,0.951056516295154,1.,0.951056516295154,1.,0.951056516295154,
1.,0.951056516295154,1.,0.951056516295154,1.,0.951056516295154,1.,0.951056516295154,
1.,0.951056516295154,1.,0.951056516295154,1.,0.951056516295154,1.,0.951056516295154,
1.,0.951056516295154,1.,0.951056516295154,1.,0.951056516295154,1.,0.951056516295154,
1.,0.951056516295154,1.,0.951056516295154,1.,0.951056516295154,1.,0.951056516295154,
1.,0.951056516295154,1.,0.951056516295154,1.,0.951056516295154,1.,0.951056516295154,
1.,0.951056516295154,1.,0.951056516295154,1.,0.951056516295154,1.,0.951056516295154,
1.,0.951056516295154,1.,0.951056516295154,1.,0.951056516295154,1.,0.951056516295154,
1.,0.951056516295154,1.,0.951056516295154,1.,0.951056516295154,1.,0.951056516295154,
1.,0.951056516295154,1.,0.951056516295154,1.,0.951056516295154,1.,0.951056516295154,
1.,0.951056516295154,1.,0.951056516295154,1.,0.951056516295154,1.,0.951056516295154,
1.,0.951056516295154,1.,0.951056516295154,1.,0.951056516295154,1.,0.951056516295154,
1.,0.951056516295154,1.,0.951056516295154,1.,0.951056516295154,1.,0.951056516295154,
1.,0.951056516295154,1.,0.951056516295154,1.,0.951056516295154,1.,0.951056516295154,
1.,0.951056516295154,1.,0.951056516295154,1.,0.951056516295154,1.,0.951056516295154,
1.,0.951056516295154,1.,0.951056516295154,1.,0.951056516295154,1.,0.951056516295154,
1.,0.951056516295154,1.,0.951056516295154,1.,0.951056516295154,1.,0.951056516295154,
1.,0.951056516295154,1.,0.951056516295154,1.,0.951056516295154,1.,0.951056516295154,
1.,0.951056516295154,1.,0.951056516295154,1.,0.951056516295154,1.,0.951056516295154,
1.,0.951056516295154,1.,0.951056516295154,1.,0.951056516295154,1.,0.951056516295154,
1.,0.951056516295154,1.,0.951056516295154,1.,0.951056516295154,1.,0.951056516295154,
1.,0.951056516295154,1.,0.951056516295154,1.,0.951056516295154,1.,0.951056516295154,
1.,0.951056516295154,1.,0.951056516295154,1.,0.951056516295154,1.,0.951056516295154,
1.,0.951056516295154,1.,0.951056516295154,1.,0.951056516295154,1.,0.951056516295154,
1.,0.951056516295154,1.,0.951056516295154,1.,0.951056516295154,1.,0.951056516295154,
1.,0.951056516295154,1.,0.951056516295154,1.,0.951056516295154,1.,0.951056516295154,
1.,0.951056516295154,1.,0.951056516295154,1.,0.951056516295154,1.,0.951056516295154,
1.,0.951056516295154,1.,0.951056516295154,1.,0.951056516295154,1.,0.951056516295154,
1.,0.951056516295154,1.,0.951056516295154,1.,0.951056516295154,1.,0.951056516295154,
1.,0.951056516295154,1.,0.951056516295154,1.,0.951056516295154,1.,0.951056516295154,
1.,0.951056516295154,1.,0.951056516295154,1.,0.951056516295154,1.,0.951056516295154,
1.,0.951056516295154,1.,0.951056516295154,1.,0.951056516295154,1.,0.951056516295154,
1.,0.951056516295154,1.,0.951056516295154,1.,0.951056516295154,1.,0.951056516295154,
1.,0.951056516295154,1.,0.951056516295154,1.,0.951056516295154,1.,0.951056516295154,
1.,0.951056516295154,1.,0.951056516295154,1.,0.951056516295154,1.,0.951056516295154,
1.,0.951056516295154,1.,0.951056516295154,1.,0.951056516295154,1.,0.951056516295154,
1.,0.951056516295154,1.,0.951056516295154,1.,0.951056516295154,1.,0.951056516295154,
1.,0.951056516295154,1.,0.951056516295154,1.,0.951056516295154,1.,0.951056516295154,
1.,0.951056516295154,1.,0.951056516295154,1.,0.951056516295154,1.,0.951056516295154,
1.,0.951056516295154,1.,0.951056516295154,1.,0.951056516295154,1.,0.951056516295154,
1.,0.951056516295154,1.,0.951056516295154,1.,0.951056516295154,1.,0.951056516295154,
1.,0.951056516295154,1.,0.951056516295154,1.,0.951056516295154,1.,0.951056516295154,
1.,0.951056516295154,1.,0.951056516295154,1.,0.951056516295154,1.,0.951056516295154,
1.,0.951056516295154,1.,0.951056516295154,1.,0.951056516295154,1.,0.951056516295154,
1.,0.951056516295154,1.,0.951056516295154,1.,0.951056516295154,1.,0.951056516295154,
1.,0.951056516295154,1.,0.951056516295154,1.,0.951056516295154,1.,0.951056516295154,
1.,0.951056516295154,1.,0.951056516295154,1.,0.951056516295154,1.,0.951056516295154,
1.,0.951056516295154,1.,0.951056516295154,1.,0.951056516295154,1.,0.951056516295154,
1.,0.951056516295154,1.,0.951056516295154,1.,0.951056516295154,1.,0.951056516295154,
1.,0.951056516295154,1.,0.951056516295154,1.,0.951056516295154,1.,0.951056516295154,
1.,0.951056516295154,1.,0.951056516295154,1.,0.951056516295154,1.,0.951056516295154,
1.,0.951056516295154,1.,0.951056516295154,1.,0.951056516295154,1.,0.951056516295154,
1.,0.951056516295154,1.,0.951056516295154,1.,0.951056516295154,1.,0.951056516295154,
1.,0.951056516295154,1.,0.951056516295154,1.,0.951056516295154,1.,0.951056516295154,
1.,0.951056516295154,1.,0.951056516295154,1.,0.951056516295154,1.,0.951056516295154,
1.,0.951056516295154,1.,0.951056516295154,1.,0.951056516295154,1.,0.951056516295154,
1.,0.951056516295154,1.,0.951056516295154,1.,0.951056516295154,1.,0.951056516295154,
1.,0.951056516295154,1.,0.951056516295154,1.,0.951056516295154,1.,0.951056516295154,
1.,0.951056516295154,1.,0.951056516295154,1.,0.951056516295154,1.,0.951056516295154,
1.,0.951056516295154,1.,0.951056516295154,1.,0.951056516295154,1.,0.951056516295154,
1.,0.951056516295154,1.,0.951056516295154,1.,0.951056516295154,1.,0.951056516295154,
1.,0.951056516295154,1.,0.951056516295154,1.,0.951056516295154,1.,0.951056516295154,
1.,0.951056516295154,1.,0.951056516295154,1.,0.951056516295154,1.,0.951056516295154,
1.,0.951056516295154,1.,0.951056516295154,1.,0.951056516295154,1.,0.951056516295154,
1.,0.951056516295154,1.,0.951056516295154,1.,0.951056516295154,1.,0.951056516295154,
1.,0.951056516295154,1.,0.951056516295154,1.,0.951056516295154,1.,0.951056516295154,
1.,0.951056516295154,1.,0.951056516295154,1.,0.951056516295154,1.,0.951056516295154,
1.,0.951056516295154,1.,0.951056516295154,1.,0.951056516295154,1.,0.951056516295154,
1.,0.951056516295154,1.,0.951056516295154,1.,0.951056516295154,1.,0.951056516295154,
1.,0.951056516295154,1.,0.951056516295154,1.,0.951056516295154,1.,0.951056516295154,
1.,0.951056516295154,1.,0.951056516295154,1.,0.951056516295154,1.,0.951056516295154,
1.,0.951056516295154,1.,0.951056516295154,1.,0.951056516295154,1.,0.951056516295154,
1.,0.951056516295154,1.,0.951056516295154,1.,0.951056516295154,1.,0.951056516295154,
1.,0.951056516295154,1.,0.951056516295154,1.,0.951056516295154,1.,0.951056516295154,
1.,0.951056516295154,1.,0.951056516295154,1.,0.951056516295154,1.,0.951056516295154,
1.,0.951056516295154,1.,0.951056516295154,1.,0.951056516295154,1.,0.951056516295154,
1.,0.951056516295154,1.,0.951056516295154,1.,0.951056516295154,1.,0.951056516295154,
1.,0.951056516295154,1.,0.951056516295154,1.,0.951056516295154,1.,0.951056516295154,
1.,0.951056516295154,1.,0.951056516295154,1.,0.951056516295154,1.,0.951056516295154,
1.,0.951056516295154,1.,0.951056516295154,1.,0.951056516295154,1.,0.951056516295154,
1.,0.951056516295154,1.,0.951056516295154,1.,0.951056516295154,1.,0.951056516295154,
1.,0.951056516295154,1.,0.951056516295154,1.,0.951056516295154,1.,0.951056516295154,
1.,0.951056516295154,1.,0.951056516295154,1.,0.951056516295154,1.,0.951056516295154,
1.,0.951056516295154,1.,0.951056516295154,1.,0.951056516295154,1.,0.951056516295154,
1.,0.951056516295154,1.,0.951056516295154,1.,0.951056516295154,1.,0.951056516295154,
1.,0.951056516295154,1.,0.951056516295154,1.,0.951056516295154,1.,0.951056516295154,
1.,0.951056516295154,1.,0.951056516295154,1.,0.951056516295154,1.,0.951056516295154,
1.,0.951056516295154,1.,0.951056516295154,1.,0.951056516295154,1.,0.951056516295154,
1.,0.951056516295154,1.,0.951056516295154,1.,0.951056516295154,1.,0.951056516295154,
1.,0.951056516295154,1.,0.951056516295154,1.,0.951056516295154,1.,0.951056516295154,
1.,0.951056516295154,1.,0.951056516295154,1.,0.951056516295154,1.,0.951056516295154,
1.,0.951056516295154,1.,0.951056516295154,1.,0.951056516295154,1.,0.951056516295154,
1.,0.951056516295154,1.,0.951056516295154,1.,0.951056516295154,1.,0.951056516295154,
1.),(1.,0.951056516295154,1.,0.951056516295154,1.,0.951056516295154,1.,
0.951056516295154,1.,0.951056516295154,1.,0.951056516295154,1.,0.951056516295154,
1.,0.951056516295154,1.,0.951056516295154,1.,0.951056516295154,1.,0.951056516295154,
1.,0.951056516295154,1.,0.951056516295154,1.,0.951056516295154,1.,0.951056516295154,
1.,0.951056516295154,1.,0.951056516295154,1.,0.951056516295154,1.,0.951056516295154,
1.,0.951056516295154,1.,0.951056516295154,1.,0.951056516295154,1.,0.951056516295154,
1.,0.951056516295154,1.,0.951056516295154,1.,0.951056516295154,1.,0.951056516295154,
1.,0.951056516295154,1.,0.951056516295154,1.,0.951056516295154,1.,0.951056516295154,
1.,0.951056516295154,1.,0.951056516295154,1.,0.951056516295154,1.,0.951056516295154,
1.,0.951056516295154,1.,0.951056516295154,1.,0.951056516295154,1.,0.951056516295154,
1.,0.951056516295154,1.,0.951056516295154,1.,0.951056516295154,1.,0.951056516295154,
1.,0.951056516295154,1.,0.951056516295154,1.,0.951056516295154,1.,0.951056516295154,
1.,0.951056516295154,1.,0.951056516295154,1.,0.951056516295154,1.,0.951056516295154,
1.,0.951056516295154,1.,0.951056516295154,1.,0.951056516295154,1.,0.951056516295154,
1.,0.951056516295154,1.,0.951056516295154,1.,0.951056516295154,1.,0.951056516295154,
1.,0.951056516295154,1.,0.951056516295154,1.,0.951056516295154,1.,0.951056516295154,
1.,0.951056516295154,1.,0.951056516295154,1.,0.951056516295154,1.,0.951056516295154,
1.,0.951056516295154,1.,0.951056516295154,1.,0.951056516295154,1.,0.951056516295154,
1.,0.951056516295154,1.,0.951056516295154,1.,0.951056516295154,1.,0.951056516295154,
1.,0.951056516295154,1.,0.951056516295154,1.,0.951056516295154,1.,0.951056516295154,
1.,0.951056516295154,1.,0.951056516295154,1.,0.951056516295154,1.,0.951056516295154,
1.,0.951056516295154,1.,0.951056516295154,1.,0.951056516295154,1.,0.951056516295154,
1.,0.951056516295154,1.,0.951056516295154,1.,0.951056516295154,1.,0.951056516295154,
1.,0.951056516295154,1.,0.951056516295154,1.,0.951056516295154,1.,0.951056516295154,
1.,0.951056516295154,1.,0.951056516295154,1.,0.951056516295154,1.,0.951056516295154,
1.,0.951056516295154,1.,0.951056516295154,1.,0.951056516295154,1.,0.951056516295154,
1.,0.951056516295154,1.,0.951056516295154,1.,0.951056516295154,1.,0.951056516295154,
1.,0.951056516295154,1.,0.951056516295154,1.,0.951056516295154,1.,0.951056516295154,
1.,0.951056516295154,1.,0.951056516295154,1.,0.951056516295154,1.,0.951056516295154,
1.,0.951056516295154,1.,0.951056516295154,1.,0.951056516295154,1.,0.951056516295154,
1.,0.951056516295154,1.,0.951056516295154,1.,0.951056516295154,1.,0.951056516295154,
1.,0.951056516295154,1.,0.951056516295154,1.,0.951056516295154,1.,0.951056516295154,
1.,0.951056516295154,1.,0.951056516295154,1.,0.951056516295154,1.,0.951056516295154,
1.,0.951056516295154,1.,0.951056516295154,1.,0.951056516295154,1.,0.951056516295154,
1.,0.951056516295154,1.,0.951056516295154,1.,0.951056516295154,1.,0.951056516295154,
1.,0.951056516295154,1.,0.951056516295154,1.,0.951056516295154,1.,0.951056516295154,
1.,0.951056516295154,1.,0.951056516295154,1.,0.951056516295154,1.,0.951056516295154,
1.,0.951056516295154,1.,0.951056516295154,1.,0.951056516295154,1.,0.951056516295154,
1.,0.951056516295154,1.,0.951056516295154,1.,0.951056516295154,1.,0.951056516295154,
1.,0.951056516295154,1.,0.951056516295154,1.,0.951056516295154,1.,0.951056516295154,
1.,0.951056516295154,1.,0.951056516295154,1.,0.951056516295154,1.,0.951056516295154,
1.,0.951056516295154,1.,0.951056516295154,1.,0.951056516295154,1.,0.951056516295154,
1.,0.951056516295154,1.,0.951056516295154,1.,0.951056516295154,1.,0.951056516295154,
1.,0.951056516295154,1.,0.951056516295154,1.,0.951056516295154,1.,0.951056516295154,
1.,0.951056516295154,1.,0.951056516295154,1.,0.951056516295154,1.,0.951056516295154,
1.,0.951056516295154,1.,0.951056516295154,1.,0.951056516295154,1.,0.951056516295154,
1.,0.951056516295154,1.,0.951056516295154,1.,0.951056516295154,1.,0.951056516295154,
1.,0.951056516295154,1.,0.951056516295154,1.,0.951056516295154,1.,0.951056516295154,
1.,0.951056516295154,1.,0.951056516295154,1.,0.951056516295154,1.,0.951056516295154,
1.,0.951056516295154,1.,0.951056516295154,1.,0.951056516295154,1.,0.951056516295154,
1.,0.951056516295154,1.,0.951056516295154,1.,0.951056516295154,1.,0.951056516295154,
1.,0.951056516295154,1.,0.951056516295154,1.,0.951056516295154,1.,0.951056516295154,
1.,0.951056516295154,1.,0.951056516295154,1.,0.951056516295154,1.,0.951056516295154,
1.,0.951056516295154,1.,0.951056516295154,1.,0.951056516295154,1.,0.951056516295154,
1.,0.951056516295154,1.,0.951056516295154,1.,0.951056516295154,1.,0.951056516295154,
1.,0.951056516295154,1.,0.951056516295154,1.,0.951056516295154,1.,0.951056516295154,
1.,0.951056516295154,1.,0.951056516295154,1.,0.951056516295154,1.,0.951056516295154,
1.,0.951056516295154,1.,0.951056516295154,1.,0.951056516295154,1.,0.951056516295154,
1.,0.951056516295154,1.,0.951056516295154,1.,0.951056516295154,1.,0.951056516295154,
1.,0.951056516295154,1.,0.951056516295154,1.,0.951056516295154,1.,0.951056516295154,
1.,0.951056516295154,1.,0.951056516295154,1.,0.951056516295154,1.,0.951056516295154,
1.,0.951056516295154,1.,0.951056516295154,1.,0.951056516295154,1.,0.951056516295154,
1.,0.951056516295154,1.,0.951056516295154,1.,0.951056516295154,1.,0.951056516295154,
1.,0.951056516295154,1.,0.951056516295154,1.,0.951056516295154,1.,0.951056516295154,
1.,0.951056516295154,1.,0.951056516295154,1.,0.951056516295154,1.,0.951056516295154,
1.,0.951056516295154,1.,0.951056516295154,1.,0.951056516295154,1.,0.951056516295154,
1.,0.951056516295154,1.,0.951056516295154,1.,0.951056516295154,1.,0.951056516295154,
1.,0.951056516295154,1.,0.951056516295154,1.,0.951056516295154,1.,0.951056516295154,
1.,0.951056516295154,1.,0.951056516295154,1.,0.951056516295154,1.,0.951056516295154,
1.,0.951056516295154,1.,0.951056516295154,1.,0.951056516295154,1.,0.951056516295154,
1.,0.951056516295154,1.,0.951056516295154,1.,0.951056516295154,1.,0.951056516295154,
1.,0.951056516295154,1.,0.951056516295154,1.,0.951056516295154,1.,0.951056516295154,
1.,0.951056516295154,1.,0.951056516295154,1.,0.951056516295154,1.,0.951056516295154,
1.,0.951056516295154,1.,0.951056516295154,1.,0.951056516295154,1.,0.951056516295154,
1.,0.951056516295154,1.,0.951056516295154,1.,0.951056516295154,1.,0.951056516295154,
1.,0.951056516295154,1.,0.951056516295154,1.,0.951056516295154,1.,0.951056516295154,
1.,0.951056516295154,1.,0.951056516295154,1.,0.951056516295154,1.,0.951056516295154,
1.,0.951056516295154,1.,0.951056516295154,1.,0.951056516295154,1.,0.951056516295154,
1.,0.951056516295154,1.,0.951056516295154,1.,0.951056516295154,1.,0.951056516295154,
1.,0.951056516295154,1.,0.951056516295154,1.,0.951056516295154,1.,0.951056516295154,
1.,0.951056516295154,1.,0.951056516295154,1.,0.951056516295154,1.,0.951056516295154,
1.,0.951056516295154,1.,0.951056516295154,1.,0.951056516295154,1.,0.951056516295154,
1.,0.951056516295154,1.,0.951056516295154,1.,0.951056516295154,1.,0.951056516295154,
1.,0.951056516295154,1.,0.951056516295154,1.,0.951056516295154,1.,0.951056516295154,
1.,0.951056516295154,1.,0.951056516295154,1.,0.951056516295154,1.,0.951056516295154,
1.,0.951056516295154,1.,0.951056516295154,1.,0.951056516295154,1.,0.951056516295154,
1.,0.951056516295154,1.,0.951056516295154,1.,0.951056516295154,1.,0.951056516295154,
1.,0.951056516295154,1.,0.951056516295154,1.,0.951056516295154,1.,0.951056516295154,
1.,0.951056516295154,1.,0.951056516295154,1.,0.951056516295154,1.,0.951056516295154,
1.,0.951056516295154,1.,0.951056516295154,1.,0.951056516295154,1.,0.951056516295154,
1.,0.951056516295154,1.,0.951056516295154,1.,0.951056516295154,1.,0.951056516295154,
1.,0.951056516295154,1.,0.951056516295154,1.,0.951056516295154,1.,0.951056516295154,
1.,0.951056516295154,1.,0.951056516295154,1.,0.951056516295154,1.,0.951056516295154,
1.,0.951056516295154,1.,0.951056516295154,1.,0.951056516295154,1.,0.951056516295154,
1.,0.951056516295154,1.,0.951056516295154,1.,0.951056516295154,1.,0.951056516295154,
1.,0.951056516295154,1.,0.951056516295154,1.,0.951056516295154,1.,0.951056516295154,
1.,0.951056516295154,1.,0.951056516295154,1.,0.951056516295154,1.,0.951056516295154,
1.,0.951056516295154,1.,0.951056516295154,1.,0.951056516295154,1.,0.951056516295154,
1.,0.951056516295154,1.,0.951056516295154,1.,0.951056516295154,1.,0.951056516295154,
1.,0.951056516295154,1.,0.951056516295154,1.,0.951056516295154,1.,0.951056516295154,
1.,0.951056516295154,1.,0.951056516295154,1.,0.951056516295154,1.,0.951056516295154,
1.,0.951056516295154,1.,0.951056516295154,1.,0.951056516295154,1.,0.951056516295154,
1.,0.951056516295154,1.,0.951056516295154,1.,0.951056516295154,1.,0.951056516295154,
1.,0.951056516295154,1.,0.951056516295154,1.,0.951056516295154,1.,0.951056516295154,
1.,0.951056516295154,1.,0.951056516295154,1.,0.951056516295154,1.,0.951056516295154,
1.,0.951056516295154,1.,0.951056516295154,1.,0.951056516295154,1.,0.951056516295154,
1.,0.951056516295154,1.,0.951056516295154,1.,0.951056516295154,1.,0.951056516295154,
1.,0.951056516295154,1.,0.951056516295154,1.,0.951056516295154,1.,0.951056516295154,
1.,0.951056516295154,1.,0.951056516295154,1.,0.951056516295154,1.,0.951056516295154,
1.,0.951056516295154,1.,0.951056516295154,1.,0.951056516295154,1.,0.951056516295154,
1.,0.951056516295154,1.,0.951056516295154,1.,0.951056516295154,1.,0.951056516295154,
1.,0.951056516295154,1.,0.951056516295154,1.,0.951056516295154,1.,0.951056516295154,
1.,0.951056516295154,1.,0.951056516295154,1.,0.951056516295154,1.,0.951056516295154,
1.,0.951056516295154,1.,0.951056516295154,1.,0.951056516295154,1.,0.951056516295154,
1.,0.951056516295154,1.,0.951056516295154,1.,0.951056516295154,1.,0.951056516295154,
1.,0.951056516295154,1.,0.951056516295154,1.,0.951056516295154,1.,0.951056516295154,
1.,0.951056516295154,1.,0.951056516295154,1.,0.951056516295154,1.,0.951056516295154,
1.,0.951056516295154,1.,0.951056516295154,1.,0.951056516295154,1.,0.951056516295154,
1.,0.951056516295154,1.,0.951056516295154,1.,0.951056516295154,1.,0.951056516295154,
1.,0.951056516295154,1.,0.951056516295154,1.,0.951056516295154,1.,0.951056516295154,
1.,0.951056516295154,1.,0.951056516295154,1.,0.951056516295154,1.,0.951056516295154,
1.,0.951056516295154,1.,0.951056516295154,1.,0.951056516295154,1.,0.951056516295154,
1.,0.951056516295154,1.,0.951056516295154,1.,0.951056516295154,1.,0.951056516295154,
1.,0.951056516295154,1.,0.951056516295154,1.,0.951056516295154,1.,0.951056516295154,
1.,0.951056516295154,1.,0.951056516295154,1.,0.951056516295154,1.,0.951056516295154,
1.,0.951056516295154,1.,0.951056516295154,1.,0.951056516295154,1.,0.951056516295154,
1.,0.951056516295154,1.,0.951056516295154,1.,0.951056516295154,1.,0.951056516295154,
1.,0.951056516295154,1.,0.951056516295154,1.,0.951056516295154,1.,0.951056516295154,
1.,0.951056516295154,1.,0.951056516295154,1.,0.951056516295154,1.,0.951056516295154,
1.,0.951056516295154,1.,0.951056516295154,1.,0.951056516295154,1.)))
REPRESENTATION_ITEM('')
SURFACE()
);
#4124=TOROIDAL_SURFACE('',#104514,44.9676630434783,0.396875);
#4125=TOROIDAL_SURFACE('',#104518,17.2301371659243,0.396875);
#4126=TOROIDAL_SURFACE('',#104524,43.9357880434783,0.635000000000001);
#6666=B_SPLINE_CURVE_WITH_KNOTS('',3,(#275737,#275738,#275739,#275740,#275741,
#275742,#275743,#275744),.UNSPECIFIED.,.F.,.F.,(4,2,2,4),(1.00000116132204E-6,
0.429497510617222,1.0120430239264,1.11775283487271),.UNSPECIFIED.);
#6667=B_SPLINE_CURVE_WITH_KNOTS('',3,(#275749,#275750,#275751,#275752),
 .UNSPECIFIED.,.F.,.F.,(4,4),(7.34352906207753,7.64557688708348),
 .UNSPECIFIED.);
#6668=B_SPLINE_CURVE_WITH_KNOTS('',3,(#275753,#275754,#275755,#275756,#275757,
#275758,#275759,#275760,#275761,#275762),.UNSPECIFIED.,.F.,.F.,(4,2,2,2,
4),(9.99999987588035E-7,0.202811370610722,0.414120939581438,0.71227877903909,
0.886181891443318),.UNSPECIFIED.);
#6669=B_SPLINE_CURVE_WITH_KNOTS('',3,(#275769,#275770,#275771,#275772,#275773,
#275774,#275775,#275776),.UNSPECIFIED.,.F.,.F.,(4,2,2,4),(-42.6556224181082,
-42.3393783982178,-42.0192508568443,-41.8325669335184),.UNSPECIFIED.);
#6670=B_SPLINE_CURVE_WITH_KNOTS('',3,(#275782,#275783,#275784,#275785,#275786,
#275787,#275788,#275789,#275790,#275791,#275792,#275793,#275794,#275795,
#275796,#275797,#275798,#275799,#275800,#275801,#275802,#275803,#275804,
#275805,#275806,#275807,#275808,#275809,#275810,#275811,#275812,#275813,
#275814,#275815,#275816,#275817),.UNSPECIFIED.,.F.,.F.,(4,2,2,2,2,2,2,2,
2,2,2,2,2,2,2,2,2,4),(-7.44116305045028,-7.17785504943678,-6.70990825692069,
-6.23401157001746,-5.76981930737753,-5.29794385498397,-4.82877043864304,
-4.36346848183658,-3.88740222504434,-3.4220963637296,-2.95310502793577,
-2.47931294698886,-2.01512664441116,-1.54211434015112,-1.0743024235615,
-0.608146386189052,-0.304927951315456,-9.99999993922529E-7),
 .UNSPECIFIED.);
#6671=B_SPLINE_CURVE_WITH_KNOTS('',3,(#275819,#275820,#275821,#275822,#275823,
#275824,#275825,#275826,#275827,#275828,#275829,#275830,#275831,#275832,
#275833,#275834,#275835,#275836,#275837,#275838,#275839,#275840,#275841,
#275842,#275843,#275844,#275845,#275846,#275847,#275848,#275849,#275850,
#275851,#275852,#275853,#275854),.UNSPECIFIED.,.F.,.F.,(4,2,2,2,2,2,2,2,
2,2,2,2,2,2,2,2,2,4),(-41.8325669335184,-41.5544565596035,-41.0761168548913,
-40.6089639671417,-40.1417104354557,-39.6676250020063,-39.2030407552377,
-38.7303486447156,-38.2603417146062,-37.7952178460956,-37.3180877048775,
-36.8519799622467,-36.3835773668435,-35.9106696866344,-35.4462857267773,
-34.9716819551014,-34.5027722391319,-34.2597187473986),.UNSPECIFIED.);
#6672=B_SPLINE_CURVE_WITH_KNOTS('',3,(#275859,#275860,#275861,#275862,#275863,
#275864,#275865,#275866,#275867,#275868,#275869,#275870,#275871,#275872,
#275873,#275874,#275875,#275876,#275877,#275878,#275879,#275880,#275881,
#275882,#275883,#275884,#275885,#275886,#275887,#275888,#275889,#275890,
#275891,#275892,#275893,#275894),.UNSPECIFIED.,.F.,.F.,(4,2,2,2,2,2,2,2,
2,2,2,2,2,2,2,2,2,4),(-15.0095788972105,-14.6891053876878,-14.2233099603447,
-13.7464994065718,-13.2816878142172,-12.8119957222621,-12.33962154027,-11.8753488433553,
-11.4015809522423,-10.9346413573587,-10.4678013743225,-9.98978205441938,
-9.52529968492163,-9.05446969804222,-8.58368061459515,-8.11893603960459,
-7.64396665170116,-7.44116305045028),.UNSPECIFIED.);
#6673=B_SPLINE_CURVE_WITH_KNOTS('',3,(#275895,#275896,#275897,#275898,#275899,
#275900,#275901,#275902,#275903,#275904,#275905,#275906,#275907,#275908,
#275909,#275910,#275911,#275912,#275913,#275914,#275915,#275916,#275917,
#275918,#275919,#275920,#275921,#275922,#275923,#275924,#275925,#275926,
#275927,#275928,#275929,#275930),.UNSPECIFIED.,.F.,.F.,(4,2,2,2,2,2,2,2,
2,2,2,2,2,2,2,2,2,4),(-34.2597187473986,-34.0370343829147,-33.5610627724172,
-33.0957264046361,-32.6258819919018,-32.1540895486335,-31.6896159949956,
-31.2128397783498,-30.7449484402703,-30.2783319795283,-29.8034272201055,
-29.338560671758,-28.8670395861306,-28.3962594537798,-27.9314186621211,
-27.4534667216445,-26.986674673592,-26.6867050296319),.UNSPECIFIED.);
#6674=B_SPLINE_CURVE_WITH_KNOTS('',3,(#275935,#275936,#275937,#275938,#275939,
#275940,#275941,#275942,#275943,#275944,#275945,#275946,#275947,#275948,
#275949,#275950,#275951,#275952,#275953,#275954,#275955,#275956,#275957,
#275958,#275959,#275960,#275961,#275962,#275963,#275964,#275965,#275966,
#275967,#275968,#275969,#275970),.UNSPECIFIED.,.F.,.F.,(4,2,2,2,2,2,2,2,
2,2,2,2,2,2,2,2,2,4),(-22.5771816796688,-22.1974829039796,-21.7329281055567,
-21.2583415224104,-20.792038573969,-20.3244607251778,-19.8480054086097,
-19.3838435875952,-18.9123672043351,-18.4428387263217,-17.9778142873194,
-17.502161518784,-17.0367364757151,-16.5681408884267,-16.0938564613078,
-15.6297840447666,-15.1571931357626,-15.0095788972105),.UNSPECIFIED.);
#6675=B_SPLINE_CURVE_WITH_KNOTS('',3,(#275971,#275972,#275973,#275974,#275975,
#275976,#275977,#275978,#275979,#275980,#275981,#275982,#275983,#275984,
#275985,#275986,#275987,#275988,#275989,#275990,#275991,#275992,#275993,
#275994,#275995,#275996,#275997,#275998,#275999,#276000,#276001,#276002,
#276003,#276004,#276005,#276006),.UNSPECIFIED.,.F.,.F.,(4,2,2,2,2,2,2,2,
2,2,2,2,2,2,2,2,2,4),(-26.6867050296319,-26.5191327937425,-26.0454265438289,
-25.5809543455129,-25.1077448664485,-24.6380946277012,-24.1728388918026,
-23.6960853050495,-23.2302611865729,-22.7658976619046,-22.2929524044554,
-21.8246432184248,-21.3585099790374,-20.8813404908684,-20.4162654100928,
-19.9462223577016,-19.4736481649645,-19.1145570626869),.UNSPECIFIED.);
#6676=B_SPLINE_CURVE_WITH_KNOTS('',3,(#276011,#276012,#276013,#276014,#276015,
#276016,#276017,#276018,#276019,#276020,#276021,#276022,#276023,#276024,
#276025,#276026,#276027,#276028,#276029,#276030,#276031,#276032,#276033,
#276034,#276035,#276036,#276037,#276038,#276039,#276040,#276041,#276042,
#276043,#276044,#276045,#276046),.UNSPECIFIED.,.F.,.F.,(4,2,2,2,2,2,2,2,
2,2,2,2,2,2,2,2,2,4),(-30.1445044786768,-29.7083751129182,-29.2402785855838,
-28.7677009365716,-28.3036318874976,-27.8293319784653,-27.3607488282678,
-26.8953199234704,-26.4196801308044,-25.9546641419191,-25.4851244920146,
-25.0136606183757,-24.5494995786249,-24.0730268352487,-23.6054605373483,
-23.1391515381628,-22.6686868414385,-22.5771816796688),.UNSPECIFIED.);
#6677=B_SPLINE_CURVE_WITH_KNOTS('',3,(#276047,#276048,#276049,#276050,#276051,
#276052,#276053,#276054,#276055,#276056,#276057,#276058,#276059,#276060,
#276061,#276062,#276063,#276064,#276065,#276066,#276067,#276068,#276069,
#276070,#276071,#276072,#276073,#276074,#276075,#276076,#276077,#276078,
#276079,#276080,#276081,#276082),.UNSPECIFIED.,.F.,.F.,(4,2,2,2,2,2,2,2,
2,2,2,2,2,2,2,2,2,4),(-19.1145570626869,-19.009069084107,-18.5349439065439,
-18.0677669735219,-17.6006289446376,-17.1224651546171,-16.6579203640066,
-16.1869539705083,-15.7161685208132,-15.2513185292807,-14.7762090591503,
-14.3100610165697,-13.8419777248235,-13.3661095595253,-12.901840724189,
-12.4298228977916,-11.9606418459535,-11.5438063668984),.UNSPECIFIED.);
#6678=B_SPLINE_CURVE_WITH_KNOTS('',3,(#276088,#276089,#276090,#276091,#276092,
#276093,#276094,#276095,#276096,#276097,#276098,#276099,#276100,#276101,
#276102,#276103,#276104,#276105,#276106,#276107),.UNSPECIFIED.,.F.,.F.,
(4,2,2,2,2,2,2,2,2,4),(-3.97345641689582,-3.50426059056884,-3.03988191488275,
-2.56866935179826,-2.09844180121526,-1.63350787928118,-1.15813639803468,
-0.692307299664475,-0.343901369245436,-9.999999992516E-7),.UNSPECIFIED.);
#6679=B_SPLINE_CURVE_WITH_KNOTS('',3,(#276110,#276111,#276112,#276113,#276114,
#276115,#276116,#276117,#276118,#276119,#276120,#276121,#276122,#276123,
#276124,#276125,#276126,#276127,#276128,#276129,#276130,#276131,#276132,
#276133),.UNSPECIFIED.,.F.,.F.,(4,2,2,2,2,2,2,2,2,2,2,4),(-42.6297087861989,
-42.2733922661027,-41.918043823783,-41.4442399042521,-40.975262620631,-40.5099558642212,
-40.0339042317455,-39.5686130984597,-39.0994318314099,-38.6275705716374,
-38.1633818297147,-37.7128902237401),.UNSPECIFIED.);
#6680=B_SPLINE_CURVE_WITH_KNOTS('',3,(#276135,#276136,#276137,#276138,#276139,
#276140,#276141,#276142,#276143,#276144,#276145,#276146,#276147,#276148,
#276149,#276150,#276151,#276152,#276153,#276154,#276155,#276156,#276157,
#276158,#276159,#276160,#276161,#276162,#276163,#276164,#276165,#276166,
#276167,#276168,#276169,#276170,#276171,#276172),.UNSPECIFIED.,.F.,.F.,
(4,2,2,2,2,2,2,2,2,2,2,2,2,2,2,2,2,2,4),(-37.7128902237401,-37.6874712538429,
-37.2195376691207,-36.7534229318995,-36.2784672722019,-35.8137309018735,
-35.3429320891482,-34.8721153061919,-34.4076341220623,-33.9296287163475,
-33.4628020605409,-32.9958564735305,-32.5221022327873,-32.0578354653717,
-31.5854484593393,-31.1157693469819,-30.6509563925439,-30.1741594603652,
-30.1445044786768),.UNSPECIFIED.);
#6681=B_SPLINE_CURVE_WITH_KNOTS('',3,(#276173,#276174,#276175,#276176,#276177,
#276178,#276179,#276180,#276181,#276182,#276183,#276184,#276185,#276186,
#276187,#276188,#276189,#276190,#276191,#276192,#276193,#276194,#276195,
#276196,#276197,#276198,#276199,#276200,#276201,#276202,#276203,#276204,
#276205,#276206,#276207,#276208,#276209,#276210),.UNSPECIFIED.,.F.,.F.,
(4,2,2,2,2,2,2,2,2,2,2,2,2,2,2,2,2,2,4),(-11.5438063668984,-11.4952185482997,
-11.0190068049884,-10.5536512371283,-10.0845187618387,-9.61074282219137,
-9.1464648778113,-8.67330637301754,-8.2054723003753,-7.73918014733004,-7.26178842260406,
-6.79695068115107,-6.32670321892208,-5.85473342556063,-5.39015939398363,
-4.91581118919752,-4.44901839880879,-3.98166664151097,-3.97345641689582),
 .UNSPECIFIED.);
#6682=B_SPLINE_CURVE_WITH_KNOTS('',3,(#276212,#276213,#276214,#276215,#276216,
#276217,#276218,#276219),.UNSPECIFIED.,.F.,.F.,(4,2,2,4),(0.886181891443318,
1.00363319154204,1.25505529473825,1.52001564473151),.UNSPECIFIED.);
#6683=B_SPLINE_CURVE_WITH_KNOTS('',3,(#276223,#276224,#276225,#276226,#276227,
#276228,#276229,#276230,#276231,#276232,#276233,#276234,#276235,#276236,
#276237,#276238,#276239,#276240,#276241,#276242,#276243,#276244,#276245,
#276246,#276247,#276248,#276249,#276250,#276251,#276252,#276253,#276254,
#276255,#276256,#276257,#276258,#276259,#276260),.UNSPECIFIED.,.F.,.F.,
(4,2,2,2,2,2,2,2,2,2,2,2,2,2,2,2,2,2,4),(1.00000002956069E-6,0.376972969184724,
0.75799918633037,1.21242033240789,1.43740179078372,1.88669535644621,2.30937841181643,
2.68597888099499,3.12649045709018,3.62482966496969,4.11196706709142,4.60170487876917,
4.84231053032182,5.29690378277065,5.76750323625794,6.27455902097634,6.7799859159262,
7.21138329694587,7.34352906207753),.UNSPECIFIED.);
#6684=B_SPLINE_CURVE_WITH_KNOTS('',3,(#276262,#276263,#276264,#276265,#276266,
#276267,#276268,#276269,#276270,#276271),.UNSPECIFIED.,.F.,.F.,(4,2,2,2,
4),(1.11775283487271,1.3201344337092,1.98402684478003,2.41673859827204,
2.92708277165291),.UNSPECIFIED.);
#6685=B_SPLINE_CURVE_WITH_KNOTS('',3,(#276273,#276274,#276275,#276276),
 .UNSPECIFIED.,.F.,.F.,(4,4),(9.99999986243288E-7,0.188629584531221),
 .UNSPECIFIED.);
#6686=B_SPLINE_CURVE_WITH_KNOTS('',3,(#276280,#276281,#276282,#276283,#276284,
#276285,#276286,#276287,#276288,#276289,#276290,#276291,#276292,#276293,
#276294,#276295,#276296,#276297,#276298,#276299,#276300,#276301,#276302,
#276303,#276304,#276305,#276306,#276307,#276308,#276309,#276310,#276311,
#276312,#276313,#276314,#276315,#276316,#276317),.UNSPECIFIED.,.F.,.F.,
(4,2,2,2,2,2,2,2,2,2,2,2,2,2,2,2,2,2,4),(0.188629584531221,0.394123083444476,
0.775094908203116,1.00161149469956,1.45530454079207,1.88145272689184,2.26155886735503,
2.69362881864141,3.16125461205091,3.61936691473805,4.07995327375831,4.56161966164196,
5.04003114519772,5.5043665714204,5.92302774285437,6.13173895340881,6.53854095434356,
6.91901551588997,7.29112327722061),.UNSPECIFIED.);
#6687=B_SPLINE_CURVE_WITH_KNOTS('',3,(#280873,#280874,#280875,#280876,#280877,
#280878,#280879,#280880),.UNSPECIFIED.,.F.,.F.,(4,2,2,4),(-46.6217887874376,
-46.2578454585251,-45.8892323703203,-45.6738876706438),.UNSPECIFIED.);
#6688=B_SPLINE_CURVE_WITH_KNOTS('',3,(#280885,#280886,#280887,#280888,#280889,
#280890,#280891,#280892,#280893,#280894,#280895,#280896,#280897,#280898,
#280899,#280900,#280901,#280902,#280903,#280904,#280905,#280906,#280907,
#280908,#280909,#280910,#280911,#280912,#280913,#280914,#280915,#280916,
#280917,#280918,#280919,#280920),.UNSPECIFIED.,.F.,.F.,(4,2,2,2,2,2,2,2,
2,2,2,2,2,2,2,2,2,4),(-7.56876057602163,-7.35729635649663,-6.88731803123374,
-6.41494627125509,-5.95046718064394,-5.47640437326289,-5.00939178691373,
-4.54231615347622,-4.06438205582116,-3.59996445059252,-3.12905565079213,
-2.658464871178,-2.19369990895879,-1.71864614164823,-1.25265148999412,-0.784624653178984,
-0.392650910730672,-1.00000001790335E-6),.UNSPECIFIED.);
#6689=B_SPLINE_CURVE_WITH_KNOTS('',3,(#280921,#280922,#280923,#280924,#280925,
#280926,#280927,#280928,#280929,#280930,#280931,#280932,#280933,#280934,
#280935,#280936,#280937,#280938,#280939,#280940,#280941,#280942,#280943,
#280944,#280945,#280946,#280947,#280948,#280949,#280950,#280951,#280952,
#280953,#280954,#280955,#280956),.UNSPECIFIED.,.F.,.F.,(4,2,2,2,2,2,2,2,
2,2,2,2,2,2,2,2,2,4),(-45.6738876706438,-45.4241622385571,-44.9471446938412,
-44.4811383037189,-44.0127611847923,-43.539964174791,-43.0756517655993,
-42.6010485658741,-42.132245850907,-41.6665520052273,-41.1906903497208,
-40.7254451393306,-40.2556172366779,-39.7839324263573,-39.3195205227013,
-38.8427377357185,-38.3749498540981,-38.1024403174797),.UNSPECIFIED.);
#6690=B_SPLINE_CURVE_WITH_KNOTS('',3,(#280961,#280962,#280963,#280964,#280965,
#280966,#280967,#280968,#280969,#280970,#280971,#280972,#280973,#280974,
#280975,#280976,#280977,#280978,#280979,#280980,#280981,#280982,#280983,
#280984,#280985,#280986,#280987,#280988,#280989,#280990,#280991,#280992,
#280993,#280994,#280995,#280996),.UNSPECIFIED.,.F.,.F.,(4,2,2,2,2,2,2,2,
2,2,2,2,2,2,2,2,2,4),(-15.1390134568254,-14.8703711811418,-14.4025233596478,
-13.9261219694299,-13.4618117547277,-12.9900535016762,-12.5205100985779,
-12.0552503764082,-11.5793093004391,-11.1137879339429,-10.6449122869091,
-10.1706599895591,-9.70640996906313,-9.23352862264522,-8.76539906730381,
-8.29933862556263,-7.82223236481082,-7.56876057602163),.UNSPECIFIED.);
#6691=B_SPLINE_CURVE_WITH_KNOTS('',3,(#280997,#280998,#280999,#281000,#281001,
#281002,#281003,#281004,#281005,#281006,#281007,#281008,#281009,#281010,
#281011,#281012,#281013,#281014,#281015,#281016,#281017,#281018,#281019,
#281020,#281021,#281022,#281023,#281024,#281025,#281026,#281027,#281028,
#281029,#281030,#281031,#281032),.UNSPECIFIED.,.F.,.F.,(4,2,2,2,2,2,2,2,
2,2,2,2,2,2,2,2,2,4),(-38.1024403174797,-37.908369141637,-37.4335703060707,
-36.9687843751113,-36.4972733014153,-36.0265964184819,-35.5618083565122,
-35.0839631626955,-34.6172720333329,-34.1497547127705,-33.6761535978443,
-33.2117526390136,-32.7385416715103,-32.2689933140818,-31.8037803554565,
-31.3271318265374,-30.8613991691482,-30.5307647496651),.UNSPECIFIED.);
#6692=B_SPLINE_CURVE_WITH_KNOTS('',3,(#281037,#281038,#281039,#281040,#281041,
#281042,#281043,#281044,#281045,#281046,#281047,#281048,#281049,#281050,
#281051,#281052,#281053,#281054,#281055,#281056,#281057,#281058,#281059,
#281060,#281061,#281062,#281063,#281064,#281065,#281066,#281067,#281068,
#281069,#281070,#281071,#281072),.UNSPECIFIED.,.F.,.F.,(4,2,2,2,2,2,2,2,
2,2,2,2,2,2,2,2,2,4),(-22.7092124132459,-22.382818915422,-21.9170703529098,
-21.4403616643235,-20.9753261216896,-20.5057249837587,-20.0328733432699,
-19.5685359670655,-19.0948722977256,-18.627606354345,-18.1608627726006,
-17.6829518794475,-17.2183013266551,-16.7475673180964,-16.2763682436002,
-15.8116091528861,-15.3367457660718,-15.1390134568254),.UNSPECIFIED.);
#6693=B_SPLINE_CURVE_WITH_KNOTS('',3,(#281073,#281074,#281075,#281076,#281077,
#281078,#281079,#281080,#281081,#281082,#281083,#281084,#281085,#281086,
#281087,#281088,#281089,#281090,#281091,#281092,#281093,#281094,#281095,
#281096,#281097,#281098,#281099,#281100,#281101,#281102,#281103,#281104,
#281105,#281106,#281107,#281108),.UNSPECIFIED.,.F.,.F.,(4,2,2,2,2,2,2,2,
2,2,2,2,2,2,2,2,2,4),(-30.5307647496651,-30.3926305138291,-29.9201905225812,
-29.4558935047261,-28.9806754193057,-28.5122020231605,-28.0462831131032,
-27.5707668457713,-27.105706206466,-26.6411884352463,-26.1670855034839,
-25.7000350708087,-25.2329199200806,-24.7549480979426,-24.2904922625418,
-23.819543534539,-23.3489150935619,-22.9601719025343),.UNSPECIFIED.);
#6694=B_SPLINE_CURVE_WITH_KNOTS('',3,(#281113,#281114,#281115,#281116,#281117,
#281118,#281119,#281120,#281121,#281122,#281123,#281124,#281125,#281126,
#281127,#281128,#281129,#281130,#281131,#281132,#281133,#281134,#281135,
#281136,#281137,#281138,#281139,#281140,#281141,#281142,#281143,#281144,
#281145,#281146,#281147,#281148),.UNSPECIFIED.,.F.,.F.,(4,2,2,2,2,2,2,2,
2,2,2,2,2,2,2,2,2,4),(-30.27910381554,-29.8960477742315,-29.4249957993259,
-28.954161031348,-28.4895402681035,-28.0115217593285,-27.5446786938516,
-27.0775194213598,-26.6037507201956,-26.1393927796599,-25.6667207227057,
-25.1970215589772,-24.73131825619,-24.2628015575025,-23.7879822109015,-23.3237890760973,
-22.8512936595655,-22.7092124132459),.UNSPECIFIED.);
#6695=B_SPLINE_CURVE_WITH_KNOTS('',3,(#281149,#281150,#281151,#281152,#281153,
#281154,#281155,#281156,#281157,#281158,#281159,#281160,#281161,#281162,
#281163,#281164,#281165,#281166,#281167,#281168,#281169,#281170,#281171,
#281172,#281173,#281174,#281175,#281176,#281177,#281178,#281179,#281180,
#281181,#281182,#281183,#281184),.UNSPECIFIED.,.F.,.F.,(4,2,2,2,2,2,2,2,
2,2,2,2,2,2,2,2,2,4),(-22.9601719025343,-22.8841111809573,-22.4090170950461,
-21.9429845050713,-21.4749179720702,-20.9992332900195,-20.5350391956014,
-20.0630335999792,-19.5939976673447,-19.128604847174,-18.65240363536,-18.187149951532,
-17.718030056841,-17.24442435561,-16.7802061331413,-16.3070565274049,-15.8393525332099,
-15.3912550272859),.UNSPECIFIED.);
#6696=B_SPLINE_CURVE_WITH_KNOTS('',3,(#281189,#281190,#281191,#281192,#281193,
#281194,#281195,#281196,#281197,#281198,#281199,#281200,#281201,#281202,
#281203,#281204,#281205,#281206,#281207,#281208,#281209,#281210,#281211,
#281212,#281213,#281214,#281215,#281216,#281217,#281218,#281219,#281220,
#281221,#281222,#281223,#281224),.UNSPECIFIED.,.F.,.F.,(4,2,2,2,2,2,2,2,
2,2,2,2,2,2,2,2,2,4),(-37.8493859968929,-37.4070914074001,-36.9390646224457,
-36.466064763649,-36.0017935798579,-35.5277130470903,-35.058726900269,-34.5932584637534,
-34.1172014784137,-33.6518686415785,-33.1824532454847,-32.71058352461,-32.2462786662642,
-31.7700701952743,-31.3021203457283,-30.8358216690874,-30.3608520954614,
-30.27910381554),.UNSPECIFIED.);
#6697=B_SPLINE_CURVE_WITH_KNOTS('',3,(#281225,#281226,#281227,#281228,#281229,
#281230,#281231,#281232,#281233,#281234,#281235,#281236,#281237,#281238,
#281239,#281240,#281241,#281242,#281243,#281244,#281245,#281246,#281247,
#281248,#281249,#281250,#281251,#281252,#281253,#281254,#281255,#281256,
#281257,#281258,#281259,#281260,#281261,#281262),.UNSPECIFIED.,.F.,.F.,
(4,2,2,2,2,2,2,2,2,2,2,2,2,2,2,2,2,2,4),(-15.3912550272859,-15.3730765213189,
-14.8956926027671,-14.4309419924448,-13.9607049000054,-13.4888885828601,
-13.0243600322952,-12.5500194056437,-12.0833400442585,-11.6159969274629,
-11.1387717209122,-10.6744669851398,-10.2032577033738,-9.73317433233838,
-9.26826994282085,-8.79289947084361,-8.32717155512522,-7.85884267836123,
-7.82217132368041),.UNSPECIFIED.);
#6698=B_SPLINE_CURVE_WITH_KNOTS('',3,(#281268,#281269,#281270,#281271),
 .UNSPECIFIED.,.F.,.F.,(4,4),(-0.254027045710766,-1.00000002078993E-6),
 .UNSPECIFIED.);
#6699=B_SPLINE_CURVE_WITH_KNOTS('',3,(#281274,#281275,#281276,#281277,#281278,
#281279,#281280,#281281),.UNSPECIFIED.,.F.,.F.,(4,2,2,4),(-46.6160574698286,
-46.238612042811,-45.8638054928735,-45.419398246854),.UNSPECIFIED.);
#6700=B_SPLINE_CURVE_WITH_KNOTS('',3,(#281283,#281284,#281285,#281286,#281287,
#281288,#281289,#281290,#281291,#281292,#281293,#281294,#281295,#281296,
#281297,#281298,#281299,#281300,#281301,#281302,#281303,#281304,#281305,
#281306,#281307,#281308,#281309,#281310,#281311,#281312,#281313,#281314,
#281315,#281316,#281317,#281318,#281319,#281320),.UNSPECIFIED.,.F.,.F.,
(4,2,2,2,2,2,2,2,2,2,2,2,2,2,2,2,2,2,4),(-45.419398246854,-45.388335458859,
-44.9201788529334,-44.4542375100199,-43.9790489160334,-43.5142083505892,
-43.0437468660947,-42.5727088239309,-42.1082957172573,-41.6305539035994,
-41.1633599487675,-40.6964212557151,-40.2222364592212,-39.7577103098546,
-39.2854822068615,-38.8153883474286,-38.3504794784601,-37.8732513328493,
-37.8493859968929),.UNSPECIFIED.);
#6701=B_SPLINE_CURVE_WITH_KNOTS('',3,(#281321,#281322,#281323,#281324,#281325,
#281326,#281327,#281328,#281329,#281330,#281331,#281332,#281333,#281334,
#281335,#281336,#281337,#281338,#281339,#281340,#281341,#281342,#281343,
#281344,#281345,#281346,#281347,#281348,#281349,#281350,#281351,#281352,
#281353,#281354,#281355,#281356),.UNSPECIFIED.,.F.,.F.,(4,2,2,2,2,2,2,2,
2,2,2,2,2,2,2,2,2,4),(-7.82217132368041,-7.38385187621001,-6.91972506820527,
-6.44742865870557,-5.97886619559227,-5.51328243212834,-5.03677797532993,
-4.57174887967328,-4.10234361258054,-3.62935221798109,-3.16511416248466,
-2.69165565360192,-2.22433643981363,-1.75778780089319,-1.28008600548505,
-0.815474412442063,-0.405490990239572,-0.254027045710766),.UNSPECIFIED.);
#6702=B_SPLINE_CURVE_WITH_KNOTS('',3,(#281409,#281410,#281411,#281412,#281413,
#281414,#281415,#281416,#281417,#281418,#281419,#281420),.UNSPECIFIED.,
 .F.,.F.,(4,2,2,2,2,4),(9.99999999029508E-7,0.392467864625591,0.772803552303566,
1.20676402389129,1.59513819877189,1.97927314617369),.UNSPECIFIED.);
#6703=B_SPLINE_CURVE_WITH_KNOTS('',3,(#281424,#281425,#281426,#281427,#281428,
#281429,#281430,#281431,#281432,#281433,#281434,#281435,#281436,#281437,
#281438,#281439,#281440,#281441,#281442,#281443,#281444,#281445,#281446,
#281447,#281448,#281449,#281450,#281451,#281452,#281453),.UNSPECIFIED.,
 .F.,.F.,(4,2,2,2,2,2,2,2,2,2,2,2,2,2,4),(1.97927314617369,2.02730718991295,
2.48197895053455,2.92990213883089,3.38495238463682,3.85815130246585,4.33242573779402,
4.79625192402839,5.21479621725514,5.42409530491494,5.83033362431084,6.24041628338956,
6.44209040988607,6.81263411618772,7.17194255907665),.UNSPECIFIED.);
#6704=B_SPLINE_CURVE_WITH_KNOTS('',3,(#281454,#281455,#281456,#281457,#281458,
#281459,#281460,#281461,#281462,#281463,#281464,#281465,#281466,#281467),
 .UNSPECIFIED.,.F.,.F.,(4,2,2,2,2,2,4),(0.,0.303989670039342,0.666040902826767,
1.36264560499374,2.25979709302026,2.777868489948,3.29723672060596),
 .UNSPECIFIED.);
#6705=B_SPLINE_CURVE_WITH_KNOTS('',3,(#281483,#281484,#281485,#281486,#281487,
#281488,#281489,#281490,#281491,#281492,#281493,#281494,#281495,#281496,
#281497,#281498),.UNSPECIFIED.,.F.,.F.,(4,2,2,2,2,2,2,4),(0.,0.238087952519387,
0.476113544168717,1.01011910515244,1.73799046632944,2.30408220983986,2.86072831234553,
3.43288601470779),.UNSPECIFIED.);
#6706=B_SPLINE_CURVE_WITH_KNOTS('',3,(#281499,#281500,#281501,#281502,#281503,
#281504,#281505,#281506,#281507,#281508,#281509,#281510,#281511,#281512,
#281513,#281514),.UNSPECIFIED.,.F.,.F.,(4,2,2,2,2,2,2,4),(1.00000044233709E-6,
0.539370132359783,1.28481747817566,1.98442658665292,2.48325218307673,2.95253551271824,
3.30333512017195,3.64287608445345),.UNSPECIFIED.);
#6707=B_SPLINE_CURVE_WITH_KNOTS('',3,(#285740,#285741,#285742,#285743,#285744,
#285745,#285746,#285747,#285748,#285749,#285750,#285751,#285752,#285753,
#285754,#285755,#285756,#285757,#285758,#285759,#285760,#285761,#285762,
#285763),.UNSPECIFIED.,.F.,.F.,(4,2,2,2,2,2,2,2,2,2,2,4),(1.00000001673761E-6,
0.323039742323442,0.634605365470257,1.07005687139309,1.45978725204872,1.89383348337783,
2.35103053579564,2.80133004158489,3.25887862097597,3.72872917648254,4.27536018155541,
4.56129717631177),.UNSPECIFIED.);
#6708=B_SPLINE_CURVE_WITH_KNOTS('',3,(#285767,#285768,#285769,#285770,#285771,
#285772,#285773,#285774,#285775,#285776,#285777,#285778,#285779,#285780,
#285781,#285782,#285783,#285784,#285785,#285786),.UNSPECIFIED.,.F.,.F.,
(4,2,2,2,2,2,2,2,2,4),(4.56129717631177,4.78025138948249,5.24019813332798,
5.47080497646155,5.91680419253928,6.36814416866029,6.58957679463825,7.00642309193714,
7.22277354918002,7.44333948969208),.UNSPECIFIED.);
#6709=B_SPLINE_CURVE_WITH_KNOTS('',3,(#285788,#285789,#285790,#285791,#285792,
#285793,#285794,#285795,#285796,#285797,#285798,#285799),.UNSPECIFIED.,
 .F.,.F.,(4,2,2,2,2,4),(-3.21369901094688,-2.40395999881897,-1.62924044691679,
-0.911220628324192,-0.414117520413494,0.),.UNSPECIFIED.);
#6710=B_SPLINE_CURVE_WITH_KNOTS('',3,(#285814,#285815,#285816,#285817,#285818,
#285819,#285820,#285821,#285822,#285823,#285824,#285825,#285826,#285827),
 .UNSPECIFIED.,.F.,.F.,(4,2,2,2,2,2,4),(-2.64506467679378,-2.30500727703039,
-1.84084072046588,-1.36787613459182,-0.900047765262215,-0.450187418519317,
-9.99999997031153E-7),.UNSPECIFIED.);
#6711=B_SPLINE_CURVE_WITH_KNOTS('',3,(#287914,#287915,#287916,#287917,#287918,
#287919,#287920,#287921,#287922,#287923,#287924,#287925,#287926,#287927,
#287928,#287929,#287930,#287931),.UNSPECIFIED.,.F.,.F.,(4,2,2,2,2,2,2,2,
4),(0.,0.226844249939865,0.465043591920983,0.874045242019083,1.423867627709,
2.24701645815008,2.92758088609289,3.21943913627986,3.52521182016246),
 .UNSPECIFIED.);
#6712=B_SPLINE_CURVE_WITH_KNOTS('',3,(#290007,#290008,#290009,#290010,#290011,
#290012,#290013,#290014,#290015,#290016,#290017,#290018,#290019,#290020,
#290021,#290022),.UNSPECIFIED.,.F.,.F.,(4,2,2,2,2,2,2,4),(9.99999979533284E-7,
0.442518894276843,1.00228459757929,1.78979762641102,2.54504033256861,3.08734332574651,
3.32519808039208,3.56352063065413),.UNSPECIFIED.);
#6713=B_SPLINE_CURVE_WITH_KNOTS('',3,(#291512,#291513,#291514,#291515,#291516,
#291517,#291518,#291519),.UNSPECIFIED.,.F.,.F.,(4,2,2,4),(93.9993055949368,
94.3962462510942,94.7498463849653,95.1031006473574),.UNSPECIFIED.);
#6714=B_SPLINE_CURVE_WITH_KNOTS('',3,(#291522,#291523,#291524,#291525),
 .UNSPECIFIED.,.F.,.F.,(4,4),(1.00000001485023E-6,0.159782552535823),
 .UNSPECIFIED.);
#6715=B_SPLINE_CURVE_WITH_KNOTS('',3,(#291530,#291531,#291532,#291533,#291534,
#291535,#291536,#291537,#291538,#291539,#291540,#291541,#291542,#291543,
#291544,#291545,#291546,#291547,#291548,#291549,#291550,#291551,#291552,
#291553,#291554,#291555,#291556,#291557,#291558,#291559,#291560,#291561,
#291562,#291563,#291564,#291565),.UNSPECIFIED.,.F.,.F.,(4,2,2,2,2,2,2,2,
2,2,2,2,2,2,2,2,2,4),(86.4283032330504,86.8841446466063,87.3485119173072,
87.820329195308,88.289929201456,88.7552467982501,89.2312474538849,89.6968255999065,
90.1657599095305,90.6400689963987,91.1043763025996,91.5773168767035,92.0455030850787,
92.5116217372129,92.9887877759706,93.4537807497936,93.9238179812892,93.9993055949368),
 .UNSPECIFIED.);
#6716=B_SPLINE_CURVE_WITH_KNOTS('',3,(#291566,#291567,#291568,#291569,#291570,
#291571,#291572,#291573,#291574,#291575,#291576,#291577,#291578,#291579,
#291580,#291581,#291582,#291583,#291584,#291585,#291586,#291587,#291588,
#291589,#291590,#291591,#291592,#291593,#291594,#291595,#291596,#291597,
#291598,#291599,#291600,#291601,#291602,#291603),.UNSPECIFIED.,.F.,.F.,
(4,2,2,2,2,2,2,2,2,2,2,2,2,2,2,2,2,2,4),(0.159782552535823,0.252910728987131,
0.508836642406898,0.981847476572238,1.45142846116938,1.91654378355729,2.3932291166619,
2.85897304032226,3.32757846013873,3.80005253365681,4.26429331421471,4.7392892518596,
5.20778983727417,5.67358966710173,6.14913633685796,6.61418480437811,7.08429819311843,
7.55567986130047,7.72908631110027),.UNSPECIFIED.);
#6717=B_SPLINE_CURVE_WITH_KNOTS('',3,(#291608,#291609,#291610,#291611,#291612,
#291613,#291614,#291615,#291616,#291617,#291618,#291619,#291620,#291621,
#291622,#291623,#291624,#291625,#291626,#291627,#291628,#291629,#291630,
#291631,#291632,#291633,#291634,#291635,#291636,#291637,#291638,#291639,
#291640,#291641,#291642,#291643,#291644,#291645),.UNSPECIFIED.,.F.,.F.,
(4,2,2,2,2,2,2,2,2,2,2,2,2,2,2,2,2,2,4),(78.8571778264449,78.8922125296406,
79.3689807828779,79.8340730116635,80.3037327862311,80.7766409809457,81.2410356474547,
81.7147585162183,82.1820809757828,82.6488828483276,83.1268534867744,83.5915609200449,
84.0623537302704,84.5336094434342,84.99842609755,85.4733488429337,85.939780108239,
86.4076863886255,86.4283032330504),.UNSPECIFIED.);
#6718=B_SPLINE_CURVE_WITH_KNOTS('',3,(#291646,#291647,#291648,#291649,#291650,
#291651,#291652,#291653,#291654,#291655,#291656,#291657,#291658,#291659,
#291660,#291661,#291662,#291663,#291664,#291665,#291666,#291667,#291668,
#291669,#291670,#291671,#291672,#291673,#291674,#291675,#291676,#291677,
#291678,#291679,#291680,#291681),.UNSPECIFIED.,.F.,.F.,(4,2,2,2,2,2,2,2,
2,2,2,2,2,2,2,2,2,4),(7.72908631110027,8.02008352434038,8.49730419371805,
8.96481300151504,9.43155223815228,9.9060622753284,10.3707187452509,10.8425562258666,
11.3129584062321,11.7777947823367,12.2553490830901,12.7217834663287,13.1895307642473,
13.6628480915371,14.1271797316805,14.600790093664,15.0700725120836,15.3003047236943),
 .UNSPECIFIED.);
#6719=B_SPLINE_CURVE_WITH_KNOTS('',3,(#291686,#291687,#291688,#291689,#291690,
#291691,#291692,#291693,#291694,#291695,#291696,#291697,#291698,#291699,
#291700,#291701,#291702,#291703,#291704,#291705,#291706,#291707,#291708,
#291709,#291710,#291711,#291712,#291713,#291714,#291715,#291716,#291717,
#291718,#291719,#291720,#291721),.UNSPECIFIED.,.F.,.F.,(4,2,2,2,2,2,2,2,
2,2,2,2,2,2,2,2,2,4),(71.286676879443,71.3793362999404,71.853916807073,
72.3206016385598,72.7881784157484,73.265266886318,73.7296623484898,74.201118681301,
74.6711421432683,75.1362347817962,75.6118593900078,76.0776192284145,76.546194373815,
77.0210702754228,77.4853204386284,77.9578748686566,78.426406018764,78.8571778264449),
 .UNSPECIFIED.);
#6720=B_SPLINE_CURVE_WITH_KNOTS('',3,(#291722,#291723,#291724,#291725,#291726,
#291727,#291728,#291729,#291730,#291731,#291732,#291733,#291734,#291735,
#291736,#291737,#291738,#291739,#291740,#291741,#291742,#291743,#291744,
#291745,#291746,#291747,#291748,#291749,#291750,#291751,#291752,#291753,
#291754,#291755,#291756,#291757),.UNSPECIFIED.,.F.,.F.,(4,2,2,2,2,2,2,2,
2,2,2,2,2,2,2,2,2,4),(15.3003047236943,15.5353971469736,16.0117656400808,
16.4773020474794,16.9463663727299,17.4185359888615,17.8828282335684,18.3585046724596,
18.8267291967529,19.2928191356463,19.7680752712759,20.2330067249166,20.7036518752658,
21.1747588162273,21.6392983776734,22.1172539198714,22.5845205862061,22.8714706980816),
 .UNSPECIFIED.);
#6721=B_SPLINE_CURVE_WITH_KNOTS('',3,(#291762,#291763,#291764,#291765,#291766,
#291767,#291768,#291769,#291770,#291771,#291772,#291773,#291774,#291775,
#291776,#291777,#291778,#291779,#291780,#291781,#291782,#291783,#291784,
#291785,#291786,#291787,#291788,#291789,#291790,#291791,#291792,#291793,
#291794,#291795,#291796,#291797),.UNSPECIFIED.,.F.,.F.,(4,2,2,2,2,2,2,2,
2,2,2,2,2,2,2,2,2,4),(63.7157748578674,63.8667739613376,64.3390086392791,
64.8079809218208,65.2735610187678,65.749997216052,66.2152806166965,66.6846270421634,
67.1581164959717,67.622456849824,68.0958431164314,68.5635163180422,69.0300112888132,
69.5076364615024,69.9724490797265,70.4429178387003,70.9146543577095,71.286676879443),
 .UNSPECIFIED.);
#6722=B_SPLINE_CURVE_WITH_KNOTS('',3,(#291798,#291799,#291800,#291801,#291802,
#291803,#291804,#291805,#291806,#291807,#291808,#291809,#291810,#291811,
#291812,#291813,#291814,#291815,#291816,#291817,#291818,#291819,#291820,
#291821,#291822,#291823,#291824,#291825,#291826,#291827,#291828,#291829,
#291830,#291831,#291832,#291833),.UNSPECIFIED.,.F.,.F.,(4,2,2,2,2,2,2,2,
2,2,2,2,2,2,2,2,2,4),(22.8714706980816,23.051617364947,23.525875102884,
23.9905047761518,24.4629235046836,24.9330920693315,25.3981376396358,25.875439535867,
26.3416800031223,26.8098780475167,27.2829520142995,27.7473381575111,28.2216223900459,
28.6906851247604,29.1563019249832,29.6324349705965,30.0978598595751,30.4439313175857),
 .UNSPECIFIED.);
#6723=B_SPLINE_CURVE_WITH_KNOTS('',3,(#291838,#291839,#291840,#291841,#291842,
#291843,#291844,#291845,#291846,#291847,#291848,#291849,#291850,#291851,
#291852,#291853,#291854,#291855,#291856,#291857,#291858,#291859,#291860,
#291861,#291862,#291863,#291864,#291865,#291866,#291867,#291868,#291869,
#291870,#291871,#291872,#291873),.UNSPECIFIED.,.F.,.F.,(4,2,2,2,2,2,2,2,
2,2,2,2,2,2,2,2,2,4),(56.144083628874,56.3525198790904,56.8227384992186,
57.2950413906242,57.7596779166521,58.2339896093383,58.7010155850834,59.1683341887742,
59.6461425436081,60.1106559537008,60.5818215910562,61.0523603629285,61.5173169435704,
61.9926351088461,62.4586675805972,62.9269512318712,63.4024908375553,63.7157748578674),
 .UNSPECIFIED.);
#6724=B_SPLINE_CURVE_WITH_KNOTS('',3,(#291874,#291875,#291876,#291877,#291878,
#291879,#291880,#291881,#291882,#291883,#291884,#291885,#291886,#291887,
#291888,#291889,#291890,#291891,#291892,#291893,#291894,#291895,#291896,
#291897,#291898,#291899,#291900,#291901,#291902,#291903,#291904,#291905,
#291906,#291907,#291908,#291909),.UNSPECIFIED.,.F.,.F.,(4,2,2,2,2,2,2,2,
2,2,2,2,2,2,2,2,2,4),(30.4439313175857,30.5674582054022,31.0394048318556,
31.5038365004404,31.9802587733485,32.4482886730917,32.914746234382,33.3897958731133,
33.8547045464092,34.3259485102396,34.7968646444142,35.2616232427546,35.7397219718357,
36.2066456605547,36.6739778191192,37.1478267439181,37.6122999116294,38.016360947702),
 .UNSPECIFIED.);
#6725=B_SPLINE_CURVE_WITH_KNOTS('',3,(#291914,#291915,#291916,#291917,#291918,
#291919,#291920,#291921,#291922,#291923,#291924,#291925,#291926,#291927,
#291928,#291929,#291930,#291931,#291932,#291933,#291934,#291935,#291936,
#291937,#291938,#291939,#291940,#291941,#291942,#291943,#291944,#291945,
#291946,#291947,#291948,#291949),.UNSPECIFIED.,.F.,.F.,(4,2,2,2,2,2,2,2,
2,2,2,2,2,2,2,2,2,4),(48.5719605686275,48.8375787381526,49.3056503252136,
49.7819246755741,50.2463296313892,50.718323774952,51.1878163381561,51.6532648716521,
52.1294480473886,52.5950075109716,53.0641172410405,53.5382674171041,54.002643888761,
54.4757697545506,54.9438783970752,55.4101593272649,55.8875150473913,56.144083628874),
 .UNSPECIFIED.);
#6726=B_SPLINE_CURVE_WITH_KNOTS('',3,(#291950,#291951,#291952,#291953,#291954,
#291955,#291956,#291957,#291958,#291959,#291960,#291961,#291962,#291963,
#291964,#291965,#291966,#291967,#291968,#291969,#291970,#291971,#291972,
#291973,#291974,#291975,#291976,#291977,#291978,#291979,#291980,#291981,
#291982,#291983,#291984,#291985),.UNSPECIFIED.,.F.,.F.,(4,2,2,2,2,2,2,2,
2,2,2,2,2,2,2,2,2,4),(38.016360947702,38.0851789736651,38.5606918019714,
39.0266489381757,39.4951197018306,39.9704047728814,40.4347225522676,40.9071580162034,
41.3759772432034,41.8417118872276,42.3183551619773,42.7836004036095,43.2531445841241,
43.7264164718864,44.1908318584271,44.664427268518,45.1319885476618,45.5876503801449),
 .UNSPECIFIED.);
#6727=B_SPLINE_CURVE_WITH_KNOTS('',3,(#291990,#291991,#291992,#291993,#291994,
#291995,#291996,#291997,#291998,#291999,#292000,#292001,#292002,#292003,
#292004,#292005,#292006,#292007,#292008,#292009,#292010,#292011,#292012,
#292013,#292014,#292015,#292016,#292017,#292018,#292019,#292020,#292021,
#292022,#292023,#292024,#292025),.UNSPECIFIED.,.F.,.F.,(4,2,2,2,2,2,2,2,
2,2,2,2,2,2,2,2,2,4),(41.0001199248139,41.3231774301242,41.78911725615,
42.2660541939051,42.7311229051682,43.2009434587001,43.6736831387611,44.1381462914927,
44.6120386288035,45.0792786949266,45.5462430113534,46.0243865775315,46.4891026897119,
46.9600595973249,47.4311852824456,47.8960997290458,48.3711933932353,48.5719605686275),
 .UNSPECIFIED.);
#6728=B_SPLINE_CURVE_WITH_KNOTS('',3,(#292026,#292027,#292028,#292029,#292030,
#292031,#292032,#292033,#292034,#292035,#292036,#292037,#292038,#292039,
#292040,#292041,#292042,#292043,#292044,#292045,#292046,#292047,#292048,
#292049,#292050,#292051,#292052,#292053,#292054,#292055,#292056,#292057,
#292058,#292059,#292060,#292061,#292062,#292063),.UNSPECIFIED.,.F.,.F.,
(4,2,2,2,2,2,2,2,2,2,2,2,2,2,2,2,2,2,4),(45.5876503801449,45.5986758559509,
46.0765148693568,46.5413289532617,47.0120009270319,47.4835655594758,47.9483600945364,
48.4231528636811,48.8897704410641,49.3575529036341,49.8344003044135,50.2988326237114,
50.7705098865814,51.2403871160248,51.7056343950673,52.1814875721346,52.6472130277606,
53.1160082110126,53.1596619246187),.UNSPECIFIED.);
#6729=B_SPLINE_CURVE_WITH_KNOTS('',3,(#292068,#292069,#292070,#292071,#292072,
#292073,#292074,#292075,#292076,#292077,#292078,#292079,#292080,#292081,
#292082,#292083,#292084,#292085,#292086,#292087,#292088,#292089,#292090,
#292091,#292092,#292093,#292094,#292095,#292096,#292097,#292098,#292099,
#292100,#292101,#292102,#292103),.UNSPECIFIED.,.F.,.F.,(4,2,2,2,2,2,2,2,
2,2,2,2,2,2,2,2,2,4),(33.4289203540015,33.8017623441053,34.2734695384679,
34.7439861866962,35.2088049428035,35.6864802632978,36.1530204914359,36.6206766322363,
37.0941120115672,37.5584735418785,38.0319244250421,38.5013175525154,38.9665989988937,
39.4430838829474,39.9177587985401,40.3820449298253,40.8547633332481,41.0001199248139),
 .UNSPECIFIED.);
#6730=B_SPLINE_CURVE_WITH_KNOTS('',3,(#292104,#292105,#292106,#292107,#292108,
#292109,#292110,#292111,#292112,#292113,#292114,#292115,#292116,#292117,
#292118,#292119,#292120,#292121,#292122,#292123,#292124,#292125,#292126,
#292127,#292128,#292129,#292130,#292131,#292132,#292133,#292134,#292135,
#292136,#292137,#292138,#292139),.UNSPECIFIED.,.F.,.F.,(4,2,2,2,2,2,2,2,
2,2,2,2,2,2,2,2,2,4),(53.1596619246187,53.590671333377,54.0549979571361,
54.5277856350263,54.9962063209033,55.4622084789415,55.9392160136559,56.4043119711095,
56.8742008482708,57.3469359753347,57.8114468705411,58.2854097230149,58.7526640946325,
59.2196972269946,59.6979123556361,60.1626628717794,60.6336888645837,60.7316199823971),
 .UNSPECIFIED.);
#6731=B_SPLINE_CURVE_WITH_KNOTS('',3,(#292144,#292145,#292146,#292147,#292148,
#292149,#292150,#292151,#292152,#292153,#292154,#292155,#292156,#292157,
#292158,#292159,#292160,#292161,#292162,#292163,#292164,#292165,#292166,
#292167,#292168,#292169,#292170,#292171,#292172,#292173,#292174,#292175,
#292176,#292177,#292178,#292179),.UNSPECIFIED.,.F.,.F.,(4,2,2,2,2,2,2,2,
2,2,2,2,2,2,2,2,2,4),(25.8580916349655,26.2897324013408,26.7582466058542,
27.2308552574274,27.6951268991933,28.1699649318621,28.638591500359,29.1043500637385,
29.580027924796,30.0451581297893,30.5151573988414,30.9866653386247,31.4510741532502,
31.9281191055042,32.39574427877,32.862421157186,33.3370514851652,33.4289203540015),
 .UNSPECIFIED.);
#6732=B_SPLINE_CURVE_WITH_KNOTS('',3,(#292180,#292181,#292182,#292183,#292184,
#292185,#292186,#292187,#292188,#292189,#292190,#292191,#292192,#292193,
#292194,#292195,#292196,#292197,#292198,#292199,#292200,#292201,#292202,
#292203,#292204,#292205,#292206,#292207,#292208,#292209,#292210,#292211,
#292212,#292213,#292214,#292215),.UNSPECIFIED.,.F.,.F.,(4,2,2,2,2,2,2,2,
2,2,2,2,2,2,2,2,2,4),(60.7316199823971,61.1048185437779,61.5697872371334,
62.0449517676864,62.5113595052275,62.9795002075708,63.4557669984041,63.9202128194296,
64.3922788870764,64.8617804579765,65.3272906155987,65.8035472390145,66.2691351401704,
66.738316236739,67.2124643837799,67.6768887040922,68.1500883737649,68.3044870520947),
 .UNSPECIFIED.);
#6733=B_SPLINE_CURVE_WITH_KNOTS('',3,(#292220,#292221,#292222,#292223,#292224,
#292225,#292226,#292227,#292228,#292229,#292230,#292231,#292232,#292233,
#292234,#292235,#292236,#292237,#292238,#292239,#292240,#292241,#292242,
#292243,#292244,#292245,#292246,#292247,#292248,#292249,#292250,#292251,
#292252,#292253,#292254,#292255,#292256,#292257),.UNSPECIFIED.,.F.,.F.,
(4,2,2,2,2,2,2,2,2,2,2,2,2,2,2,2,2,2,4),(18.2865751343784,18.3079357785441,
18.7758965839359,19.2423287253566,19.7173075924809,20.1821613811676,20.6533968732839,
21.1242439543697,21.5889660187706,22.0669933427192,22.5338486997724,23.0011628723484,
23.4749414259118,23.9393657833007,24.4122441508144,24.8819572888962,25.3470560430857,
25.823879834484,25.8580916349655),.UNSPECIFIED.);
#6734=B_SPLINE_CURVE_WITH_KNOTS('',3,(#292258,#292259,#292260,#292261,#292262,
#292263,#292264,#292265,#292266,#292267,#292268,#292269,#292270,#292271,
#292272,#292273,#292274,#292275,#292276,#292277,#292278,#292279,#292280,
#292281,#292282,#292283,#292284,#292285,#292286,#292287,#292288,#292289,
#292290,#292291,#292292,#292293),.UNSPECIFIED.,.F.,.F.,(4,2,2,2,2,2,2,2,
2,2,2,2,2,2,2,2,2,4),(68.3044870520947,68.6182126328683,69.0845621343954,
69.5619929048661,70.0270329255262,70.4973242517696,70.9696324304201,71.4343235782796,
71.9087100116139,72.3757591231006,72.8431508542522,73.3209523395419,73.7855068821371,
74.2567488157943,74.7272966253318,75.1923153308094,75.6677115997742,75.8772668463336),
 .UNSPECIFIED.);
#6735=B_SPLINE_CURVE_WITH_KNOTS('',3,(#292298,#292299,#292300,#292301,#292302,
#292303,#292304,#292305,#292306,#292307,#292308,#292309,#292310,#292311,
#292312,#292313,#292314,#292315,#292316,#292317,#292318,#292319,#292320,
#292321,#292322,#292323,#292324,#292325,#292326,#292327,#292328,#292329,
#292330,#292331,#292332,#292333),.UNSPECIFIED.,.F.,.F.,(4,2,2,2,2,2,2,2,
2,2,2,2,2,2,2,2,2,4),(10.7151222517789,10.7913599012759,11.2614558718779,
11.7264642452055,12.203691307493,12.6698634933475,13.138042532141,13.611042890141,
14.0753800813121,14.5496616010084,15.0186530670319,15.4842389138994,15.960298702674,
16.4256618397833,16.8952472113547,17.3671220636508,17.8315112596137,18.2865751343784),
 .UNSPECIFIED.);
#6736=B_SPLINE_CURVE_WITH_KNOTS('',3,(#292334,#292335,#292336,#292337,#292338,
#292339,#292340,#292341,#292342,#292343,#292344,#292345,#292346,#292347,
#292348,#292349,#292350,#292351,#292352,#292353,#292354,#292355,#292356,
#292357,#292358,#292359,#292360,#292361,#292362,#292363,#292364,#292365,
#292366,#292367,#292368,#292369),.UNSPECIFIED.,.F.,.F.,(4,2,2,2,2,2,2,2,
2,2,2,2,2,2,2,2,2,4),(75.8772668463336,76.1337725928702,76.6021323698784,
77.0776691799798,77.5420003802429,78.014314023934,78.4833010889462,78.9489509317474,
79.4254676248807,79.8907861158707,80.3602107320054,80.833703738573,81.2980994399929,
81.7715663367368,82.2392615376057,82.705833195356,83.1835402439425,83.4488930554441),
 .UNSPECIFIED.);
#6737=B_SPLINE_CURVE_WITH_KNOTS('',3,(#292374,#292375,#292376,#292377,#292378,
#292379,#292380,#292381,#292382,#292383,#292384,#292385,#292386,#292387,
#292388,#292389,#292390,#292391,#292392,#292393,#292394,#292395,#292396,
#292397,#292398,#292399,#292400,#292401,#292402,#292403,#292404,#292405,
#292406,#292407,#292408,#292409),.UNSPECIFIED.,.F.,.F.,(4,2,2,2,2,2,2,2,
2,2,2,2,2,2,2,2,2,4),(3.14443208990716,3.27554668679239,3.74763766305925,
4.2118807700592,4.68755559513844,5.15570421655467,5.62176327704835,6.09694161106962,
6.56181075862647,7.03244318834201,7.50347408717017,7.96797097464197,8.44592850904672,
8.91312216961858,9.38019300365707,9.85437618111417,10.3189505589872,10.7151222517789),
 .UNSPECIFIED.);
#6738=B_SPLINE_CURVE_WITH_KNOTS('',3,(#292410,#292411,#292412,#292413,#292414,
#292415,#292416,#292417,#292418,#292419,#292420,#292421,#292422,#292423,
#292424,#292425,#292426,#292427,#292428,#292429,#292430,#292431,#292432,
#292433,#292434,#292435,#292436,#292437,#292438,#292439,#292440,#292441,
#292442,#292443,#292444,#292445),.UNSPECIFIED.,.F.,.F.,(4,2,2,2,2,2,2,2,
2,2,2,2,2,2,2,2,2,4),(83.4488930554441,83.6483950281211,84.1189431117052,
84.5906911700159,85.0554352920183,85.5300971477342,85.9968119055917,86.4644682251567,
86.9415561790123,87.4060001152473,87.877539120961,88.3475784949245,88.8127409501058,
89.2884500085642,89.754245569256,90.2229029989712,90.6977831716255,91.0207492930948),
 .UNSPECIFIED.);
#6739=B_SPLINE_CURVE_WITH_KNOTS('',3,(#292451,#292452,#292453,#292454,#292455,
#292456,#292457,#292458,#292459,#292460,#292461,#292462,#292463,#292464,
#292465,#292466,#292467,#292468,#292469,#292470,#292471,#292472),
 .UNSPECIFIED.,.F.,.F.,(4,2,2,2,2,2,2,2,2,2,4),(136.24403458457,136.622483679541,
137.087116542782,137.561813612369,138.028135240898,138.495820731345,138.972238243539,
139.436453120851,139.908042383763,140.37046393164,140.833986548193),
 .UNSPECIFIED.);
#6740=B_SPLINE_CURVE_WITH_KNOTS('',3,(#292475,#292476,#292477,#292478,#292479,
#292480,#292481,#292482,#292483,#292484,#292485,#292486,#292487,#292488,
#292489,#292490,#292491,#292492),.UNSPECIFIED.,.F.,.F.,(4,2,2,2,2,2,2,2,
4),(1.00000002595246E-6,0.432220701825413,0.859903589947374,1.3366986521,
1.80250598802853,2.27083750612852,2.74341592545933,3.20758955595405,3.63988072813663),
 .UNSPECIFIED.);
#6741=B_SPLINE_CURVE_WITH_KNOTS('',3,(#292497,#292498,#292499,#292500,#292501,
#292502,#292503,#292504,#292505,#292506,#292507,#292508,#292509,#292510,
#292511,#292512,#292513,#292514,#292515,#292516,#292517,#292518,#292519,
#292520,#292521,#292522,#292523,#292524,#292525,#292526,#292527,#292528,
#292529,#292530,#292531,#292532),.UNSPECIFIED.,.F.,.F.,(4,2,2,2,2,2,2,2,
2,2,2,2,2,2,2,2,2,4),(128.675938040482,129.112558893719,129.576657723443,
130.048991214851,130.517448780484,130.983053196247,131.459596796231,131.924568127943,
132.394009334762,132.866869411823,133.331095846395,133.804594400205,134.271825895138,
134.738410083798,135.216153340899,135.680723343159,136.151295376315,136.24403458457),
 .UNSPECIFIED.);
#6742=B_SPLINE_CURVE_WITH_KNOTS('',3,(#292533,#292534,#292535,#292536,#292537,
#292538,#292539,#292540,#292541,#292542,#292543,#292544,#292545,#292546,
#292547,#292548,#292549,#292550,#292551,#292552,#292553,#292554,#292555,
#292556,#292557,#292558,#292559,#292560,#292561,#292562,#292563,#292564,
#292565,#292566,#292567,#292568,#292569,#292570),.UNSPECIFIED.,.F.,.F.,
(4,2,2,2,2,2,2,2,2,2,2,2,2,2,2,2,2,2,4),(3.63988072813663,3.68219744944784,
4.15078913768896,4.61639991622148,5.09204469600563,5.55711167641085,6.02691203047307,
6.49838465537246,6.96267787157272,7.43947959951173,7.9070637451659,8.37357792866613,
8.84816816756442,9.31279714879658,9.78429353632221,10.2547672182533,10.7194544807213,
11.1970895372671,11.2094799248909),.UNSPECIFIED.);
#6743=B_SPLINE_CURVE_WITH_KNOTS('',3,(#292575,#292576,#292577,#292578,#292579,
#292580,#292581,#292582,#292583,#292584,#292585,#292586,#292587,#292588,
#292589,#292590,#292591,#292592,#292593,#292594,#292595,#292596,#292597,
#292598,#292599,#292600,#292601,#292602,#292603,#292604,#292605,#292606,
#292607,#292608,#292609,#292610,#292611,#292612),.UNSPECIFIED.,.F.,.F.,
(4,2,2,2,2,2,2,2,2,2,2,2,2,2,2,2,2,2,4),(121.107364429924,121.123955006208,
121.60136663952,122.066059079849,122.536320554389,123.008007747065,123.472523016408,
123.94689130063,124.413484347362,124.880853415232,125.35792043923,125.822181143827,
126.293422250453,126.763386474281,127.228294640259,127.703699650335,128.169354359971,
128.637715264481,128.675938040482),.UNSPECIFIED.);
#6744=B_SPLINE_CURVE_WITH_KNOTS('',3,(#292613,#292614,#292615,#292616,#292617,
#292618,#292619,#292620,#292621,#292622,#292623,#292624,#292625,#292626,
#292627,#292628,#292629,#292630,#292631,#292632,#292633,#292634,#292635,
#292636,#292637,#292638,#292639,#292640,#292641,#292642,#292643,#292644,
#292645,#292646,#292647,#292648),.UNSPECIFIED.,.F.,.F.,(4,2,2,2,2,2,2,2,
2,2,2,2,2,2,2,2,2,4),(11.2094799248909,11.6635829376649,12.1310561877189,
12.6044504052173,13.0687133826433,13.5419326181211,14.011280641485,14.4764127911059,
14.9528547084907,15.418408801106,15.887154115734,16.3593915318822,16.8235710185186,
17.298815974715,17.7670945040135,18.2329514101939,18.7082674324183,18.7784627545738),
 .UNSPECIFIED.);
#6745=B_SPLINE_CURVE_WITH_KNOTS('',3,(#292653,#292654,#292655,#292656,#292657,
#292658,#292659,#292660,#292661,#292662,#292663,#292664,#292665,#292666,
#292667,#292668,#292669,#292670,#292671,#292672,#292673,#292674,#292675,
#292676,#292677,#292678,#292679,#292680,#292681,#292682,#292683,#292684,
#292685,#292686,#292687,#292688),.UNSPECIFIED.,.F.,.F.,(4,2,2,2,2,2,2,2,
2,2,2,2,2,2,2,2,2,4),(113.539080310834,113.613535836383,114.088649521034,
114.554593310473,115.022677384666,115.498200419705,115.962349691178,116.434377971026,
116.903293351852,117.368689275545,117.844915288929,118.31009488851,118.779236801359,
119.252695251587,119.71688487643,120.190060730064,120.657660459202,121.107364429924),
 .UNSPECIFIED.);
#6746=B_SPLINE_CURVE_WITH_KNOTS('',3,(#292689,#292690,#292691,#292692,#292693,
#292694,#292695,#292696,#292697,#292698,#292699,#292700,#292701,#292702,
#292703,#292704,#292705,#292706,#292707,#292708,#292709,#292710,#292711,
#292712,#292713,#292714,#292715,#292716,#292717,#292718,#292719,#292720,
#292721,#292722,#292723,#292724),.UNSPECIFIED.,.F.,.F.,(4,2,2,2,2,2,2,2,
2,2,2,2,2,2,2,2,2,4),(18.7784627545738,19.1731708477413,19.6434607197414,
20.1146201965419,20.5790046301623,21.056501945035,21.5238052639034,21.9906354266554,
22.4649335203834,22.9294898734969,23.4015289871598,23.8717291250978,24.3365830363145,
24.8139245228879,25.28017495983,25.7480597722722,26.2211694508468,26.3486586062954),
 .UNSPECIFIED.);
#6747=B_SPLINE_CURVE_WITH_KNOTS('',3,(#292729,#292730,#292731,#292732,#292733,
#292734,#292735,#292736,#292737,#292738,#292739,#292740,#292741,#292742,
#292743,#292744,#292745,#292746,#292747,#292748,#292749,#292750,#292751,
#292752,#292753,#292754,#292755,#292756,#292757,#292758,#292759,#292760,
#292761,#292762,#292763,#292764),.UNSPECIFIED.,.F.,.F.,(4,2,2,2,2,2,2,2,
2,2,2,2,2,2,2,2,2,4),(105.969272897385,106.100976102842,106.573907730878,
107.041957253409,107.508056840031,107.985215205638,108.4501158598,108.920142879015,
109.392410355181,109.856897820666,110.331012971347,110.797962572073,111.265088687778,
111.742889573364,112.20728516231,112.67825074303,113.148745691294,113.539080310834),
 .UNSPECIFIED.);
#6748=B_SPLINE_CURVE_WITH_KNOTS('',3,(#292765,#292766,#292767,#292768,#292769,
#292770,#292771,#292772,#292773,#292774,#292775,#292776,#292777,#292778,
#292779,#292780,#292781,#292782,#292783,#292784,#292785,#292786,#292787,
#292788,#292789,#292790,#292791,#292792,#292793,#292794,#292795,#292796,
#292797,#292798,#292799,#292800),.UNSPECIFIED.,.F.,.F.,(4,2,2,2,2,2,2,2,
2,2,2,2,2,2,2,2,2,4),(26.3486586062954,26.6854413743924,27.1592999290633,
27.6283870794954,28.0937707301691,28.5699346677542,29.0353280725909,29.5045718253718,
29.9765437467173,30.4408187574263,30.916779883259,31.3848214438468,31.8510084094083,
32.3260742260102,32.7909070779018,33.2617645498638,33.7326896544931,33.9189878766126),
 .UNSPECIFIED.);
#6749=B_SPLINE_CURVE_WITH_KNOTS('',3,(#292805,#292806,#292807,#292808,#292809,
#292810,#292811,#292812,#292813,#292814,#292815,#292816,#292817,#292818,
#292819,#292820,#292821,#292822,#292823,#292824,#292825,#292826,#292827,
#292828,#292829,#292830,#292831,#292832,#292833,#292834,#292835,#292836,
#292837,#292838,#292839,#292840),.UNSPECIFIED.,.F.,.F.,(4,2,2,2,2,2,2,2,
2,2,2,2,2,2,2,2,2,4),(98.3990302152714,98.5893892664047,99.0601631139654,
99.5312560680723,99.9960223863912,100.470928647386,100.937239158569,101.405127708902,
101.881395775322,102.34568347646,102.817487868981,103.286936380357,103.752219724559,
104.228209394403,104.693680205075,105.162601564527,105.636732990254,105.969272897385),
 .UNSPECIFIED.);
#6750=B_SPLINE_CURVE_WITH_KNOTS('',3,(#292841,#292842,#292843,#292844,#292845,
#292846,#292847,#292848,#292849,#292850,#292851,#292852,#292853,#292854,
#292855,#292856,#292857,#292858,#292859,#292860,#292861,#292862,#292863,
#292864,#292865,#292866,#292867,#292868,#292869,#292870,#292871,#292872,
#292873,#292874,#292875,#292876),.UNSPECIFIED.,.F.,.F.,(4,2,2,2,2,2,2,2,
2,2,2,2,2,2,2,2,2,4),(33.9189878766126,34.1972520714663,34.6753685555233,
35.1423031461174,35.6093148345641,36.0831788632793,36.5475371071326,37.0199763319678,
37.4897630905891,37.9546518147693,38.4315589904034,38.8974462320601,39.3656030133063,
39.8382894090536,40.3024443511905,40.7767910367888,41.2454804759632,41.4881001708513),
 .UNSPECIFIED.);
#6751=B_SPLINE_CURVE_WITH_KNOTS('',3,(#292881,#292882,#292883,#292884,#292885,
#292886,#292887,#292888,#292889,#292890,#292891,#292892,#292893,#292894,
#292895,#292896,#292897,#292898,#292899,#292900,#292901,#292902,#292903,
#292904,#292905,#292906,#292907,#292908,#292909,#292910,#292911,#292912,
#292913,#292914,#292915,#292916),.UNSPECIFIED.,.F.,.F.,(4,2,2,2,2,2,2,2,
2,2,2,2,2,2,2,2,2,4),(90.8296974779451,91.0766374667577,91.5451887830606,
92.0198667981449,92.4840365654737,92.9565715147367,93.424946900688,93.8907200849939,
94.3674702844793,94.8324529999625,95.3020923813277,95.7748187956589,96.2391488853637,
96.7128547646713,97.1800385313284,97.6468211298733,98.1247755874545,98.3990302152714),
 .UNSPECIFIED.);
#6752=B_SPLINE_CURVE_WITH_KNOTS('',3,(#292917,#292918,#292919,#292920,#292921,
#292922,#292923,#292924,#292925,#292926,#292927,#292928,#292929,#292930,
#292931,#292932,#292933,#292934,#292935,#292936,#292937,#292938,#292939,
#292940,#292941,#292942,#292943,#292944,#292945,#292946,#292947,#292948,
#292949,#292950,#292951,#292952),.UNSPECIFIED.,.F.,.F.,(4,2,2,2,2,2,2,2,
2,2,2,2,2,2,2,2,2,4),(41.4881001708513,41.7109798361461,42.1867282812913,
42.6518413385742,43.1214362960486,43.5930071060109,44.0572484489647,44.5337641130283,
45.0014346112672,45.4678094666162,45.9424903699166,46.4071305173474,46.8783991571689,
47.3489568235663,47.8135623653808,48.2912890647894,48.7578601251999,49.0573549288453),
 .UNSPECIFIED.);
#6753=B_SPLINE_CURVE_WITH_KNOTS('',3,(#292957,#292958,#292959,#292960,#292961,
#292962,#292963,#292964,#292965,#292966,#292967,#292968,#292969,#292970,
#292971,#292972,#292973,#292974,#292975,#292976,#292977,#292978,#292979,
#292980,#292981,#292982,#292983,#292984,#292985,#292986,#292987,#292988,
#292989,#292990,#292991,#292992),.UNSPECIFIED.,.F.,.F.,(4,2,2,2,2,2,2,2,
2,2,2,2,2,2,2,2,2,4),(83.2599065759065,83.5638785446524,84.0303385225607,
84.5079350778034,84.9726374682993,85.4430751168375,85.9146310054686,86.379246812249,
86.8537988530033,87.3203457237915,87.787893113324,88.2647721317994,88.7290714467532,
89.2005035658084,89.6703568226975,90.1353999365597,90.6110024064959,90.8296974779451),
 .UNSPECIFIED.);
#6754=B_SPLINE_CURVE_WITH_KNOTS('',3,(#292993,#292994,#292995,#292996,#292997,
#292998,#292999,#293000,#293001,#293002,#293003,#293004,#293005,#293006,
#293007,#293008,#293009,#293010,#293011,#293012,#293013,#293014,#293015,
#293016,#293017,#293018,#293019,#293020,#293021,#293022,#293023,#293024,
#293025,#293026,#293027,#293028),.UNSPECIFIED.,.F.,.F.,(4,2,2,2,2,2,2,2,
2,2,2,2,2,2,2,2,2,4),(49.0573549288453,49.2251563365931,49.6986391379984,
50.1628821752712,50.6358346231852,51.105262582369,51.5702796770147,52.0468081452395,
52.5124088045048,52.980941975819,53.4532615481695,53.9173873063535,54.3923333888046,
54.8606834805659,55.3263937313117,55.8017864800737,56.2667015279438,56.6256830979513),
 .UNSPECIFIED.);
#6755=B_SPLINE_CURVE_WITH_KNOTS('',3,(#293033,#293034,#293035,#293036,#293037,
#293038,#293039,#293040,#293041,#293042,#293043,#293044,#293045,#293046,
#293047,#293048,#293049,#293050,#293051,#293052,#293053,#293054,#293055,
#293056,#293057,#293058,#293059,#293060,#293061,#293062,#293063,#293064,
#293065,#293066,#293067,#293068),.UNSPECIFIED.,.F.,.F.,(4,2,2,2,2,2,2,2,
2,2,2,2,2,2,2,2,2,4),(75.6907199874016,76.0542240558732,76.5191143039749,
76.9943966225301,77.4602882622359,77.9285347773458,78.4038604257591,78.8680465700418,
79.3402486234638,79.8090485605776,80.2745788198699,80.7509839140138,81.216141299872,
81.6854546385995,82.1587450732675,82.6230044270935,83.0963611965978,83.2599065759065),
 .UNSPECIFIED.);
#6756=B_SPLINE_CURVE_WITH_KNOTS('',3,(#293069,#293070,#293071,#293072,#293073,
#293074,#293075,#293076,#293077,#293078,#293079,#293080,#293081,#293082,
#293083,#293084,#293085,#293086,#293087,#293088,#293089,#293090,#293091,
#293092,#293093,#293094,#293095,#293096,#293097,#293098,#293099,#293100,
#293101,#293102,#293103,#293104),.UNSPECIFIED.,.F.,.F.,(4,2,2,2,2,2,2,2,
2,2,2,2,2,2,2,2,2,4),(56.6256830979513,56.7367504130986,57.2079808841007,
57.6722786679109,58.1494551797369,58.6168172394204,59.0813134132729,59.5522332371109,
60.0229669193424,60.4877698659642,60.9628324484622,61.4289307276113,61.8969677657921,
62.3727826769255,62.8370034526151,63.308974812071,63.7781046940472,64.1949548606005),
 .UNSPECIFIED.);
#6757=B_SPLINE_CURVE_WITH_KNOTS('',3,(#293109,#293110,#293111,#293112,#293113,
#293114,#293115,#293116,#293117,#293118,#293119,#293120,#293121,#293122,
#293123,#293124,#293125,#293126,#293127,#293128,#293129,#293130,#293131,
#293132,#293133,#293134,#293135,#293136,#293137,#293138,#293139,#293140,
#293141,#293142,#293143,#293144),.UNSPECIFIED.,.F.,.F.,(4,2,2,2,2,2,2,2,
2,2,2,2,2,2,2,2,2,4),(68.1203183363462,68.5417873876646,69.0060663283817,
69.4791478952628,69.9470862950396,70.4133145452217,70.8906268551915,71.3555059566908,
71.8256791140487,72.2977871709703,72.7623409711255,73.2366098835529,73.7034826895161,
74.1707580079406,74.6483423631239,75.1127433836254,75.5838710201412,75.6907199874016),
 .UNSPECIFIED.);
#6758=B_SPLINE_CURVE_WITH_KNOTS('',3,(#293145,#293146,#293147,#293148,#293149,
#293150,#293151,#293152,#293153,#293154,#293155,#293156,#293157,#293158,
#293159,#293160,#293161,#293162,#293163,#293164,#293165,#293166,#293167,
#293168,#293169,#293170,#293171,#293172,#293173,#293174,#293175,#293176,
#293177,#293178,#293179,#293180,#293181,#293182),.UNSPECIFIED.,.F.,.F.,
(4,2,2,2,2,2,2,2,2,2,2,2,2,2,2,2,2,2,4),(64.1949548606005,64.2434814748872,
64.7196464066227,65.1849527935229,65.6540390711369,66.1277624520122,66.5919928976285,
67.0651049508879,67.5328885452889,67.9991346350153,68.476479537035,68.9412686999514,
69.4114699402805,69.8833879753948,70.3479150134625,70.8222167019006,71.2889597376057,
71.7562656212209,71.7645272101572),.UNSPECIFIED.);
#6759=B_SPLINE_CURVE_WITH_KNOTS('',3,(#293187,#293188,#293189,#293190,#293191,
#293192,#293193,#293194,#293195,#293196,#293197,#293198,#293199,#293200,
#293201,#293202,#293203,#293204,#293205,#293206,#293207,#293208,#293209,
#293210,#293211,#293212,#293213,#293214,#293215,#293216,#293217,#293218,
#293219,#293220,#293221,#293222,#293223,#293224),.UNSPECIFIED.,.F.,.F.,
(4,2,2,2,2,2,2,2,2,2,2,2,2,2,2,2,2,2,4),(60.5498333392294,60.5516208768603,
61.029713077203,61.4943018268745,61.9652050391113,62.4361334285903,62.9009642299098,
63.3760063085563,63.8422370545959,64.310256257033,64.7863055900214,65.2505975962196,
65.7225438217246,66.1918509203695,66.6572318432376,67.1333686185619,67.5987872086308,
68.0678490351813,68.1203183363462),.UNSPECIFIED.);
#6760=B_SPLINE_CURVE_WITH_KNOTS('',3,(#293225,#293226,#293227,#293228,#293229,
#293230,#293231,#293232,#293233,#293234,#293235,#293236,#293237,#293238,
#293239,#293240,#293241,#293242,#293243,#293244,#293245,#293246,#293247,
#293248,#293249,#293250,#293251,#293252,#293253,#293254,#293255,#293256,
#293257,#293258,#293259,#293260),.UNSPECIFIED.,.F.,.F.,(4,2,2,2,2,2,2,2,
2,2,2,2,2,2,2,2,2,4),(71.7645272101572,72.2336184703587,72.6979492173401,
73.1691158463344,73.6392922669799,74.1041798706507,74.5795050993304,75.0452851065681,
75.5135711699015,75.9886800701136,76.4528185565236,76.9250674549146,77.3937104149963,
77.8592621871405,78.3357171236383,78.8007845612436,79.2701433689272,79.3329795049996),
 .UNSPECIFIED.);
#6761=B_SPLINE_CURVE_WITH_KNOTS('',3,(#293265,#293266,#293267,#293268,#293269,
#293270,#293271,#293272,#293273,#293274,#293275,#293276,#293277,#293278,
#293279,#293280,#293281,#293282,#293283,#293284,#293285,#293286,#293287,
#293288,#293289,#293290,#293291,#293292,#293293,#293294,#293295,#293296,
#293297,#293298,#293299,#293300),.UNSPECIFIED.,.F.,.F.,(4,2,2,2,2,2,2,2,
2,2,2,2,2,2,2,2,2,4),(52.9806944783428,53.0476758259382,53.5172526200669,
53.9822867329294,54.4589700451137,54.9246978883063,55.3931826697128,55.8656533421869,
56.3298377489955,56.8046773546697,57.2731706643284,57.7388763386877,58.2144173370291,
58.679435794573,59.1438011651963,59.6176416939812,60.0847089200864,60.5498333392294),
 .UNSPECIFIED.);
#6762=B_SPLINE_CURVE_WITH_KNOTS('',3,(#293301,#293302,#293303,#293304,#293305,
#293306,#293307,#293308,#293309,#293310,#293311,#293312,#293313,#293314,
#293315,#293316,#293317,#293318,#293319,#293320,#293321,#293322,#293323,
#293324,#293325,#293326,#293327,#293328,#293329,#293330,#293331,#293332,
#293333,#293334,#293335,#293336),.UNSPECIFIED.,.F.,.F.,(4,2,2,2,2,2,2,2,
2,2,2,2,2,2,2,2,2,4),(79.3329795049996,79.7432389050355,80.2074739405494,
80.6808821375356,81.1482665820861,81.6147697069897,82.092419760985,82.5570552029074,
83.0275412408173,83.4989290104156,83.9635421064772,84.4381471318181,84.9045871045244,
85.3721846846847,85.8488549269602,86.313107852614,86.7845983573231,86.9020880596309),
 .UNSPECIFIED.);
#6763=B_SPLINE_CURVE_WITH_KNOTS('',3,(#293341,#293342,#293343,#293344,#293345,
#293346,#293347,#293348,#293349,#293350,#293351,#293352,#293353,#293354,
#293355,#293356,#293357,#293358,#293359,#293360,#293361,#293362,#293363,
#293364,#293365,#293366,#293367,#293368,#293369,#293370,#293371,#293372,
#293373,#293374,#293375,#293376),.UNSPECIFIED.,.F.,.F.,(4,2,2,2,2,2,2,2,
2,2,2,2,2,2,2,2,2,4),(45.4104974364304,45.5321719174255,46.0039037540315,
46.4682050210216,46.9446247162805,47.4124476030884,47.8788235312033,48.3536612318455,
48.8184039399149,49.2896146811765,49.7603238968664,50.2249690616266,50.702854011143,
51.1695732360491,51.6368449971586,52.1104831991918,52.5748078362504,52.9806944783428),
 .UNSPECIFIED.);
#6764=B_SPLINE_CURVE_WITH_KNOTS('',3,(#293377,#293378,#293379,#293380,#293381,
#293382,#293383,#293384,#293385,#293386,#293387,#293388,#293389,#293390,
#293391,#293392,#293393,#293394,#293395,#293396,#293397,#293398,#293399,
#293400,#293401,#293402,#293403,#293404,#293405,#293406,#293407,#293408,
#293409,#293410,#293411,#293412),.UNSPECIFIED.,.F.,.F.,(4,2,2,2,2,2,2,2,
2,2,2,2,2,2,2,2,2,4),(86.9020880596309,87.2542987090969,87.7193633179202,
88.1950279435794,88.6605753005546,89.1291848608632,89.6036709318418,90.0678172046687,
90.5404173981671,91.0086608535846,91.4744790277654,91.9512973083383,92.4162144467835,
92.8859170622057,93.3584748655669,93.8228043442849,94.2965791009012,94.4707808282852),
 .UNSPECIFIED.);
#6765=B_SPLINE_CURVE_WITH_KNOTS('',3,(#293417,#293418,#293419,#293420,#293421,
#293422,#293423,#293424,#293425,#293426,#293427,#293428,#293429,#293430,
#293431,#293432,#293433,#293434,#293435,#293436,#293437,#293438,#293439,
#293440,#293441,#293442,#293443,#293444,#293445,#293446,#293447,#293448,
#293449,#293450,#293451,#293452),.UNSPECIFIED.,.F.,.F.,(4,2,2,2,2,2,2,2,
2,2,2,2,2,2,2,2,2,4),(37.8404050120038,38.0187279036585,38.4927627146799,
38.9572252071081,39.4296082914203,39.8995596682351,40.3644899534552,40.8415681146096,
41.3076041454195,41.7757390083765,42.2485928495683,42.7128300300082,43.1870976300135,
43.6559470476141,44.1214664273962,44.5973803361899,45.0626195647578,45.4104974364304),
 .UNSPECIFIED.);
#6766=B_SPLINE_CURVE_WITH_KNOTS('',3,(#293453,#293454,#293455,#293456,#293457,
#293458,#293459,#293460,#293461,#293462,#293463,#293464,#293465,#293466,
#293467,#293468,#293469,#293470,#293471,#293472,#293473,#293474,#293475,
#293476,#293477,#293478,#293479,#293480,#293481,#293482,#293483,#293484,
#293485,#293486,#293487,#293488),.UNSPECIFIED.,.F.,.F.,(4,2,2,2,2,2,2,2,
2,2,2,2,2,2,2,2,2,4),(94.4707808282852,94.763655618974,95.230503489999,
95.7085287786169,96.1730996219083,96.6439388214966,97.1148906048698,97.5796768167616,
98.0546527520435,98.5208818428841,98.9888368347847,99.4649253819484,99.9291907564215,
100.40106925086,100.870392847739,101.33571930717,101.811786571165,102.040885959867),
 .UNSPECIFIED.);
#6767=B_SPLINE_CURVE_WITH_KNOTS('',3,(#293493,#293494,#293495,#293496,#293497,
#293498,#293499,#293500,#293501,#293502,#293503,#293504,#293505,#293506,
#293507,#293508,#293509,#293510,#293511,#293512,#293513,#293514,#293515,
#293516,#293517,#293518,#293519,#293520,#293521,#293522,#293523,#293524,
#293525,#293526,#293527,#293528),.UNSPECIFIED.,.F.,.F.,(4,2,2,2,2,2,2,2,
2,2,2,2,2,2,2,2,2,4),(30.2717430383538,30.5048631953018,30.9809925676507,
31.4463209930157,31.9153253368422,32.3872602441844,32.8514030187422,33.3270662479309,
33.7950640259182,34.2610568702298,34.7360806920456,35.2008248414998,35.6714249241691,
36.1423047011262,36.6067133213153,37.0846658279564,37.5517141448292,37.8404050120038),
 .UNSPECIFIED.);
#6768=B_SPLINE_CURVE_WITH_KNOTS('',3,(#293529,#293530,#293531,#293532,#293533,
#293534,#293535,#293536,#293537,#293538,#293539,#293540,#293541,#293542,
#293543,#293544,#293545,#293546,#293547,#293548,#293549,#293550,#293551,
#293552,#293553,#293554,#293555,#293556,#293557,#293558,#293559,#293560,
#293561,#293562,#293563,#293564),.UNSPECIFIED.,.F.,.F.,(4,2,2,2,2,2,2,2,
2,2,2,2,2,2,2,2,2,4),(102.040885959867,102.277195302756,102.746189989452,
103.220159927948,103.684402850689,104.157414263722,104.625360157971,105.09152469262,
105.568765443022,106.033625572829,106.503729888608,106.975859544708,107.440368265367,
107.914565867975,108.381435986137,108.848641741376,109.326264303091,109.610952863519),
 .UNSPECIFIED.);
#6769=B_SPLINE_CURVE_WITH_KNOTS('',3,(#293569,#293570,#293571,#293572,#293573,
#293574,#293575,#293576,#293577,#293578,#293579,#293580,#293581,#293582,
#293583,#293584,#293585,#293586,#293587,#293588,#293589,#293590,#293591,
#293592,#293593,#293594,#293595,#293596,#293597,#293598,#293599,#293600,
#293601,#293602,#293603,#293604),.UNSPECIFIED.,.F.,.F.,(4,2,2,2,2,2,2,2,
2,2,2,2,2,2,2,2,2,4),(22.7031707982564,22.99208933736,23.4692920572669,
23.9365641978222,24.403203099421,24.8774713373835,25.3419400064753,25.8137267074878,
26.2838928645293,26.7485956743227,27.2259067851868,27.692114101337,28.1597823250655,
28.632860104015,29.0970226309293,29.570603328209,30.0396530967059,30.2717430383538),
 .UNSPECIFIED.);
#6770=B_SPLINE_CURVE_WITH_KNOTS('',3,(#293605,#293606,#293607,#293608,#293609,
#293610,#293611,#293612,#293613,#293614,#293615,#293616,#293617,#293618,
#293619,#293620,#293621,#293622,#293623,#293624,#293625,#293626,#293627,
#293628,#293629,#293630,#293631,#293632,#293633,#293634,#293635,#293636,
#293637,#293638,#293639,#293640),.UNSPECIFIED.,.F.,.F.,(4,2,2,2,2,2,2,2,
2,2,2,2,2,2,2,2,2,4),(109.610952863519,109.790638320685,110.261692394934,
110.732061827133,111.19689695249,111.672103550742,112.137985181828,112.60615820867,
113.081516385384,113.545666191462,114.017791207714,114.486599692481,114.952064672917,
115.428390947034,115.893529453424,116.362766636795,116.836080905819,117.179557539184),
 .UNSPECIFIED.);
#6771=B_SPLINE_CURVE_WITH_KNOTS('',3,(#293645,#293646,#293647,#293648,#293649,
#293650,#293651,#293652,#293653,#293654,#293655,#293656,#293657,#293658,
#293659,#293660,#293661,#293662,#293663,#293664,#293665,#293666,#293667,
#293668,#293669,#293670,#293671,#293672,#293673,#293674,#293675,#293676,
#293677,#293678,#293679,#293680),.UNSPECIFIED.,.F.,.F.,(4,2,2,2,2,2,2,2,
2,2,2,2,2,2,2,2,2,4),(15.1357479359638,15.483569442746,15.9565317531947,
16.4258630167518,16.8908441963327,17.3672728159874,17.8327873664142,18.3013141843795,
18.7735358974931,19.2376068561131,19.7125725507048,20.1808286512787,20.6465127188702,
21.1218087780823,21.5866486252242,22.0566999630034,22.5278361424121,22.7031707982564),
 .UNSPECIFIED.);
#6772=B_SPLINE_CURVE_WITH_KNOTS('',3,(#293681,#293682,#293683,#293684,#293685,
#293686,#293687,#293688,#293689,#293690,#293691,#293692,#293693,#293694,
#293695,#293696,#293697,#293698,#293699,#293700,#293701,#293702,#293703,
#293704,#293705,#293706,#293707,#293708,#293709,#293710,#293711,#293712,
#293713,#293714,#293715,#293716),.UNSPECIFIED.,.F.,.F.,(4,2,2,2,2,2,2,2,
2,2,2,2,2,2,2,2,2,4),(117.179557539184,117.300294191774,117.77357180019,
118.241087915831,118.707473413946,119.184989407627,119.649663411256,120.12002348497,
120.591592365583,121.056153005238,121.53062502556,121.997159979772,122.464629349127,
122.941537765749,123.405800210544,123.877150376116,124.347010613714,124.748512061832),
 .UNSPECIFIED.);
#6773=B_SPLINE_CURVE_WITH_KNOTS('',3,(#293721,#293722,#293723,#293724,#293725,
#293726,#293727,#293728,#293729,#293730,#293731,#293732,#293733,#293734,
#293735,#293736,#293737,#293738,#293739,#293740,#293741,#293742,#293743,
#293744,#293745,#293746,#293747,#293748,#293749,#293750,#293751,#293752,
#293753,#293754,#293755,#293756),.UNSPECIFIED.,.F.,.F.,(4,2,2,2,2,2,2,2,
2,2,2,2,2,2,2,2,2,4),(7.56765982270858,7.97350892375056,8.44309508726157,
8.91456334139144,9.37874929116443,9.85528007747227,10.3228522472463,10.7891984448817,
11.2637785971085,11.7283438168659,12.1996104140286,12.6700700074204,13.1346293640203,
13.6122545095522,14.0787297444021,14.5460088545426,15.0193916841404,15.1357479359638),
 .UNSPECIFIED.);
#6774=B_SPLINE_CURVE_WITH_KNOTS('',3,(#293757,#293758,#293759,#293760,#293761,
#293762,#293763,#293764,#293765,#293766,#293767,#293768,#293769,#293770,
#293771,#293772,#293773,#293774,#293775,#293776,#293777,#293778,#293779,
#293780,#293781,#293782,#293783,#293784,#293785,#293786,#293787,#293788,
#293789,#293790,#293791,#293792),.UNSPECIFIED.,.F.,.F.,(4,2,2,2,2,2,2,2,
2,2,2,2,2,2,2,2,2,4),(124.748512061832,124.811988382779,125.287506788249,
125.753122095665,126.221591824151,126.6962926315,127.16041598402,127.632865894423,
128.101239772114,128.56693763404,129.043601068422,129.50855488633,129.978110384247,
130.450850185154,130.915124226038,131.388743327773,131.855915452059,132.31674072404),
 .UNSPECIFIED.);
#6775=B_SPLINE_CURVE_WITH_KNOTS('',3,(#293797,#293798,#293799,#293800,#293801,
#293802,#293803,#293804,#293805,#293806,#293807,#293808,#293809,#293810,
#293811,#293812,#293813,#293814,#293815,#293816,#293817,#293818,#293819,
#293820,#293821,#293822,#293823,#293824,#293825,#293826,#293827,#293828,
#293829,#293830,#293831,#293832),.UNSPECIFIED.,.F.,.F.,(4,2,2,2,2,2,2,2,
2,2,2,2,2,2,2,2,2,4),(9.99999998750232E-7,0.467334061734382,0.932035384281994,
1.40579202308201,1.87007446664982,2.3425110483518,2.81219352801155,3.27703519012564,
3.75383474865014,4.21962567702159,4.68776432105674,5.16034500528953,5.62443429016073,
6.0987886077358,6.56737603804431,7.0328381371557,7.50848165018001,7.56765982270858),
 .UNSPECIFIED.);
#6776=B_SPLINE_CURVE_WITH_KNOTS('',3,(#293833,#293834,#293835,#293836,#293837,
#293838,#293839,#293840,#293841,#293842,#293843,#293844,#293845,#293846,
#293847,#293848,#293849,#293850,#293851,#293852,#293853,#293854,#293855,
#293856,#293857,#293858,#293859,#293860,#293861,#293862,#293863,#293864,
#293865,#293866,#293867,#293868,#293869,#293870),.UNSPECIFIED.,.F.,.F.,
(4,2,2,2,2,2,2,2,2,2,2,2,2,2,2,2,2,2,4),(132.31674072404,132.322614006903,
132.800480328936,133.265055617999,133.73574449305,134.206839604717,134.671541151825,
135.14636009418,135.612648248539,136.080451677917,136.556737472824,137.020978236111,
137.492693772341,137.962137920711,138.427346634022,138.903245442099,139.368685915427,
139.837519056432,139.886098987271),.UNSPECIFIED.);
#6777=B_SPLINE_CURVE_WITH_KNOTS('',3,(#293873,#293874,#293875,#293876,#293877,
#293878,#293879,#293880),.UNSPECIFIED.,.F.,.F.,(4,2,2,4),(139.886098987271,
140.311661019487,140.573832875075,140.83351486988),.UNSPECIFIED.);
#6778=B_SPLINE_CURVE_WITH_KNOTS('',3,(#293884,#293885,#293886,#293887,#293888,
#293889,#293890,#293891,#293892,#293893,#293894,#293895,#293896,#293897,
#293898,#293899,#293900,#293901),.UNSPECIFIED.,.F.,.F.,(4,2,2,2,2,2,2,2,
4),(9.99999997069479E-7,0.291089014559669,0.5781604735274,0.773666909719169,
1.23141972216497,1.66182200097359,2.04579418676715,2.48304347384049,2.8013006831538),
 .UNSPECIFIED.);
#6779=B_SPLINE_CURVE_WITH_KNOTS('',3,(#293906,#293907,#293908,#293909,#293910,
#293911,#293912,#293913,#293914,#293915,#293916,#293917,#293918,#293919,
#293920,#293921,#293922,#293923,#293924,#293925,#293926,#293927,#293928,
#293929,#293930,#293931),.UNSPECIFIED.,.F.,.F.,(4,2,2,2,2,2,2,2,2,2,2,2,
4),(2.8013006831538,2.95750567567089,3.42207211239295,3.6534557788092,4.11157474291367,
4.54312783084037,4.99497502157467,5.49320161115939,6.01905209027688,6.51964999377779,
7.02384354840784,7.35807870641489,7.69625303519648),.UNSPECIFIED.);
#6780=B_SPLINE_CURVE_WITH_KNOTS('',3,(#293934,#293935,#293936,#293937,#293938,
#293939,#293940,#293941,#293942,#293943,#293944,#293945),.UNSPECIFIED.,
 .F.,.F.,(4,2,2,2,2,4),(0.,0.283334890257164,0.52169392280916,0.820631417753867,
1.09721857907454,1.42693465649552),.UNSPECIFIED.);
#6781=B_SPLINE_CURVE_WITH_KNOTS('',3,(#293949,#293950,#293951,#293952,#293953,
#293954,#293955,#293956,#293957,#293958),.UNSPECIFIED.,.F.,.F.,(4,2,2,2,
4),(6.45298424781494,6.58701147725645,7.0135559745479,7.32969503217713,
7.63409751686082),.UNSPECIFIED.);
#6782=B_SPLINE_CURVE_WITH_KNOTS('',3,(#293961,#293962,#293963,#293964,#293965,
#293966,#293967,#293968,#293969,#293970,#293971,#293972,#293973,#293974),
 .UNSPECIFIED.,.F.,.F.,(4,2,2,2,2,2,4),(-2.13428009774412,-1.60549823782287,
-1.17695770942762,-0.961094502946938,-0.74633863203622,-0.362979450140088,
0.),.UNSPECIFIED.);
#6783=B_SPLINE_CURVE_WITH_KNOTS('',3,(#293975,#293976,#293977,#293978,#293979,
#293980,#293981,#293982,#293983,#293984,#293985,#293986,#293987,#293988,
#293989,#293990,#293991,#293992,#293993,#293994,#293995,#293996,#293997,
#293998,#293999,#294000,#294001,#294002,#294003,#294004,#294005,#294006,
#294007,#294008),.UNSPECIFIED.,.F.,.F.,(4,2,2,2,2,2,2,2,2,2,2,2,2,2,2,2,
4),(9.99999953768269E-7,0.370257533413155,0.742867260998573,1.22246490552703,
1.7557170645661,2.25159185055114,2.4791417967581,2.93209432879808,3.15576838975421,
3.59500286984314,4.03092164371551,4.46885846514905,4.94125635881584,5.43523086524786,
5.92378997433212,6.3646784653317,6.45298424781494),.UNSPECIFIED.);
#6784=B_SPLINE_CURVE_WITH_KNOTS('',3,(#294014,#294015,#294016,#294017,#294018,
#294019,#294020,#294021,#294022,#294023,#294024,#294025,#294026,#294027,
#294028,#294029,#294030,#294031,#294032,#294033,#294034,#294035),
 .UNSPECIFIED.,.F.,.F.,(4,2,2,2,2,2,2,2,2,2,4),(91.0207492930948,91.1620889064705,
91.6347282811689,92.1032814796637,92.5691652146226,93.0460199029874,93.5111545444713,
93.9808982819425,94.4538175435407,94.7823719061299,95.1098199853164),
 .UNSPECIFIED.);
#6785=B_SPLINE_CURVE_WITH_KNOTS('',3,(#294038,#294039,#294040,#294041,#294042,
#294043,#294044,#294045,#294046,#294047,#294048,#294049,#294050,#294051,
#294052,#294053),.UNSPECIFIED.,.F.,.F.,(4,2,2,2,2,2,2,4),(9.99999994972016E-7,
0.464678467060016,0.930253604102473,1.399457943134,1.86474545923474,2.34103365921871,
2.80650042650129,3.14443208990716),.UNSPECIFIED.);
#6786=B_SPLINE_CURVE_WITH_KNOTS('',3,(#296128,#296129,#296130,#296131,#296132,
#296133,#296134,#296135,#296136,#296137,#296138,#296139,#296140,#296141,
#296142,#296143),.UNSPECIFIED.,.F.,.F.,(4,2,2,2,2,2,2,4),(0.,0.225987015547473,
0.464252847533295,0.875453617456248,1.4357921506269,2.26570179526748,2.85663059455104,
3.35180761336525),.UNSPECIFIED.);
#6787=B_SPLINE_CURVE_WITH_KNOTS('',3,(#298233,#298234,#298235,#298236,#298237,
#298238,#298239,#298240,#298241,#298242,#298243,#298244,#298245,#298246,
#298247,#298248,#298249,#298250),.UNSPECIFIED.,.F.,.F.,(4,2,2,2,2,2,2,2,
4),(9.99999986121495E-7,0.329680585623105,0.669907801738523,0.890088500101439,
1.29558589654613,1.65011885938668,1.91244034489391,2.02969065103336,2.13124206648743),
 .UNSPECIFIED.);
#6788=B_SPLINE_CURVE_WITH_KNOTS('',3,(#298430,#298431,#298432,#298433,#298434,
#298435,#298436,#298437,#298438,#298439,#298440,#298441,#298442,#298443,
#298444,#298445),.UNSPECIFIED.,.F.,.F.,(4,2,2,2,2,2,2,4),(1.00000044233709E-6,
0.539370132359783,1.28481747817566,1.98442658665292,2.48325218307673,2.95253551271824,
3.30333512017195,3.64287608445345),.UNSPECIFIED.);
#6789=B_SPLINE_CURVE_WITH_KNOTS('',3,(#298446,#298447,#298448,#298449,#298450,
#298451,#298452,#298453,#298454,#298455,#298456,#298457,#298458,#298459,
#298460,#298461),.UNSPECIFIED.,.F.,.F.,(4,2,2,2,2,2,2,4),(0.,0.238087952519387,
0.476113544168717,1.01011910515244,1.73799046632944,2.30408220983986,2.86072831234553,
3.43288601470779),.UNSPECIFIED.);
#7164=CONICAL_SURFACE('',#104257,12.,0.785398163397447);
#7165=CONICAL_SURFACE('',#104258,13.05,0.785398163397443);
#7166=CONICAL_SURFACE('',#104269,13.05,0.785398163397443);
#7167=CONICAL_SURFACE('',#104271,12.,0.785398163397447);
#7168=CONICAL_SURFACE('',#104293,18.,1.0471975511966);
#7169=CONICAL_SURFACE('',#104294,18.,1.0471975511966);
#7170=CONICAL_SURFACE('',#104295,18.,1.0471975511966);
#7171=CONICAL_SURFACE('',#104296,18.,1.0471975511966);
#7172=CONICAL_SURFACE('',#104297,18.,1.0471975511966);
#7173=CONICAL_SURFACE('',#104298,18.,1.0471975511966);
#7174=CONICAL_SURFACE('',#104299,18.,1.0471975511966);
#7175=CONICAL_SURFACE('',#104300,18.,1.0471975511966);
#7176=CONICAL_SURFACE('',#104301,18.,1.0471975511966);
#7177=CONICAL_SURFACE('',#104302,18.,1.0471975511966);
#7178=CONICAL_SURFACE('',#104303,18.,1.0471975511966);
#7179=CONICAL_SURFACE('',#104304,18.,1.0471975511966);
#7180=CONICAL_SURFACE('',#104334,12.9453125,0.610865238198017);
#7181=CONICAL_SURFACE('',#104336,12.,0.785398163397456);
#7182=CONICAL_SURFACE('',#104350,12.,0.785398163397447);
#7183=CONICAL_SURFACE('',#104429,13.05,0.785398163397443);
#7184=CONICAL_SURFACE('',#104432,9.90000000000002,0.785398163397447);
#7185=CONICAL_SURFACE('',#104464,18.,1.0471975511966);
#7186=CONICAL_SURFACE('',#104465,18.,1.0471975511966);
#7187=CONICAL_SURFACE('',#104466,18.,1.0471975511966);
#7188=CONICAL_SURFACE('',#104467,18.,1.0471975511966);
#7189=CONICAL_SURFACE('',#104468,18.,1.0471975511966);
#7190=CONICAL_SURFACE('',#104469,18.,1.0471975511966);
#7191=CONICAL_SURFACE('',#104470,18.,1.0471975511966);
#7192=CONICAL_SURFACE('',#104471,18.,1.0471975511966);
#7193=CONICAL_SURFACE('',#104472,18.,1.0471975511966);
#7194=CONICAL_SURFACE('',#104473,18.,1.0471975511966);
#7195=CONICAL_SURFACE('',#104474,18.,1.0471975511966);
#7196=CONICAL_SURFACE('',#104475,18.,1.0471975511966);
#7232=SHAPE_REPRESENTATION_RELATIONSHIP('SRR','None',#310905,#7249);
#7249=ADVANCED_BREP_SHAPE_REPRESENTATION('',(#7382,#7383,#12,#7384),#310614);
#7314=STYLED_ITEM('',(#311005),#7382);
#7315=STYLED_ITEM('',(#311005),#7383);
#7316=STYLED_ITEM('',(#311005),#12);
#7317=STYLED_ITEM('',(#311005),#7384);
#7382=MANIFOLD_SOLID_BREP('Body1',#93764);
#7383=MANIFOLD_SOLID_BREP('Body2',#93765);
#7384=MANIFOLD_SOLID_BREP('Body4',#93768);
#7652=FACE_BOUND('',#20035,.T.);
#7653=FACE_BOUND('',#20043,.T.);
#7654=FACE_BOUND('',#20075,.T.);
#7655=FACE_BOUND('',#20079,.T.);
#7656=FACE_BOUND('',#20087,.T.);
#7657=FACE_BOUND('',#20099,.T.);
#7658=FACE_BOUND('',#20174,.T.);
#7659=FACE_BOUND('',#20176,.T.);
#7660=FACE_BOUND('',#20188,.T.);
#7661=FACE_BOUND('',#20217,.T.);
#7662=FACE_BOUND('',#20224,.T.);
#7663=FACE_BOUND('',#20226,.T.);
#7664=FACE_BOUND('',#20229,.T.);
#7665=FACE_BOUND('',#20240,.T.);
#7666=FACE_BOUND('',#20241,.T.);
#7667=FACE_BOUND('',#20242,.T.);
#7668=FACE_BOUND('',#20243,.T.);
#7669=FACE_BOUND('',#20244,.T.);
#7670=FACE_BOUND('',#20245,.T.);
#7671=FACE_BOUND('',#20246,.T.);
#7672=FACE_BOUND('',#20247,.T.);
#7673=FACE_BOUND('',#20248,.T.);
#8569=PLANE('',#104273);
#8570=PLANE('',#104280);
#8571=PLANE('',#104281);
#8572=PLANE('',#104282);
#8573=PLANE('',#104283);
#8574=PLANE('',#104284);
#8575=PLANE('',#104285);
#8576=PLANE('',#104286);
#8577=PLANE('',#104338);
#8578=PLANE('',#104339);
#8579=PLANE('',#104340);
#8580=PLANE('',#104341);
#8581=PLANE('',#104342);
#8582=PLANE('',#104343);
#8583=PLANE('',#104344);
#8584=PLANE('',#104345);
#8585=PLANE('',#104346);
#8586=PLANE('',#104357);
#8587=PLANE('',#104438);
#8588=PLANE('',#104439);
#8589=PLANE('',#104440);
#8590=PLANE('',#104447);
#8591=PLANE('',#104448);
#8592=PLANE('',#104449);
#8593=PLANE('',#104450);
#8594=PLANE('',#104451);
#8595=PLANE('',#104452);
#8596=PLANE('',#104453);
#8597=PLANE('',#104454);
#8598=PLANE('',#104455);
#8599=PLANE('',#104456);
#8600=PLANE('',#104457);
#8601=PLANE('',#104476);
#8602=PLANE('',#104529);
#8603=PLANE('',#104530);
#8604=PLANE('',#104531);
#8605=PLANE('',#104532);
#8606=PLANE('',#104533);
#8607=PLANE('',#104534);
#8608=PLANE('',#104535);
#8609=PLANE('',#104536);
#8610=PLANE('',#104537);
#8611=PLANE('',#104538);
#8612=PLANE('',#104539);
#8613=PLANE('',#104540);
#8614=PLANE('',#104541);
#8615=PLANE('',#104542);
#14018=FACE_OUTER_BOUND('',#20018,.T.);
#14019=FACE_OUTER_BOUND('',#20019,.T.);
#14020=FACE_OUTER_BOUND('',#20020,.T.);
#14021=FACE_OUTER_BOUND('',#20021,.T.);
#14022=FACE_OUTER_BOUND('',#20022,.T.);
#14023=FACE_OUTER_BOUND('',#20023,.T.);
#14024=FACE_OUTER_BOUND('',#20024,.T.);
#14025=FACE_OUTER_BOUND('',#20025,.T.);
#14026=FACE_OUTER_BOUND('',#20026,.T.);
#14027=FACE_OUTER_BOUND('',#20027,.T.);
#14028=FACE_OUTER_BOUND('',#20028,.T.);
#14029=FACE_OUTER_BOUND('',#20029,.T.);
#14030=FACE_OUTER_BOUND('',#20030,.T.);
#14031=FACE_OUTER_BOUND('',#20031,.T.);
#14032=FACE_OUTER_BOUND('',#20032,.T.);
#14033=FACE_OUTER_BOUND('',#20033,.T.);
#14034=FACE_OUTER_BOUND('',#20034,.T.);
#14035=FACE_OUTER_BOUND('',#20036,.T.);
#14036=FACE_OUTER_BOUND('',#20037,.T.);
#14037=FACE_OUTER_BOUND('',#20038,.T.);
#14038=FACE_OUTER_BOUND('',#20039,.T.);
#14039=FACE_OUTER_BOUND('',#20040,.T.);
#14040=FACE_OUTER_BOUND('',#20041,.T.);
#14041=FACE_OUTER_BOUND('',#20042,.T.);
#14042=FACE_OUTER_BOUND('',#20044,.T.);
#14043=FACE_OUTER_BOUND('',#20045,.T.);
#14044=FACE_OUTER_BOUND('',#20046,.T.);
#14045=FACE_OUTER_BOUND('',#20047,.T.);
#14046=FACE_OUTER_BOUND('',#20048,.T.);
#14047=FACE_OUTER_BOUND('',#20049,.T.);
#14048=FACE_OUTER_BOUND('',#20050,.T.);
#14049=FACE_OUTER_BOUND('',#20051,.T.);
#14050=FACE_OUTER_BOUND('',#20052,.T.);
#14051=FACE_OUTER_BOUND('',#20053,.T.);
#14052=FACE_OUTER_BOUND('',#20054,.T.);
#14053=FACE_OUTER_BOUND('',#20055,.T.);
#14054=FACE_OUTER_BOUND('',#20056,.T.);
#14055=FACE_OUTER_BOUND('',#20057,.T.);
#14056=FACE_OUTER_BOUND('',#20058,.T.);
#14057=FACE_OUTER_BOUND('',#20059,.T.);
#14058=FACE_OUTER_BOUND('',#20060,.T.);
#14059=FACE_OUTER_BOUND('',#20061,.T.);
#14060=FACE_OUTER_BOUND('',#20062,.T.);
#14061=FACE_OUTER_BOUND('',#20063,.T.);
#14062=FACE_OUTER_BOUND('',#20064,.T.);
#14063=FACE_OUTER_BOUND('',#20065,.T.);
#14064=FACE_OUTER_BOUND('',#20066,.T.);
#14065=FACE_OUTER_BOUND('',#20067,.T.);
#14066=FACE_OUTER_BOUND('',#20068,.T.);
#14067=FACE_OUTER_BOUND('',#20069,.T.);
#14068=FACE_OUTER_BOUND('',#20070,.T.);
#14069=FACE_OUTER_BOUND('',#20071,.T.);
#14070=FACE_OUTER_BOUND('',#20072,.T.);
#14071=FACE_OUTER_BOUND('',#20073,.T.);
#14072=FACE_OUTER_BOUND('',#20074,.T.);
#14073=FACE_OUTER_BOUND('',#20076,.T.);
#14074=FACE_OUTER_BOUND('',#20077,.T.);
#14075=FACE_OUTER_BOUND('',#20078,.T.);
#14076=FACE_OUTER_BOUND('',#20080,.T.);
#14077=FACE_OUTER_BOUND('',#20081,.T.);
#14078=FACE_OUTER_BOUND('',#20082,.T.);
#14079=FACE_OUTER_BOUND('',#20083,.T.);
#14080=FACE_OUTER_BOUND('',#20084,.T.);
#14081=FACE_OUTER_BOUND('',#20085,.T.);
#14082=FACE_OUTER_BOUND('',#20086,.T.);
#14083=FACE_OUTER_BOUND('',#20088,.T.);
#14084=FACE_OUTER_BOUND('',#20089,.T.);
#14085=FACE_OUTER_BOUND('',#20090,.T.);
#14086=FACE_OUTER_BOUND('',#20091,.T.);
#14087=FACE_OUTER_BOUND('',#20092,.T.);
#14088=FACE_OUTER_BOUND('',#20093,.T.);
#14089=FACE_OUTER_BOUND('',#20094,.T.);
#14090=FACE_OUTER_BOUND('',#20095,.T.);
#14091=FACE_OUTER_BOUND('',#20096,.T.);
#14092=FACE_OUTER_BOUND('',#20097,.T.);
#14093=FACE_OUTER_BOUND('',#20098,.T.);
#14094=FACE_OUTER_BOUND('',#20100,.T.);
#14095=FACE_OUTER_BOUND('',#20101,.T.);
#14096=FACE_OUTER_BOUND('',#20102,.T.);
#14097=FACE_OUTER_BOUND('',#20103,.T.);
#14098=FACE_OUTER_BOUND('',#20104,.T.);
#14099=FACE_OUTER_BOUND('',#20105,.T.);
#14100=FACE_OUTER_BOUND('',#20106,.T.);
#14101=FACE_OUTER_BOUND('',#20107,.T.);
#14102=FACE_OUTER_BOUND('',#20108,.T.);
#14103=FACE_OUTER_BOUND('',#20109,.T.);
#14104=FACE_OUTER_BOUND('',#20110,.T.);
#14105=FACE_OUTER_BOUND('',#20111,.T.);
#14106=FACE_OUTER_BOUND('',#20112,.T.);
#14107=FACE_OUTER_BOUND('',#20113,.T.);
#14108=FACE_OUTER_BOUND('',#20114,.T.);
#14109=FACE_OUTER_BOUND('',#20115,.T.);
#14110=FACE_OUTER_BOUND('',#20116,.T.);
#14111=FACE_OUTER_BOUND('',#20117,.T.);
#14112=FACE_OUTER_BOUND('',#20118,.T.);
#14113=FACE_OUTER_BOUND('',#20119,.T.);
#14114=FACE_OUTER_BOUND('',#20120,.T.);
#14115=FACE_OUTER_BOUND('',#20121,.T.);
#14116=FACE_OUTER_BOUND('',#20122,.T.);
#14117=FACE_OUTER_BOUND('',#20123,.T.);
#14118=FACE_OUTER_BOUND('',#20124,.T.);
#14119=FACE_OUTER_BOUND('',#20125,.T.);
#14120=FACE_OUTER_BOUND('',#20126,.T.);
#14121=FACE_OUTER_BOUND('',#20127,.T.);
#14122=FACE_OUTER_BOUND('',#20128,.T.);
#14123=FACE_OUTER_BOUND('',#20129,.T.);
#14124=FACE_OUTER_BOUND('',#20130,.T.);
#14125=FACE_OUTER_BOUND('',#20131,.T.);
#14126=FACE_OUTER_BOUND('',#20132,.T.);
#14127=FACE_OUTER_BOUND('',#20133,.T.);
#14128=FACE_OUTER_BOUND('',#20134,.T.);
#14129=FACE_OUTER_BOUND('',#20135,.T.);
#14130=FACE_OUTER_BOUND('',#20136,.T.);
#14131=FACE_OUTER_BOUND('',#20137,.T.);
#14132=FACE_OUTER_BOUND('',#20138,.T.);
#14133=FACE_OUTER_BOUND('',#20139,.T.);
#14134=FACE_OUTER_BOUND('',#20140,.T.);
#14135=FACE_OUTER_BOUND('',#20141,.T.);
#14136=FACE_OUTER_BOUND('',#20142,.T.);
#14137=FACE_OUTER_BOUND('',#20143,.T.);
#14138=FACE_OUTER_BOUND('',#20144,.T.);
#14139=FACE_OUTER_BOUND('',#20145,.T.);
#14140=FACE_OUTER_BOUND('',#20146,.T.);
#14141=FACE_OUTER_BOUND('',#20147,.T.);
#14142=FACE_OUTER_BOUND('',#20148,.T.);
#14143=FACE_OUTER_BOUND('',#20149,.T.);
#14144=FACE_OUTER_BOUND('',#20150,.T.);
#14145=FACE_OUTER_BOUND('',#20151,.T.);
#14146=FACE_OUTER_BOUND('',#20152,.T.);
#14147=FACE_OUTER_BOUND('',#20153,.T.);
#14148=FACE_OUTER_BOUND('',#20154,.T.);
#14149=FACE_OUTER_BOUND('',#20155,.T.);
#14150=FACE_OUTER_BOUND('',#20156,.T.);
#14151=FACE_OUTER_BOUND('',#20157,.T.);
#14152=FACE_OUTER_BOUND('',#20158,.T.);
#14153=FACE_OUTER_BOUND('',#20159,.T.);
#14154=FACE_OUTER_BOUND('',#20160,.T.);
#14155=FACE_OUTER_BOUND('',#20161,.T.);
#14156=FACE_OUTER_BOUND('',#20162,.T.);
#14157=FACE_OUTER_BOUND('',#20163,.T.);
#14158=FACE_OUTER_BOUND('',#20164,.T.);
#14159=FACE_OUTER_BOUND('',#20165,.T.);
#14160=FACE_OUTER_BOUND('',#20166,.T.);
#14161=FACE_OUTER_BOUND('',#20167,.T.);
#14162=FACE_OUTER_BOUND('',#20168,.T.);
#14163=FACE_OUTER_BOUND('',#20169,.T.);
#14164=FACE_OUTER_BOUND('',#20170,.T.);
#14165=FACE_OUTER_BOUND('',#20171,.T.);
#14166=FACE_OUTER_BOUND('',#20172,.T.);
#14167=FACE_OUTER_BOUND('',#20173,.T.);
#14168=FACE_OUTER_BOUND('',#20175,.T.);
#14169=FACE_OUTER_BOUND('',#20177,.T.);
#14170=FACE_OUTER_BOUND('',#20178,.T.);
#14171=FACE_OUTER_BOUND('',#20179,.T.);
#14172=FACE_OUTER_BOUND('',#20180,.T.);
#14173=FACE_OUTER_BOUND('',#20181,.T.);
#14174=FACE_OUTER_BOUND('',#20182,.T.);
#14175=FACE_OUTER_BOUND('',#20183,.T.);
#14176=FACE_OUTER_BOUND('',#20184,.T.);
#14177=FACE_OUTER_BOUND('',#20185,.T.);
#14178=FACE_OUTER_BOUND('',#20186,.T.);
#14179=FACE_OUTER_BOUND('',#20187,.T.);
#14180=FACE_OUTER_BOUND('',#20189,.T.);
#14181=FACE_OUTER_BOUND('',#20190,.T.);
#14182=FACE_OUTER_BOUND('',#20191,.T.);
#14183=FACE_OUTER_BOUND('',#20192,.T.);
#14184=FACE_OUTER_BOUND('',#20193,.T.);
#14185=FACE_OUTER_BOUND('',#20194,.T.);
#14186=FACE_OUTER_BOUND('',#20195,.T.);
#14187=FACE_OUTER_BOUND('',#20196,.T.);
#14188=FACE_OUTER_BOUND('',#20197,.T.);
#14189=FACE_OUTER_BOUND('',#20198,.T.);
#14190=FACE_OUTER_BOUND('',#20199,.T.);
#14191=FACE_OUTER_BOUND('',#20200,.T.);
#14192=FACE_OUTER_BOUND('',#20201,.T.);
#14193=FACE_OUTER_BOUND('',#20202,.T.);
#14194=FACE_OUTER_BOUND('',#20203,.T.);
#14195=FACE_OUTER_BOUND('',#20204,.T.);
#14196=FACE_OUTER_BOUND('',#20205,.T.);
#14197=FACE_OUTER_BOUND('',#20206,.T.);
#14198=FACE_OUTER_BOUND('',#20207,.T.);
#14199=FACE_OUTER_BOUND('',#20208,.T.);
#14200=FACE_OUTER_BOUND('',#20209,.T.);
#14201=FACE_OUTER_BOUND('',#20210,.T.);
#14202=FACE_OUTER_BOUND('',#20211,.T.);
#14203=FACE_OUTER_BOUND('',#20212,.T.);
#14204=FACE_OUTER_BOUND('',#20213,.T.);
#14205=FACE_OUTER_BOUND('',#20214,.T.);
#14206=FACE_OUTER_BOUND('',#20215,.T.);
#14207=FACE_OUTER_BOUND('',#20216,.T.);
#14208=FACE_OUTER_BOUND('',#20218,.T.);
#14209=FACE_OUTER_BOUND('',#20219,.T.);
#14210=FACE_OUTER_BOUND('',#20220,.T.);
#14211=FACE_OUTER_BOUND('',#20221,.T.);
#14212=FACE_OUTER_BOUND('',#20222,.T.);
#14213=FACE_OUTER_BOUND('',#20223,.T.);
#14214=FACE_OUTER_BOUND('',#20225,.T.);
#14215=FACE_OUTER_BOUND('',#20227,.T.);
#14216=FACE_OUTER_BOUND('',#20228,.T.);
#14217=FACE_OUTER_BOUND('',#20230,.T.);
#14218=FACE_OUTER_BOUND('',#20231,.T.);
#14219=FACE_OUTER_BOUND('',#20232,.T.);
#14220=FACE_OUTER_BOUND('',#20233,.T.);
#14221=FACE_OUTER_BOUND('',#20234,.T.);
#14222=FACE_OUTER_BOUND('',#20235,.T.);
#14223=FACE_OUTER_BOUND('',#20236,.T.);
#14224=FACE_OUTER_BOUND('',#20237,.T.);
#14225=FACE_OUTER_BOUND('',#20238,.T.);
#14226=FACE_OUTER_BOUND('',#20239,.T.);
#20018=EDGE_LOOP('',(#83715,#83716,#83717));
#20019=EDGE_LOOP('',(#83718,#83719,#83720,#83721,#83722));
#20020=EDGE_LOOP('',(#83723,#83724,#83725,#83726));
#20021=EDGE_LOOP('',(#83727,#83728,#83729,#83730));
#20022=EDGE_LOOP('',(#83731,#83732,#83733,#83734));
#20023=EDGE_LOOP('',(#83735,#83736,#83737));
#20024=EDGE_LOOP('',(#83738,#83739,#83740,#83741));
#20025=EDGE_LOOP('',(#83742,#83743,#83744));
#20026=EDGE_LOOP('',(#83745,#83746,#83747,#83748,#83749));
#20027=EDGE_LOOP('',(#83750,#83751,#83752,#83753));
#20028=EDGE_LOOP('',(#83754,#83755,#83756,#83757));
#20029=EDGE_LOOP('',(#83758,#83759,#83760,#83761));
#20030=EDGE_LOOP('',(#83762,#83763,#83764,#83765));
#20031=EDGE_LOOP('',(#83766,#83767,#83768,#83769));
#20032=EDGE_LOOP('',(#83770,#83771,#83772,#83773,#83774,#83775,#83776,#83777));
#20033=EDGE_LOOP('',(#83778,#83779,#83780,#83781,#83782,#83783,#83784,#83785,
#83786));
#20034=EDGE_LOOP('',(#83787,#83788,#83789,#83790,#83791,#83792));
#20035=EDGE_LOOP('',(#83793));
#20036=EDGE_LOOP('',(#83794,#83795,#83796,#83797,#83798,#83799));
#20037=EDGE_LOOP('',(#83800,#83801,#83802,#83803,#83804,#83805));
#20038=EDGE_LOOP('',(#83806,#83807,#83808,#83809,#83810,#83811));
#20039=EDGE_LOOP('',(#83812,#83813,#83814,#83815,#83816,#83817));
#20040=EDGE_LOOP('',(#83818,#83819,#83820,#83821,#83822,#83823));
#20041=EDGE_LOOP('',(#83824,#83825,#83826,#83827,#83828,#83829));
#20042=EDGE_LOOP('',(#83830,#83831,#83832,#83833,#83834,#83835));
#20043=EDGE_LOOP('',(#83836));
#20044=EDGE_LOOP('',(#83837,#83838,#83839));
#20045=EDGE_LOOP('',(#83840,#83841,#83842));
#20046=EDGE_LOOP('',(#83843,#83844,#83845));
#20047=EDGE_LOOP('',(#83846,#83847,#83848));
#20048=EDGE_LOOP('',(#83849,#83850,#83851));
#20049=EDGE_LOOP('',(#83852,#83853,#83854));
#20050=EDGE_LOOP('',(#83855,#83856,#83857));
#20051=EDGE_LOOP('',(#83858,#83859,#83860));
#20052=EDGE_LOOP('',(#83861,#83862,#83863));
#20053=EDGE_LOOP('',(#83864,#83865,#83866));
#20054=EDGE_LOOP('',(#83867,#83868,#83869));
#20055=EDGE_LOOP('',(#83870,#83871,#83872));
#20056=EDGE_LOOP('',(#83873,#83874,#83875,#83876,#83877,#83878,#83879,#83880,
#83881,#83882,#83883,#83884,#83885,#83886,#83887));
#20057=EDGE_LOOP('',(#83888,#83889,#83890,#83891,#83892,#83893,#83894,#83895,
#83896,#83897,#83898,#83899,#83900,#83901,#83902,#83903,#83904));
#20058=EDGE_LOOP('',(#83905,#83906,#83907,#83908));
#20059=EDGE_LOOP('',(#83909,#83910,#83911,#83912));
#20060=EDGE_LOOP('',(#83913,#83914,#83915,#83916));
#20061=EDGE_LOOP('',(#83917,#83918,#83919,#83920));
#20062=EDGE_LOOP('',(#83921,#83922,#83923,#83924));
#20063=EDGE_LOOP('',(#83925,#83926,#83927,#83928));
#20064=EDGE_LOOP('',(#83929,#83930,#83931));
#20065=EDGE_LOOP('',(#83932,#83933,#83934));
#20066=EDGE_LOOP('',(#83935,#83936,#83937,#83938));
#20067=EDGE_LOOP('',(#83939,#83940,#83941,#83942));
#20068=EDGE_LOOP('',(#83943,#83944,#83945,#83946));
#20069=EDGE_LOOP('',(#83947,#83948,#83949,#83950));
#20070=EDGE_LOOP('',(#83951,#83952,#83953,#83954));
#20071=EDGE_LOOP('',(#83955,#83956,#83957,#83958));
#20072=EDGE_LOOP('',(#83959,#83960,#83961,#83962));
#20073=EDGE_LOOP('',(#83963));
#20074=EDGE_LOOP('',(#83964));
#20075=EDGE_LOOP('',(#83965,#83966,#83967,#83968,#83969,#83970));
#20076=EDGE_LOOP('',(#83971,#83972,#83973,#83974,#83975,#83976,#83977,#83978,
#83979,#83980));
#20077=EDGE_LOOP('',(#83981,#83982,#83983,#83984,#83985,#83986,#83987,#83988));
#20078=EDGE_LOOP('',(#83989));
#20079=EDGE_LOOP('',(#83990));
#20080=EDGE_LOOP('',(#83991,#83992,#83993,#83994));
#20081=EDGE_LOOP('',(#83995,#83996,#83997,#83998));
#20082=EDGE_LOOP('',(#83999,#84000,#84001,#84002));
#20083=EDGE_LOOP('',(#84003,#84004,#84005,#84006));
#20084=EDGE_LOOP('',(#84007,#84008,#84009,#84010));
#20085=EDGE_LOOP('',(#84011,#84012,#84013,#84014,#84015));
#20086=EDGE_LOOP('',(#84016));
#20087=EDGE_LOOP('',(#84017));
#20088=EDGE_LOOP('',(#84018,#84019,#84020,#84021));
#20089=EDGE_LOOP('',(#84022,#84023,#84024,#84025,#84026,#84027,#84028,#84029,
#84030,#84031,#84032,#84033,#84034,#84035,#84036,#84037));
#20090=EDGE_LOOP('',(#84038,#84039,#84040,#84041,#84042,#84043,#84044,#84045,
#84046,#84047,#84048,#84049,#84050,#84051,#84052,#84053,#84054));
#20091=EDGE_LOOP('',(#84055,#84056,#84057,#84058));
#20092=EDGE_LOOP('',(#84059,#84060,#84061,#84062));
#20093=EDGE_LOOP('',(#84063,#84064,#84065,#84066,#84067,#84068,#84069,#84070));
#20094=EDGE_LOOP('',(#84071,#84072,#84073,#84074));
#20095=EDGE_LOOP('',(#84075,#84076,#84077,#84078,#84079));
#20096=EDGE_LOOP('',(#84080,#84081,#84082,#84083,#84084,#84085));
#20097=EDGE_LOOP('',(#84086,#84087,#84088,#84089));
#20098=EDGE_LOOP('',(#84090));
#20099=EDGE_LOOP('',(#84091,#84092,#84093,#84094));
#20100=EDGE_LOOP('',(#84095,#84096,#84097));
#20101=EDGE_LOOP('',(#84098,#84099,#84100,#84101));
#20102=EDGE_LOOP('',(#84102,#84103,#84104,#84105));
#20103=EDGE_LOOP('',(#84106,#84107,#84108,#84109));
#20104=EDGE_LOOP('',(#84110,#84111,#84112,#84113));
#20105=EDGE_LOOP('',(#84114,#84115,#84116,#84117));
#20106=EDGE_LOOP('',(#84118,#84119,#84120,#84121));
#20107=EDGE_LOOP('',(#84122,#84123,#84124,#84125));
#20108=EDGE_LOOP('',(#84126,#84127,#84128,#84129));
#20109=EDGE_LOOP('',(#84130,#84131,#84132,#84133));
#20110=EDGE_LOOP('',(#84134,#84135,#84136,#84137));
#20111=EDGE_LOOP('',(#84138,#84139,#84140,#84141));
#20112=EDGE_LOOP('',(#84142,#84143,#84144,#84145));
#20113=EDGE_LOOP('',(#84146,#84147,#84148,#84149));
#20114=EDGE_LOOP('',(#84150,#84151,#84152,#84153));
#20115=EDGE_LOOP('',(#84154,#84155,#84156,#84157));
#20116=EDGE_LOOP('',(#84158,#84159,#84160,#84161));
#20117=EDGE_LOOP('',(#84162,#84163,#84164,#84165));
#20118=EDGE_LOOP('',(#84166,#84167,#84168,#84169));
#20119=EDGE_LOOP('',(#84170,#84171,#84172,#84173));
#20120=EDGE_LOOP('',(#84174,#84175,#84176,#84177));
#20121=EDGE_LOOP('',(#84178,#84179,#84180,#84181));
#20122=EDGE_LOOP('',(#84182,#84183,#84184,#84185));
#20123=EDGE_LOOP('',(#84186,#84187,#84188,#84189));
#20124=EDGE_LOOP('',(#84190,#84191,#84192,#84193));
#20125=EDGE_LOOP('',(#84194,#84195,#84196,#84197));
#20126=EDGE_LOOP('',(#84198,#84199,#84200,#84201));
#20127=EDGE_LOOP('',(#84202,#84203,#84204,#84205));
#20128=EDGE_LOOP('',(#84206,#84207,#84208,#84209));
#20129=EDGE_LOOP('',(#84210,#84211,#84212,#84213));
#20130=EDGE_LOOP('',(#84214,#84215,#84216,#84217));
#20131=EDGE_LOOP('',(#84218,#84219,#84220,#84221));
#20132=EDGE_LOOP('',(#84222,#84223,#84224,#84225));
#20133=EDGE_LOOP('',(#84226,#84227,#84228,#84229));
#20134=EDGE_LOOP('',(#84230,#84231,#84232,#84233));
#20135=EDGE_LOOP('',(#84234,#84235,#84236,#84237));
#20136=EDGE_LOOP('',(#84238,#84239,#84240,#84241));
#20137=EDGE_LOOP('',(#84242,#84243,#84244,#84245));
#20138=EDGE_LOOP('',(#84246,#84247,#84248,#84249));
#20139=EDGE_LOOP('',(#84250,#84251,#84252,#84253));
#20140=EDGE_LOOP('',(#84254,#84255,#84256,#84257));
#20141=EDGE_LOOP('',(#84258,#84259,#84260,#84261));
#20142=EDGE_LOOP('',(#84262,#84263,#84264,#84265));
#20143=EDGE_LOOP('',(#84266,#84267,#84268,#84269));
#20144=EDGE_LOOP('',(#84270,#84271,#84272,#84273));
#20145=EDGE_LOOP('',(#84274,#84275,#84276,#84277));
#20146=EDGE_LOOP('',(#84278,#84279,#84280,#84281));
#20147=EDGE_LOOP('',(#84282,#84283,#84284,#84285));
#20148=EDGE_LOOP('',(#84286,#84287,#84288,#84289));
#20149=EDGE_LOOP('',(#84290,#84291,#84292,#84293));
#20150=EDGE_LOOP('',(#84294,#84295,#84296,#84297));
#20151=EDGE_LOOP('',(#84298,#84299,#84300,#84301));
#20152=EDGE_LOOP('',(#84302,#84303,#84304,#84305));
#20153=EDGE_LOOP('',(#84306,#84307,#84308,#84309));
#20154=EDGE_LOOP('',(#84310,#84311,#84312,#84313));
#20155=EDGE_LOOP('',(#84314,#84315,#84316,#84317));
#20156=EDGE_LOOP('',(#84318,#84319,#84320,#84321));
#20157=EDGE_LOOP('',(#84322,#84323,#84324,#84325));
#20158=EDGE_LOOP('',(#84326,#84327,#84328,#84329));
#20159=EDGE_LOOP('',(#84330,#84331,#84332,#84333));
#20160=EDGE_LOOP('',(#84334,#84335,#84336,#84337));
#20161=EDGE_LOOP('',(#84338,#84339,#84340,#84341));
#20162=EDGE_LOOP('',(#84342,#84343,#84344,#84345));
#20163=EDGE_LOOP('',(#84346,#84347,#84348,#84349));
#20164=EDGE_LOOP('',(#84350,#84351,#84352,#84353));
#20165=EDGE_LOOP('',(#84354,#84355,#84356));
#20166=EDGE_LOOP('',(#84357,#84358,#84359,#84360,#84361,#84362,#84363,#84364));
#20167=EDGE_LOOP('',(#84365,#84366,#84367,#84368,#84369,#84370,#84371,#84372));
#20168=EDGE_LOOP('',(#84373,#84374,#84375,#84376));
#20169=EDGE_LOOP('',(#84377,#84378,#84379,#84380,#84381,#84382,#84383,#84384,
#84385,#84386,#84387,#84388,#84389,#84390,#84391,#84392,#84393,#84394,#84395,
#84396,#84397,#84398,#84399,#84400,#84401,#84402,#84403,#84404,#84405,#84406,
#84407));
#20170=EDGE_LOOP('',(#84408,#84409,#84410,#84411,#84412,#84413,#84414,#84415,
#84416,#84417,#84418,#84419,#84420,#84421,#84422,#84423,#84424,#84425,#84426,
#84427,#84428,#84429,#84430,#84431,#84432,#84433,#84434,#84435,#84436,#84437));
#20171=EDGE_LOOP('',(#84438,#84439,#84440,#84441));
#20172=EDGE_LOOP('',(#84442));
#20173=EDGE_LOOP('',(#84443,#84444,#84445,#84446));
#20174=EDGE_LOOP('',(#84447,#84448,#84449,#84450));
#20175=EDGE_LOOP('',(#84451,#84452,#84453,#84454));
#20176=EDGE_LOOP('',(#84455,#84456,#84457,#84458,#84459,#84460));
#20177=EDGE_LOOP('',(#84461,#84462,#84463,#84464));
#20178=EDGE_LOOP('',(#84465,#84466,#84467,#84468));
#20179=EDGE_LOOP('',(#84469,#84470,#84471,#84472));
#20180=EDGE_LOOP('',(#84473,#84474,#84475,#84476));
#20181=EDGE_LOOP('',(#84477,#84478,#84479,#84480,#84481,#84482));
#20182=EDGE_LOOP('',(#84483,#84484,#84485,#84486,#84487,#84488));
#20183=EDGE_LOOP('',(#84489,#84490,#84491,#84492,#84493,#84494));
#20184=EDGE_LOOP('',(#84495,#84496,#84497,#84498,#84499,#84500));
#20185=EDGE_LOOP('',(#84501,#84502,#84503,#84504,#84505,#84506));
#20186=EDGE_LOOP('',(#84507,#84508,#84509,#84510,#84511,#84512));
#20187=EDGE_LOOP('',(#84513,#84514,#84515,#84516,#84517,#84518));
#20188=EDGE_LOOP('',(#84519));
#20189=EDGE_LOOP('',(#84520,#84521,#84522));
#20190=EDGE_LOOP('',(#84523,#84524,#84525));
#20191=EDGE_LOOP('',(#84526,#84527,#84528));
#20192=EDGE_LOOP('',(#84529,#84530,#84531));
#20193=EDGE_LOOP('',(#84532,#84533,#84534));
#20194=EDGE_LOOP('',(#84535,#84536,#84537));
#20195=EDGE_LOOP('',(#84538,#84539,#84540));
#20196=EDGE_LOOP('',(#84541,#84542,#84543));
#20197=EDGE_LOOP('',(#84544,#84545,#84546));
#20198=EDGE_LOOP('',(#84547,#84548,#84549));
#20199=EDGE_LOOP('',(#84550,#84551,#84552));
#20200=EDGE_LOOP('',(#84553,#84554,#84555));
#20201=EDGE_LOOP('',(#84556,#84557,#84558,#84559));
#20202=EDGE_LOOP('',(#84560,#84561,#84562,#84563,#84564,#84565,#84566,#84567,
#84568,#84569,#84570,#84571,#84572,#84573,#84574,#84575,#84576,#84577,#84578,
#84579,#84580,#84581,#84582,#84583,#84584,#84585,#84586,#84587,#84588,#84589,
#84590,#84591,#84592,#84593,#84594,#84595,#84596,#84597,#84598,#84599,#84600,
#84601,#84602));
#20203=EDGE_LOOP('',(#84603,#84604,#84605,#84606,#84607,#84608,#84609,#84610,
#84611,#84612,#84613,#84614,#84615,#84616,#84617,#84618,#84619,#84620,#84621,
#84622,#84623,#84624,#84625,#84626,#84627,#84628,#84629,#84630,#84631,#84632,
#84633,#84634,#84635,#84636,#84637,#84638,#84639,#84640,#84641,#84642,#84643,
#84644));
#20204=EDGE_LOOP('',(#84645,#84646,#84647,#84648));
#20205=EDGE_LOOP('',(#84649,#84650,#84651,#84652));
#20206=EDGE_LOOP('',(#84653,#84654,#84655,#84656));
#20207=EDGE_LOOP('',(#84657,#84658,#84659,#84660));
#20208=EDGE_LOOP('',(#84661,#84662,#84663,#84664));
#20209=EDGE_LOOP('',(#84665,#84666,#84667,#84668));
#20210=EDGE_LOOP('',(#84669,#84670,#84671,#84672));
#20211=EDGE_LOOP('',(#84673,#84674,#84675,#84676));
#20212=EDGE_LOOP('',(#84677,#84678,#84679,#84680));
#20213=EDGE_LOOP('',(#84681,#84682,#84683,#84684));
#20214=EDGE_LOOP('',(#84685,#84686,#84687,#84688));
#20215=EDGE_LOOP('',(#84689,#84690,#84691,#84692));
#20216=EDGE_LOOP('',(#84693));
#20217=EDGE_LOOP('',(#84694));
#20218=EDGE_LOOP('',(#84695,#84696,#84697,#84698));
#20219=EDGE_LOOP('',(#84699,#84700,#84701,#84702,#84703));
#20220=EDGE_LOOP('',(#84704,#84705,#84706,#84707,#84708));
#20221=EDGE_LOOP('',(#84709,#84710,#84711,#84712));
#20222=EDGE_LOOP('',(#84713,#84714,#84715,#84716));
#20223=EDGE_LOOP('',(#84717));
#20224=EDGE_LOOP('',(#84718));
#20225=EDGE_LOOP('',(#84719));
#20226=EDGE_LOOP('',(#84720));
#20227=EDGE_LOOP('',(#84721));
#20228=EDGE_LOOP('',(#84722));
#20229=EDGE_LOOP('',(#84723));
#20230=EDGE_LOOP('',(#84724));
#20231=EDGE_LOOP('',(#84725));
#20232=EDGE_LOOP('',(#84726));
#20233=EDGE_LOOP('',(#84727));
#20234=EDGE_LOOP('',(#84728));
#20235=EDGE_LOOP('',(#84729));
#20236=EDGE_LOOP('',(#84730));
#20237=EDGE_LOOP('',(#84731));
#20238=EDGE_LOOP('',(#84732));
#20239=EDGE_LOOP('',(#84733));
#20240=EDGE_LOOP('',(#84734));
#20241=EDGE_LOOP('',(#84735));
#20242=EDGE_LOOP('',(#84736));
#20243=EDGE_LOOP('',(#84737));
#20244=EDGE_LOOP('',(#84738));
#20245=EDGE_LOOP('',(#84739));
#20246=EDGE_LOOP('',(#84740));
#20247=EDGE_LOOP('',(#84741));
#20248=EDGE_LOOP('',(#84742));
#24462=LINE('',#275563,#28809);
#24463=LINE('',#275572,#28810);
#24464=LINE('',#275618,#28811);
#24465=LINE('',#275664,#28812);
#24466=LINE('',#275710,#28813);
#24467=LINE('',#275736,#28814);
#24468=LINE('',#275748,#28815);
#24469=LINE('',#275766,#28816);
#24470=LINE('',#275780,#28817);
#24471=LINE('',#275858,#28818);
#24472=LINE('',#275934,#28819);
#24473=LINE('',#276010,#28820);
#24474=LINE('',#276086,#28821);
#24475=LINE('',#276221,#28822);
#24476=LINE('',#276278,#28823);
#24477=LINE('',#276337,#28824);
#24478=LINE('',#276347,#28825);
#24479=LINE('',#276364,#28826);
#24480=LINE('',#276381,#28827);
#24481=LINE('',#276398,#28828);
#24482=LINE('',#276415,#28829);
#24483=LINE('',#280646,#28830);
#24484=LINE('',#280675,#28831);
#24485=LINE('',#280721,#28832);
#24486=LINE('',#280767,#28833);
#24487=LINE('',#280813,#28834);
#24488=LINE('',#280859,#28835);
#24489=LINE('',#280870,#28836);
#24490=LINE('',#280884,#28837);
#24491=LINE('',#280960,#28838);
#24492=LINE('',#281036,#28839);
#24493=LINE('',#281112,#28840);
#24494=LINE('',#281188,#28841);
#24495=LINE('',#281266,#28842);
#24496=LINE('',#281394,#28843);
#24497=LINE('',#281422,#28844);
#24498=LINE('',#281470,#28845);
#24499=LINE('',#281471,#28846);
#24500=LINE('',#281473,#28847);
#24501=LINE('',#281475,#28848);
#24502=LINE('',#281477,#28849);
#24503=LINE('',#281479,#28850);
#24504=LINE('',#285709,#28851);
#24505=LINE('',#285765,#28852);
#24506=LINE('',#290042,#28853);
#24507=LINE('',#290053,#28854);
#24508=LINE('',#290099,#28855);
#24509=LINE('',#290145,#28856);
#24510=LINE('',#290191,#28857);
#24511=LINE('',#290237,#28858);
#24512=LINE('',#290283,#28859);
#24513=LINE('',#290329,#28860);
#24514=LINE('',#290375,#28861);
#24515=LINE('',#290421,#28862);
#24516=LINE('',#290467,#28863);
#24517=LINE('',#290513,#28864);
#24518=LINE('',#290559,#28865);
#24519=LINE('',#290605,#28866);
#24520=LINE('',#290651,#28867);
#24521=LINE('',#290697,#28868);
#24522=LINE('',#290743,#28869);
#24523=LINE('',#290789,#28870);
#24524=LINE('',#290835,#28871);
#24525=LINE('',#290881,#28872);
#24526=LINE('',#290927,#28873);
#24527=LINE('',#290958,#28874);
#24528=LINE('',#291004,#28875);
#24529=LINE('',#291050,#28876);
#24530=LINE('',#291096,#28877);
#24531=LINE('',#291142,#28878);
#24532=LINE('',#291188,#28879);
#24533=LINE('',#291234,#28880);
#24534=LINE('',#291280,#28881);
#24535=LINE('',#291326,#28882);
#24536=LINE('',#291372,#28883);
#24537=LINE('',#291418,#28884);
#24538=LINE('',#291464,#28885);
#24539=LINE('',#291510,#28886);
#24540=LINE('',#291529,#28887);
#24541=LINE('',#291607,#28888);
#24542=LINE('',#291685,#28889);
#24543=LINE('',#291761,#28890);
#24544=LINE('',#291837,#28891);
#24545=LINE('',#291913,#28892);
#24546=LINE('',#291989,#28893);
#24547=LINE('',#292067,#28894);
#24548=LINE('',#292143,#28895);
#24549=LINE('',#292219,#28896);
#24550=LINE('',#292297,#28897);
#24551=LINE('',#292373,#28898);
#24552=LINE('',#292449,#28899);
#24553=LINE('',#292496,#28900);
#24554=LINE('',#292574,#28901);
#24555=LINE('',#292652,#28902);
#24556=LINE('',#292728,#28903);
#24557=LINE('',#292804,#28904);
#24558=LINE('',#292880,#28905);
#24559=LINE('',#292956,#28906);
#24560=LINE('',#293032,#28907);
#24561=LINE('',#293108,#28908);
#24562=LINE('',#293186,#28909);
#24563=LINE('',#293264,#28910);
#24564=LINE('',#293340,#28911);
#24565=LINE('',#293416,#28912);
#24566=LINE('',#293492,#28913);
#24567=LINE('',#293568,#28914);
#24568=LINE('',#293644,#28915);
#24569=LINE('',#293720,#28916);
#24570=LINE('',#293796,#28917);
#24571=LINE('',#293903,#28918);
#24572=LINE('',#294010,#28919);
#24573=LINE('',#298273,#28920);
#24574=LINE('',#298275,#28921);
#24575=LINE('',#298277,#28922);
#24576=LINE('',#298278,#28923);
#24577=LINE('',#298282,#28924);
#24578=LINE('',#298284,#28925);
#24579=LINE('',#298286,#28926);
#24580=LINE('',#298287,#28927);
#24581=LINE('',#298301,#28928);
#24582=LINE('',#298302,#28929);
#24583=LINE('',#298304,#28930);
#24584=LINE('',#298306,#28931);
#24585=LINE('',#298311,#28932);
#24586=LINE('',#298320,#28933);
#24587=LINE('',#298337,#28934);
#24588=LINE('',#298354,#28935);
#24589=LINE('',#298371,#28936);
#24590=LINE('',#298388,#28937);
#24591=LINE('',#302627,#28938);
#24592=LINE('',#302633,#28939);
#24593=LINE('',#302639,#28940);
#24594=LINE('',#302645,#28941);
#24595=LINE('',#302651,#28942);
#24596=LINE('',#302657,#28943);
#24597=LINE('',#302663,#28944);
#24598=LINE('',#302669,#28945);
#24599=LINE('',#302675,#28946);
#24600=LINE('',#302681,#28947);
#24601=LINE('',#302687,#28948);
#24602=LINE('',#302709,#28949);
#24603=LINE('',#302717,#28950);
#28809=VECTOR('',#129419,10.0514428414941);
#28810=VECTOR('',#129424,10.0514428414941);
#28811=VECTOR('',#129429,10.0514428414941);
#28812=VECTOR('',#129432,10.0514428414941);
#28813=VECTOR('',#129435,10.0514428414941);
#28814=VECTOR('',#129440,12.);
#28815=VECTOR('',#129443,13.05);
#28816=VECTOR('',#129446,12.);
#28817=VECTOR('',#129451,12.);
#28818=VECTOR('',#129456,12.);
#28819=VECTOR('',#129459,12.);
#28820=VECTOR('',#129462,12.);
#28821=VECTOR('',#129465,12.);
#28822=VECTOR('',#129472,13.05);
#28823=VECTOR('',#129477,12.);
#28824=VECTOR('',#129496,1000.);
#28825=VECTOR('',#129497,1000.);
#28826=VECTOR('',#129500,1000.);
#28827=VECTOR('',#129503,1000.);
#28828=VECTOR('',#129506,1000.);
#28829=VECTOR('',#129509,1000.);
#28830=VECTOR('',#129554,10.0514428414941);
#28831=VECTOR('',#129559,10.0514428414941);
#28832=VECTOR('',#129562,10.0514428414941);
#28833=VECTOR('',#129565,10.0514428414941);
#28834=VECTOR('',#129568,10.0514428414941);
#28835=VECTOR('',#129571,10.0514428414941);
#28836=VECTOR('',#129576,12.);
#28837=VECTOR('',#129581,12.);
#28838=VECTOR('',#129584,12.);
#28839=VECTOR('',#129587,12.);
#28840=VECTOR('',#129590,12.);
#28841=VECTOR('',#129593,12.);
#28842=VECTOR('',#129596,12.);
#28843=VECTOR('',#129623,12.9453125);
#28844=VECTOR('',#129628,12.);
#28845=VECTOR('',#129635,1000.);
#28846=VECTOR('',#129636,1000.);
#28847=VECTOR('',#129639,1000.);
#28848=VECTOR('',#129642,1000.);
#28849=VECTOR('',#129645,1000.);
#28850=VECTOR('',#129648,1000.);
#28851=VECTOR('',#129659,10.0514428414941);
#28852=VECTOR('',#129664,12.);
#28853=VECTOR('',#129681,10.0514428414941);
#28854=VECTOR('',#129686,10.0514428414941);
#28855=VECTOR('',#129689,10.0514428414941);
#28856=VECTOR('',#129692,10.0514428414941);
#28857=VECTOR('',#129695,10.0514428414941);
#28858=VECTOR('',#129698,10.0514428414941);
#28859=VECTOR('',#129701,10.0514428414941);
#28860=VECTOR('',#129704,10.0514428414941);
#28861=VECTOR('',#129707,10.0514428414941);
#28862=VECTOR('',#129710,10.0514428414941);
#28863=VECTOR('',#129713,10.0514428414941);
#28864=VECTOR('',#129716,10.0514428414941);
#28865=VECTOR('',#129719,10.0514428414941);
#28866=VECTOR('',#129722,10.0514428414941);
#28867=VECTOR('',#129725,10.0514428414941);
#28868=VECTOR('',#129728,10.0514428414941);
#28869=VECTOR('',#129731,10.0514428414941);
#28870=VECTOR('',#129734,10.0514428414941);
#28871=VECTOR('',#129737,10.0514428414941);
#28872=VECTOR('',#129740,10.0514428414941);
#28873=VECTOR('',#129743,10.0514428414941);
#28874=VECTOR('',#129748,10.0514428414941);
#28875=VECTOR('',#129751,10.0514428414941);
#28876=VECTOR('',#129754,10.0514428414941);
#28877=VECTOR('',#129757,10.0514428414941);
#28878=VECTOR('',#129760,10.0514428414941);
#28879=VECTOR('',#129763,10.0514428414941);
#28880=VECTOR('',#129766,10.0514428414941);
#28881=VECTOR('',#129769,10.0514428414941);
#28882=VECTOR('',#129772,10.0514428414941);
#28883=VECTOR('',#129775,10.0514428414941);
#28884=VECTOR('',#129778,10.0514428414941);
#28885=VECTOR('',#129781,10.0514428414941);
#28886=VECTOR('',#129784,12.);
#28887=VECTOR('',#129789,12.);
#28888=VECTOR('',#129792,12.);
#28889=VECTOR('',#129795,12.);
#28890=VECTOR('',#129798,12.);
#28891=VECTOR('',#129801,12.);
#28892=VECTOR('',#129804,12.);
#28893=VECTOR('',#129807,12.);
#28894=VECTOR('',#129810,12.);
#28895=VECTOR('',#129813,12.);
#28896=VECTOR('',#129816,12.);
#28897=VECTOR('',#129819,12.);
#28898=VECTOR('',#129822,12.);
#28899=VECTOR('',#129825,12.);
#28900=VECTOR('',#129830,12.);
#28901=VECTOR('',#129833,12.);
#28902=VECTOR('',#129836,12.);
#28903=VECTOR('',#129839,12.);
#28904=VECTOR('',#129842,12.);
#28905=VECTOR('',#129845,12.);
#28906=VECTOR('',#129848,12.);
#28907=VECTOR('',#129851,12.);
#28908=VECTOR('',#129854,12.);
#28909=VECTOR('',#129857,12.);
#28910=VECTOR('',#129860,12.);
#28911=VECTOR('',#129863,12.);
#28912=VECTOR('',#129866,12.);
#28913=VECTOR('',#129869,12.);
#28914=VECTOR('',#129872,12.);
#28915=VECTOR('',#129875,12.);
#28916=VECTOR('',#129878,12.);
#28917=VECTOR('',#129881,12.);
#28918=VECTOR('',#129888,13.05);
#28919=VECTOR('',#129897,9.90000000000001);
#28920=VECTOR('',#129910,1000.);
#28921=VECTOR('',#129911,1000.);
#28922=VECTOR('',#129912,1000.);
#28923=VECTOR('',#129913,1000.);
#28924=VECTOR('',#129916,1000.);
#28925=VECTOR('',#129917,1000.);
#28926=VECTOR('',#129918,1000.);
#28927=VECTOR('',#129919,1000.);
#28928=VECTOR('',#129934,1000.);
#28929=VECTOR('',#129935,1000.);
#28930=VECTOR('',#129938,1000.);
#28931=VECTOR('',#129941,1000.);
#28932=VECTOR('',#129946,1000.);
#28933=VECTOR('',#129947,1000.);
#28934=VECTOR('',#129950,1000.);
#28935=VECTOR('',#129953,1000.);
#28936=VECTOR('',#129956,1000.);
#28937=VECTOR('',#129959,1000.);
#28938=VECTOR('',#130008,1.190625);
#28939=VECTOR('',#130015,1.190625);
#28940=VECTOR('',#130022,1.190625);
#28941=VECTOR('',#130029,1.19062499999999);
#28942=VECTOR('',#130036,1.190625);
#28943=VECTOR('',#130043,1.190625);
#28944=VECTOR('',#130050,1.190625);
#28945=VECTOR('',#130057,1.190625);
#28946=VECTOR('',#130064,1.190625);
#28947=VECTOR('',#130071,55.2538194444444);
#28948=VECTOR('',#130078,44.5707880434783);
#28949=VECTOR('',#130107,16.8332621659243);
#28950=VECTOR('',#130118,44.5707880434783);
#34946=CIRCLE('',#104250,10.0514428414941);
#34947=CIRCLE('',#104252,10.0514428414941);
#34948=CIRCLE('',#104256,10.0514428414944);
#34949=CIRCLE('',#104260,12.);
#34950=CIRCLE('',#104262,12.);
#34951=CIRCLE('',#104267,12.);
#34952=CIRCLE('',#104270,13.05);
#34953=CIRCLE('',#104272,13.05);
#34954=CIRCLE('',#104274,18.);
#34955=CIRCLE('',#104275,18.);
#34956=CIRCLE('',#104276,18.);
#34957=CIRCLE('',#104277,18.);
#34958=CIRCLE('',#104278,18.);
#34959=CIRCLE('',#104279,18.);
#34960=CIRCLE('',#104287,18.);
#34961=CIRCLE('',#104288,18.);
#34962=CIRCLE('',#104289,18.);
#34963=CIRCLE('',#104290,18.);
#34964=CIRCLE('',#104291,18.);
#34965=CIRCLE('',#104292,18.);
#34966=CIRCLE('',#104307,10.0514428414941);
#34967=CIRCLE('',#104313,10.0514428414941);
#34968=CIRCLE('',#104315,12.);
#34969=CIRCLE('',#104322,12.);
#34970=CIRCLE('',#104325,44.1739130434783);
#34971=CIRCLE('',#104327,22.0315642065426);
#34972=CIRCLE('',#104328,20.8911550302128);
#34973=CIRCLE('',#104329,20.8911550302128);
#34974=CIRCLE('',#104330,20.8911550302128);
#34975=CIRCLE('',#104331,20.8911550302128);
#34976=CIRCLE('',#104332,20.8911550302128);
#34977=CIRCLE('',#104333,20.8911550302128);
#34978=CIRCLE('',#104335,12.9453125);
#34979=CIRCLE('',#104337,12.525);
#34980=CIRCLE('',#104349,10.0514428414939);
#34981=CIRCLE('',#104351,13.05);
#34982=CIRCLE('',#104352,12.);
#34983=CIRCLE('',#104354,12.);
#34984=CIRCLE('',#104356,10.0514428414941);
#34985=CIRCLE('',#104359,10.0514428414941);
#34986=CIRCLE('',#104380,10.0514428414941);
#34987=CIRCLE('',#104394,12.);
#34988=CIRCLE('',#104408,12.);
#34989=CIRCLE('',#104428,12.);
#34990=CIRCLE('',#104430,13.05);
#34991=CIRCLE('',#104431,10.0514428414942);
#34992=CIRCLE('',#104433,10.0514428414949);
#34993=CIRCLE('',#104434,9.90000000000002);
#34994=CIRCLE('',#104436,12.);
#34995=CIRCLE('',#104441,18.);
#34996=CIRCLE('',#104442,18.);
#34997=CIRCLE('',#104443,18.);
#34998=CIRCLE('',#104444,18.);
#34999=CIRCLE('',#104445,18.);
#35000=CIRCLE('',#104446,18.);
#35001=CIRCLE('',#104458,18.);
#35002=CIRCLE('',#104459,18.);
#35003=CIRCLE('',#104460,18.);
#35004=CIRCLE('',#104461,18.);
#35005=CIRCLE('',#104462,18.);
#35006=CIRCLE('',#104463,18.);
#35007=CIRCLE('',#104479,1.190625);
#35008=CIRCLE('',#104480,1.190625);
#35009=CIRCLE('',#104482,1.190625);
#35010=CIRCLE('',#104483,1.190625);
#35011=CIRCLE('',#104485,1.190625);
#35012=CIRCLE('',#104486,1.190625);
#35013=CIRCLE('',#104488,1.19062499999999);
#35014=CIRCLE('',#104489,1.19062499999999);
#35015=CIRCLE('',#104491,1.190625);
#35016=CIRCLE('',#104492,1.190625);
#35017=CIRCLE('',#104494,1.190625);
#35018=CIRCLE('',#104495,1.190625);
#35019=CIRCLE('',#104497,1.190625);
#35020=CIRCLE('',#104498,1.190625);
#35021=CIRCLE('',#104500,1.190625);
#35022=CIRCLE('',#104501,1.190625);
#35023=CIRCLE('',#104503,1.190625);
#35024=CIRCLE('',#104504,1.190625);
#35025=CIRCLE('',#104506,55.2538194444444);
#35026=CIRCLE('',#104507,55.2538194444444);
#35027=CIRCLE('',#104509,44.5707880434783);
#35028=CIRCLE('',#104510,44.5707880434783);
#35029=CIRCLE('',#104512,22.4667164334275);
#35030=CIRCLE('',#104513,16.8332621659243);
#35031=CIRCLE('',#104515,44.5707880434783);
#35032=CIRCLE('',#104516,0.396875);
#35033=CIRCLE('',#104517,44.9676630434783);
#35034=CIRCLE('',#104519,17.2301371659243);
#35035=CIRCLE('',#104520,0.396875);
#35036=CIRCLE('',#104521,16.8332621659243);
#35037=CIRCLE('',#104522,16.8332621659243);
#35038=CIRCLE('',#104525,43.9357880434783);
#35039=CIRCLE('',#104526,0.635000000000001);
#35040=CIRCLE('',#104527,44.5707880434783);
#42949=VERTEX_POINT('',#275561);
#42950=VERTEX_POINT('',#275562);
#42951=VERTEX_POINT('',#275564);
#42952=VERTEX_POINT('',#275570);
#42953=VERTEX_POINT('',#275571);
#42954=VERTEX_POINT('',#275573);
#42955=VERTEX_POINT('',#275616);
#42956=VERTEX_POINT('',#275617);
#42957=VERTEX_POINT('',#275662);
#42958=VERTEX_POINT('',#275663);
#42959=VERTEX_POINT('',#275708);
#42960=VERTEX_POINT('',#275709);
#42961=VERTEX_POINT('',#275711);
#42962=VERTEX_POINT('',#275721);
#42963=VERTEX_POINT('',#275735);
#42964=VERTEX_POINT('',#275746);
#42965=VERTEX_POINT('',#275747);
#42966=VERTEX_POINT('',#275764);
#42967=VERTEX_POINT('',#275765);
#42968=VERTEX_POINT('',#275767);
#42969=VERTEX_POINT('',#275778);
#42970=VERTEX_POINT('',#275779);
#42971=VERTEX_POINT('',#275781);
#42972=VERTEX_POINT('',#275856);
#42973=VERTEX_POINT('',#275857);
#42974=VERTEX_POINT('',#275932);
#42975=VERTEX_POINT('',#275933);
#42976=VERTEX_POINT('',#276008);
#42977=VERTEX_POINT('',#276009);
#42978=VERTEX_POINT('',#276084);
#42979=VERTEX_POINT('',#276085);
#42980=VERTEX_POINT('',#276087);
#42981=VERTEX_POINT('',#276108);
#42982=VERTEX_POINT('',#276220);
#42983=VERTEX_POINT('',#276272);
#42984=VERTEX_POINT('',#276277);
#42985=VERTEX_POINT('',#276319);
#42986=VERTEX_POINT('',#276320);
#42987=VERTEX_POINT('',#276322);
#42988=VERTEX_POINT('',#276324);
#42989=VERTEX_POINT('',#276326);
#42990=VERTEX_POINT('',#276328);
#42991=VERTEX_POINT('',#276332);
#42992=VERTEX_POINT('',#276336);
#42993=VERTEX_POINT('',#276338);
#42994=VERTEX_POINT('',#276342);
#42995=VERTEX_POINT('',#276346);
#42996=VERTEX_POINT('',#276355);
#42997=VERTEX_POINT('',#276359);
#42998=VERTEX_POINT('',#276363);
#42999=VERTEX_POINT('',#276372);
#43000=VERTEX_POINT('',#276376);
#43001=VERTEX_POINT('',#276380);
#43002=VERTEX_POINT('',#276389);
#43003=VERTEX_POINT('',#276393);
#43004=VERTEX_POINT('',#276397);
#43005=VERTEX_POINT('',#276406);
#43006=VERTEX_POINT('',#276410);
#43007=VERTEX_POINT('',#276414);
#43008=VERTEX_POINT('',#276423);
#43009=VERTEX_POINT('',#280644);
#43010=VERTEX_POINT('',#280645);
#43011=VERTEX_POINT('',#280647);
#43012=VERTEX_POINT('',#280657);
#43013=VERTEX_POINT('',#280673);
#43014=VERTEX_POINT('',#280674);
#43015=VERTEX_POINT('',#280719);
#43016=VERTEX_POINT('',#280720);
#43017=VERTEX_POINT('',#280765);
#43018=VERTEX_POINT('',#280766);
#43019=VERTEX_POINT('',#280811);
#43020=VERTEX_POINT('',#280812);
#43021=VERTEX_POINT('',#280857);
#43022=VERTEX_POINT('',#280858);
#43023=VERTEX_POINT('',#280860);
#43024=VERTEX_POINT('',#280868);
#43025=VERTEX_POINT('',#280869);
#43026=VERTEX_POINT('',#280871);
#43027=VERTEX_POINT('',#280882);
#43028=VERTEX_POINT('',#280883);
#43029=VERTEX_POINT('',#280958);
#43030=VERTEX_POINT('',#280959);
#43031=VERTEX_POINT('',#281034);
#43032=VERTEX_POINT('',#281035);
#43033=VERTEX_POINT('',#281110);
#43034=VERTEX_POINT('',#281111);
#43035=VERTEX_POINT('',#281186);
#43036=VERTEX_POINT('',#281187);
#43037=VERTEX_POINT('',#281264);
#43038=VERTEX_POINT('',#281265);
#43039=VERTEX_POINT('',#281267);
#43040=VERTEX_POINT('',#281272);
#43041=VERTEX_POINT('',#281358);
#43042=VERTEX_POINT('',#281361);
#43043=VERTEX_POINT('',#281363);
#43044=VERTEX_POINT('',#281364);
#43045=VERTEX_POINT('',#281366);
#43046=VERTEX_POINT('',#281368);
#43047=VERTEX_POINT('',#281370);
#43048=VERTEX_POINT('',#281372);
#43049=VERTEX_POINT('',#281376);
#43050=VERTEX_POINT('',#281377);
#43051=VERTEX_POINT('',#281381);
#43052=VERTEX_POINT('',#281385);
#43053=VERTEX_POINT('',#281389);
#43054=VERTEX_POINT('',#281393);
#43055=VERTEX_POINT('',#281396);
#43056=VERTEX_POINT('',#281400);
#43057=VERTEX_POINT('',#281408);
#43058=VERTEX_POINT('',#281421);
#43059=VERTEX_POINT('',#285707);
#43060=VERTEX_POINT('',#285708);
#43061=VERTEX_POINT('',#285710);
#43062=VERTEX_POINT('',#285724);
#43063=VERTEX_POINT('',#285738);
#43064=VERTEX_POINT('',#285739);
#43065=VERTEX_POINT('',#285764);
#43066=VERTEX_POINT('',#285787);
#43067=VERTEX_POINT('',#285802);
#43068=VERTEX_POINT('',#285803);
#43069=VERTEX_POINT('',#287902);
#43070=VERTEX_POINT('',#290006);
#43071=VERTEX_POINT('',#290040);
#43072=VERTEX_POINT('',#290041);
#43073=VERTEX_POINT('',#290043);
#43074=VERTEX_POINT('',#290051);
#43075=VERTEX_POINT('',#290052);
#43076=VERTEX_POINT('',#290097);
#43077=VERTEX_POINT('',#290098);
#43078=VERTEX_POINT('',#290143);
#43079=VERTEX_POINT('',#290144);
#43080=VERTEX_POINT('',#290189);
#43081=VERTEX_POINT('',#290190);
#43082=VERTEX_POINT('',#290235);
#43083=VERTEX_POINT('',#290236);
#43084=VERTEX_POINT('',#290281);
#43085=VERTEX_POINT('',#290282);
#43086=VERTEX_POINT('',#290327);
#43087=VERTEX_POINT('',#290328);
#43088=VERTEX_POINT('',#290373);
#43089=VERTEX_POINT('',#290374);
#43090=VERTEX_POINT('',#290419);
#43091=VERTEX_POINT('',#290420);
#43092=VERTEX_POINT('',#290465);
#43093=VERTEX_POINT('',#290466);
#43094=VERTEX_POINT('',#290511);
#43095=VERTEX_POINT('',#290512);
#43096=VERTEX_POINT('',#290557);
#43097=VERTEX_POINT('',#290558);
#43098=VERTEX_POINT('',#290603);
#43099=VERTEX_POINT('',#290604);
#43100=VERTEX_POINT('',#290649);
#43101=VERTEX_POINT('',#290650);
#43102=VERTEX_POINT('',#290695);
#43103=VERTEX_POINT('',#290696);
#43104=VERTEX_POINT('',#290741);
#43105=VERTEX_POINT('',#290742);
#43106=VERTEX_POINT('',#290787);
#43107=VERTEX_POINT('',#290788);
#43108=VERTEX_POINT('',#290833);
#43109=VERTEX_POINT('',#290834);
#43110=VERTEX_POINT('',#290879);
#43111=VERTEX_POINT('',#290880);
#43112=VERTEX_POINT('',#290925);
#43113=VERTEX_POINT('',#290926);
#43114=VERTEX_POINT('',#290928);
#43115=VERTEX_POINT('',#290942);
#43116=VERTEX_POINT('',#290956);
#43117=VERTEX_POINT('',#290957);
#43118=VERTEX_POINT('',#291002);
#43119=VERTEX_POINT('',#291003);
#43120=VERTEX_POINT('',#291048);
#43121=VERTEX_POINT('',#291049);
#43122=VERTEX_POINT('',#291094);
#43123=VERTEX_POINT('',#291095);
#43124=VERTEX_POINT('',#291140);
#43125=VERTEX_POINT('',#291141);
#43126=VERTEX_POINT('',#291186);
#43127=VERTEX_POINT('',#291187);
#43128=VERTEX_POINT('',#291232);
#43129=VERTEX_POINT('',#291233);
#43130=VERTEX_POINT('',#291278);
#43131=VERTEX_POINT('',#291279);
#43132=VERTEX_POINT('',#291324);
#43133=VERTEX_POINT('',#291325);
#43134=VERTEX_POINT('',#291370);
#43135=VERTEX_POINT('',#291371);
#43136=VERTEX_POINT('',#291416);
#43137=VERTEX_POINT('',#291417);
#43138=VERTEX_POINT('',#291462);
#43139=VERTEX_POINT('',#291463);
#43140=VERTEX_POINT('',#291508);
#43141=VERTEX_POINT('',#291509);
#43142=VERTEX_POINT('',#291511);
#43143=VERTEX_POINT('',#291520);
#43144=VERTEX_POINT('',#291527);
#43145=VERTEX_POINT('',#291528);
#43146=VERTEX_POINT('',#291605);
#43147=VERTEX_POINT('',#291606);
#43148=VERTEX_POINT('',#291683);
#43149=VERTEX_POINT('',#291684);
#43150=VERTEX_POINT('',#291759);
#43151=VERTEX_POINT('',#291760);
#43152=VERTEX_POINT('',#291835);
#43153=VERTEX_POINT('',#291836);
#43154=VERTEX_POINT('',#291911);
#43155=VERTEX_POINT('',#291912);
#43156=VERTEX_POINT('',#291987);
#43157=VERTEX_POINT('',#291988);
#43158=VERTEX_POINT('',#292065);
#43159=VERTEX_POINT('',#292066);
#43160=VERTEX_POINT('',#292141);
#43161=VERTEX_POINT('',#292142);
#43162=VERTEX_POINT('',#292217);
#43163=VERTEX_POINT('',#292218);
#43164=VERTEX_POINT('',#292295);
#43165=VERTEX_POINT('',#292296);
#43166=VERTEX_POINT('',#292371);
#43167=VERTEX_POINT('',#292372);
#43168=VERTEX_POINT('',#292447);
#43169=VERTEX_POINT('',#292448);
#43170=VERTEX_POINT('',#292450);
#43171=VERTEX_POINT('',#292473);
#43172=VERTEX_POINT('',#292494);
#43173=VERTEX_POINT('',#292495);
#43174=VERTEX_POINT('',#292572);
#43175=VERTEX_POINT('',#292573);
#43176=VERTEX_POINT('',#292650);
#43177=VERTEX_POINT('',#292651);
#43178=VERTEX_POINT('',#292726);
#43179=VERTEX_POINT('',#292727);
#43180=VERTEX_POINT('',#292802);
#43181=VERTEX_POINT('',#292803);
#43182=VERTEX_POINT('',#292878);
#43183=VERTEX_POINT('',#292879);
#43184=VERTEX_POINT('',#292954);
#43185=VERTEX_POINT('',#292955);
#43186=VERTEX_POINT('',#293030);
#43187=VERTEX_POINT('',#293031);
#43188=VERTEX_POINT('',#293106);
#43189=VERTEX_POINT('',#293107);
#43190=VERTEX_POINT('',#293184);
#43191=VERTEX_POINT('',#293185);
#43192=VERTEX_POINT('',#293262);
#43193=VERTEX_POINT('',#293263);
#43194=VERTEX_POINT('',#293338);
#43195=VERTEX_POINT('',#293339);
#43196=VERTEX_POINT('',#293414);
#43197=VERTEX_POINT('',#293415);
#43198=VERTEX_POINT('',#293490);
#43199=VERTEX_POINT('',#293491);
#43200=VERTEX_POINT('',#293566);
#43201=VERTEX_POINT('',#293567);
#43202=VERTEX_POINT('',#293642);
#43203=VERTEX_POINT('',#293643);
#43204=VERTEX_POINT('',#293718);
#43205=VERTEX_POINT('',#293719);
#43206=VERTEX_POINT('',#293794);
#43207=VERTEX_POINT('',#293795);
#43208=VERTEX_POINT('',#293872);
#43209=VERTEX_POINT('',#293883);
#43210=VERTEX_POINT('',#293902);
#43211=VERTEX_POINT('',#293905);
#43212=VERTEX_POINT('',#293932);
#43213=VERTEX_POINT('',#293947);
#43214=VERTEX_POINT('',#293948);
#43215=VERTEX_POINT('',#293959);
#43216=VERTEX_POINT('',#294009);
#43217=VERTEX_POINT('',#294013);
#43218=VERTEX_POINT('',#294036);
#43219=VERTEX_POINT('',#298271);
#43220=VERTEX_POINT('',#298272);
#43221=VERTEX_POINT('',#298274);
#43222=VERTEX_POINT('',#298276);
#43223=VERTEX_POINT('',#298280);
#43224=VERTEX_POINT('',#298281);
#43225=VERTEX_POINT('',#298283);
#43226=VERTEX_POINT('',#298285);
#43227=VERTEX_POINT('',#298288);
#43228=VERTEX_POINT('',#298289);
#43229=VERTEX_POINT('',#298291);
#43230=VERTEX_POINT('',#298293);
#43231=VERTEX_POINT('',#298295);
#43232=VERTEX_POINT('',#298297);
#43233=VERTEX_POINT('',#298309);
#43234=VERTEX_POINT('',#298310);
#43235=VERTEX_POINT('',#298315);
#43236=VERTEX_POINT('',#298319);
#43237=VERTEX_POINT('',#298321);
#43238=VERTEX_POINT('',#298332);
#43239=VERTEX_POINT('',#298336);
#43240=VERTEX_POINT('',#298338);
#43241=VERTEX_POINT('',#298349);
#43242=VERTEX_POINT('',#298353);
#43243=VERTEX_POINT('',#298355);
#43244=VERTEX_POINT('',#298366);
#43245=VERTEX_POINT('',#298370);
#43246=VERTEX_POINT('',#298372);
#43247=VERTEX_POINT('',#298383);
#43248=VERTEX_POINT('',#298387);
#43249=VERTEX_POINT('',#298389);
#43250=VERTEX_POINT('',#298403);
#43251=VERTEX_POINT('',#302624);
#43252=VERTEX_POINT('',#302626);
#43253=VERTEX_POINT('',#302630);
#43254=VERTEX_POINT('',#302632);
#43255=VERTEX_POINT('',#302636);
#43256=VERTEX_POINT('',#302638);
#43257=VERTEX_POINT('',#302642);
#43258=VERTEX_POINT('',#302644);
#43259=VERTEX_POINT('',#302648);
#43260=VERTEX_POINT('',#302650);
#43261=VERTEX_POINT('',#302654);
#43262=VERTEX_POINT('',#302656);
#43263=VERTEX_POINT('',#302660);
#43264=VERTEX_POINT('',#302662);
#43265=VERTEX_POINT('',#302666);
#43266=VERTEX_POINT('',#302668);
#43267=VERTEX_POINT('',#302672);
#43268=VERTEX_POINT('',#302674);
#43269=VERTEX_POINT('',#302678);
#43270=VERTEX_POINT('',#302680);
#43271=VERTEX_POINT('',#302684);
#43272=VERTEX_POINT('',#302686);
#43273=VERTEX_POINT('',#302690);
#43274=VERTEX_POINT('',#302692);
#43275=VERTEX_POINT('',#302695);
#43276=VERTEX_POINT('',#302697);
#43277=VERTEX_POINT('',#302701);
#43278=VERTEX_POINT('',#302703);
#43279=VERTEX_POINT('',#302705);
#43280=VERTEX_POINT('',#302711);
#43281=VERTEX_POINT('',#302713);
#56637=EDGE_CURVE('',#42949,#42950,#24462,.T.);
#56638=EDGE_CURVE('',#42951,#42950,#34946,.T.);
#56639=EDGE_CURVE('',#42949,#42951,#1539,.T.);
#56640=EDGE_CURVE('',#42952,#42953,#24463,.T.);
#56641=EDGE_CURVE('',#42953,#42954,#1540,.T.);
#56642=EDGE_CURVE('',#42950,#42954,#34947,.T.);
#56643=EDGE_CURVE('',#42952,#42949,#1541,.T.);
#56644=EDGE_CURVE('',#42955,#42956,#24464,.T.);
#56645=EDGE_CURVE('',#42956,#42953,#1542,.T.);
#56646=EDGE_CURVE('',#42955,#42952,#1543,.T.);
#56647=EDGE_CURVE('',#42957,#42958,#24465,.T.);
#56648=EDGE_CURVE('',#42958,#42956,#1544,.T.);
#56649=EDGE_CURVE('',#42957,#42955,#1545,.T.);
#56650=EDGE_CURVE('',#42959,#42960,#24466,.T.);
#56651=EDGE_CURVE('',#42961,#42959,#1546,.T.);
#56652=EDGE_CURVE('',#42962,#42961,#34948,.T.);
#56653=EDGE_CURVE('',#42962,#42960,#1547,.T.);
#56654=EDGE_CURVE('',#42950,#42963,#24467,.T.);
#56655=EDGE_CURVE('',#42954,#42963,#6666,.T.);
#56656=EDGE_CURVE('',#42964,#42965,#24468,.T.);
#56657=EDGE_CURVE('',#42964,#42962,#6667,.T.);
#56658=EDGE_CURVE('',#42961,#42965,#6668,.T.);
#56659=EDGE_CURVE('',#42966,#42967,#24469,.T.);
#56660=EDGE_CURVE('',#42968,#42967,#34949,.T.);
#56661=EDGE_CURVE('',#42966,#42968,#6669,.F.);
#56662=EDGE_CURVE('',#42969,#42970,#24470,.T.);
#56663=EDGE_CURVE('',#42971,#42970,#6670,.F.);
#56664=EDGE_CURVE('',#42967,#42971,#34950,.T.);
#56665=EDGE_CURVE('',#42969,#42966,#6671,.F.);
#56666=EDGE_CURVE('',#42972,#42973,#24471,.T.);
#56667=EDGE_CURVE('',#42970,#42973,#6672,.F.);
#56668=EDGE_CURVE('',#42972,#42969,#6673,.F.);
#56669=EDGE_CURVE('',#42974,#42975,#24472,.T.);
#56670=EDGE_CURVE('',#42973,#42975,#6674,.F.);
#56671=EDGE_CURVE('',#42974,#42972,#6675,.F.);
#56672=EDGE_CURVE('',#42976,#42977,#24473,.T.);
#56673=EDGE_CURVE('',#42975,#42977,#6676,.F.);
#56674=EDGE_CURVE('',#42976,#42974,#6677,.F.);
#56675=EDGE_CURVE('',#42978,#42979,#24474,.T.);
#56676=EDGE_CURVE('',#42980,#42978,#6678,.F.);
#56677=EDGE_CURVE('',#42981,#42980,#34951,.T.);
#56678=EDGE_CURVE('',#42979,#42981,#6679,.F.);
#56679=EDGE_CURVE('',#42977,#42979,#6680,.F.);
#56680=EDGE_CURVE('',#42978,#42976,#6681,.F.);
#56681=EDGE_CURVE('',#42965,#42968,#6682,.T.);
#56682=EDGE_CURVE('',#42967,#42982,#24475,.T.);
#56683=EDGE_CURVE('',#42982,#42982,#34952,.T.);
#56684=EDGE_CURVE('',#42971,#42964,#6683,.T.);
#56685=EDGE_CURVE('',#42963,#42981,#6684,.T.);
#56686=EDGE_CURVE('',#42980,#42983,#6685,.T.);
#56687=EDGE_CURVE('',#42983,#42984,#24476,.T.);
#56688=EDGE_CURVE('',#42984,#42984,#34953,.T.);
#56689=EDGE_CURVE('',#42983,#42951,#6686,.T.);
#56690=EDGE_CURVE('',#42985,#42986,#34954,.T.);
#56691=EDGE_CURVE('',#42985,#42987,#34955,.T.);
#56692=EDGE_CURVE('',#42987,#42988,#34956,.T.);
#56693=EDGE_CURVE('',#42988,#42989,#34957,.T.);
#56694=EDGE_CURVE('',#42989,#42990,#34958,.T.);
#56695=EDGE_CURVE('',#42990,#42986,#34959,.T.);
#56696=EDGE_CURVE('',#42991,#42987,#1548,.T.);
#56697=EDGE_CURVE('',#42991,#42992,#24477,.T.);
#56698=EDGE_CURVE('',#42992,#42993,#1549,.T.);
#56699=EDGE_CURVE('',#42993,#42994,#1550,.T.);
#56700=EDGE_CURVE('',#42995,#42994,#24478,.T.);
#56701=EDGE_CURVE('',#42987,#42995,#1551,.T.);
#56702=EDGE_CURVE('',#42995,#42988,#1552,.T.);
#56703=EDGE_CURVE('',#42994,#42996,#1553,.T.);
#56704=EDGE_CURVE('',#42996,#42997,#1554,.T.);
#56705=EDGE_CURVE('',#42998,#42997,#24479,.T.);
#56706=EDGE_CURVE('',#42988,#42998,#1555,.T.);
#56707=EDGE_CURVE('',#42998,#42989,#1556,.T.);
#56708=EDGE_CURVE('',#42997,#42999,#1557,.T.);
#56709=EDGE_CURVE('',#42999,#43000,#1558,.T.);
#56710=EDGE_CURVE('',#43001,#43000,#24480,.T.);
#56711=EDGE_CURVE('',#42989,#43001,#1559,.T.);
#56712=EDGE_CURVE('',#43001,#42990,#1560,.T.);
#56713=EDGE_CURVE('',#43000,#43002,#1561,.T.);
#56714=EDGE_CURVE('',#43002,#43003,#1562,.T.);
#56715=EDGE_CURVE('',#43004,#43003,#24481,.T.);
#56716=EDGE_CURVE('',#42990,#43004,#1563,.T.);
#56717=EDGE_CURVE('',#43004,#42986,#1564,.T.);
#56718=EDGE_CURVE('',#43003,#43005,#1565,.T.);
#56719=EDGE_CURVE('',#43005,#43006,#1566,.T.);
#56720=EDGE_CURVE('',#43007,#43006,#24482,.T.);
#56721=EDGE_CURVE('',#42986,#43007,#1567,.T.);
#56722=EDGE_CURVE('',#43007,#42985,#1568,.T.);
#56723=EDGE_CURVE('',#43006,#43008,#1569,.T.);
#56724=EDGE_CURVE('',#43008,#42992,#1570,.T.);
#56725=EDGE_CURVE('',#42985,#42991,#1571,.T.);
#56726=EDGE_CURVE('',#42993,#43008,#34960,.T.);
#56727=EDGE_CURVE('',#43008,#43005,#34961,.T.);
#56728=EDGE_CURVE('',#43005,#43002,#34962,.T.);
#56729=EDGE_CURVE('',#43002,#42999,#34963,.T.);
#56730=EDGE_CURVE('',#42999,#42996,#34964,.T.);
#56731=EDGE_CURVE('',#42996,#42993,#34965,.T.);
#56732=EDGE_CURVE('',#42960,#42958,#1572,.T.);
#56733=EDGE_CURVE('',#42959,#42957,#1573,.T.);
#56734=EDGE_CURVE('',#43009,#43010,#24483,.T.);
#56735=EDGE_CURVE('',#43010,#43011,#1574,.T.);
#56736=EDGE_CURVE('',#43012,#43011,#34966,.T.);
#56737=EDGE_CURVE('',#43009,#43012,#1575,.T.);
#56738=EDGE_CURVE('',#43013,#43014,#24484,.T.);
#56739=EDGE_CURVE('',#43014,#43010,#1576,.T.);
#56740=EDGE_CURVE('',#43013,#43009,#1577,.T.);
#56741=EDGE_CURVE('',#43015,#43016,#24485,.T.);
#56742=EDGE_CURVE('',#43016,#43014,#1578,.T.);
#56743=EDGE_CURVE('',#43015,#43013,#1579,.T.);
#56744=EDGE_CURVE('',#43017,#43018,#24486,.T.);
#56745=EDGE_CURVE('',#43018,#43016,#1580,.T.);
#56746=EDGE_CURVE('',#43017,#43015,#1581,.T.);
#56747=EDGE_CURVE('',#43019,#43020,#24487,.T.);
#56748=EDGE_CURVE('',#43020,#43018,#1582,.T.);
#56749=EDGE_CURVE('',#43019,#43017,#1583,.T.);
#56750=EDGE_CURVE('',#43021,#43022,#24488,.T.);
#56751=EDGE_CURVE('',#43023,#43021,#34967,.T.);
#56752=EDGE_CURVE('',#43023,#43022,#1584,.T.);
#56753=EDGE_CURVE('',#43024,#43025,#24489,.T.);
#56754=EDGE_CURVE('',#43026,#43025,#34968,.T.);
#56755=EDGE_CURVE('',#43024,#43026,#6687,.F.);
#56756=EDGE_CURVE('',#43027,#43028,#24490,.T.);
#56757=EDGE_CURVE('',#43025,#43028,#6688,.F.);
#56758=EDGE_CURVE('',#43027,#43024,#6689,.F.);
#56759=EDGE_CURVE('',#43029,#43030,#24491,.T.);
#56760=EDGE_CURVE('',#43028,#43030,#6690,.F.);
#56761=EDGE_CURVE('',#43029,#43027,#6691,.F.);
#56762=EDGE_CURVE('',#43031,#43032,#24492,.T.);
#56763=EDGE_CURVE('',#43030,#43032,#6692,.F.);
#56764=EDGE_CURVE('',#43031,#43029,#6693,.F.);
#56765=EDGE_CURVE('',#43033,#43034,#24493,.T.);
#56766=EDGE_CURVE('',#43032,#43034,#6694,.F.);
#56767=EDGE_CURVE('',#43033,#43031,#6695,.F.);
#56768=EDGE_CURVE('',#43035,#43036,#24494,.T.);
#56769=EDGE_CURVE('',#43034,#43036,#6696,.F.);
#56770=EDGE_CURVE('',#43035,#43033,#6697,.F.);
#56771=EDGE_CURVE('',#43037,#43038,#24495,.T.);
#56772=EDGE_CURVE('',#43039,#43037,#6698,.F.);
#56773=EDGE_CURVE('',#43040,#43039,#34969,.T.);
#56774=EDGE_CURVE('',#43038,#43040,#6699,.F.);
#56775=EDGE_CURVE('',#43036,#43038,#6700,.F.);
#56776=EDGE_CURVE('',#43037,#43035,#6701,.F.);
#56777=EDGE_CURVE('',#43041,#43041,#34970,.T.);
#56778=EDGE_CURVE('',#43042,#43042,#34971,.T.);
#56779=EDGE_CURVE('',#43043,#43044,#34972,.T.);
#56780=EDGE_CURVE('',#43045,#43043,#34973,.T.);
#56781=EDGE_CURVE('',#43046,#43045,#34974,.T.);
#56782=EDGE_CURVE('',#43047,#43046,#34975,.T.);
#56783=EDGE_CURVE('',#43048,#43047,#34976,.T.);
#56784=EDGE_CURVE('',#43044,#43048,#34977,.T.);
#56785=EDGE_CURVE('',#43049,#43050,#1585,.F.);
#56786=EDGE_CURVE('',#43050,#43051,#1586,.T.);
#56787=EDGE_CURVE('',#43051,#43052,#1587,.T.);
#56788=EDGE_CURVE('',#43052,#43053,#1588,.T.);
#56789=EDGE_CURVE('',#43053,#43054,#24496,.T.);
#56790=EDGE_CURVE('',#43054,#43054,#34978,.T.);
#56791=EDGE_CURVE('',#43053,#43055,#1589,.T.);
#56792=EDGE_CURVE('',#43055,#43056,#1590,.T.);
#56793=EDGE_CURVE('',#43056,#43049,#1591,.T.);
#56794=EDGE_CURVE('',#43039,#43057,#6702,.T.);
#56795=EDGE_CURVE('',#43057,#43058,#24497,.T.);
#56796=EDGE_CURVE('',#43058,#43058,#34979,.T.);
#56797=EDGE_CURVE('',#43057,#43012,#6703,.T.);
#56798=EDGE_CURVE('',#43011,#43040,#6704,.T.);
#56799=EDGE_CURVE('',#43055,#43043,#24498,.T.);
#56800=EDGE_CURVE('',#43056,#43044,#24499,.T.);
#56801=EDGE_CURVE('',#43049,#43048,#24500,.T.);
#56802=EDGE_CURVE('',#43050,#43047,#24501,.T.);
#56803=EDGE_CURVE('',#43051,#43046,#24502,.T.);
#56804=EDGE_CURVE('',#43052,#43045,#24503,.T.);
#56805=EDGE_CURVE('',#43021,#43026,#6705,.T.);
#56806=EDGE_CURVE('',#43025,#43023,#6706,.T.);
#56807=EDGE_CURVE('',#43022,#43020,#1592,.T.);
#56808=EDGE_CURVE('',#43021,#43019,#1593,.T.);
#56809=EDGE_CURVE('',#43059,#43060,#24504,.T.);
#56810=EDGE_CURVE('',#43061,#43059,#1594,.T.);
#56811=EDGE_CURVE('',#43062,#43061,#34980,.T.);
#56812=EDGE_CURVE('',#43062,#43060,#1595,.T.);
#56813=EDGE_CURVE('',#43063,#43064,#6707,.T.);
#56814=EDGE_CURVE('',#43064,#43065,#24505,.T.);
#56815=EDGE_CURVE('',#43065,#43065,#34981,.T.);
#56816=EDGE_CURVE('',#43064,#43062,#6708,.T.);
#56817=EDGE_CURVE('',#43061,#43066,#6709,.F.);
#56818=EDGE_CURVE('',#43066,#43063,#34982,.T.);
#56819=EDGE_CURVE('',#43067,#43068,#34983,.T.);
#56820=EDGE_CURVE('',#43068,#43063,#1596,.T.);
#56821=EDGE_CURVE('',#43066,#43067,#6710,.F.);
#56822=EDGE_CURVE('',#43059,#43069,#1597,.T.);
#56823=EDGE_CURVE('',#43069,#43067,#6711,.T.);
#56824=EDGE_CURVE('',#43068,#43070,#6712,.T.);
#56825=EDGE_CURVE('',#43060,#43070,#1598,.T.);
#56826=EDGE_CURVE('',#43070,#43069,#34984,.T.);
#56827=EDGE_CURVE('',#43071,#43072,#24506,.T.);
#56828=EDGE_CURVE('',#43073,#43071,#1599,.T.);
#56829=EDGE_CURVE('',#43073,#43072,#34985,.T.);
#56830=EDGE_CURVE('',#43074,#43075,#24507,.T.);
#56831=EDGE_CURVE('',#43071,#43074,#1600,.T.);
#56832=EDGE_CURVE('',#43072,#43075,#1601,.T.);
#56833=EDGE_CURVE('',#43076,#43077,#24508,.T.);
#56834=EDGE_CURVE('',#43074,#43076,#1602,.T.);
#56835=EDGE_CURVE('',#43075,#43077,#1603,.T.);
#56836=EDGE_CURVE('',#43078,#43079,#24509,.T.);
#56837=EDGE_CURVE('',#43076,#43078,#1604,.T.);
#56838=EDGE_CURVE('',#43077,#43079,#1605,.T.);
#56839=EDGE_CURVE('',#43080,#43081,#24510,.T.);
#56840=EDGE_CURVE('',#43078,#43080,#1606,.T.);
#56841=EDGE_CURVE('',#43079,#43081,#1607,.T.);
#56842=EDGE_CURVE('',#43082,#43083,#24511,.T.);
#56843=EDGE_CURVE('',#43080,#43082,#1608,.T.);
#56844=EDGE_CURVE('',#43081,#43083,#1609,.T.);
#56845=EDGE_CURVE('',#43084,#43085,#24512,.T.);
#56846=EDGE_CURVE('',#43082,#43084,#1610,.T.);
#56847=EDGE_CURVE('',#43083,#43085,#1611,.T.);
#56848=EDGE_CURVE('',#43086,#43087,#24513,.T.);
#56849=EDGE_CURVE('',#43084,#43086,#1612,.T.);
#56850=EDGE_CURVE('',#43085,#43087,#1613,.T.);
#56851=EDGE_CURVE('',#43088,#43089,#24514,.T.);
#56852=EDGE_CURVE('',#43086,#43088,#1614,.T.);
#56853=EDGE_CURVE('',#43087,#43089,#1615,.T.);
#56854=EDGE_CURVE('',#43090,#43091,#24515,.T.);
#56855=EDGE_CURVE('',#43088,#43090,#1616,.T.);
#56856=EDGE_CURVE('',#43089,#43091,#1617,.T.);
#56857=EDGE_CURVE('',#43092,#43093,#24516,.T.);
#56858=EDGE_CURVE('',#43090,#43092,#1618,.T.);
#56859=EDGE_CURVE('',#43091,#43093,#1619,.T.);
#56860=EDGE_CURVE('',#43094,#43095,#24517,.T.);
#56861=EDGE_CURVE('',#43092,#43094,#1620,.T.);
#56862=EDGE_CURVE('',#43093,#43095,#1621,.T.);
#56863=EDGE_CURVE('',#43096,#43097,#24518,.T.);
#56864=EDGE_CURVE('',#43094,#43096,#1622,.T.);
#56865=EDGE_CURVE('',#43095,#43097,#1623,.T.);
#56866=EDGE_CURVE('',#43098,#43099,#24519,.T.);
#56867=EDGE_CURVE('',#43096,#43098,#1624,.T.);
#56868=EDGE_CURVE('',#43097,#43099,#1625,.T.);
#56869=EDGE_CURVE('',#43100,#43101,#24520,.T.);
#56870=EDGE_CURVE('',#43098,#43100,#1626,.T.);
#56871=EDGE_CURVE('',#43099,#43101,#1627,.T.);
#56872=EDGE_CURVE('',#43102,#43103,#24521,.T.);
#56873=EDGE_CURVE('',#43100,#43102,#1628,.T.);
#56874=EDGE_CURVE('',#43101,#43103,#1629,.T.);
#56875=EDGE_CURVE('',#43104,#43105,#24522,.T.);
#56876=EDGE_CURVE('',#43102,#43104,#1630,.T.);
#56877=EDGE_CURVE('',#43103,#43105,#1631,.T.);
#56878=EDGE_CURVE('',#43106,#43107,#24523,.T.);
#56879=EDGE_CURVE('',#43104,#43106,#1632,.T.);
#56880=EDGE_CURVE('',#43105,#43107,#1633,.T.);
#56881=EDGE_CURVE('',#43108,#43109,#24524,.T.);
#56882=EDGE_CURVE('',#43106,#43108,#1634,.T.);
#56883=EDGE_CURVE('',#43107,#43109,#1635,.T.);
#56884=EDGE_CURVE('',#43110,#43111,#24525,.T.);
#56885=EDGE_CURVE('',#43108,#43110,#1636,.T.);
#56886=EDGE_CURVE('',#43109,#43111,#1637,.T.);
#56887=EDGE_CURVE('',#43112,#43113,#24526,.T.);
#56888=EDGE_CURVE('',#43114,#43112,#1638,.T.);
#56889=EDGE_CURVE('',#43115,#43114,#34986,.T.);
#56890=EDGE_CURVE('',#43115,#43113,#1639,.T.);
#56891=EDGE_CURVE('',#43116,#43117,#24527,.T.);
#56892=EDGE_CURVE('',#43112,#43116,#1640,.T.);
#56893=EDGE_CURVE('',#43113,#43117,#1641,.T.);
#56894=EDGE_CURVE('',#43118,#43119,#24528,.T.);
#56895=EDGE_CURVE('',#43116,#43118,#1642,.T.);
#56896=EDGE_CURVE('',#43117,#43119,#1643,.T.);
#56897=EDGE_CURVE('',#43120,#43121,#24529,.T.);
#56898=EDGE_CURVE('',#43118,#43120,#1644,.T.);
#56899=EDGE_CURVE('',#43119,#43121,#1645,.T.);
#56900=EDGE_CURVE('',#43122,#43123,#24530,.T.);
#56901=EDGE_CURVE('',#43120,#43122,#1646,.T.);
#56902=EDGE_CURVE('',#43121,#43123,#1647,.T.);
#56903=EDGE_CURVE('',#43124,#43125,#24531,.T.);
#56904=EDGE_CURVE('',#43122,#43124,#1648,.T.);
#56905=EDGE_CURVE('',#43123,#43125,#1649,.T.);
#56906=EDGE_CURVE('',#43126,#43127,#24532,.T.);
#56907=EDGE_CURVE('',#43124,#43126,#1650,.T.);
#56908=EDGE_CURVE('',#43125,#43127,#1651,.T.);
#56909=EDGE_CURVE('',#43128,#43129,#24533,.T.);
#56910=EDGE_CURVE('',#43126,#43128,#1652,.T.);
#56911=EDGE_CURVE('',#43127,#43129,#1653,.T.);
#56912=EDGE_CURVE('',#43130,#43131,#24534,.T.);
#56913=EDGE_CURVE('',#43128,#43130,#1654,.T.);
#56914=EDGE_CURVE('',#43129,#43131,#1655,.T.);
#56915=EDGE_CURVE('',#43132,#43133,#24535,.T.);
#56916=EDGE_CURVE('',#43130,#43132,#1656,.T.);
#56917=EDGE_CURVE('',#43131,#43133,#1657,.T.);
#56918=EDGE_CURVE('',#43134,#43135,#24536,.T.);
#56919=EDGE_CURVE('',#43132,#43134,#1658,.T.);
#56920=EDGE_CURVE('',#43133,#43135,#1659,.T.);
#56921=EDGE_CURVE('',#43136,#43137,#24537,.T.);
#56922=EDGE_CURVE('',#43134,#43136,#1660,.T.);
#56923=EDGE_CURVE('',#43135,#43137,#1661,.T.);
#56924=EDGE_CURVE('',#43138,#43139,#24538,.T.);
#56925=EDGE_CURVE('',#43136,#43138,#1662,.T.);
#56926=EDGE_CURVE('',#43137,#43139,#1663,.T.);
#56927=EDGE_CURVE('',#43140,#43141,#24539,.T.);
#56928=EDGE_CURVE('',#43140,#43142,#6713,.T.);
#56929=EDGE_CURVE('',#43142,#43143,#34987,.T.);
#56930=EDGE_CURVE('',#43143,#43141,#6714,.T.);
#56931=EDGE_CURVE('',#43144,#43145,#24540,.T.);
#56932=EDGE_CURVE('',#43144,#43140,#6715,.T.);
#56933=EDGE_CURVE('',#43141,#43145,#6716,.T.);
#56934=EDGE_CURVE('',#43146,#43147,#24541,.T.);
#56935=EDGE_CURVE('',#43146,#43144,#6717,.T.);
#56936=EDGE_CURVE('',#43145,#43147,#6718,.T.);
#56937=EDGE_CURVE('',#43148,#43149,#24542,.T.);
#56938=EDGE_CURVE('',#43148,#43146,#6719,.T.);
#56939=EDGE_CURVE('',#43147,#43149,#6720,.T.);
#56940=EDGE_CURVE('',#43150,#43151,#24543,.T.);
#56941=EDGE_CURVE('',#43150,#43148,#6721,.T.);
#56942=EDGE_CURVE('',#43149,#43151,#6722,.T.);
#56943=EDGE_CURVE('',#43152,#43153,#24544,.T.);
#56944=EDGE_CURVE('',#43152,#43150,#6723,.T.);
#56945=EDGE_CURVE('',#43151,#43153,#6724,.T.);
#56946=EDGE_CURVE('',#43154,#43155,#24545,.T.);
#56947=EDGE_CURVE('',#43154,#43152,#6725,.T.);
#56948=EDGE_CURVE('',#43153,#43155,#6726,.T.);
#56949=EDGE_CURVE('',#43156,#43157,#24546,.T.);
#56950=EDGE_CURVE('',#43156,#43154,#6727,.T.);
#56951=EDGE_CURVE('',#43155,#43157,#6728,.T.);
#56952=EDGE_CURVE('',#43158,#43159,#24547,.T.);
#56953=EDGE_CURVE('',#43158,#43156,#6729,.T.);
#56954=EDGE_CURVE('',#43157,#43159,#6730,.T.);
#56955=EDGE_CURVE('',#43160,#43161,#24548,.T.);
#56956=EDGE_CURVE('',#43160,#43158,#6731,.T.);
#56957=EDGE_CURVE('',#43159,#43161,#6732,.T.);
#56958=EDGE_CURVE('',#43162,#43163,#24549,.T.);
#56959=EDGE_CURVE('',#43162,#43160,#6733,.T.);
#56960=EDGE_CURVE('',#43161,#43163,#6734,.T.);
#56961=EDGE_CURVE('',#43164,#43165,#24550,.T.);
#56962=EDGE_CURVE('',#43164,#43162,#6735,.T.);
#56963=EDGE_CURVE('',#43163,#43165,#6736,.T.);
#56964=EDGE_CURVE('',#43166,#43167,#24551,.T.);
#56965=EDGE_CURVE('',#43166,#43164,#6737,.T.);
#56966=EDGE_CURVE('',#43165,#43167,#6738,.T.);
#56967=EDGE_CURVE('',#43168,#43169,#24552,.T.);
#56968=EDGE_CURVE('',#43168,#43170,#6739,.T.);
#56969=EDGE_CURVE('',#43171,#43170,#34988,.T.);
#56970=EDGE_CURVE('',#43171,#43169,#6740,.T.);
#56971=EDGE_CURVE('',#43172,#43173,#24553,.T.);
#56972=EDGE_CURVE('',#43172,#43168,#6741,.T.);
#56973=EDGE_CURVE('',#43169,#43173,#6742,.T.);
#56974=EDGE_CURVE('',#43174,#43175,#24554,.T.);
#56975=EDGE_CURVE('',#43174,#43172,#6743,.T.);
#56976=EDGE_CURVE('',#43173,#43175,#6744,.T.);
#56977=EDGE_CURVE('',#43176,#43177,#24555,.T.);
#56978=EDGE_CURVE('',#43176,#43174,#6745,.T.);
#56979=EDGE_CURVE('',#43175,#43177,#6746,.T.);
#56980=EDGE_CURVE('',#43178,#43179,#24556,.T.);
#56981=EDGE_CURVE('',#43178,#43176,#6747,.T.);
#56982=EDGE_CURVE('',#43177,#43179,#6748,.T.);
#56983=EDGE_CURVE('',#43180,#43181,#24557,.T.);
#56984=EDGE_CURVE('',#43180,#43178,#6749,.T.);
#56985=EDGE_CURVE('',#43179,#43181,#6750,.T.);
#56986=EDGE_CURVE('',#43182,#43183,#24558,.T.);
#56987=EDGE_CURVE('',#43182,#43180,#6751,.T.);
#56988=EDGE_CURVE('',#43181,#43183,#6752,.T.);
#56989=EDGE_CURVE('',#43184,#43185,#24559,.T.);
#56990=EDGE_CURVE('',#43184,#43182,#6753,.T.);
#56991=EDGE_CURVE('',#43183,#43185,#6754,.T.);
#56992=EDGE_CURVE('',#43186,#43187,#24560,.T.);
#56993=EDGE_CURVE('',#43186,#43184,#6755,.T.);
#56994=EDGE_CURVE('',#43185,#43187,#6756,.T.);
#56995=EDGE_CURVE('',#43188,#43189,#24561,.T.);
#56996=EDGE_CURVE('',#43188,#43186,#6757,.T.);
#56997=EDGE_CURVE('',#43187,#43189,#6758,.T.);
#56998=EDGE_CURVE('',#43190,#43191,#24562,.T.);
#56999=EDGE_CURVE('',#43190,#43188,#6759,.T.);
#57000=EDGE_CURVE('',#43189,#43191,#6760,.T.);
#57001=EDGE_CURVE('',#43192,#43193,#24563,.T.);
#57002=EDGE_CURVE('',#43192,#43190,#6761,.T.);
#57003=EDGE_CURVE('',#43191,#43193,#6762,.T.);
#57004=EDGE_CURVE('',#43194,#43195,#24564,.T.);
#57005=EDGE_CURVE('',#43194,#43192,#6763,.T.);
#57006=EDGE_CURVE('',#43193,#43195,#6764,.T.);
#57007=EDGE_CURVE('',#43196,#43197,#24565,.T.);
#57008=EDGE_CURVE('',#43196,#43194,#6765,.T.);
#57009=EDGE_CURVE('',#43195,#43197,#6766,.T.);
#57010=EDGE_CURVE('',#43198,#43199,#24566,.T.);
#57011=EDGE_CURVE('',#43198,#43196,#6767,.T.);
#57012=EDGE_CURVE('',#43197,#43199,#6768,.T.);
#57013=EDGE_CURVE('',#43200,#43201,#24567,.T.);
#57014=EDGE_CURVE('',#43200,#43198,#6769,.T.);
#57015=EDGE_CURVE('',#43199,#43201,#6770,.T.);
#57016=EDGE_CURVE('',#43202,#43203,#24568,.T.);
#57017=EDGE_CURVE('',#43202,#43200,#6771,.T.);
#57018=EDGE_CURVE('',#43201,#43203,#6772,.T.);
#57019=EDGE_CURVE('',#43204,#43205,#24569,.T.);
#57020=EDGE_CURVE('',#43204,#43202,#6773,.T.);
#57021=EDGE_CURVE('',#43203,#43205,#6774,.T.);
#57022=EDGE_CURVE('',#43206,#43207,#24570,.T.);
#57023=EDGE_CURVE('',#43206,#43204,#6775,.T.);
#57024=EDGE_CURVE('',#43205,#43207,#6776,.T.);
#57025=EDGE_CURVE('',#43207,#43208,#6777,.T.);
#57026=EDGE_CURVE('',#43208,#43206,#34989,.T.);
#57027=EDGE_CURVE('',#43170,#43209,#6778,.T.);
#57028=EDGE_CURVE('',#43209,#43210,#24571,.T.);
#57029=EDGE_CURVE('',#43210,#43210,#34990,.T.);
#57030=EDGE_CURVE('',#43209,#43211,#6779,.T.);
#57031=EDGE_CURVE('',#43211,#43212,#34991,.T.);
#57032=EDGE_CURVE('',#43212,#43171,#6780,.T.);
#57033=EDGE_CURVE('',#43213,#43214,#6781,.F.);
#57034=EDGE_CURVE('',#43215,#43213,#34992,.T.);
#57035=EDGE_CURVE('',#43143,#43215,#6782,.T.);
#57036=EDGE_CURVE('',#43214,#43142,#6783,.F.);
#57037=EDGE_CURVE('',#43214,#43216,#24572,.T.);
#57038=EDGE_CURVE('',#43216,#43216,#34993,.T.);
#57039=EDGE_CURVE('',#43167,#43217,#6784,.T.);
#57040=EDGE_CURVE('',#43218,#43217,#34994,.T.);
#57041=EDGE_CURVE('',#43218,#43166,#6785,.T.);
#57042=EDGE_CURVE('',#43114,#43218,#6786,.T.);
#57043=EDGE_CURVE('',#43138,#43213,#1664,.T.);
#57044=EDGE_CURVE('',#43217,#43115,#6787,.T.);
#57045=EDGE_CURVE('',#43139,#43215,#1665,.T.);
#57046=EDGE_CURVE('',#43219,#43220,#24573,.T.);
#57047=EDGE_CURVE('',#43220,#43221,#24574,.T.);
#57048=EDGE_CURVE('',#43221,#43222,#24575,.T.);
#57049=EDGE_CURVE('',#43222,#43219,#24576,.T.);
#57050=EDGE_CURVE('',#43223,#43224,#24577,.T.);
#57051=EDGE_CURVE('',#43225,#43223,#24578,.T.);
#57052=EDGE_CURVE('',#43226,#43225,#24579,.T.);
#57053=EDGE_CURVE('',#43224,#43226,#24580,.T.);
#57054=EDGE_CURVE('',#43227,#43228,#34995,.T.);
#57055=EDGE_CURVE('',#43228,#43229,#34996,.T.);
#57056=EDGE_CURVE('',#43229,#43230,#34997,.T.);
#57057=EDGE_CURVE('',#43230,#43231,#34998,.T.);
#57058=EDGE_CURVE('',#43231,#43232,#34999,.T.);
#57059=EDGE_CURVE('',#43232,#43227,#35000,.T.);
#57060=EDGE_CURVE('',#43220,#43224,#24581,.T.);
#57061=EDGE_CURVE('',#43219,#43223,#24582,.T.);
#57062=EDGE_CURVE('',#43221,#43226,#24583,.T.);
#57063=EDGE_CURVE('',#43222,#43225,#24584,.T.);
#57064=EDGE_CURVE('',#43233,#43234,#24585,.T.);
#57065=EDGE_CURVE('',#43234,#43229,#1666,.T.);
#57066=EDGE_CURVE('',#43229,#43235,#1667,.T.);
#57067=EDGE_CURVE('',#43236,#43235,#24586,.T.);
#57068=EDGE_CURVE('',#43237,#43236,#1668,.T.);
#57069=EDGE_CURVE('',#43233,#43237,#1669,.T.);
#57070=EDGE_CURVE('',#43235,#43228,#1670,.T.);
#57071=EDGE_CURVE('',#43228,#43238,#1671,.T.);
#57072=EDGE_CURVE('',#43239,#43238,#24587,.T.);
#57073=EDGE_CURVE('',#43240,#43239,#1672,.T.);
#57074=EDGE_CURVE('',#43236,#43240,#1673,.T.);
#57075=EDGE_CURVE('',#43238,#43227,#1674,.T.);
#57076=EDGE_CURVE('',#43227,#43241,#1675,.T.);
#57077=EDGE_CURVE('',#43242,#43241,#24588,.T.);
#57078=EDGE_CURVE('',#43243,#43242,#1676,.T.);
#57079=EDGE_CURVE('',#43239,#43243,#1677,.T.);
#57080=EDGE_CURVE('',#43241,#43232,#1678,.T.);
#57081=EDGE_CURVE('',#43232,#43244,#1679,.T.);
#57082=EDGE_CURVE('',#43245,#43244,#24589,.T.);
#57083=EDGE_CURVE('',#43246,#43245,#1680,.T.);
#57084=EDGE_CURVE('',#43242,#43246,#1681,.T.);
#57085=EDGE_CURVE('',#43244,#43231,#1682,.T.);
#57086=EDGE_CURVE('',#43231,#43247,#1683,.T.);
#57087=EDGE_CURVE('',#43248,#43247,#24590,.T.);
#57088=EDGE_CURVE('',#43249,#43248,#1684,.T.);
#57089=EDGE_CURVE('',#43245,#43249,#1685,.T.);
#57090=EDGE_CURVE('',#43247,#43230,#1686,.T.);
#57091=EDGE_CURVE('',#43230,#43234,#1687,.T.);
#57092=EDGE_CURVE('',#43250,#43233,#1688,.T.);
#57093=EDGE_CURVE('',#43248,#43250,#1689,.T.);
#57094=EDGE_CURVE('',#43240,#43237,#35001,.T.);
#57095=EDGE_CURVE('',#43240,#43243,#35002,.T.);
#57096=EDGE_CURVE('',#43243,#43246,#35003,.T.);
#57097=EDGE_CURVE('',#43246,#43249,#35004,.T.);
#57098=EDGE_CURVE('',#43249,#43250,#35005,.T.);
#57099=EDGE_CURVE('',#43250,#43237,#35006,.T.);
#57100=EDGE_CURVE('',#43206,#43073,#6788,.T.);
#57101=EDGE_CURVE('',#43072,#43208,#6789,.T.);
#57102=EDGE_CURVE('',#43110,#43211,#1690,.T.);
#57103=EDGE_CURVE('',#43111,#43212,#1691,.T.);
#57104=EDGE_CURVE('',#43251,#43251,#35007,.T.);
#57105=EDGE_CURVE('',#43251,#43252,#24591,.T.);
#57106=EDGE_CURVE('',#43252,#43252,#35008,.T.);
#57107=EDGE_CURVE('',#43253,#43253,#35009,.T.);
#57108=EDGE_CURVE('',#43253,#43254,#24592,.T.);
#57109=EDGE_CURVE('',#43254,#43254,#35010,.T.);
#57110=EDGE_CURVE('',#43255,#43255,#35011,.T.);
#57111=EDGE_CURVE('',#43255,#43256,#24593,.T.);
#57112=EDGE_CURVE('',#43256,#43256,#35012,.T.);
#57113=EDGE_CURVE('',#43257,#43257,#35013,.T.);
#57114=EDGE_CURVE('',#43257,#43258,#24594,.T.);
#57115=EDGE_CURVE('',#43258,#43258,#35014,.T.);
#57116=EDGE_CURVE('',#43259,#43259,#35015,.T.);
#57117=EDGE_CURVE('',#43259,#43260,#24595,.T.);
#57118=EDGE_CURVE('',#43260,#43260,#35016,.T.);
#57119=EDGE_CURVE('',#43261,#43261,#35017,.T.);
#57120=EDGE_CURVE('',#43261,#43262,#24596,.T.);
#57121=EDGE_CURVE('',#43262,#43262,#35018,.T.);
#57122=EDGE_CURVE('',#43263,#43263,#35019,.T.);
#57123=EDGE_CURVE('',#43263,#43264,#24597,.T.);
#57124=EDGE_CURVE('',#43264,#43264,#35020,.T.);
#57125=EDGE_CURVE('',#43265,#43265,#35021,.T.);
#57126=EDGE_CURVE('',#43265,#43266,#24598,.T.);
#57127=EDGE_CURVE('',#43266,#43266,#35022,.T.);
#57128=EDGE_CURVE('',#43267,#43267,#35023,.T.);
#57129=EDGE_CURVE('',#43267,#43268,#24599,.T.);
#57130=EDGE_CURVE('',#43268,#43268,#35024,.T.);
#57131=EDGE_CURVE('',#43269,#43269,#35025,.T.);
#57132=EDGE_CURVE('',#43269,#43270,#24600,.T.);
#57133=EDGE_CURVE('',#43270,#43270,#35026,.T.);
#57134=EDGE_CURVE('',#43271,#43271,#35027,.T.);
#57135=EDGE_CURVE('',#43271,#43272,#24601,.T.);
#57136=EDGE_CURVE('',#43272,#43272,#35028,.T.);
#57137=EDGE_CURVE('',#43273,#43273,#35029,.T.);
#57138=EDGE_CURVE('',#43274,#43274,#35030,.T.);
#57139=EDGE_CURVE('',#43275,#43275,#35031,.T.);
#57140=EDGE_CURVE('',#43275,#43276,#35032,.T.);
#57141=EDGE_CURVE('',#43276,#43276,#35033,.T.);
#57142=EDGE_CURVE('',#43277,#43277,#35034,.T.);
#57143=EDGE_CURVE('',#43277,#43278,#35035,.T.);
#57144=EDGE_CURVE('',#43279,#43278,#35036,.T.);
#57145=EDGE_CURVE('',#43278,#43279,#35037,.T.);
#57146=EDGE_CURVE('',#43274,#43279,#24602,.T.);
#57147=EDGE_CURVE('',#43280,#43280,#35038,.T.);
#57148=EDGE_CURVE('',#43280,#43281,#35039,.T.);
#57149=EDGE_CURVE('',#43281,#43281,#35040,.T.);
#57150=EDGE_CURVE('',#43281,#43275,#24603,.T.);
#83715=ORIENTED_EDGE('',*,*,#56637,.T.);
#83716=ORIENTED_EDGE('',*,*,#56638,.F.);
#83717=ORIENTED_EDGE('',*,*,#56639,.F.);
#83718=ORIENTED_EDGE('',*,*,#56640,.T.);
#83719=ORIENTED_EDGE('',*,*,#56641,.T.);
#83720=ORIENTED_EDGE('',*,*,#56642,.F.);
#83721=ORIENTED_EDGE('',*,*,#56637,.F.);
#83722=ORIENTED_EDGE('',*,*,#56643,.F.);
#83723=ORIENTED_EDGE('',*,*,#56644,.T.);
#83724=ORIENTED_EDGE('',*,*,#56645,.T.);
#83725=ORIENTED_EDGE('',*,*,#56640,.F.);
#83726=ORIENTED_EDGE('',*,*,#56646,.F.);
#83727=ORIENTED_EDGE('',*,*,#56647,.T.);
#83728=ORIENTED_EDGE('',*,*,#56648,.T.);
#83729=ORIENTED_EDGE('',*,*,#56644,.F.);
#83730=ORIENTED_EDGE('',*,*,#56649,.F.);
#83731=ORIENTED_EDGE('',*,*,#56650,.F.);
#83732=ORIENTED_EDGE('',*,*,#56651,.F.);
#83733=ORIENTED_EDGE('',*,*,#56652,.F.);
#83734=ORIENTED_EDGE('',*,*,#56653,.T.);
#83735=ORIENTED_EDGE('',*,*,#56654,.F.);
#83736=ORIENTED_EDGE('',*,*,#56642,.T.);
#83737=ORIENTED_EDGE('',*,*,#56655,.T.);
#83738=ORIENTED_EDGE('',*,*,#56656,.F.);
#83739=ORIENTED_EDGE('',*,*,#56657,.T.);
#83740=ORIENTED_EDGE('',*,*,#56652,.T.);
#83741=ORIENTED_EDGE('',*,*,#56658,.T.);
#83742=ORIENTED_EDGE('',*,*,#56659,.T.);
#83743=ORIENTED_EDGE('',*,*,#56660,.F.);
#83744=ORIENTED_EDGE('',*,*,#56661,.F.);
#83745=ORIENTED_EDGE('',*,*,#56662,.T.);
#83746=ORIENTED_EDGE('',*,*,#56663,.F.);
#83747=ORIENTED_EDGE('',*,*,#56664,.F.);
#83748=ORIENTED_EDGE('',*,*,#56659,.F.);
#83749=ORIENTED_EDGE('',*,*,#56665,.F.);
#83750=ORIENTED_EDGE('',*,*,#56666,.T.);
#83751=ORIENTED_EDGE('',*,*,#56667,.F.);
#83752=ORIENTED_EDGE('',*,*,#56662,.F.);
#83753=ORIENTED_EDGE('',*,*,#56668,.F.);
#83754=ORIENTED_EDGE('',*,*,#56669,.T.);
#83755=ORIENTED_EDGE('',*,*,#56670,.F.);
#83756=ORIENTED_EDGE('',*,*,#56666,.F.);
#83757=ORIENTED_EDGE('',*,*,#56671,.F.);
#83758=ORIENTED_EDGE('',*,*,#56672,.T.);
#83759=ORIENTED_EDGE('',*,*,#56673,.F.);
#83760=ORIENTED_EDGE('',*,*,#56669,.F.);
#83761=ORIENTED_EDGE('',*,*,#56674,.F.);
#83762=ORIENTED_EDGE('',*,*,#56675,.F.);
#83763=ORIENTED_EDGE('',*,*,#56676,.F.);
#83764=ORIENTED_EDGE('',*,*,#56677,.F.);
#83765=ORIENTED_EDGE('',*,*,#56678,.F.);
#83766=ORIENTED_EDGE('',*,*,#56675,.T.);
#83767=ORIENTED_EDGE('',*,*,#56679,.F.);
#83768=ORIENTED_EDGE('',*,*,#56672,.F.);
#83769=ORIENTED_EDGE('',*,*,#56680,.F.);
#83770=ORIENTED_EDGE('',*,*,#56656,.T.);
#83771=ORIENTED_EDGE('',*,*,#56681,.T.);
#83772=ORIENTED_EDGE('',*,*,#56660,.T.);
#83773=ORIENTED_EDGE('',*,*,#56682,.T.);
#83774=ORIENTED_EDGE('',*,*,#56683,.F.);
#83775=ORIENTED_EDGE('',*,*,#56682,.F.);
#83776=ORIENTED_EDGE('',*,*,#56664,.T.);
#83777=ORIENTED_EDGE('',*,*,#56684,.T.);
#83778=ORIENTED_EDGE('',*,*,#56654,.T.);
#83779=ORIENTED_EDGE('',*,*,#56685,.T.);
#83780=ORIENTED_EDGE('',*,*,#56677,.T.);
#83781=ORIENTED_EDGE('',*,*,#56686,.T.);
#83782=ORIENTED_EDGE('',*,*,#56687,.T.);
#83783=ORIENTED_EDGE('',*,*,#56688,.F.);
#83784=ORIENTED_EDGE('',*,*,#56687,.F.);
#83785=ORIENTED_EDGE('',*,*,#56689,.T.);
#83786=ORIENTED_EDGE('',*,*,#56638,.T.);
#83787=ORIENTED_EDGE('',*,*,#56690,.F.);
#83788=ORIENTED_EDGE('',*,*,#56691,.T.);
#83789=ORIENTED_EDGE('',*,*,#56692,.T.);
#83790=ORIENTED_EDGE('',*,*,#56693,.T.);
#83791=ORIENTED_EDGE('',*,*,#56694,.T.);
#83792=ORIENTED_EDGE('',*,*,#56695,.T.);
#83793=ORIENTED_EDGE('',*,*,#56683,.T.);
#83794=ORIENTED_EDGE('',*,*,#56696,.F.);
#83795=ORIENTED_EDGE('',*,*,#56697,.T.);
#83796=ORIENTED_EDGE('',*,*,#56698,.T.);
#83797=ORIENTED_EDGE('',*,*,#56699,.T.);
#83798=ORIENTED_EDGE('',*,*,#56700,.F.);
#83799=ORIENTED_EDGE('',*,*,#56701,.F.);
#83800=ORIENTED_EDGE('',*,*,#56702,.F.);
#83801=ORIENTED_EDGE('',*,*,#56700,.T.);
#83802=ORIENTED_EDGE('',*,*,#56703,.T.);
#83803=ORIENTED_EDGE('',*,*,#56704,.T.);
#83804=ORIENTED_EDGE('',*,*,#56705,.F.);
#83805=ORIENTED_EDGE('',*,*,#56706,.F.);
#83806=ORIENTED_EDGE('',*,*,#56707,.F.);
#83807=ORIENTED_EDGE('',*,*,#56705,.T.);
#83808=ORIENTED_EDGE('',*,*,#56708,.T.);
#83809=ORIENTED_EDGE('',*,*,#56709,.T.);
#83810=ORIENTED_EDGE('',*,*,#56710,.F.);
#83811=ORIENTED_EDGE('',*,*,#56711,.F.);
#83812=ORIENTED_EDGE('',*,*,#56712,.F.);
#83813=ORIENTED_EDGE('',*,*,#56710,.T.);
#83814=ORIENTED_EDGE('',*,*,#56713,.T.);
#83815=ORIENTED_EDGE('',*,*,#56714,.T.);
#83816=ORIENTED_EDGE('',*,*,#56715,.F.);
#83817=ORIENTED_EDGE('',*,*,#56716,.F.);
#83818=ORIENTED_EDGE('',*,*,#56717,.F.);
#83819=ORIENTED_EDGE('',*,*,#56715,.T.);
#83820=ORIENTED_EDGE('',*,*,#56718,.T.);
#83821=ORIENTED_EDGE('',*,*,#56719,.T.);
#83822=ORIENTED_EDGE('',*,*,#56720,.F.);
#83823=ORIENTED_EDGE('',*,*,#56721,.F.);
#83824=ORIENTED_EDGE('',*,*,#56722,.F.);
#83825=ORIENTED_EDGE('',*,*,#56720,.T.);
#83826=ORIENTED_EDGE('',*,*,#56723,.T.);
#83827=ORIENTED_EDGE('',*,*,#56724,.T.);
#83828=ORIENTED_EDGE('',*,*,#56697,.F.);
#83829=ORIENTED_EDGE('',*,*,#56725,.F.);
#83830=ORIENTED_EDGE('',*,*,#56726,.T.);
#83831=ORIENTED_EDGE('',*,*,#56727,.T.);
#83832=ORIENTED_EDGE('',*,*,#56728,.T.);
#83833=ORIENTED_EDGE('',*,*,#56729,.T.);
#83834=ORIENTED_EDGE('',*,*,#56730,.T.);
#83835=ORIENTED_EDGE('',*,*,#56731,.T.);
#83836=ORIENTED_EDGE('',*,*,#56688,.T.);
#83837=ORIENTED_EDGE('',*,*,#56724,.F.);
#83838=ORIENTED_EDGE('',*,*,#56726,.F.);
#83839=ORIENTED_EDGE('',*,*,#56698,.F.);
#83840=ORIENTED_EDGE('',*,*,#56731,.F.);
#83841=ORIENTED_EDGE('',*,*,#56703,.F.);
#83842=ORIENTED_EDGE('',*,*,#56699,.F.);
#83843=ORIENTED_EDGE('',*,*,#56730,.F.);
#83844=ORIENTED_EDGE('',*,*,#56708,.F.);
#83845=ORIENTED_EDGE('',*,*,#56704,.F.);
#83846=ORIENTED_EDGE('',*,*,#56729,.F.);
#83847=ORIENTED_EDGE('',*,*,#56713,.F.);
#83848=ORIENTED_EDGE('',*,*,#56709,.F.);
#83849=ORIENTED_EDGE('',*,*,#56728,.F.);
#83850=ORIENTED_EDGE('',*,*,#56718,.F.);
#83851=ORIENTED_EDGE('',*,*,#56714,.F.);
#83852=ORIENTED_EDGE('',*,*,#56727,.F.);
#83853=ORIENTED_EDGE('',*,*,#56723,.F.);
#83854=ORIENTED_EDGE('',*,*,#56719,.F.);
#83855=ORIENTED_EDGE('',*,*,#56721,.T.);
#83856=ORIENTED_EDGE('',*,*,#56722,.T.);
#83857=ORIENTED_EDGE('',*,*,#56690,.T.);
#83858=ORIENTED_EDGE('',*,*,#56716,.T.);
#83859=ORIENTED_EDGE('',*,*,#56717,.T.);
#83860=ORIENTED_EDGE('',*,*,#56695,.F.);
#83861=ORIENTED_EDGE('',*,*,#56711,.T.);
#83862=ORIENTED_EDGE('',*,*,#56712,.T.);
#83863=ORIENTED_EDGE('',*,*,#56694,.F.);
#83864=ORIENTED_EDGE('',*,*,#56706,.T.);
#83865=ORIENTED_EDGE('',*,*,#56707,.T.);
#83866=ORIENTED_EDGE('',*,*,#56693,.F.);
#83867=ORIENTED_EDGE('',*,*,#56701,.T.);
#83868=ORIENTED_EDGE('',*,*,#56702,.T.);
#83869=ORIENTED_EDGE('',*,*,#56692,.F.);
#83870=ORIENTED_EDGE('',*,*,#56696,.T.);
#83871=ORIENTED_EDGE('',*,*,#56691,.F.);
#83872=ORIENTED_EDGE('',*,*,#56725,.T.);
#83873=ORIENTED_EDGE('',*,*,#56653,.F.);
#83874=ORIENTED_EDGE('',*,*,#56657,.F.);
#83875=ORIENTED_EDGE('',*,*,#56684,.F.);
#83876=ORIENTED_EDGE('',*,*,#56663,.T.);
#83877=ORIENTED_EDGE('',*,*,#56667,.T.);
#83878=ORIENTED_EDGE('',*,*,#56670,.T.);
#83879=ORIENTED_EDGE('',*,*,#56673,.T.);
#83880=ORIENTED_EDGE('',*,*,#56679,.T.);
#83881=ORIENTED_EDGE('',*,*,#56678,.T.);
#83882=ORIENTED_EDGE('',*,*,#56685,.F.);
#83883=ORIENTED_EDGE('',*,*,#56655,.F.);
#83884=ORIENTED_EDGE('',*,*,#56641,.F.);
#83885=ORIENTED_EDGE('',*,*,#56645,.F.);
#83886=ORIENTED_EDGE('',*,*,#56648,.F.);
#83887=ORIENTED_EDGE('',*,*,#56732,.F.);
#83888=ORIENTED_EDGE('',*,*,#56676,.T.);
#83889=ORIENTED_EDGE('',*,*,#56680,.T.);
#83890=ORIENTED_EDGE('',*,*,#56674,.T.);
#83891=ORIENTED_EDGE('',*,*,#56671,.T.);
#83892=ORIENTED_EDGE('',*,*,#56668,.T.);
#83893=ORIENTED_EDGE('',*,*,#56665,.T.);
#83894=ORIENTED_EDGE('',*,*,#56661,.T.);
#83895=ORIENTED_EDGE('',*,*,#56681,.F.);
#83896=ORIENTED_EDGE('',*,*,#56658,.F.);
#83897=ORIENTED_EDGE('',*,*,#56651,.T.);
#83898=ORIENTED_EDGE('',*,*,#56733,.T.);
#83899=ORIENTED_EDGE('',*,*,#56649,.T.);
#83900=ORIENTED_EDGE('',*,*,#56646,.T.);
#83901=ORIENTED_EDGE('',*,*,#56643,.T.);
#83902=ORIENTED_EDGE('',*,*,#56639,.T.);
#83903=ORIENTED_EDGE('',*,*,#56689,.F.);
#83904=ORIENTED_EDGE('',*,*,#56686,.F.);
#83905=ORIENTED_EDGE('',*,*,#56650,.T.);
#83906=ORIENTED_EDGE('',*,*,#56732,.T.);
#83907=ORIENTED_EDGE('',*,*,#56647,.F.);
#83908=ORIENTED_EDGE('',*,*,#56733,.F.);
#83909=ORIENTED_EDGE('',*,*,#56734,.T.);
#83910=ORIENTED_EDGE('',*,*,#56735,.T.);
#83911=ORIENTED_EDGE('',*,*,#56736,.F.);
#83912=ORIENTED_EDGE('',*,*,#56737,.F.);
#83913=ORIENTED_EDGE('',*,*,#56738,.T.);
#83914=ORIENTED_EDGE('',*,*,#56739,.T.);
#83915=ORIENTED_EDGE('',*,*,#56734,.F.);
#83916=ORIENTED_EDGE('',*,*,#56740,.F.);
#83917=ORIENTED_EDGE('',*,*,#56741,.T.);
#83918=ORIENTED_EDGE('',*,*,#56742,.T.);
#83919=ORIENTED_EDGE('',*,*,#56738,.F.);
#83920=ORIENTED_EDGE('',*,*,#56743,.F.);
#83921=ORIENTED_EDGE('',*,*,#56744,.T.);
#83922=ORIENTED_EDGE('',*,*,#56745,.T.);
#83923=ORIENTED_EDGE('',*,*,#56741,.F.);
#83924=ORIENTED_EDGE('',*,*,#56746,.F.);
#83925=ORIENTED_EDGE('',*,*,#56747,.T.);
#83926=ORIENTED_EDGE('',*,*,#56748,.T.);
#83927=ORIENTED_EDGE('',*,*,#56744,.F.);
#83928=ORIENTED_EDGE('',*,*,#56749,.F.);
#83929=ORIENTED_EDGE('',*,*,#56750,.F.);
#83930=ORIENTED_EDGE('',*,*,#56751,.F.);
#83931=ORIENTED_EDGE('',*,*,#56752,.T.);
#83932=ORIENTED_EDGE('',*,*,#56753,.T.);
#83933=ORIENTED_EDGE('',*,*,#56754,.F.);
#83934=ORIENTED_EDGE('',*,*,#56755,.F.);
#83935=ORIENTED_EDGE('',*,*,#56756,.T.);
#83936=ORIENTED_EDGE('',*,*,#56757,.F.);
#83937=ORIENTED_EDGE('',*,*,#56753,.F.);
#83938=ORIENTED_EDGE('',*,*,#56758,.F.);
#83939=ORIENTED_EDGE('',*,*,#56759,.T.);
#83940=ORIENTED_EDGE('',*,*,#56760,.F.);
#83941=ORIENTED_EDGE('',*,*,#56756,.F.);
#83942=ORIENTED_EDGE('',*,*,#56761,.F.);
#83943=ORIENTED_EDGE('',*,*,#56762,.T.);
#83944=ORIENTED_EDGE('',*,*,#56763,.F.);
#83945=ORIENTED_EDGE('',*,*,#56759,.F.);
#83946=ORIENTED_EDGE('',*,*,#56764,.F.);
#83947=ORIENTED_EDGE('',*,*,#56765,.T.);
#83948=ORIENTED_EDGE('',*,*,#56766,.F.);
#83949=ORIENTED_EDGE('',*,*,#56762,.F.);
#83950=ORIENTED_EDGE('',*,*,#56767,.F.);
#83951=ORIENTED_EDGE('',*,*,#56768,.T.);
#83952=ORIENTED_EDGE('',*,*,#56769,.F.);
#83953=ORIENTED_EDGE('',*,*,#56765,.F.);
#83954=ORIENTED_EDGE('',*,*,#56770,.F.);
#83955=ORIENTED_EDGE('',*,*,#56771,.F.);
#83956=ORIENTED_EDGE('',*,*,#56772,.F.);
#83957=ORIENTED_EDGE('',*,*,#56773,.F.);
#83958=ORIENTED_EDGE('',*,*,#56774,.F.);
#83959=ORIENTED_EDGE('',*,*,#56771,.T.);
#83960=ORIENTED_EDGE('',*,*,#56775,.F.);
#83961=ORIENTED_EDGE('',*,*,#56768,.F.);
#83962=ORIENTED_EDGE('',*,*,#56776,.F.);
#83963=ORIENTED_EDGE('',*,*,#56777,.F.);
#83964=ORIENTED_EDGE('',*,*,#56778,.T.);
#83965=ORIENTED_EDGE('',*,*,#56779,.F.);
#83966=ORIENTED_EDGE('',*,*,#56780,.F.);
#83967=ORIENTED_EDGE('',*,*,#56781,.F.);
#83968=ORIENTED_EDGE('',*,*,#56782,.F.);
#83969=ORIENTED_EDGE('',*,*,#56783,.F.);
#83970=ORIENTED_EDGE('',*,*,#56784,.F.);
#83971=ORIENTED_EDGE('',*,*,#56785,.T.);
#83972=ORIENTED_EDGE('',*,*,#56786,.T.);
#83973=ORIENTED_EDGE('',*,*,#56787,.T.);
#83974=ORIENTED_EDGE('',*,*,#56788,.T.);
#83975=ORIENTED_EDGE('',*,*,#56789,.T.);
#83976=ORIENTED_EDGE('',*,*,#56790,.F.);
#83977=ORIENTED_EDGE('',*,*,#56789,.F.);
#83978=ORIENTED_EDGE('',*,*,#56791,.T.);
#83979=ORIENTED_EDGE('',*,*,#56792,.T.);
#83980=ORIENTED_EDGE('',*,*,#56793,.T.);
#83981=ORIENTED_EDGE('',*,*,#56794,.T.);
#83982=ORIENTED_EDGE('',*,*,#56795,.T.);
#83983=ORIENTED_EDGE('',*,*,#56796,.F.);
#83984=ORIENTED_EDGE('',*,*,#56795,.F.);
#83985=ORIENTED_EDGE('',*,*,#56797,.T.);
#83986=ORIENTED_EDGE('',*,*,#56736,.T.);
#83987=ORIENTED_EDGE('',*,*,#56798,.T.);
#83988=ORIENTED_EDGE('',*,*,#56773,.T.);
#83989=ORIENTED_EDGE('',*,*,#56790,.T.);
#83990=ORIENTED_EDGE('',*,*,#56796,.T.);
#83991=ORIENTED_EDGE('',*,*,#56799,.T.);
#83992=ORIENTED_EDGE('',*,*,#56779,.T.);
#83993=ORIENTED_EDGE('',*,*,#56800,.F.);
#83994=ORIENTED_EDGE('',*,*,#56792,.F.);
#83995=ORIENTED_EDGE('',*,*,#56800,.T.);
#83996=ORIENTED_EDGE('',*,*,#56784,.T.);
#83997=ORIENTED_EDGE('',*,*,#56801,.F.);
#83998=ORIENTED_EDGE('',*,*,#56793,.F.);
#83999=ORIENTED_EDGE('',*,*,#56801,.T.);
#84000=ORIENTED_EDGE('',*,*,#56783,.T.);
#84001=ORIENTED_EDGE('',*,*,#56802,.F.);
#84002=ORIENTED_EDGE('',*,*,#56785,.F.);
#84003=ORIENTED_EDGE('',*,*,#56802,.T.);
#84004=ORIENTED_EDGE('',*,*,#56782,.T.);
#84005=ORIENTED_EDGE('',*,*,#56803,.F.);
#84006=ORIENTED_EDGE('',*,*,#56786,.F.);
#84007=ORIENTED_EDGE('',*,*,#56803,.T.);
#84008=ORIENTED_EDGE('',*,*,#56781,.T.);
#84009=ORIENTED_EDGE('',*,*,#56804,.F.);
#84010=ORIENTED_EDGE('',*,*,#56787,.F.);
#84011=ORIENTED_EDGE('',*,*,#56804,.T.);
#84012=ORIENTED_EDGE('',*,*,#56780,.T.);
#84013=ORIENTED_EDGE('',*,*,#56799,.F.);
#84014=ORIENTED_EDGE('',*,*,#56791,.F.);
#84015=ORIENTED_EDGE('',*,*,#56788,.F.);
#84016=ORIENTED_EDGE('',*,*,#56777,.T.);
#84017=ORIENTED_EDGE('',*,*,#56778,.F.);
#84018=ORIENTED_EDGE('',*,*,#56751,.T.);
#84019=ORIENTED_EDGE('',*,*,#56805,.T.);
#84020=ORIENTED_EDGE('',*,*,#56754,.T.);
#84021=ORIENTED_EDGE('',*,*,#56806,.T.);
#84022=ORIENTED_EDGE('',*,*,#56752,.F.);
#84023=ORIENTED_EDGE('',*,*,#56806,.F.);
#84024=ORIENTED_EDGE('',*,*,#56757,.T.);
#84025=ORIENTED_EDGE('',*,*,#56760,.T.);
#84026=ORIENTED_EDGE('',*,*,#56763,.T.);
#84027=ORIENTED_EDGE('',*,*,#56766,.T.);
#84028=ORIENTED_EDGE('',*,*,#56769,.T.);
#84029=ORIENTED_EDGE('',*,*,#56775,.T.);
#84030=ORIENTED_EDGE('',*,*,#56774,.T.);
#84031=ORIENTED_EDGE('',*,*,#56798,.F.);
#84032=ORIENTED_EDGE('',*,*,#56735,.F.);
#84033=ORIENTED_EDGE('',*,*,#56739,.F.);
#84034=ORIENTED_EDGE('',*,*,#56742,.F.);
#84035=ORIENTED_EDGE('',*,*,#56745,.F.);
#84036=ORIENTED_EDGE('',*,*,#56748,.F.);
#84037=ORIENTED_EDGE('',*,*,#56807,.F.);
#84038=ORIENTED_EDGE('',*,*,#56772,.T.);
#84039=ORIENTED_EDGE('',*,*,#56776,.T.);
#84040=ORIENTED_EDGE('',*,*,#56770,.T.);
#84041=ORIENTED_EDGE('',*,*,#56767,.T.);
#84042=ORIENTED_EDGE('',*,*,#56764,.T.);
#84043=ORIENTED_EDGE('',*,*,#56761,.T.);
#84044=ORIENTED_EDGE('',*,*,#56758,.T.);
#84045=ORIENTED_EDGE('',*,*,#56755,.T.);
#84046=ORIENTED_EDGE('',*,*,#56805,.F.);
#84047=ORIENTED_EDGE('',*,*,#56808,.T.);
#84048=ORIENTED_EDGE('',*,*,#56749,.T.);
#84049=ORIENTED_EDGE('',*,*,#56746,.T.);
#84050=ORIENTED_EDGE('',*,*,#56743,.T.);
#84051=ORIENTED_EDGE('',*,*,#56740,.T.);
#84052=ORIENTED_EDGE('',*,*,#56737,.T.);
#84053=ORIENTED_EDGE('',*,*,#56797,.F.);
#84054=ORIENTED_EDGE('',*,*,#56794,.F.);
#84055=ORIENTED_EDGE('',*,*,#56750,.T.);
#84056=ORIENTED_EDGE('',*,*,#56807,.T.);
#84057=ORIENTED_EDGE('',*,*,#56747,.F.);
#84058=ORIENTED_EDGE('',*,*,#56808,.F.);
#84059=ORIENTED_EDGE('',*,*,#56809,.F.);
#84060=ORIENTED_EDGE('',*,*,#56810,.F.);
#84061=ORIENTED_EDGE('',*,*,#56811,.F.);
#84062=ORIENTED_EDGE('',*,*,#56812,.T.);
#84063=ORIENTED_EDGE('',*,*,#56813,.T.);
#84064=ORIENTED_EDGE('',*,*,#56814,.T.);
#84065=ORIENTED_EDGE('',*,*,#56815,.T.);
#84066=ORIENTED_EDGE('',*,*,#56814,.F.);
#84067=ORIENTED_EDGE('',*,*,#56816,.T.);
#84068=ORIENTED_EDGE('',*,*,#56811,.T.);
#84069=ORIENTED_EDGE('',*,*,#56817,.T.);
#84070=ORIENTED_EDGE('',*,*,#56818,.T.);
#84071=ORIENTED_EDGE('',*,*,#56819,.T.);
#84072=ORIENTED_EDGE('',*,*,#56820,.T.);
#84073=ORIENTED_EDGE('',*,*,#56818,.F.);
#84074=ORIENTED_EDGE('',*,*,#56821,.T.);
#84075=ORIENTED_EDGE('',*,*,#56821,.F.);
#84076=ORIENTED_EDGE('',*,*,#56817,.F.);
#84077=ORIENTED_EDGE('',*,*,#56810,.T.);
#84078=ORIENTED_EDGE('',*,*,#56822,.T.);
#84079=ORIENTED_EDGE('',*,*,#56823,.T.);
#84080=ORIENTED_EDGE('',*,*,#56812,.F.);
#84081=ORIENTED_EDGE('',*,*,#56816,.F.);
#84082=ORIENTED_EDGE('',*,*,#56813,.F.);
#84083=ORIENTED_EDGE('',*,*,#56820,.F.);
#84084=ORIENTED_EDGE('',*,*,#56824,.T.);
#84085=ORIENTED_EDGE('',*,*,#56825,.F.);
#84086=ORIENTED_EDGE('',*,*,#56809,.T.);
#84087=ORIENTED_EDGE('',*,*,#56825,.T.);
#84088=ORIENTED_EDGE('',*,*,#56826,.T.);
#84089=ORIENTED_EDGE('',*,*,#56822,.F.);
#84090=ORIENTED_EDGE('',*,*,#56815,.F.);
#84091=ORIENTED_EDGE('',*,*,#56819,.F.);
#84092=ORIENTED_EDGE('',*,*,#56823,.F.);
#84093=ORIENTED_EDGE('',*,*,#56826,.F.);
#84094=ORIENTED_EDGE('',*,*,#56824,.F.);
#84095=ORIENTED_EDGE('',*,*,#56827,.F.);
#84096=ORIENTED_EDGE('',*,*,#56828,.F.);
#84097=ORIENTED_EDGE('',*,*,#56829,.T.);
#84098=ORIENTED_EDGE('',*,*,#56830,.F.);
#84099=ORIENTED_EDGE('',*,*,#56831,.F.);
#84100=ORIENTED_EDGE('',*,*,#56827,.T.);
#84101=ORIENTED_EDGE('',*,*,#56832,.T.);
#84102=ORIENTED_EDGE('',*,*,#56833,.F.);
#84103=ORIENTED_EDGE('',*,*,#56834,.F.);
#84104=ORIENTED_EDGE('',*,*,#56830,.T.);
#84105=ORIENTED_EDGE('',*,*,#56835,.T.);
#84106=ORIENTED_EDGE('',*,*,#56836,.F.);
#84107=ORIENTED_EDGE('',*,*,#56837,.F.);
#84108=ORIENTED_EDGE('',*,*,#56833,.T.);
#84109=ORIENTED_EDGE('',*,*,#56838,.T.);
#84110=ORIENTED_EDGE('',*,*,#56839,.F.);
#84111=ORIENTED_EDGE('',*,*,#56840,.F.);
#84112=ORIENTED_EDGE('',*,*,#56836,.T.);
#84113=ORIENTED_EDGE('',*,*,#56841,.T.);
#84114=ORIENTED_EDGE('',*,*,#56842,.F.);
#84115=ORIENTED_EDGE('',*,*,#56843,.F.);
#84116=ORIENTED_EDGE('',*,*,#56839,.T.);
#84117=ORIENTED_EDGE('',*,*,#56844,.T.);
#84118=ORIENTED_EDGE('',*,*,#56845,.F.);
#84119=ORIENTED_EDGE('',*,*,#56846,.F.);
#84120=ORIENTED_EDGE('',*,*,#56842,.T.);
#84121=ORIENTED_EDGE('',*,*,#56847,.T.);
#84122=ORIENTED_EDGE('',*,*,#56848,.F.);
#84123=ORIENTED_EDGE('',*,*,#56849,.F.);
#84124=ORIENTED_EDGE('',*,*,#56845,.T.);
#84125=ORIENTED_EDGE('',*,*,#56850,.T.);
#84126=ORIENTED_EDGE('',*,*,#56851,.F.);
#84127=ORIENTED_EDGE('',*,*,#56852,.F.);
#84128=ORIENTED_EDGE('',*,*,#56848,.T.);
#84129=ORIENTED_EDGE('',*,*,#56853,.T.);
#84130=ORIENTED_EDGE('',*,*,#56854,.F.);
#84131=ORIENTED_EDGE('',*,*,#56855,.F.);
#84132=ORIENTED_EDGE('',*,*,#56851,.T.);
#84133=ORIENTED_EDGE('',*,*,#56856,.T.);
#84134=ORIENTED_EDGE('',*,*,#56857,.F.);
#84135=ORIENTED_EDGE('',*,*,#56858,.F.);
#84136=ORIENTED_EDGE('',*,*,#56854,.T.);
#84137=ORIENTED_EDGE('',*,*,#56859,.T.);
#84138=ORIENTED_EDGE('',*,*,#56860,.F.);
#84139=ORIENTED_EDGE('',*,*,#56861,.F.);
#84140=ORIENTED_EDGE('',*,*,#56857,.T.);
#84141=ORIENTED_EDGE('',*,*,#56862,.T.);
#84142=ORIENTED_EDGE('',*,*,#56863,.F.);
#84143=ORIENTED_EDGE('',*,*,#56864,.F.);
#84144=ORIENTED_EDGE('',*,*,#56860,.T.);
#84145=ORIENTED_EDGE('',*,*,#56865,.T.);
#84146=ORIENTED_EDGE('',*,*,#56866,.F.);
#84147=ORIENTED_EDGE('',*,*,#56867,.F.);
#84148=ORIENTED_EDGE('',*,*,#56863,.T.);
#84149=ORIENTED_EDGE('',*,*,#56868,.T.);
#84150=ORIENTED_EDGE('',*,*,#56869,.F.);
#84151=ORIENTED_EDGE('',*,*,#56870,.F.);
#84152=ORIENTED_EDGE('',*,*,#56866,.T.);
#84153=ORIENTED_EDGE('',*,*,#56871,.T.);
#84154=ORIENTED_EDGE('',*,*,#56872,.F.);
#84155=ORIENTED_EDGE('',*,*,#56873,.F.);
#84156=ORIENTED_EDGE('',*,*,#56869,.T.);
#84157=ORIENTED_EDGE('',*,*,#56874,.T.);
#84158=ORIENTED_EDGE('',*,*,#56875,.F.);
#84159=ORIENTED_EDGE('',*,*,#56876,.F.);
#84160=ORIENTED_EDGE('',*,*,#56872,.T.);
#84161=ORIENTED_EDGE('',*,*,#56877,.T.);
#84162=ORIENTED_EDGE('',*,*,#56878,.F.);
#84163=ORIENTED_EDGE('',*,*,#56879,.F.);
#84164=ORIENTED_EDGE('',*,*,#56875,.T.);
#84165=ORIENTED_EDGE('',*,*,#56880,.T.);
#84166=ORIENTED_EDGE('',*,*,#56881,.F.);
#84167=ORIENTED_EDGE('',*,*,#56882,.F.);
#84168=ORIENTED_EDGE('',*,*,#56878,.T.);
#84169=ORIENTED_EDGE('',*,*,#56883,.T.);
#84170=ORIENTED_EDGE('',*,*,#56884,.F.);
#84171=ORIENTED_EDGE('',*,*,#56885,.F.);
#84172=ORIENTED_EDGE('',*,*,#56881,.T.);
#84173=ORIENTED_EDGE('',*,*,#56886,.T.);
#84174=ORIENTED_EDGE('',*,*,#56887,.F.);
#84175=ORIENTED_EDGE('',*,*,#56888,.F.);
#84176=ORIENTED_EDGE('',*,*,#56889,.F.);
#84177=ORIENTED_EDGE('',*,*,#56890,.T.);
#84178=ORIENTED_EDGE('',*,*,#56891,.F.);
#84179=ORIENTED_EDGE('',*,*,#56892,.F.);
#84180=ORIENTED_EDGE('',*,*,#56887,.T.);
#84181=ORIENTED_EDGE('',*,*,#56893,.T.);
#84182=ORIENTED_EDGE('',*,*,#56894,.F.);
#84183=ORIENTED_EDGE('',*,*,#56895,.F.);
#84184=ORIENTED_EDGE('',*,*,#56891,.T.);
#84185=ORIENTED_EDGE('',*,*,#56896,.T.);
#84186=ORIENTED_EDGE('',*,*,#56897,.F.);
#84187=ORIENTED_EDGE('',*,*,#56898,.F.);
#84188=ORIENTED_EDGE('',*,*,#56894,.T.);
#84189=ORIENTED_EDGE('',*,*,#56899,.T.);
#84190=ORIENTED_EDGE('',*,*,#56900,.F.);
#84191=ORIENTED_EDGE('',*,*,#56901,.F.);
#84192=ORIENTED_EDGE('',*,*,#56897,.T.);
#84193=ORIENTED_EDGE('',*,*,#56902,.T.);
#84194=ORIENTED_EDGE('',*,*,#56903,.F.);
#84195=ORIENTED_EDGE('',*,*,#56904,.F.);
#84196=ORIENTED_EDGE('',*,*,#56900,.T.);
#84197=ORIENTED_EDGE('',*,*,#56905,.T.);
#84198=ORIENTED_EDGE('',*,*,#56906,.F.);
#84199=ORIENTED_EDGE('',*,*,#56907,.F.);
#84200=ORIENTED_EDGE('',*,*,#56903,.T.);
#84201=ORIENTED_EDGE('',*,*,#56908,.T.);
#84202=ORIENTED_EDGE('',*,*,#56909,.F.);
#84203=ORIENTED_EDGE('',*,*,#56910,.F.);
#84204=ORIENTED_EDGE('',*,*,#56906,.T.);
#84205=ORIENTED_EDGE('',*,*,#56911,.T.);
#84206=ORIENTED_EDGE('',*,*,#56912,.F.);
#84207=ORIENTED_EDGE('',*,*,#56913,.F.);
#84208=ORIENTED_EDGE('',*,*,#56909,.T.);
#84209=ORIENTED_EDGE('',*,*,#56914,.T.);
#84210=ORIENTED_EDGE('',*,*,#56915,.F.);
#84211=ORIENTED_EDGE('',*,*,#56916,.F.);
#84212=ORIENTED_EDGE('',*,*,#56912,.T.);
#84213=ORIENTED_EDGE('',*,*,#56917,.T.);
#84214=ORIENTED_EDGE('',*,*,#56918,.F.);
#84215=ORIENTED_EDGE('',*,*,#56919,.F.);
#84216=ORIENTED_EDGE('',*,*,#56915,.T.);
#84217=ORIENTED_EDGE('',*,*,#56920,.T.);
#84218=ORIENTED_EDGE('',*,*,#56921,.F.);
#84219=ORIENTED_EDGE('',*,*,#56922,.F.);
#84220=ORIENTED_EDGE('',*,*,#56918,.T.);
#84221=ORIENTED_EDGE('',*,*,#56923,.T.);
#84222=ORIENTED_EDGE('',*,*,#56924,.F.);
#84223=ORIENTED_EDGE('',*,*,#56925,.F.);
#84224=ORIENTED_EDGE('',*,*,#56921,.T.);
#84225=ORIENTED_EDGE('',*,*,#56926,.T.);
#84226=ORIENTED_EDGE('',*,*,#56927,.F.);
#84227=ORIENTED_EDGE('',*,*,#56928,.T.);
#84228=ORIENTED_EDGE('',*,*,#56929,.T.);
#84229=ORIENTED_EDGE('',*,*,#56930,.T.);
#84230=ORIENTED_EDGE('',*,*,#56931,.F.);
#84231=ORIENTED_EDGE('',*,*,#56932,.T.);
#84232=ORIENTED_EDGE('',*,*,#56927,.T.);
#84233=ORIENTED_EDGE('',*,*,#56933,.T.);
#84234=ORIENTED_EDGE('',*,*,#56934,.F.);
#84235=ORIENTED_EDGE('',*,*,#56935,.T.);
#84236=ORIENTED_EDGE('',*,*,#56931,.T.);
#84237=ORIENTED_EDGE('',*,*,#56936,.T.);
#84238=ORIENTED_EDGE('',*,*,#56937,.F.);
#84239=ORIENTED_EDGE('',*,*,#56938,.T.);
#84240=ORIENTED_EDGE('',*,*,#56934,.T.);
#84241=ORIENTED_EDGE('',*,*,#56939,.T.);
#84242=ORIENTED_EDGE('',*,*,#56940,.F.);
#84243=ORIENTED_EDGE('',*,*,#56941,.T.);
#84244=ORIENTED_EDGE('',*,*,#56937,.T.);
#84245=ORIENTED_EDGE('',*,*,#56942,.T.);
#84246=ORIENTED_EDGE('',*,*,#56943,.F.);
#84247=ORIENTED_EDGE('',*,*,#56944,.T.);
#84248=ORIENTED_EDGE('',*,*,#56940,.T.);
#84249=ORIENTED_EDGE('',*,*,#56945,.T.);
#84250=ORIENTED_EDGE('',*,*,#56946,.F.);
#84251=ORIENTED_EDGE('',*,*,#56947,.T.);
#84252=ORIENTED_EDGE('',*,*,#56943,.T.);
#84253=ORIENTED_EDGE('',*,*,#56948,.T.);
#84254=ORIENTED_EDGE('',*,*,#56949,.F.);
#84255=ORIENTED_EDGE('',*,*,#56950,.T.);
#84256=ORIENTED_EDGE('',*,*,#56946,.T.);
#84257=ORIENTED_EDGE('',*,*,#56951,.T.);
#84258=ORIENTED_EDGE('',*,*,#56952,.F.);
#84259=ORIENTED_EDGE('',*,*,#56953,.T.);
#84260=ORIENTED_EDGE('',*,*,#56949,.T.);
#84261=ORIENTED_EDGE('',*,*,#56954,.T.);
#84262=ORIENTED_EDGE('',*,*,#56955,.F.);
#84263=ORIENTED_EDGE('',*,*,#56956,.T.);
#84264=ORIENTED_EDGE('',*,*,#56952,.T.);
#84265=ORIENTED_EDGE('',*,*,#56957,.T.);
#84266=ORIENTED_EDGE('',*,*,#56958,.F.);
#84267=ORIENTED_EDGE('',*,*,#56959,.T.);
#84268=ORIENTED_EDGE('',*,*,#56955,.T.);
#84269=ORIENTED_EDGE('',*,*,#56960,.T.);
#84270=ORIENTED_EDGE('',*,*,#56961,.F.);
#84271=ORIENTED_EDGE('',*,*,#56962,.T.);
#84272=ORIENTED_EDGE('',*,*,#56958,.T.);
#84273=ORIENTED_EDGE('',*,*,#56963,.T.);
#84274=ORIENTED_EDGE('',*,*,#56964,.F.);
#84275=ORIENTED_EDGE('',*,*,#56965,.T.);
#84276=ORIENTED_EDGE('',*,*,#56961,.T.);
#84277=ORIENTED_EDGE('',*,*,#56966,.T.);
#84278=ORIENTED_EDGE('',*,*,#56967,.F.);
#84279=ORIENTED_EDGE('',*,*,#56968,.T.);
#84280=ORIENTED_EDGE('',*,*,#56969,.F.);
#84281=ORIENTED_EDGE('',*,*,#56970,.T.);
#84282=ORIENTED_EDGE('',*,*,#56971,.F.);
#84283=ORIENTED_EDGE('',*,*,#56972,.T.);
#84284=ORIENTED_EDGE('',*,*,#56967,.T.);
#84285=ORIENTED_EDGE('',*,*,#56973,.T.);
#84286=ORIENTED_EDGE('',*,*,#56974,.F.);
#84287=ORIENTED_EDGE('',*,*,#56975,.T.);
#84288=ORIENTED_EDGE('',*,*,#56971,.T.);
#84289=ORIENTED_EDGE('',*,*,#56976,.T.);
#84290=ORIENTED_EDGE('',*,*,#56977,.F.);
#84291=ORIENTED_EDGE('',*,*,#56978,.T.);
#84292=ORIENTED_EDGE('',*,*,#56974,.T.);
#84293=ORIENTED_EDGE('',*,*,#56979,.T.);
#84294=ORIENTED_EDGE('',*,*,#56980,.F.);
#84295=ORIENTED_EDGE('',*,*,#56981,.T.);
#84296=ORIENTED_EDGE('',*,*,#56977,.T.);
#84297=ORIENTED_EDGE('',*,*,#56982,.T.);
#84298=ORIENTED_EDGE('',*,*,#56983,.F.);
#84299=ORIENTED_EDGE('',*,*,#56984,.T.);
#84300=ORIENTED_EDGE('',*,*,#56980,.T.);
#84301=ORIENTED_EDGE('',*,*,#56985,.T.);
#84302=ORIENTED_EDGE('',*,*,#56986,.F.);
#84303=ORIENTED_EDGE('',*,*,#56987,.T.);
#84304=ORIENTED_EDGE('',*,*,#56983,.T.);
#84305=ORIENTED_EDGE('',*,*,#56988,.T.);
#84306=ORIENTED_EDGE('',*,*,#56989,.F.);
#84307=ORIENTED_EDGE('',*,*,#56990,.T.);
#84308=ORIENTED_EDGE('',*,*,#56986,.T.);
#84309=ORIENTED_EDGE('',*,*,#56991,.T.);
#84310=ORIENTED_EDGE('',*,*,#56992,.F.);
#84311=ORIENTED_EDGE('',*,*,#56993,.T.);
#84312=ORIENTED_EDGE('',*,*,#56989,.T.);
#84313=ORIENTED_EDGE('',*,*,#56994,.T.);
#84314=ORIENTED_EDGE('',*,*,#56995,.F.);
#84315=ORIENTED_EDGE('',*,*,#56996,.T.);
#84316=ORIENTED_EDGE('',*,*,#56992,.T.);
#84317=ORIENTED_EDGE('',*,*,#56997,.T.);
#84318=ORIENTED_EDGE('',*,*,#56998,.F.);
#84319=ORIENTED_EDGE('',*,*,#56999,.T.);
#84320=ORIENTED_EDGE('',*,*,#56995,.T.);
#84321=ORIENTED_EDGE('',*,*,#57000,.T.);
#84322=ORIENTED_EDGE('',*,*,#57001,.F.);
#84323=ORIENTED_EDGE('',*,*,#57002,.T.);
#84324=ORIENTED_EDGE('',*,*,#56998,.T.);
#84325=ORIENTED_EDGE('',*,*,#57003,.T.);
#84326=ORIENTED_EDGE('',*,*,#57004,.F.);
#84327=ORIENTED_EDGE('',*,*,#57005,.T.);
#84328=ORIENTED_EDGE('',*,*,#57001,.T.);
#84329=ORIENTED_EDGE('',*,*,#57006,.T.);
#84330=ORIENTED_EDGE('',*,*,#57007,.F.);
#84331=ORIENTED_EDGE('',*,*,#57008,.T.);
#84332=ORIENTED_EDGE('',*,*,#57004,.T.);
#84333=ORIENTED_EDGE('',*,*,#57009,.T.);
#84334=ORIENTED_EDGE('',*,*,#57010,.F.);
#84335=ORIENTED_EDGE('',*,*,#57011,.T.);
#84336=ORIENTED_EDGE('',*,*,#57007,.T.);
#84337=ORIENTED_EDGE('',*,*,#57012,.T.);
#84338=ORIENTED_EDGE('',*,*,#57013,.F.);
#84339=ORIENTED_EDGE('',*,*,#57014,.T.);
#84340=ORIENTED_EDGE('',*,*,#57010,.T.);
#84341=ORIENTED_EDGE('',*,*,#57015,.T.);
#84342=ORIENTED_EDGE('',*,*,#57016,.F.);
#84343=ORIENTED_EDGE('',*,*,#57017,.T.);
#84344=ORIENTED_EDGE('',*,*,#57013,.T.);
#84345=ORIENTED_EDGE('',*,*,#57018,.T.);
#84346=ORIENTED_EDGE('',*,*,#57019,.F.);
#84347=ORIENTED_EDGE('',*,*,#57020,.T.);
#84348=ORIENTED_EDGE('',*,*,#57016,.T.);
#84349=ORIENTED_EDGE('',*,*,#57021,.T.);
#84350=ORIENTED_EDGE('',*,*,#57022,.F.);
#84351=ORIENTED_EDGE('',*,*,#57023,.T.);
#84352=ORIENTED_EDGE('',*,*,#57019,.T.);
#84353=ORIENTED_EDGE('',*,*,#57024,.T.);
#84354=ORIENTED_EDGE('',*,*,#57022,.T.);
#84355=ORIENTED_EDGE('',*,*,#57025,.T.);
#84356=ORIENTED_EDGE('',*,*,#57026,.T.);
#84357=ORIENTED_EDGE('',*,*,#56969,.T.);
#84358=ORIENTED_EDGE('',*,*,#57027,.T.);
#84359=ORIENTED_EDGE('',*,*,#57028,.T.);
#84360=ORIENTED_EDGE('',*,*,#57029,.F.);
#84361=ORIENTED_EDGE('',*,*,#57028,.F.);
#84362=ORIENTED_EDGE('',*,*,#57030,.T.);
#84363=ORIENTED_EDGE('',*,*,#57031,.T.);
#84364=ORIENTED_EDGE('',*,*,#57032,.T.);
#84365=ORIENTED_EDGE('',*,*,#57033,.F.);
#84366=ORIENTED_EDGE('',*,*,#57034,.F.);
#84367=ORIENTED_EDGE('',*,*,#57035,.F.);
#84368=ORIENTED_EDGE('',*,*,#56929,.F.);
#84369=ORIENTED_EDGE('',*,*,#57036,.F.);
#84370=ORIENTED_EDGE('',*,*,#57037,.T.);
#84371=ORIENTED_EDGE('',*,*,#57038,.F.);
#84372=ORIENTED_EDGE('',*,*,#57037,.F.);
#84373=ORIENTED_EDGE('',*,*,#56964,.T.);
#84374=ORIENTED_EDGE('',*,*,#57039,.T.);
#84375=ORIENTED_EDGE('',*,*,#57040,.F.);
#84376=ORIENTED_EDGE('',*,*,#57041,.T.);
#84377=ORIENTED_EDGE('',*,*,#57042,.F.);
#84378=ORIENTED_EDGE('',*,*,#56888,.T.);
#84379=ORIENTED_EDGE('',*,*,#56892,.T.);
#84380=ORIENTED_EDGE('',*,*,#56895,.T.);
#84381=ORIENTED_EDGE('',*,*,#56898,.T.);
#84382=ORIENTED_EDGE('',*,*,#56901,.T.);
#84383=ORIENTED_EDGE('',*,*,#56904,.T.);
#84384=ORIENTED_EDGE('',*,*,#56907,.T.);
#84385=ORIENTED_EDGE('',*,*,#56910,.T.);
#84386=ORIENTED_EDGE('',*,*,#56913,.T.);
#84387=ORIENTED_EDGE('',*,*,#56916,.T.);
#84388=ORIENTED_EDGE('',*,*,#56919,.T.);
#84389=ORIENTED_EDGE('',*,*,#56922,.T.);
#84390=ORIENTED_EDGE('',*,*,#56925,.T.);
#84391=ORIENTED_EDGE('',*,*,#57043,.T.);
#84392=ORIENTED_EDGE('',*,*,#57033,.T.);
#84393=ORIENTED_EDGE('',*,*,#57036,.T.);
#84394=ORIENTED_EDGE('',*,*,#56928,.F.);
#84395=ORIENTED_EDGE('',*,*,#56932,.F.);
#84396=ORIENTED_EDGE('',*,*,#56935,.F.);
#84397=ORIENTED_EDGE('',*,*,#56938,.F.);
#84398=ORIENTED_EDGE('',*,*,#56941,.F.);
#84399=ORIENTED_EDGE('',*,*,#56944,.F.);
#84400=ORIENTED_EDGE('',*,*,#56947,.F.);
#84401=ORIENTED_EDGE('',*,*,#56950,.F.);
#84402=ORIENTED_EDGE('',*,*,#56953,.F.);
#84403=ORIENTED_EDGE('',*,*,#56956,.F.);
#84404=ORIENTED_EDGE('',*,*,#56959,.F.);
#84405=ORIENTED_EDGE('',*,*,#56962,.F.);
#84406=ORIENTED_EDGE('',*,*,#56965,.F.);
#84407=ORIENTED_EDGE('',*,*,#57041,.F.);
#84408=ORIENTED_EDGE('',*,*,#57044,.F.);
#84409=ORIENTED_EDGE('',*,*,#57039,.F.);
#84410=ORIENTED_EDGE('',*,*,#56966,.F.);
#84411=ORIENTED_EDGE('',*,*,#56963,.F.);
#84412=ORIENTED_EDGE('',*,*,#56960,.F.);
#84413=ORIENTED_EDGE('',*,*,#56957,.F.);
#84414=ORIENTED_EDGE('',*,*,#56954,.F.);
#84415=ORIENTED_EDGE('',*,*,#56951,.F.);
#84416=ORIENTED_EDGE('',*,*,#56948,.F.);
#84417=ORIENTED_EDGE('',*,*,#56945,.F.);
#84418=ORIENTED_EDGE('',*,*,#56942,.F.);
#84419=ORIENTED_EDGE('',*,*,#56939,.F.);
#84420=ORIENTED_EDGE('',*,*,#56936,.F.);
#84421=ORIENTED_EDGE('',*,*,#56933,.F.);
#84422=ORIENTED_EDGE('',*,*,#56930,.F.);
#84423=ORIENTED_EDGE('',*,*,#57035,.T.);
#84424=ORIENTED_EDGE('',*,*,#57045,.F.);
#84425=ORIENTED_EDGE('',*,*,#56926,.F.);
#84426=ORIENTED_EDGE('',*,*,#56923,.F.);
#84427=ORIENTED_EDGE('',*,*,#56920,.F.);
#84428=ORIENTED_EDGE('',*,*,#56917,.F.);
#84429=ORIENTED_EDGE('',*,*,#56914,.F.);
#84430=ORIENTED_EDGE('',*,*,#56911,.F.);
#84431=ORIENTED_EDGE('',*,*,#56908,.F.);
#84432=ORIENTED_EDGE('',*,*,#56905,.F.);
#84433=ORIENTED_EDGE('',*,*,#56902,.F.);
#84434=ORIENTED_EDGE('',*,*,#56899,.F.);
#84435=ORIENTED_EDGE('',*,*,#56896,.F.);
#84436=ORIENTED_EDGE('',*,*,#56893,.F.);
#84437=ORIENTED_EDGE('',*,*,#56890,.F.);
#84438=ORIENTED_EDGE('',*,*,#56924,.T.);
#84439=ORIENTED_EDGE('',*,*,#57045,.T.);
#84440=ORIENTED_EDGE('',*,*,#57034,.T.);
#84441=ORIENTED_EDGE('',*,*,#57043,.F.);
#84442=ORIENTED_EDGE('',*,*,#57038,.T.);
#84443=ORIENTED_EDGE('',*,*,#57046,.T.);
#84444=ORIENTED_EDGE('',*,*,#57047,.T.);
#84445=ORIENTED_EDGE('',*,*,#57048,.T.);
#84446=ORIENTED_EDGE('',*,*,#57049,.T.);
#84447=ORIENTED_EDGE('',*,*,#57042,.T.);
#84448=ORIENTED_EDGE('',*,*,#57040,.T.);
#84449=ORIENTED_EDGE('',*,*,#57044,.T.);
#84450=ORIENTED_EDGE('',*,*,#56889,.T.);
#84451=ORIENTED_EDGE('',*,*,#57050,.F.);
#84452=ORIENTED_EDGE('',*,*,#57051,.F.);
#84453=ORIENTED_EDGE('',*,*,#57052,.F.);
#84454=ORIENTED_EDGE('',*,*,#57053,.F.);
#84455=ORIENTED_EDGE('',*,*,#57054,.T.);
#84456=ORIENTED_EDGE('',*,*,#57055,.T.);
#84457=ORIENTED_EDGE('',*,*,#57056,.T.);
#84458=ORIENTED_EDGE('',*,*,#57057,.T.);
#84459=ORIENTED_EDGE('',*,*,#57058,.T.);
#84460=ORIENTED_EDGE('',*,*,#57059,.T.);
#84461=ORIENTED_EDGE('',*,*,#57050,.T.);
#84462=ORIENTED_EDGE('',*,*,#57060,.F.);
#84463=ORIENTED_EDGE('',*,*,#57046,.F.);
#84464=ORIENTED_EDGE('',*,*,#57061,.T.);
#84465=ORIENTED_EDGE('',*,*,#57053,.T.);
#84466=ORIENTED_EDGE('',*,*,#57062,.F.);
#84467=ORIENTED_EDGE('',*,*,#57047,.F.);
#84468=ORIENTED_EDGE('',*,*,#57060,.T.);
#84469=ORIENTED_EDGE('',*,*,#57052,.T.);
#84470=ORIENTED_EDGE('',*,*,#57063,.F.);
#84471=ORIENTED_EDGE('',*,*,#57048,.F.);
#84472=ORIENTED_EDGE('',*,*,#57062,.T.);
#84473=ORIENTED_EDGE('',*,*,#57051,.T.);
#84474=ORIENTED_EDGE('',*,*,#57061,.F.);
#84475=ORIENTED_EDGE('',*,*,#57049,.F.);
#84476=ORIENTED_EDGE('',*,*,#57063,.T.);
#84477=ORIENTED_EDGE('',*,*,#57064,.T.);
#84478=ORIENTED_EDGE('',*,*,#57065,.T.);
#84479=ORIENTED_EDGE('',*,*,#57066,.T.);
#84480=ORIENTED_EDGE('',*,*,#57067,.F.);
#84481=ORIENTED_EDGE('',*,*,#57068,.F.);
#84482=ORIENTED_EDGE('',*,*,#57069,.F.);
#84483=ORIENTED_EDGE('',*,*,#57067,.T.);
#84484=ORIENTED_EDGE('',*,*,#57070,.T.);
#84485=ORIENTED_EDGE('',*,*,#57071,.T.);
#84486=ORIENTED_EDGE('',*,*,#57072,.F.);
#84487=ORIENTED_EDGE('',*,*,#57073,.F.);
#84488=ORIENTED_EDGE('',*,*,#57074,.F.);
#84489=ORIENTED_EDGE('',*,*,#57072,.T.);
#84490=ORIENTED_EDGE('',*,*,#57075,.T.);
#84491=ORIENTED_EDGE('',*,*,#57076,.T.);
#84492=ORIENTED_EDGE('',*,*,#57077,.F.);
#84493=ORIENTED_EDGE('',*,*,#57078,.F.);
#84494=ORIENTED_EDGE('',*,*,#57079,.F.);
#84495=ORIENTED_EDGE('',*,*,#57077,.T.);
#84496=ORIENTED_EDGE('',*,*,#57080,.T.);
#84497=ORIENTED_EDGE('',*,*,#57081,.T.);
#84498=ORIENTED_EDGE('',*,*,#57082,.F.);
#84499=ORIENTED_EDGE('',*,*,#57083,.F.);
#84500=ORIENTED_EDGE('',*,*,#57084,.F.);
#84501=ORIENTED_EDGE('',*,*,#57082,.T.);
#84502=ORIENTED_EDGE('',*,*,#57085,.T.);
#84503=ORIENTED_EDGE('',*,*,#57086,.T.);
#84504=ORIENTED_EDGE('',*,*,#57087,.F.);
#84505=ORIENTED_EDGE('',*,*,#57088,.F.);
#84506=ORIENTED_EDGE('',*,*,#57089,.F.);
#84507=ORIENTED_EDGE('',*,*,#57087,.T.);
#84508=ORIENTED_EDGE('',*,*,#57090,.T.);
#84509=ORIENTED_EDGE('',*,*,#57091,.T.);
#84510=ORIENTED_EDGE('',*,*,#57064,.F.);
#84511=ORIENTED_EDGE('',*,*,#57092,.F.);
#84512=ORIENTED_EDGE('',*,*,#57093,.F.);
#84513=ORIENTED_EDGE('',*,*,#57094,.F.);
#84514=ORIENTED_EDGE('',*,*,#57095,.T.);
#84515=ORIENTED_EDGE('',*,*,#57096,.T.);
#84516=ORIENTED_EDGE('',*,*,#57097,.T.);
#84517=ORIENTED_EDGE('',*,*,#57098,.T.);
#84518=ORIENTED_EDGE('',*,*,#57099,.T.);
#84519=ORIENTED_EDGE('',*,*,#57029,.T.);
#84520=ORIENTED_EDGE('',*,*,#57068,.T.);
#84521=ORIENTED_EDGE('',*,*,#57074,.T.);
#84522=ORIENTED_EDGE('',*,*,#57094,.T.);
#84523=ORIENTED_EDGE('',*,*,#57069,.T.);
#84524=ORIENTED_EDGE('',*,*,#57099,.F.);
#84525=ORIENTED_EDGE('',*,*,#57092,.T.);
#84526=ORIENTED_EDGE('',*,*,#57088,.T.);
#84527=ORIENTED_EDGE('',*,*,#57093,.T.);
#84528=ORIENTED_EDGE('',*,*,#57098,.F.);
#84529=ORIENTED_EDGE('',*,*,#57083,.T.);
#84530=ORIENTED_EDGE('',*,*,#57089,.T.);
#84531=ORIENTED_EDGE('',*,*,#57097,.F.);
#84532=ORIENTED_EDGE('',*,*,#57078,.T.);
#84533=ORIENTED_EDGE('',*,*,#57084,.T.);
#84534=ORIENTED_EDGE('',*,*,#57096,.F.);
#84535=ORIENTED_EDGE('',*,*,#57073,.T.);
#84536=ORIENTED_EDGE('',*,*,#57079,.T.);
#84537=ORIENTED_EDGE('',*,*,#57095,.F.);
#84538=ORIENTED_EDGE('',*,*,#57054,.F.);
#84539=ORIENTED_EDGE('',*,*,#57075,.F.);
#84540=ORIENTED_EDGE('',*,*,#57071,.F.);
#84541=ORIENTED_EDGE('',*,*,#57059,.F.);
#84542=ORIENTED_EDGE('',*,*,#57080,.F.);
#84543=ORIENTED_EDGE('',*,*,#57076,.F.);
#84544=ORIENTED_EDGE('',*,*,#57058,.F.);
#84545=ORIENTED_EDGE('',*,*,#57085,.F.);
#84546=ORIENTED_EDGE('',*,*,#57081,.F.);
#84547=ORIENTED_EDGE('',*,*,#57057,.F.);
#84548=ORIENTED_EDGE('',*,*,#57090,.F.);
#84549=ORIENTED_EDGE('',*,*,#57086,.F.);
#84550=ORIENTED_EDGE('',*,*,#57091,.F.);
#84551=ORIENTED_EDGE('',*,*,#57056,.F.);
#84552=ORIENTED_EDGE('',*,*,#57065,.F.);
#84553=ORIENTED_EDGE('',*,*,#57055,.F.);
#84554=ORIENTED_EDGE('',*,*,#57070,.F.);
#84555=ORIENTED_EDGE('',*,*,#57066,.F.);
#84556=ORIENTED_EDGE('',*,*,#56829,.F.);
#84557=ORIENTED_EDGE('',*,*,#57100,.F.);
#84558=ORIENTED_EDGE('',*,*,#57026,.F.);
#84559=ORIENTED_EDGE('',*,*,#57101,.F.);
#84560=ORIENTED_EDGE('',*,*,#56828,.T.);
#84561=ORIENTED_EDGE('',*,*,#56831,.T.);
#84562=ORIENTED_EDGE('',*,*,#56834,.T.);
#84563=ORIENTED_EDGE('',*,*,#56837,.T.);
#84564=ORIENTED_EDGE('',*,*,#56840,.T.);
#84565=ORIENTED_EDGE('',*,*,#56843,.T.);
#84566=ORIENTED_EDGE('',*,*,#56846,.T.);
#84567=ORIENTED_EDGE('',*,*,#56849,.T.);
#84568=ORIENTED_EDGE('',*,*,#56852,.T.);
#84569=ORIENTED_EDGE('',*,*,#56855,.T.);
#84570=ORIENTED_EDGE('',*,*,#56858,.T.);
#84571=ORIENTED_EDGE('',*,*,#56861,.T.);
#84572=ORIENTED_EDGE('',*,*,#56864,.T.);
#84573=ORIENTED_EDGE('',*,*,#56867,.T.);
#84574=ORIENTED_EDGE('',*,*,#56870,.T.);
#84575=ORIENTED_EDGE('',*,*,#56873,.T.);
#84576=ORIENTED_EDGE('',*,*,#56876,.T.);
#84577=ORIENTED_EDGE('',*,*,#56879,.T.);
#84578=ORIENTED_EDGE('',*,*,#56882,.T.);
#84579=ORIENTED_EDGE('',*,*,#56885,.T.);
#84580=ORIENTED_EDGE('',*,*,#57102,.T.);
#84581=ORIENTED_EDGE('',*,*,#57030,.F.);
#84582=ORIENTED_EDGE('',*,*,#57027,.F.);
#84583=ORIENTED_EDGE('',*,*,#56968,.F.);
#84584=ORIENTED_EDGE('',*,*,#56972,.F.);
#84585=ORIENTED_EDGE('',*,*,#56975,.F.);
#84586=ORIENTED_EDGE('',*,*,#56978,.F.);
#84587=ORIENTED_EDGE('',*,*,#56981,.F.);
#84588=ORIENTED_EDGE('',*,*,#56984,.F.);
#84589=ORIENTED_EDGE('',*,*,#56987,.F.);
#84590=ORIENTED_EDGE('',*,*,#56990,.F.);
#84591=ORIENTED_EDGE('',*,*,#56993,.F.);
#84592=ORIENTED_EDGE('',*,*,#56996,.F.);
#84593=ORIENTED_EDGE('',*,*,#56999,.F.);
#84594=ORIENTED_EDGE('',*,*,#57002,.F.);
#84595=ORIENTED_EDGE('',*,*,#57005,.F.);
#84596=ORIENTED_EDGE('',*,*,#57008,.F.);
#84597=ORIENTED_EDGE('',*,*,#57011,.F.);
#84598=ORIENTED_EDGE('',*,*,#57014,.F.);
#84599=ORIENTED_EDGE('',*,*,#57017,.F.);
#84600=ORIENTED_EDGE('',*,*,#57020,.F.);
#84601=ORIENTED_EDGE('',*,*,#57023,.F.);
#84602=ORIENTED_EDGE('',*,*,#57100,.T.);
#84603=ORIENTED_EDGE('',*,*,#56970,.F.);
#84604=ORIENTED_EDGE('',*,*,#57032,.F.);
#84605=ORIENTED_EDGE('',*,*,#57103,.F.);
#84606=ORIENTED_EDGE('',*,*,#56886,.F.);
#84607=ORIENTED_EDGE('',*,*,#56883,.F.);
#84608=ORIENTED_EDGE('',*,*,#56880,.F.);
#84609=ORIENTED_EDGE('',*,*,#56877,.F.);
#84610=ORIENTED_EDGE('',*,*,#56874,.F.);
#84611=ORIENTED_EDGE('',*,*,#56871,.F.);
#84612=ORIENTED_EDGE('',*,*,#56868,.F.);
#84613=ORIENTED_EDGE('',*,*,#56865,.F.);
#84614=ORIENTED_EDGE('',*,*,#56862,.F.);
#84615=ORIENTED_EDGE('',*,*,#56859,.F.);
#84616=ORIENTED_EDGE('',*,*,#56856,.F.);
#84617=ORIENTED_EDGE('',*,*,#56853,.F.);
#84618=ORIENTED_EDGE('',*,*,#56850,.F.);
#84619=ORIENTED_EDGE('',*,*,#56847,.F.);
#84620=ORIENTED_EDGE('',*,*,#56844,.F.);
#84621=ORIENTED_EDGE('',*,*,#56841,.F.);
#84622=ORIENTED_EDGE('',*,*,#56838,.F.);
#84623=ORIENTED_EDGE('',*,*,#56835,.F.);
#84624=ORIENTED_EDGE('',*,*,#56832,.F.);
#84625=ORIENTED_EDGE('',*,*,#57101,.T.);
#84626=ORIENTED_EDGE('',*,*,#57025,.F.);
#84627=ORIENTED_EDGE('',*,*,#57024,.F.);
#84628=ORIENTED_EDGE('',*,*,#57021,.F.);
#84629=ORIENTED_EDGE('',*,*,#57018,.F.);
#84630=ORIENTED_EDGE('',*,*,#57015,.F.);
#84631=ORIENTED_EDGE('',*,*,#57012,.F.);
#84632=ORIENTED_EDGE('',*,*,#57009,.F.);
#84633=ORIENTED_EDGE('',*,*,#57006,.F.);
#84634=ORIENTED_EDGE('',*,*,#57003,.F.);
#84635=ORIENTED_EDGE('',*,*,#57000,.F.);
#84636=ORIENTED_EDGE('',*,*,#56997,.F.);
#84637=ORIENTED_EDGE('',*,*,#56994,.F.);
#84638=ORIENTED_EDGE('',*,*,#56991,.F.);
#84639=ORIENTED_EDGE('',*,*,#56988,.F.);
#84640=ORIENTED_EDGE('',*,*,#56985,.F.);
#84641=ORIENTED_EDGE('',*,*,#56982,.F.);
#84642=ORIENTED_EDGE('',*,*,#56979,.F.);
#84643=ORIENTED_EDGE('',*,*,#56976,.F.);
#84644=ORIENTED_EDGE('',*,*,#56973,.F.);
#84645=ORIENTED_EDGE('',*,*,#56884,.T.);
#84646=ORIENTED_EDGE('',*,*,#57103,.T.);
#84647=ORIENTED_EDGE('',*,*,#57031,.F.);
#84648=ORIENTED_EDGE('',*,*,#57102,.F.);
#84649=ORIENTED_EDGE('',*,*,#57104,.F.);
#84650=ORIENTED_EDGE('',*,*,#57105,.T.);
#84651=ORIENTED_EDGE('',*,*,#57106,.T.);
#84652=ORIENTED_EDGE('',*,*,#57105,.F.);
#84653=ORIENTED_EDGE('',*,*,#57107,.F.);
#84654=ORIENTED_EDGE('',*,*,#57108,.T.);
#84655=ORIENTED_EDGE('',*,*,#57109,.T.);
#84656=ORIENTED_EDGE('',*,*,#57108,.F.);
#84657=ORIENTED_EDGE('',*,*,#57110,.F.);
#84658=ORIENTED_EDGE('',*,*,#57111,.T.);
#84659=ORIENTED_EDGE('',*,*,#57112,.T.);
#84660=ORIENTED_EDGE('',*,*,#57111,.F.);
#84661=ORIENTED_EDGE('',*,*,#57113,.F.);
#84662=ORIENTED_EDGE('',*,*,#57114,.T.);
#84663=ORIENTED_EDGE('',*,*,#57115,.T.);
#84664=ORIENTED_EDGE('',*,*,#57114,.F.);
#84665=ORIENTED_EDGE('',*,*,#57116,.F.);
#84666=ORIENTED_EDGE('',*,*,#57117,.T.);
#84667=ORIENTED_EDGE('',*,*,#57118,.T.);
#84668=ORIENTED_EDGE('',*,*,#57117,.F.);
#84669=ORIENTED_EDGE('',*,*,#57119,.F.);
#84670=ORIENTED_EDGE('',*,*,#57120,.T.);
#84671=ORIENTED_EDGE('',*,*,#57121,.T.);
#84672=ORIENTED_EDGE('',*,*,#57120,.F.);
#84673=ORIENTED_EDGE('',*,*,#57122,.F.);
#84674=ORIENTED_EDGE('',*,*,#57123,.T.);
#84675=ORIENTED_EDGE('',*,*,#57124,.T.);
#84676=ORIENTED_EDGE('',*,*,#57123,.F.);
#84677=ORIENTED_EDGE('',*,*,#57125,.F.);
#84678=ORIENTED_EDGE('',*,*,#57126,.T.);
#84679=ORIENTED_EDGE('',*,*,#57127,.T.);
#84680=ORIENTED_EDGE('',*,*,#57126,.F.);
#84681=ORIENTED_EDGE('',*,*,#57128,.F.);
#84682=ORIENTED_EDGE('',*,*,#57129,.T.);
#84683=ORIENTED_EDGE('',*,*,#57130,.T.);
#84684=ORIENTED_EDGE('',*,*,#57129,.F.);
#84685=ORIENTED_EDGE('',*,*,#57131,.F.);
#84686=ORIENTED_EDGE('',*,*,#57132,.T.);
#84687=ORIENTED_EDGE('',*,*,#57133,.F.);
#84688=ORIENTED_EDGE('',*,*,#57132,.F.);
#84689=ORIENTED_EDGE('',*,*,#57134,.F.);
#84690=ORIENTED_EDGE('',*,*,#57135,.T.);
#84691=ORIENTED_EDGE('',*,*,#57136,.T.);
#84692=ORIENTED_EDGE('',*,*,#57135,.F.);
#84693=ORIENTED_EDGE('',*,*,#57137,.F.);
#84694=ORIENTED_EDGE('',*,*,#57138,.T.);
#84695=ORIENTED_EDGE('',*,*,#57139,.F.);
#84696=ORIENTED_EDGE('',*,*,#57140,.T.);
#84697=ORIENTED_EDGE('',*,*,#57141,.F.);
#84698=ORIENTED_EDGE('',*,*,#57140,.F.);
#84699=ORIENTED_EDGE('',*,*,#57142,.F.);
#84700=ORIENTED_EDGE('',*,*,#57143,.T.);
#84701=ORIENTED_EDGE('',*,*,#57144,.F.);
#84702=ORIENTED_EDGE('',*,*,#57145,.F.);
#84703=ORIENTED_EDGE('',*,*,#57143,.F.);
#84704=ORIENTED_EDGE('',*,*,#57138,.F.);
#84705=ORIENTED_EDGE('',*,*,#57146,.T.);
#84706=ORIENTED_EDGE('',*,*,#57144,.T.);
#84707=ORIENTED_EDGE('',*,*,#57145,.T.);
#84708=ORIENTED_EDGE('',*,*,#57146,.F.);
#84709=ORIENTED_EDGE('',*,*,#57147,.F.);
#84710=ORIENTED_EDGE('',*,*,#57148,.T.);
#84711=ORIENTED_EDGE('',*,*,#57149,.T.);
#84712=ORIENTED_EDGE('',*,*,#57148,.F.);
#84713=ORIENTED_EDGE('',*,*,#57149,.F.);
#84714=ORIENTED_EDGE('',*,*,#57150,.T.);
#84715=ORIENTED_EDGE('',*,*,#57139,.T.);
#84716=ORIENTED_EDGE('',*,*,#57150,.F.);
#84717=ORIENTED_EDGE('',*,*,#57133,.T.);
#84718=ORIENTED_EDGE('',*,*,#57141,.T.);
#84719=ORIENTED_EDGE('',*,*,#57147,.T.);
#84720=ORIENTED_EDGE('',*,*,#57142,.T.);
#84721=ORIENTED_EDGE('',*,*,#57134,.T.);
#84722=ORIENTED_EDGE('',*,*,#57136,.F.);
#84723=ORIENTED_EDGE('',*,*,#57137,.T.);
#84724=ORIENTED_EDGE('',*,*,#57128,.T.);
#84725=ORIENTED_EDGE('',*,*,#57125,.T.);
#84726=ORIENTED_EDGE('',*,*,#57122,.T.);
#84727=ORIENTED_EDGE('',*,*,#57119,.T.);
#84728=ORIENTED_EDGE('',*,*,#57116,.T.);
#84729=ORIENTED_EDGE('',*,*,#57113,.T.);
#84730=ORIENTED_EDGE('',*,*,#57110,.T.);
#84731=ORIENTED_EDGE('',*,*,#57107,.T.);
#84732=ORIENTED_EDGE('',*,*,#57104,.T.);
#84733=ORIENTED_EDGE('',*,*,#57131,.T.);
#84734=ORIENTED_EDGE('',*,*,#57106,.F.);
#84735=ORIENTED_EDGE('',*,*,#57109,.F.);
#84736=ORIENTED_EDGE('',*,*,#57112,.F.);
#84737=ORIENTED_EDGE('',*,*,#57115,.F.);
#84738=ORIENTED_EDGE('',*,*,#57118,.F.);
#84739=ORIENTED_EDGE('',*,*,#57121,.F.);
#84740=ORIENTED_EDGE('',*,*,#57124,.F.);
#84741=ORIENTED_EDGE('',*,*,#57127,.F.);
#84742=ORIENTED_EDGE('',*,*,#57130,.F.);
#87787=CYLINDRICAL_SURFACE('',#104249,10.0514428414941);
#87788=CYLINDRICAL_SURFACE('',#104251,10.0514428414941);
#87789=CYLINDRICAL_SURFACE('',#104253,10.0514428414941);
#87790=CYLINDRICAL_SURFACE('',#104254,10.0514428414941);
#87791=CYLINDRICAL_SURFACE('',#104255,10.0514428414941);
#87792=CYLINDRICAL_SURFACE('',#104259,12.);
#87793=CYLINDRICAL_SURFACE('',#104261,12.);
#87794=CYLINDRICAL_SURFACE('',#104263,12.);
#87795=CYLINDRICAL_SURFACE('',#104264,12.);
#87796=CYLINDRICAL_SURFACE('',#104265,12.);
#87797=CYLINDRICAL_SURFACE('',#104266,12.);
#87798=CYLINDRICAL_SURFACE('',#104268,12.);
#87799=CYLINDRICAL_SURFACE('',#104305,10.0514428414941);
#87800=CYLINDRICAL_SURFACE('',#104306,10.0514428414941);
#87801=CYLINDRICAL_SURFACE('',#104308,10.0514428414941);
#87802=CYLINDRICAL_SURFACE('',#104309,10.0514428414941);
#87803=CYLINDRICAL_SURFACE('',#104310,10.0514428414941);
#87804=CYLINDRICAL_SURFACE('',#104311,10.0514428414941);
#87805=CYLINDRICAL_SURFACE('',#104312,10.0514428414941);
#87806=CYLINDRICAL_SURFACE('',#104314,12.);
#87807=CYLINDRICAL_SURFACE('',#104316,12.);
#87808=CYLINDRICAL_SURFACE('',#104317,12.);
#87809=CYLINDRICAL_SURFACE('',#104318,12.);
#87810=CYLINDRICAL_SURFACE('',#104319,12.);
#87811=CYLINDRICAL_SURFACE('',#104320,12.);
#87812=CYLINDRICAL_SURFACE('',#104321,12.);
#87813=CYLINDRICAL_SURFACE('',#104323,12.);
#87814=CYLINDRICAL_SURFACE('',#104347,10.0514428414941);
#87815=CYLINDRICAL_SURFACE('',#104348,10.0514428414941);
#87816=CYLINDRICAL_SURFACE('',#104353,12.);
#87817=CYLINDRICAL_SURFACE('',#104355,10.0514428414941);
#87818=CYLINDRICAL_SURFACE('',#104358,10.0514428414941);
#87819=CYLINDRICAL_SURFACE('',#104360,10.0514428414941);
#87820=CYLINDRICAL_SURFACE('',#104361,10.0514428414941);
#87821=CYLINDRICAL_SURFACE('',#104362,10.0514428414941);
#87822=CYLINDRICAL_SURFACE('',#104363,10.0514428414941);
#87823=CYLINDRICAL_SURFACE('',#104364,10.0514428414941);
#87824=CYLINDRICAL_SURFACE('',#104365,10.0514428414941);
#87825=CYLINDRICAL_SURFACE('',#104366,10.0514428414941);
#87826=CYLINDRICAL_SURFACE('',#104367,10.0514428414941);
#87827=CYLINDRICAL_SURFACE('',#104368,10.0514428414941);
#87828=CYLINDRICAL_SURFACE('',#104369,10.0514428414941);
#87829=CYLINDRICAL_SURFACE('',#104370,10.0514428414941);
#87830=CYLINDRICAL_SURFACE('',#104371,10.0514428414941);
#87831=CYLINDRICAL_SURFACE('',#104372,10.0514428414941);
#87832=CYLINDRICAL_SURFACE('',#104373,10.0514428414941);
#87833=CYLINDRICAL_SURFACE('',#104374,10.0514428414941);
#87834=CYLINDRICAL_SURFACE('',#104375,10.0514428414941);
#87835=CYLINDRICAL_SURFACE('',#104376,10.0514428414941);
#87836=CYLINDRICAL_SURFACE('',#104377,10.0514428414941);
#87837=CYLINDRICAL_SURFACE('',#104378,10.0514428414941);
#87838=CYLINDRICAL_SURFACE('',#104379,10.0514428414941);
#87839=CYLINDRICAL_SURFACE('',#104381,10.0514428414941);
#87840=CYLINDRICAL_SURFACE('',#104382,10.0514428414941);
#87841=CYLINDRICAL_SURFACE('',#104383,10.0514428414941);
#87842=CYLINDRICAL_SURFACE('',#104384,10.0514428414941);
#87843=CYLINDRICAL_SURFACE('',#104385,10.0514428414941);
#87844=CYLINDRICAL_SURFACE('',#104386,10.0514428414941);
#87845=CYLINDRICAL_SURFACE('',#104387,10.0514428414941);
#87846=CYLINDRICAL_SURFACE('',#104388,10.0514428414941);
#87847=CYLINDRICAL_SURFACE('',#104389,10.0514428414941);
#87848=CYLINDRICAL_SURFACE('',#104390,10.0514428414941);
#87849=CYLINDRICAL_SURFACE('',#104391,10.0514428414941);
#87850=CYLINDRICAL_SURFACE('',#104392,10.0514428414941);
#87851=CYLINDRICAL_SURFACE('',#104393,12.);
#87852=CYLINDRICAL_SURFACE('',#104395,12.);
#87853=CYLINDRICAL_SURFACE('',#104396,12.);
#87854=CYLINDRICAL_SURFACE('',#104397,12.);
#87855=CYLINDRICAL_SURFACE('',#104398,12.);
#87856=CYLINDRICAL_SURFACE('',#104399,12.);
#87857=CYLINDRICAL_SURFACE('',#104400,12.);
#87858=CYLINDRICAL_SURFACE('',#104401,12.);
#87859=CYLINDRICAL_SURFACE('',#104402,12.);
#87860=CYLINDRICAL_SURFACE('',#104403,12.);
#87861=CYLINDRICAL_SURFACE('',#104404,12.);
#87862=CYLINDRICAL_SURFACE('',#104405,12.);
#87863=CYLINDRICAL_SURFACE('',#104406,12.);
#87864=CYLINDRICAL_SURFACE('',#104407,12.);
#87865=CYLINDRICAL_SURFACE('',#104409,12.);
#87866=CYLINDRICAL_SURFACE('',#104410,12.);
#87867=CYLINDRICAL_SURFACE('',#104411,12.);
#87868=CYLINDRICAL_SURFACE('',#104412,12.);
#87869=CYLINDRICAL_SURFACE('',#104413,12.);
#87870=CYLINDRICAL_SURFACE('',#104414,12.);
#87871=CYLINDRICAL_SURFACE('',#104415,12.);
#87872=CYLINDRICAL_SURFACE('',#104416,12.);
#87873=CYLINDRICAL_SURFACE('',#104417,12.);
#87874=CYLINDRICAL_SURFACE('',#104418,12.);
#87875=CYLINDRICAL_SURFACE('',#104419,12.);
#87876=CYLINDRICAL_SURFACE('',#104420,12.);
#87877=CYLINDRICAL_SURFACE('',#104421,12.);
#87878=CYLINDRICAL_SURFACE('',#104422,12.);
#87879=CYLINDRICAL_SURFACE('',#104423,12.);
#87880=CYLINDRICAL_SURFACE('',#104424,12.);
#87881=CYLINDRICAL_SURFACE('',#104425,12.);
#87882=CYLINDRICAL_SURFACE('',#104426,12.);
#87883=CYLINDRICAL_SURFACE('',#104427,12.);
#87884=CYLINDRICAL_SURFACE('',#104435,12.);
#87885=CYLINDRICAL_SURFACE('',#104437,10.0514428414941);
#87886=CYLINDRICAL_SURFACE('',#104477,10.0514428414941);
#87887=CYLINDRICAL_SURFACE('',#104478,1.190625);
#87888=CYLINDRICAL_SURFACE('',#104481,1.190625);
#87889=CYLINDRICAL_SURFACE('',#104484,1.190625);
#87890=CYLINDRICAL_SURFACE('',#104487,1.19062499999999);
#87891=CYLINDRICAL_SURFACE('',#104490,1.190625);
#87892=CYLINDRICAL_SURFACE('',#104493,1.190625);
#87893=CYLINDRICAL_SURFACE('',#104496,1.190625);
#87894=CYLINDRICAL_SURFACE('',#104499,1.190625);
#87895=CYLINDRICAL_SURFACE('',#104502,1.190625);
#87896=CYLINDRICAL_SURFACE('',#104505,55.2538194444444);
#87897=CYLINDRICAL_SURFACE('',#104508,44.5707880434783);
#87898=CYLINDRICAL_SURFACE('',#104523,16.8332621659243);
#87899=CYLINDRICAL_SURFACE('',#104528,44.5707880434783);
#93297=ADVANCED_FACE('',(#14018),#87787,.F.);
#93298=ADVANCED_FACE('',(#14019),#87788,.F.);
#93299=ADVANCED_FACE('',(#14020),#87789,.F.);
#93300=ADVANCED_FACE('',(#14021),#87790,.F.);
#93301=ADVANCED_FACE('',(#14022),#87791,.F.);
#93302=ADVANCED_FACE('',(#14023),#7164,.F.);
#93303=ADVANCED_FACE('',(#14024),#7165,.F.);
#93304=ADVANCED_FACE('',(#14025),#87792,.F.);
#93305=ADVANCED_FACE('',(#14026),#87793,.F.);
#93306=ADVANCED_FACE('',(#14027),#87794,.F.);
#93307=ADVANCED_FACE('',(#14028),#87795,.F.);
#93308=ADVANCED_FACE('',(#14029),#87796,.F.);
#93309=ADVANCED_FACE('',(#14030),#87797,.F.);
#93310=ADVANCED_FACE('',(#14031),#87798,.F.);
#93311=ADVANCED_FACE('',(#14032),#7166,.F.);
#93312=ADVANCED_FACE('',(#14033),#7167,.F.);
#93313=ADVANCED_FACE('',(#14034,#7652),#8569,.F.);
#93314=ADVANCED_FACE('',(#14035),#8570,.T.);
#93315=ADVANCED_FACE('',(#14036),#8571,.T.);
#93316=ADVANCED_FACE('',(#14037),#8572,.T.);
#93317=ADVANCED_FACE('',(#14038),#8573,.T.);
#93318=ADVANCED_FACE('',(#14039),#8574,.T.);
#93319=ADVANCED_FACE('',(#14040),#8575,.T.);
#93320=ADVANCED_FACE('',(#14041,#7653),#8576,.T.);
#93321=ADVANCED_FACE('',(#14042),#7168,.T.);
#93322=ADVANCED_FACE('',(#14043),#7169,.T.);
#93323=ADVANCED_FACE('',(#14044),#7170,.T.);
#93324=ADVANCED_FACE('',(#14045),#7171,.T.);
#93325=ADVANCED_FACE('',(#14046),#7172,.T.);
#93326=ADVANCED_FACE('',(#14047),#7173,.T.);
#93327=ADVANCED_FACE('',(#14048),#7174,.T.);
#93328=ADVANCED_FACE('',(#14049),#7175,.T.);
#93329=ADVANCED_FACE('',(#14050),#7176,.T.);
#93330=ADVANCED_FACE('',(#14051),#7177,.T.);
#93331=ADVANCED_FACE('',(#14052),#7178,.T.);
#93332=ADVANCED_FACE('',(#14053),#7179,.T.);
#93333=ADVANCED_FACE('',(#14054),#3192,.T.);
#93334=ADVANCED_FACE('',(#14055),#3193,.T.);
#93335=ADVANCED_FACE('',(#14056),#87799,.F.);
#93336=ADVANCED_FACE('',(#14057),#87800,.F.);
#93337=ADVANCED_FACE('',(#14058),#87801,.F.);
#93338=ADVANCED_FACE('',(#14059),#87802,.F.);
#93339=ADVANCED_FACE('',(#14060),#87803,.F.);
#93340=ADVANCED_FACE('',(#14061),#87804,.F.);
#93341=ADVANCED_FACE('',(#14062),#87805,.F.);
#93342=ADVANCED_FACE('',(#14063),#87806,.F.);
#93343=ADVANCED_FACE('',(#14064),#87807,.F.);
#93344=ADVANCED_FACE('',(#14065),#87808,.F.);
#93345=ADVANCED_FACE('',(#14066),#87809,.F.);
#93346=ADVANCED_FACE('',(#14067),#87810,.F.);
#93347=ADVANCED_FACE('',(#14068),#87811,.F.);
#93348=ADVANCED_FACE('',(#14069),#87812,.F.);
#93349=ADVANCED_FACE('',(#14070),#87813,.F.);
#93350=ADVANCED_FACE('',(#14071),#1065,.T.);
#93351=ADVANCED_FACE('',(#14072,#7654),#1066,.T.);
#93352=ADVANCED_FACE('',(#14073),#7180,.T.);
#93353=ADVANCED_FACE('',(#14074),#7181,.F.);
#93354=ADVANCED_FACE('',(#14075,#7655),#8577,.T.);
#93355=ADVANCED_FACE('',(#14076),#8578,.F.);
#93356=ADVANCED_FACE('',(#14077),#8579,.F.);
#93357=ADVANCED_FACE('',(#14078),#8580,.F.);
#93358=ADVANCED_FACE('',(#14079),#8581,.F.);
#93359=ADVANCED_FACE('',(#14080),#8582,.F.);
#93360=ADVANCED_FACE('',(#14081),#8583,.F.);
#93361=ADVANCED_FACE('',(#14082,#7656),#8584,.T.);
#93362=ADVANCED_FACE('',(#14083),#8585,.T.);
#93363=ADVANCED_FACE('',(#14084),#3194,.T.);
#93364=ADVANCED_FACE('',(#14085),#3195,.T.);
#93365=ADVANCED_FACE('',(#14086),#87814,.F.);
#93366=ADVANCED_FACE('',(#14087),#87815,.T.);
#93367=ADVANCED_FACE('',(#14088),#7182,.F.);
#93368=ADVANCED_FACE('',(#14089),#87816,.T.);
#93369=ADVANCED_FACE('',(#14090),#3196,.F.);
#93370=ADVANCED_FACE('',(#14091),#3197,.F.);
#93371=ADVANCED_FACE('',(#14092),#87817,.T.);
#93372=ADVANCED_FACE('',(#14093,#7657),#8586,.T.);
#93373=ADVANCED_FACE('',(#14094),#87818,.T.);
#93374=ADVANCED_FACE('',(#14095),#87819,.T.);
#93375=ADVANCED_FACE('',(#14096),#87820,.T.);
#93376=ADVANCED_FACE('',(#14097),#87821,.T.);
#93377=ADVANCED_FACE('',(#14098),#87822,.T.);
#93378=ADVANCED_FACE('',(#14099),#87823,.T.);
#93379=ADVANCED_FACE('',(#14100),#87824,.T.);
#93380=ADVANCED_FACE('',(#14101),#87825,.T.);
#93381=ADVANCED_FACE('',(#14102),#87826,.T.);
#93382=ADVANCED_FACE('',(#14103),#87827,.T.);
#93383=ADVANCED_FACE('',(#14104),#87828,.T.);
#93384=ADVANCED_FACE('',(#14105),#87829,.T.);
#93385=ADVANCED_FACE('',(#14106),#87830,.T.);
#93386=ADVANCED_FACE('',(#14107),#87831,.T.);
#93387=ADVANCED_FACE('',(#14108),#87832,.T.);
#93388=ADVANCED_FACE('',(#14109),#87833,.T.);
#93389=ADVANCED_FACE('',(#14110),#87834,.T.);
#93390=ADVANCED_FACE('',(#14111),#87835,.T.);
#93391=ADVANCED_FACE('',(#14112),#87836,.T.);
#93392=ADVANCED_FACE('',(#14113),#87837,.T.);
#93393=ADVANCED_FACE('',(#14114),#87838,.T.);
#93394=ADVANCED_FACE('',(#14115),#87839,.T.);
#93395=ADVANCED_FACE('',(#14116),#87840,.T.);
#93396=ADVANCED_FACE('',(#14117),#87841,.T.);
#93397=ADVANCED_FACE('',(#14118),#87842,.T.);
#93398=ADVANCED_FACE('',(#14119),#87843,.T.);
#93399=ADVANCED_FACE('',(#14120),#87844,.T.);
#93400=ADVANCED_FACE('',(#14121),#87845,.T.);
#93401=ADVANCED_FACE('',(#14122),#87846,.T.);
#93402=ADVANCED_FACE('',(#14123),#87847,.T.);
#93403=ADVANCED_FACE('',(#14124),#87848,.T.);
#93404=ADVANCED_FACE('',(#14125),#87849,.T.);
#93405=ADVANCED_FACE('',(#14126),#87850,.T.);
#93406=ADVANCED_FACE('',(#14127),#87851,.T.);
#93407=ADVANCED_FACE('',(#14128),#87852,.T.);
#93408=ADVANCED_FACE('',(#14129),#87853,.T.);
#93409=ADVANCED_FACE('',(#14130),#87854,.T.);
#93410=ADVANCED_FACE('',(#14131),#87855,.T.);
#93411=ADVANCED_FACE('',(#14132),#87856,.T.);
#93412=ADVANCED_FACE('',(#14133),#87857,.T.);
#93413=ADVANCED_FACE('',(#14134),#87858,.T.);
#93414=ADVANCED_FACE('',(#14135),#87859,.T.);
#93415=ADVANCED_FACE('',(#14136),#87860,.T.);
#93416=ADVANCED_FACE('',(#14137),#87861,.T.);
#93417=ADVANCED_FACE('',(#14138),#87862,.T.);
#93418=ADVANCED_FACE('',(#14139),#87863,.T.);
#93419=ADVANCED_FACE('',(#14140),#87864,.T.);
#93420=ADVANCED_FACE('',(#14141),#87865,.T.);
#93421=ADVANCED_FACE('',(#14142),#87866,.T.);
#93422=ADVANCED_FACE('',(#14143),#87867,.T.);
#93423=ADVANCED_FACE('',(#14144),#87868,.T.);
#93424=ADVANCED_FACE('',(#14145),#87869,.T.);
#93425=ADVANCED_FACE('',(#14146),#87870,.T.);
#93426=ADVANCED_FACE('',(#14147),#87871,.T.);
#93427=ADVANCED_FACE('',(#14148),#87872,.T.);
#93428=ADVANCED_FACE('',(#14149),#87873,.T.);
#93429=ADVANCED_FACE('',(#14150),#87874,.T.);
#93430=ADVANCED_FACE('',(#14151),#87875,.T.);
#93431=ADVANCED_FACE('',(#14152),#87876,.T.);
#93432=ADVANCED_FACE('',(#14153),#87877,.T.);
#93433=ADVANCED_FACE('',(#14154),#87878,.T.);
#93434=ADVANCED_FACE('',(#14155),#87879,.T.);
#93435=ADVANCED_FACE('',(#14156),#87880,.T.);
#93436=ADVANCED_FACE('',(#14157),#87881,.T.);
#93437=ADVANCED_FACE('',(#14158),#87882,.T.);
#93438=ADVANCED_FACE('',(#14159),#87883,.T.);
#93439=ADVANCED_FACE('',(#14160),#7183,.F.);
#93440=ADVANCED_FACE('',(#14161),#7184,.T.);
#93441=ADVANCED_FACE('',(#14162),#87884,.T.);
#93442=ADVANCED_FACE('',(#14163),#3198,.F.);
#93443=ADVANCED_FACE('',(#14164),#3199,.F.);
#93444=ADVANCED_FACE('',(#14165),#87885,.T.);
#93445=ADVANCED_FACE('',(#14166),#8587,.T.);
#93446=ADVANCED_FACE('',(#14167,#7658),#8588,.F.);
#93447=ADVANCED_FACE('',(#14168,#7659),#8589,.T.);
#93448=ADVANCED_FACE('',(#14169),#8590,.F.);
#93449=ADVANCED_FACE('',(#14170),#8591,.F.);
#93450=ADVANCED_FACE('',(#14171),#8592,.F.);
#93451=ADVANCED_FACE('',(#14172),#8593,.F.);
#93452=ADVANCED_FACE('',(#14173),#8594,.T.);
#93453=ADVANCED_FACE('',(#14174),#8595,.T.);
#93454=ADVANCED_FACE('',(#14175),#8596,.T.);
#93455=ADVANCED_FACE('',(#14176),#8597,.T.);
#93456=ADVANCED_FACE('',(#14177),#8598,.T.);
#93457=ADVANCED_FACE('',(#14178),#8599,.T.);
#93458=ADVANCED_FACE('',(#14179,#7660),#8600,.F.);
#93459=ADVANCED_FACE('',(#14180),#7185,.T.);
#93460=ADVANCED_FACE('',(#14181),#7186,.T.);
#93461=ADVANCED_FACE('',(#14182),#7187,.T.);
#93462=ADVANCED_FACE('',(#14183),#7188,.T.);
#93463=ADVANCED_FACE('',(#14184),#7189,.T.);
#93464=ADVANCED_FACE('',(#14185),#7190,.T.);
#93465=ADVANCED_FACE('',(#14186),#7191,.T.);
#93466=ADVANCED_FACE('',(#14187),#7192,.T.);
#93467=ADVANCED_FACE('',(#14188),#7193,.T.);
#93468=ADVANCED_FACE('',(#14189),#7194,.T.);
#93469=ADVANCED_FACE('',(#14190),#7195,.T.);
#93470=ADVANCED_FACE('',(#14191),#7196,.T.);
#93471=ADVANCED_FACE('',(#14192),#8601,.F.);
#93472=ADVANCED_FACE('',(#14193),#3200,.F.);
#93473=ADVANCED_FACE('',(#14194),#3201,.F.);
#93474=ADVANCED_FACE('',(#14195),#87886,.T.);
#93475=ADVANCED_FACE('',(#14196),#87887,.F.);
#93476=ADVANCED_FACE('',(#14197),#87888,.F.);
#93477=ADVANCED_FACE('',(#14198),#87889,.F.);
#93478=ADVANCED_FACE('',(#14199),#87890,.F.);
#93479=ADVANCED_FACE('',(#14200),#87891,.F.);
#93480=ADVANCED_FACE('',(#14201),#87892,.F.);
#93481=ADVANCED_FACE('',(#14202),#87893,.F.);
#93482=ADVANCED_FACE('',(#14203),#87894,.F.);
#93483=ADVANCED_FACE('',(#14204),#87895,.F.);
#93484=ADVANCED_FACE('',(#14205),#87896,.T.);
#93485=ADVANCED_FACE('',(#14206),#87897,.F.);
#93486=ADVANCED_FACE('',(#14207,#7661),#1067,.F.);
#93487=ADVANCED_FACE('',(#14208),#4124,.T.);
#93488=ADVANCED_FACE('',(#14209),#4125,.T.);
#93489=ADVANCED_FACE('',(#14210),#87898,.F.);
#93490=ADVANCED_FACE('',(#14211),#4126,.F.);
#93491=ADVANCED_FACE('',(#14212),#87899,.F.);
#93492=ADVANCED_FACE('',(#14213,#7662),#8602,.T.);
#93493=ADVANCED_FACE('',(#14214,#7663),#8603,.F.);
#93494=ADVANCED_FACE('',(#14215),#8604,.F.);
#93495=ADVANCED_FACE('',(#14216,#7664),#8605,.F.);
#93496=ADVANCED_FACE('',(#14217),#8606,.T.);
#93497=ADVANCED_FACE('',(#14218),#8607,.T.);
#93498=ADVANCED_FACE('',(#14219),#8608,.T.);
#93499=ADVANCED_FACE('',(#14220),#8609,.T.);
#93500=ADVANCED_FACE('',(#14221),#8610,.T.);
#93501=ADVANCED_FACE('',(#14222),#8611,.T.);
#93502=ADVANCED_FACE('',(#14223),#8612,.T.);
#93503=ADVANCED_FACE('',(#14224),#8613,.T.);
#93504=ADVANCED_FACE('',(#14225),#8614,.T.);
#93505=ADVANCED_FACE('',(#14226,#7665,#7666,#7667,#7668,#7669,#7670,#7671,
#7672,#7673),#8615,.F.);
#93764=CLOSED_SHELL('',(#93297,#93298,#93299,#93300,#93301,#93302,#93303,
#93304,#93305,#93306,#93307,#93308,#93309,#93310,#93311,#93312,#93313,#93314,
#93315,#93316,#93317,#93318,#93319,#93320,#93321,#93322,#93323,#93324,#93325,
#93326,#93327,#93328,#93329,#93330,#93331,#93332,#93333,#93334,#93335));
#93765=CLOSED_SHELL('',(#93336,#93337,#93338,#93339,#93340,#93341,#93342,
#93343,#93344,#93345,#93346,#93347,#93348,#93349,#93350,#93351,#93352,#93353,
#93354,#93355,#93356,#93357,#93358,#93359,#93360,#93361,#93362,#93363,#93364,
#93365));
#93766=CLOSED_SHELL('',(#93366,#93367,#93368,#93369,#93370,#93371,#93372));
#93767=CLOSED_SHELL('',(#93373,#93374,#93375,#93376,#93377,#93378,#93379,
#93380,#93381,#93382,#93383,#93384,#93385,#93386,#93387,#93388,#93389,#93390,
#93391,#93392,#93393,#93394,#93395,#93396,#93397,#93398,#93399,#93400,#93401,
#93402,#93403,#93404,#93405,#93406,#93407,#93408,#93409,#93410,#93411,#93412,
#93413,#93414,#93415,#93416,#93417,#93418,#93419,#93420,#93421,#93422,#93423,
#93424,#93425,#93426,#93427,#93428,#93429,#93430,#93431,#93432,#93433,#93434,
#93435,#93436,#93437,#93438,#93439,#93440,#93441,#93442,#93443,#93444,#93445,
#93446,#93447,#93448,#93449,#93450,#93451,#93452,#93453,#93454,#93455,#93456,
#93457,#93458,#93459,#93460,#93461,#93462,#93463,#93464,#93465,#93466,#93467,
#93468,#93469,#93470,#93471,#93472,#93473,#93474));
#93768=CLOSED_SHELL('',(#93475,#93476,#93477,#93478,#93479,#93480,#93481,
#93482,#93483,#93484,#93485,#93486,#93487,#93488,#93489,#93490,#93491,#93492,
#93493,#93494,#93495,#93496,#93497,#93498,#93499,#93500,#93501,#93502,#93503,
#93504,#93505));
#104248=AXIS2_PLACEMENT_3D('',#275559,#129415,#129416);
#104249=AXIS2_PLACEMENT_3D('',#275560,#129417,#129418);
#104250=AXIS2_PLACEMENT_3D('',#275565,#129420,#129421);
#104251=AXIS2_PLACEMENT_3D('',#275569,#129422,#129423);
#104252=AXIS2_PLACEMENT_3D('',#275593,#129425,#129426);
#104253=AXIS2_PLACEMENT_3D('',#275615,#129427,#129428);
#104254=AXIS2_PLACEMENT_3D('',#275661,#129430,#129431);
#104255=AXIS2_PLACEMENT_3D('',#275707,#129433,#129434);
#104256=AXIS2_PLACEMENT_3D('',#275722,#129436,#129437);
#104257=AXIS2_PLACEMENT_3D('',#275734,#129438,#129439);
#104258=AXIS2_PLACEMENT_3D('',#275745,#129441,#129442);
#104259=AXIS2_PLACEMENT_3D('',#275763,#129444,#129445);
#104260=AXIS2_PLACEMENT_3D('',#275768,#129447,#129448);
#104261=AXIS2_PLACEMENT_3D('',#275777,#129449,#129450);
#104262=AXIS2_PLACEMENT_3D('',#275818,#129452,#129453);
#104263=AXIS2_PLACEMENT_3D('',#275855,#129454,#129455);
#104264=AXIS2_PLACEMENT_3D('',#275931,#129457,#129458);
#104265=AXIS2_PLACEMENT_3D('',#276007,#129460,#129461);
#104266=AXIS2_PLACEMENT_3D('',#276083,#129463,#129464);
#104267=AXIS2_PLACEMENT_3D('',#276109,#129466,#129467);
#104268=AXIS2_PLACEMENT_3D('',#276134,#129468,#129469);
#104269=AXIS2_PLACEMENT_3D('',#276211,#129470,#129471);
#104270=AXIS2_PLACEMENT_3D('',#276222,#129473,#129474);
#104271=AXIS2_PLACEMENT_3D('',#276261,#129475,#129476);
#104272=AXIS2_PLACEMENT_3D('',#276279,#129478,#129479);
#104273=AXIS2_PLACEMENT_3D('',#276318,#129480,#129481);
#104274=AXIS2_PLACEMENT_3D('',#276321,#129482,#129483);
#104275=AXIS2_PLACEMENT_3D('',#276323,#129484,#129485);
#104276=AXIS2_PLACEMENT_3D('',#276325,#129486,#129487);
#104277=AXIS2_PLACEMENT_3D('',#276327,#129488,#129489);
#104278=AXIS2_PLACEMENT_3D('',#276329,#129490,#129491);
#104279=AXIS2_PLACEMENT_3D('',#276330,#129492,#129493);
#104280=AXIS2_PLACEMENT_3D('',#276331,#129494,#129495);
#104281=AXIS2_PLACEMENT_3D('',#276351,#129498,#129499);
#104282=AXIS2_PLACEMENT_3D('',#276368,#129501,#129502);
#104283=AXIS2_PLACEMENT_3D('',#276385,#129504,#129505);
#104284=AXIS2_PLACEMENT_3D('',#276402,#129507,#129508);
#104285=AXIS2_PLACEMENT_3D('',#276419,#129510,#129511);
#104286=AXIS2_PLACEMENT_3D('',#276433,#129512,#129513);
#104287=AXIS2_PLACEMENT_3D('',#276434,#129514,#129515);
#104288=AXIS2_PLACEMENT_3D('',#276435,#129516,#129517);
#104289=AXIS2_PLACEMENT_3D('',#276436,#129518,#129519);
#104290=AXIS2_PLACEMENT_3D('',#276437,#129520,#129521);
#104291=AXIS2_PLACEMENT_3D('',#276438,#129522,#129523);
#104292=AXIS2_PLACEMENT_3D('',#276439,#129524,#129525);
#104293=AXIS2_PLACEMENT_3D('',#276440,#129526,#129527);
#104294=AXIS2_PLACEMENT_3D('',#276441,#129528,#129529);
#104295=AXIS2_PLACEMENT_3D('',#276442,#129530,#129531);
#104296=AXIS2_PLACEMENT_3D('',#276443,#129532,#129533);
#104297=AXIS2_PLACEMENT_3D('',#276444,#129534,#129535);
#104298=AXIS2_PLACEMENT_3D('',#276445,#129536,#129537);
#104299=AXIS2_PLACEMENT_3D('',#276446,#129538,#129539);
#104300=AXIS2_PLACEMENT_3D('',#276447,#129540,#129541);
#104301=AXIS2_PLACEMENT_3D('',#276448,#129542,#129543);
#104302=AXIS2_PLACEMENT_3D('',#276449,#129544,#129545);
#104303=AXIS2_PLACEMENT_3D('',#276450,#129546,#129547);
#104304=AXIS2_PLACEMENT_3D('',#276451,#129548,#129549);
#104305=AXIS2_PLACEMENT_3D('',#280642,#129550,#129551);
#104306=AXIS2_PLACEMENT_3D('',#280643,#129552,#129553);
#104307=AXIS2_PLACEMENT_3D('',#280658,#129555,#129556);
#104308=AXIS2_PLACEMENT_3D('',#280672,#129557,#129558);
#104309=AXIS2_PLACEMENT_3D('',#280718,#129560,#129561);
#104310=AXIS2_PLACEMENT_3D('',#280764,#129563,#129564);
#104311=AXIS2_PLACEMENT_3D('',#280810,#129566,#129567);
#104312=AXIS2_PLACEMENT_3D('',#280856,#129569,#129570);
#104313=AXIS2_PLACEMENT_3D('',#280861,#129572,#129573);
#104314=AXIS2_PLACEMENT_3D('',#280867,#129574,#129575);
#104315=AXIS2_PLACEMENT_3D('',#280872,#129577,#129578);
#104316=AXIS2_PLACEMENT_3D('',#280881,#129579,#129580);
#104317=AXIS2_PLACEMENT_3D('',#280957,#129582,#129583);
#104318=AXIS2_PLACEMENT_3D('',#281033,#129585,#129586);
#104319=AXIS2_PLACEMENT_3D('',#281109,#129588,#129589);
#104320=AXIS2_PLACEMENT_3D('',#281185,#129591,#129592);
#104321=AXIS2_PLACEMENT_3D('',#281263,#129594,#129595);
#104322=AXIS2_PLACEMENT_3D('',#281273,#129597,#129598);
#104323=AXIS2_PLACEMENT_3D('',#281282,#129599,#129600);
#104324=AXIS2_PLACEMENT_3D('',#281357,#129601,#129602);
#104325=AXIS2_PLACEMENT_3D('',#281359,#129603,#129604);
#104326=AXIS2_PLACEMENT_3D('',#281360,#129605,#129606);
#104327=AXIS2_PLACEMENT_3D('',#281362,#129607,#129608);
#104328=AXIS2_PLACEMENT_3D('',#281365,#129609,#129610);
#104329=AXIS2_PLACEMENT_3D('',#281367,#129611,#129612);
#104330=AXIS2_PLACEMENT_3D('',#281369,#129613,#129614);
#104331=AXIS2_PLACEMENT_3D('',#281371,#129615,#129616);
#104332=AXIS2_PLACEMENT_3D('',#281373,#129617,#129618);
#104333=AXIS2_PLACEMENT_3D('',#281374,#129619,#129620);
#104334=AXIS2_PLACEMENT_3D('',#281375,#129621,#129622);
#104335=AXIS2_PLACEMENT_3D('',#281395,#129624,#129625);
#104336=AXIS2_PLACEMENT_3D('',#281407,#129626,#129627);
#104337=AXIS2_PLACEMENT_3D('',#281423,#129629,#129630);
#104338=AXIS2_PLACEMENT_3D('',#281468,#129631,#129632);
#104339=AXIS2_PLACEMENT_3D('',#281469,#129633,#129634);
#104340=AXIS2_PLACEMENT_3D('',#281472,#129637,#129638);
#104341=AXIS2_PLACEMENT_3D('',#281474,#129640,#129641);
#104342=AXIS2_PLACEMENT_3D('',#281476,#129643,#129644);
#104343=AXIS2_PLACEMENT_3D('',#281478,#129646,#129647);
#104344=AXIS2_PLACEMENT_3D('',#281480,#129649,#129650);
#104345=AXIS2_PLACEMENT_3D('',#281481,#129651,#129652);
#104346=AXIS2_PLACEMENT_3D('',#281482,#129653,#129654);
#104347=AXIS2_PLACEMENT_3D('',#285705,#129655,#129656);
#104348=AXIS2_PLACEMENT_3D('',#285706,#129657,#129658);
#104349=AXIS2_PLACEMENT_3D('',#285725,#129660,#129661);
#104350=AXIS2_PLACEMENT_3D('',#285737,#129662,#129663);
#104351=AXIS2_PLACEMENT_3D('',#285766,#129665,#129666);
#104352=AXIS2_PLACEMENT_3D('',#285800,#129667,#129668);
#104353=AXIS2_PLACEMENT_3D('',#285801,#129669,#129670);
#104354=AXIS2_PLACEMENT_3D('',#285804,#129671,#129672);
#104355=AXIS2_PLACEMENT_3D('',#290036,#129673,#129674);
#104356=AXIS2_PLACEMENT_3D('',#290037,#129675,#129676);
#104357=AXIS2_PLACEMENT_3D('',#290038,#129677,#129678);
#104358=AXIS2_PLACEMENT_3D('',#290039,#129679,#129680);
#104359=AXIS2_PLACEMENT_3D('',#290049,#129682,#129683);
#104360=AXIS2_PLACEMENT_3D('',#290050,#129684,#129685);
#104361=AXIS2_PLACEMENT_3D('',#290096,#129687,#129688);
#104362=AXIS2_PLACEMENT_3D('',#290142,#129690,#129691);
#104363=AXIS2_PLACEMENT_3D('',#290188,#129693,#129694);
#104364=AXIS2_PLACEMENT_3D('',#290234,#129696,#129697);
#104365=AXIS2_PLACEMENT_3D('',#290280,#129699,#129700);
#104366=AXIS2_PLACEMENT_3D('',#290326,#129702,#129703);
#104367=AXIS2_PLACEMENT_3D('',#290372,#129705,#129706);
#104368=AXIS2_PLACEMENT_3D('',#290418,#129708,#129709);
#104369=AXIS2_PLACEMENT_3D('',#290464,#129711,#129712);
#104370=AXIS2_PLACEMENT_3D('',#290510,#129714,#129715);
#104371=AXIS2_PLACEMENT_3D('',#290556,#129717,#129718);
#104372=AXIS2_PLACEMENT_3D('',#290602,#129720,#129721);
#104373=AXIS2_PLACEMENT_3D('',#290648,#129723,#129724);
#104374=AXIS2_PLACEMENT_3D('',#290694,#129726,#129727);
#104375=AXIS2_PLACEMENT_3D('',#290740,#129729,#129730);
#104376=AXIS2_PLACEMENT_3D('',#290786,#129732,#129733);
#104377=AXIS2_PLACEMENT_3D('',#290832,#129735,#129736);
#104378=AXIS2_PLACEMENT_3D('',#290878,#129738,#129739);
#104379=AXIS2_PLACEMENT_3D('',#290924,#129741,#129742);
#104380=AXIS2_PLACEMENT_3D('',#290943,#129744,#129745);
#104381=AXIS2_PLACEMENT_3D('',#290955,#129746,#129747);
#104382=AXIS2_PLACEMENT_3D('',#291001,#129749,#129750);
#104383=AXIS2_PLACEMENT_3D('',#291047,#129752,#129753);
#104384=AXIS2_PLACEMENT_3D('',#291093,#129755,#129756);
#104385=AXIS2_PLACEMENT_3D('',#291139,#129758,#129759);
#104386=AXIS2_PLACEMENT_3D('',#291185,#129761,#129762);
#104387=AXIS2_PLACEMENT_3D('',#291231,#129764,#129765);
#104388=AXIS2_PLACEMENT_3D('',#291277,#129767,#129768);
#104389=AXIS2_PLACEMENT_3D('',#291323,#129770,#129771);
#104390=AXIS2_PLACEMENT_3D('',#291369,#129773,#129774);
#104391=AXIS2_PLACEMENT_3D('',#291415,#129776,#129777);
#104392=AXIS2_PLACEMENT_3D('',#291461,#129779,#129780);
#104393=AXIS2_PLACEMENT_3D('',#291507,#129782,#129783);
#104394=AXIS2_PLACEMENT_3D('',#291521,#129785,#129786);
#104395=AXIS2_PLACEMENT_3D('',#291526,#129787,#129788);
#104396=AXIS2_PLACEMENT_3D('',#291604,#129790,#129791);
#104397=AXIS2_PLACEMENT_3D('',#291682,#129793,#129794);
#104398=AXIS2_PLACEMENT_3D('',#291758,#129796,#129797);
#104399=AXIS2_PLACEMENT_3D('',#291834,#129799,#129800);
#104400=AXIS2_PLACEMENT_3D('',#291910,#129802,#129803);
#104401=AXIS2_PLACEMENT_3D('',#291986,#129805,#129806);
#104402=AXIS2_PLACEMENT_3D('',#292064,#129808,#129809);
#104403=AXIS2_PLACEMENT_3D('',#292140,#129811,#129812);
#104404=AXIS2_PLACEMENT_3D('',#292216,#129814,#129815);
#104405=AXIS2_PLACEMENT_3D('',#292294,#129817,#129818);
#104406=AXIS2_PLACEMENT_3D('',#292370,#129820,#129821);
#104407=AXIS2_PLACEMENT_3D('',#292446,#129823,#129824);
#104408=AXIS2_PLACEMENT_3D('',#292474,#129826,#129827);
#104409=AXIS2_PLACEMENT_3D('',#292493,#129828,#129829);
#104410=AXIS2_PLACEMENT_3D('',#292571,#129831,#129832);
#104411=AXIS2_PLACEMENT_3D('',#292649,#129834,#129835);
#104412=AXIS2_PLACEMENT_3D('',#292725,#129837,#129838);
#104413=AXIS2_PLACEMENT_3D('',#292801,#129840,#129841);
#104414=AXIS2_PLACEMENT_3D('',#292877,#129843,#129844);
#104415=AXIS2_PLACEMENT_3D('',#292953,#129846,#129847);
#104416=AXIS2_PLACEMENT_3D('',#293029,#129849,#129850);
#104417=AXIS2_PLACEMENT_3D('',#293105,#129852,#129853);
#104418=AXIS2_PLACEMENT_3D('',#293183,#129855,#129856);
#104419=AXIS2_PLACEMENT_3D('',#293261,#129858,#129859);
#104420=AXIS2_PLACEMENT_3D('',#293337,#129861,#129862);
#104421=AXIS2_PLACEMENT_3D('',#293413,#129864,#129865);
#104422=AXIS2_PLACEMENT_3D('',#293489,#129867,#129868);
#104423=AXIS2_PLACEMENT_3D('',#293565,#129870,#129871);
#104424=AXIS2_PLACEMENT_3D('',#293641,#129873,#129874);
#104425=AXIS2_PLACEMENT_3D('',#293717,#129876,#129877);
#104426=AXIS2_PLACEMENT_3D('',#293793,#129879,#129880);
#104427=AXIS2_PLACEMENT_3D('',#293871,#129882,#129883);
#104428=AXIS2_PLACEMENT_3D('',#293881,#129884,#129885);
#104429=AXIS2_PLACEMENT_3D('',#293882,#129886,#129887);
#104430=AXIS2_PLACEMENT_3D('',#293904,#129889,#129890);
#104431=AXIS2_PLACEMENT_3D('',#293933,#129891,#129892);
#104432=AXIS2_PLACEMENT_3D('',#293946,#129893,#129894);
#104433=AXIS2_PLACEMENT_3D('',#293960,#129895,#129896);
#104434=AXIS2_PLACEMENT_3D('',#294011,#129898,#129899);
#104435=AXIS2_PLACEMENT_3D('',#294012,#129900,#129901);
#104436=AXIS2_PLACEMENT_3D('',#294037,#129902,#129903);
#104437=AXIS2_PLACEMENT_3D('',#298268,#129904,#129905);
#104438=AXIS2_PLACEMENT_3D('',#298269,#129906,#129907);
#104439=AXIS2_PLACEMENT_3D('',#298270,#129908,#129909);
#104440=AXIS2_PLACEMENT_3D('',#298279,#129914,#129915);
#104441=AXIS2_PLACEMENT_3D('',#298290,#129920,#129921);
#104442=AXIS2_PLACEMENT_3D('',#298292,#129922,#129923);
#104443=AXIS2_PLACEMENT_3D('',#298294,#129924,#129925);
#104444=AXIS2_PLACEMENT_3D('',#298296,#129926,#129927);
#104445=AXIS2_PLACEMENT_3D('',#298298,#129928,#129929);
#104446=AXIS2_PLACEMENT_3D('',#298299,#129930,#129931);
#104447=AXIS2_PLACEMENT_3D('',#298300,#129932,#129933);
#104448=AXIS2_PLACEMENT_3D('',#298303,#129936,#129937);
#104449=AXIS2_PLACEMENT_3D('',#298305,#129939,#129940);
#104450=AXIS2_PLACEMENT_3D('',#298307,#129942,#129943);
#104451=AXIS2_PLACEMENT_3D('',#298308,#129944,#129945);
#104452=AXIS2_PLACEMENT_3D('',#298328,#129948,#129949);
#104453=AXIS2_PLACEMENT_3D('',#298345,#129951,#129952);
#104454=AXIS2_PLACEMENT_3D('',#298362,#129954,#129955);
#104455=AXIS2_PLACEMENT_3D('',#298379,#129957,#129958);
#104456=AXIS2_PLACEMENT_3D('',#298396,#129960,#129961);
#104457=AXIS2_PLACEMENT_3D('',#298410,#129962,#129963);
#104458=AXIS2_PLACEMENT_3D('',#298411,#129964,#129965);
#104459=AXIS2_PLACEMENT_3D('',#298412,#129966,#129967);
#104460=AXIS2_PLACEMENT_3D('',#298413,#129968,#129969);
#104461=AXIS2_PLACEMENT_3D('',#298414,#129970,#129971);
#104462=AXIS2_PLACEMENT_3D('',#298415,#129972,#129973);
#104463=AXIS2_PLACEMENT_3D('',#298416,#129974,#129975);
#104464=AXIS2_PLACEMENT_3D('',#298417,#129976,#129977);
#104465=AXIS2_PLACEMENT_3D('',#298418,#129978,#129979);
#104466=AXIS2_PLACEMENT_3D('',#298419,#129980,#129981);
#104467=AXIS2_PLACEMENT_3D('',#298420,#129982,#129983);
#104468=AXIS2_PLACEMENT_3D('',#298421,#129984,#129985);
#104469=AXIS2_PLACEMENT_3D('',#298422,#129986,#129987);
#104470=AXIS2_PLACEMENT_3D('',#298423,#129988,#129989);
#104471=AXIS2_PLACEMENT_3D('',#298424,#129990,#129991);
#104472=AXIS2_PLACEMENT_3D('',#298425,#129992,#129993);
#104473=AXIS2_PLACEMENT_3D('',#298426,#129994,#129995);
#104474=AXIS2_PLACEMENT_3D('',#298427,#129996,#129997);
#104475=AXIS2_PLACEMENT_3D('',#298428,#129998,#129999);
#104476=AXIS2_PLACEMENT_3D('',#298429,#130000,#130001);
#104477=AXIS2_PLACEMENT_3D('',#302622,#130002,#130003);
#104478=AXIS2_PLACEMENT_3D('',#302623,#130004,#130005);
#104479=AXIS2_PLACEMENT_3D('',#302625,#130006,#130007);
#104480=AXIS2_PLACEMENT_3D('',#302628,#130009,#130010);
#104481=AXIS2_PLACEMENT_3D('',#302629,#130011,#130012);
#104482=AXIS2_PLACEMENT_3D('',#302631,#130013,#130014);
#104483=AXIS2_PLACEMENT_3D('',#302634,#130016,#130017);
#104484=AXIS2_PLACEMENT_3D('',#302635,#130018,#130019);
#104485=AXIS2_PLACEMENT_3D('',#302637,#130020,#130021);
#104486=AXIS2_PLACEMENT_3D('',#302640,#130023,#130024);
#104487=AXIS2_PLACEMENT_3D('',#302641,#130025,#130026);
#104488=AXIS2_PLACEMENT_3D('',#302643,#130027,#130028);
#104489=AXIS2_PLACEMENT_3D('',#302646,#130030,#130031);
#104490=AXIS2_PLACEMENT_3D('',#302647,#130032,#130033);
#104491=AXIS2_PLACEMENT_3D('',#302649,#130034,#130035);
#104492=AXIS2_PLACEMENT_3D('',#302652,#130037,#130038);
#104493=AXIS2_PLACEMENT_3D('',#302653,#130039,#130040);
#104494=AXIS2_PLACEMENT_3D('',#302655,#130041,#130042);
#104495=AXIS2_PLACEMENT_3D('',#302658,#130044,#130045);
#104496=AXIS2_PLACEMENT_3D('',#302659,#130046,#130047);
#104497=AXIS2_PLACEMENT_3D('',#302661,#130048,#130049);
#104498=AXIS2_PLACEMENT_3D('',#302664,#130051,#130052);
#104499=AXIS2_PLACEMENT_3D('',#302665,#130053,#130054);
#104500=AXIS2_PLACEMENT_3D('',#302667,#130055,#130056);
#104501=AXIS2_PLACEMENT_3D('',#302670,#130058,#130059);
#104502=AXIS2_PLACEMENT_3D('',#302671,#130060,#130061);
#104503=AXIS2_PLACEMENT_3D('',#302673,#130062,#130063);
#104504=AXIS2_PLACEMENT_3D('',#302676,#130065,#130066);
#104505=AXIS2_PLACEMENT_3D('',#302677,#130067,#130068);
#104506=AXIS2_PLACEMENT_3D('',#302679,#130069,#130070);
#104507=AXIS2_PLACEMENT_3D('',#302682,#130072,#130073);
#104508=AXIS2_PLACEMENT_3D('',#302683,#130074,#130075);
#104509=AXIS2_PLACEMENT_3D('',#302685,#130076,#130077);
#104510=AXIS2_PLACEMENT_3D('',#302688,#130079,#130080);
#104511=AXIS2_PLACEMENT_3D('',#302689,#130081,#130082);
#104512=AXIS2_PLACEMENT_3D('',#302691,#130083,#130084);
#104513=AXIS2_PLACEMENT_3D('',#302693,#130085,#130086);
#104514=AXIS2_PLACEMENT_3D('',#302694,#130087,#130088);
#104515=AXIS2_PLACEMENT_3D('',#302696,#130089,#130090);
#104516=AXIS2_PLACEMENT_3D('',#302698,#130091,#130092);
#104517=AXIS2_PLACEMENT_3D('',#302699,#130093,#130094);
#104518=AXIS2_PLACEMENT_3D('',#302700,#130095,#130096);
#104519=AXIS2_PLACEMENT_3D('',#302702,#130097,#130098);
#104520=AXIS2_PLACEMENT_3D('',#302704,#130099,#130100);
#104521=AXIS2_PLACEMENT_3D('',#302706,#130101,#130102);
#104522=AXIS2_PLACEMENT_3D('',#302707,#130103,#130104);
#104523=AXIS2_PLACEMENT_3D('',#302708,#130105,#130106);
#104524=AXIS2_PLACEMENT_3D('',#302710,#130108,#130109);
#104525=AXIS2_PLACEMENT_3D('',#302712,#130110,#130111);
#104526=AXIS2_PLACEMENT_3D('',#302714,#130112,#130113);
#104527=AXIS2_PLACEMENT_3D('',#302715,#130114,#130115);
#104528=AXIS2_PLACEMENT_3D('',#302716,#130116,#130117);
#104529=AXIS2_PLACEMENT_3D('',#302718,#130119,#130120);
#104530=AXIS2_PLACEMENT_3D('',#302719,#130121,#130122);
#104531=AXIS2_PLACEMENT_3D('',#302720,#130123,#130124);
#104532=AXIS2_PLACEMENT_3D('',#302721,#130125,#130126);
#104533=AXIS2_PLACEMENT_3D('',#302722,#130127,#130128);
#104534=AXIS2_PLACEMENT_3D('',#302723,#130129,#130130);
#104535=AXIS2_PLACEMENT_3D('',#302724,#130131,#130132);
#104536=AXIS2_PLACEMENT_3D('',#302725,#130133,#130134);
#104537=AXIS2_PLACEMENT_3D('',#302726,#130135,#130136);
#104538=AXIS2_PLACEMENT_3D('',#302727,#130137,#130138);
#104539=AXIS2_PLACEMENT_3D('',#302728,#130139,#130140);
#104540=AXIS2_PLACEMENT_3D('',#302729,#130141,#130142);
#104541=AXIS2_PLACEMENT_3D('',#302730,#130143,#130144);
#104542=AXIS2_PLACEMENT_3D('',#302731,#130145,#130146);
#129415=DIRECTION('axis',(0.,0.,1.));
#129416=DIRECTION('refdir',(1.,0.,0.));
#129417=DIRECTION('center_axis',(-1.8547604288613E-34,-1.,8.30248970910064E-18));
#129418=DIRECTION('ref_axis',(-1.,0.,-2.23398100310589E-17));
#129419=DIRECTION('',(1.8547604288613E-34,1.,-8.30248970910064E-18));
#129420=DIRECTION('center_axis',(-1.8547604288613E-34,-1.,8.30248970910064E-18));
#129421=DIRECTION('ref_axis',(-1.,0.,-2.23398100310589E-17));
#129422=DIRECTION('center_axis',(-1.8547604288613E-34,-1.,8.30248970910064E-18));
#129423=DIRECTION('ref_axis',(-1.,0.,-2.23398100310589E-17));
#129424=DIRECTION('',(1.8547604288613E-34,1.,-8.30248970910064E-18));
#129425=DIRECTION('center_axis',(-1.8547604288613E-34,-1.,8.30248970910064E-18));
#129426=DIRECTION('ref_axis',(-1.,0.,-2.23398100310589E-17));
#129427=DIRECTION('center_axis',(-1.8547604288613E-34,-1.,8.30248970910064E-18));
#129428=DIRECTION('ref_axis',(-1.,0.,-2.23398100310589E-17));
#129429=DIRECTION('',(1.8547604288613E-34,1.,-8.30248970910064E-18));
#129430=DIRECTION('center_axis',(-1.8547604288613E-34,-1.,8.30248970910064E-18));
#129431=DIRECTION('ref_axis',(-1.,0.,-2.23398100310589E-17));
#129432=DIRECTION('',(1.8547604288613E-34,1.,-8.30248970910064E-18));
#129433=DIRECTION('center_axis',(-1.8547604288613E-34,-1.,8.30248970910064E-18));
#129434=DIRECTION('ref_axis',(-1.,0.,-2.23398100310589E-17));
#129435=DIRECTION('',(1.8547604288613E-34,1.,-8.30248970910064E-18));
#129436=DIRECTION('center_axis',(1.85999217976422E-14,1.,-1.41266321642785E-14));
#129437=DIRECTION('ref_axis',(-0.505304800152355,2.12071862805656E-14,0.862940935952739));
#129438=DIRECTION('center_axis',(-5.75903090556243E-16,1.,0.));
#129439=DIRECTION('ref_axis',(-1.,-5.75903090556243E-16,0.));
#129440=DIRECTION('',(0.707106781186546,0.707106781186549,-8.65956056235492E-17));
#129441=DIRECTION('center_axis',(5.75903090556247E-16,-1.,0.));
#129442=DIRECTION('ref_axis',(1.,5.75903090556247E-16,0.));
#129443=DIRECTION('',(-0.707106781186543,-0.707106781186552,-8.65956056235488E-17));
#129444=DIRECTION('center_axis',(5.7590309055625E-16,-1.,0.));
#129445=DIRECTION('ref_axis',(1.,5.7590309055625E-16,0.));
#129446=DIRECTION('',(5.7590309055625E-16,-1.,0.));
#129447=DIRECTION('center_axis',(-5.75903090556247E-16,1.,0.));
#129448=DIRECTION('ref_axis',(1.,5.75903090556247E-16,1.77635683940025E-15));
#129449=DIRECTION('center_axis',(5.7590309055625E-16,-1.,0.));
#129450=DIRECTION('ref_axis',(1.,5.7590309055625E-16,0.));
#129451=DIRECTION('',(5.7590309055625E-16,-1.,0.));
#129452=DIRECTION('center_axis',(-5.75903090556247E-16,1.,0.));
#129453=DIRECTION('ref_axis',(1.,5.75903090556247E-16,1.77635683940025E-15));
#129454=DIRECTION('center_axis',(5.7590309055625E-16,-1.,0.));
#129455=DIRECTION('ref_axis',(1.,5.7590309055625E-16,0.));
#129456=DIRECTION('',(5.7590309055625E-16,-1.,0.));
#129457=DIRECTION('center_axis',(5.7590309055625E-16,-1.,0.));
#129458=DIRECTION('ref_axis',(1.,5.7590309055625E-16,0.));
#129459=DIRECTION('',(5.7590309055625E-16,-1.,0.));
#129460=DIRECTION('center_axis',(5.7590309055625E-16,-1.,0.));
#129461=DIRECTION('ref_axis',(1.,5.7590309055625E-16,0.));
#129462=DIRECTION('',(5.7590309055625E-16,-1.,0.));
#129463=DIRECTION('center_axis',(5.7590309055625E-16,-1.,0.));
#129464=DIRECTION('ref_axis',(1.,5.7590309055625E-16,0.));
#129465=DIRECTION('',(5.7590309055625E-16,-1.,0.));
#129466=DIRECTION('center_axis',(5.75903090556243E-16,-1.,0.));
#129467=DIRECTION('ref_axis',(-1.,-5.75903090556243E-16,0.));
#129468=DIRECTION('center_axis',(5.7590309055625E-16,-1.,0.));
#129469=DIRECTION('ref_axis',(1.,5.7590309055625E-16,0.));
#129470=DIRECTION('center_axis',(5.75903090556247E-16,-1.,0.));
#129471=DIRECTION('ref_axis',(1.,5.75903090556247E-16,0.));
#129472=DIRECTION('',(-0.707106781186543,-0.707106781186552,-8.65956056235488E-17));
#129473=DIRECTION('center_axis',(0.,1.,0.));
#129474=DIRECTION('ref_axis',(0.,0.,1.));
#129475=DIRECTION('center_axis',(-5.75903090556243E-16,1.,0.));
#129476=DIRECTION('ref_axis',(-1.,-5.75903090556243E-16,0.));
#129477=DIRECTION('',(0.707106781186546,0.707106781186549,-8.65956056235492E-17));
#129478=DIRECTION('center_axis',(0.,-1.,0.));
#129479=DIRECTION('ref_axis',(0.,0.,1.));
#129480=DIRECTION('center_axis',(0.,1.,0.));
#129481=DIRECTION('ref_axis',(0.,0.,1.));
#129482=DIRECTION('center_axis',(0.,1.,0.));
#129483=DIRECTION('ref_axis',(0.,0.,1.));
#129484=DIRECTION('center_axis',(0.,-1.,0.));
#129485=DIRECTION('ref_axis',(0.,0.,1.));
#129486=DIRECTION('center_axis',(0.,-1.,0.));
#129487=DIRECTION('ref_axis',(0.,0.,1.));
#129488=DIRECTION('center_axis',(0.,-1.,0.));
#129489=DIRECTION('ref_axis',(1.77635683940025E-15,0.,1.));
#129490=DIRECTION('center_axis',(0.,-1.,0.));
#129491=DIRECTION('ref_axis',(0.,0.,1.));
#129492=DIRECTION('center_axis',(0.,-1.,0.));
#129493=DIRECTION('ref_axis',(-8.88178419700125E-16,0.,1.));
#129494=DIRECTION('center_axis',(-0.866025403784439,-4.98746706539683E-16,
0.5));
#129495=DIRECTION('ref_axis',(0.5,1.55703595698071E-32,0.866025403784439));
#129496=DIRECTION('',(-5.7590309055625E-16,1.,0.));
#129497=DIRECTION('',(-5.7590309055625E-16,1.,0.));
#129498=DIRECTION('center_axis',(-0.866025403784439,-4.98746706539683E-16,
-0.5));
#129499=DIRECTION('ref_axis',(-0.5,-4.12937143755386E-33,0.866025403784439));
#129500=DIRECTION('',(-5.7590309055625E-16,1.,0.));
#129501=DIRECTION('center_axis',(0.,0.,-1.));
#129502=DIRECTION('ref_axis',(-1.,0.,0.));
#129503=DIRECTION('',(-5.7590309055625E-16,1.,0.));
#129504=DIRECTION('center_axis',(0.866025403784439,4.98746706539683E-16,
-0.5));
#129505=DIRECTION('ref_axis',(-0.5,-4.50262904462734E-32,-0.866025403784439));
#129506=DIRECTION('',(-5.7590309055625E-16,1.,0.));
#129507=DIRECTION('center_axis',(0.866025403784439,4.98746706539683E-16,
0.5));
#129508=DIRECTION('ref_axis',(0.5,1.3768929580165E-32,-0.866025403784439));
#129509=DIRECTION('',(-5.7590309055625E-16,1.,0.));
#129510=DIRECTION('center_axis',(0.,0.,1.));
#129511=DIRECTION('ref_axis',(1.,0.,0.));
#129512=DIRECTION('center_axis',(0.,1.,0.));
#129513=DIRECTION('ref_axis',(0.,0.,1.));
#129514=DIRECTION('center_axis',(0.,1.,0.));
#129515=DIRECTION('ref_axis',(0.,0.,1.));
#129516=DIRECTION('center_axis',(0.,1.,0.));
#129517=DIRECTION('ref_axis',(0.,0.,1.));
#129518=DIRECTION('center_axis',(0.,1.,0.));
#129519=DIRECTION('ref_axis',(0.,0.,1.));
#129520=DIRECTION('center_axis',(0.,1.,0.));
#129521=DIRECTION('ref_axis',(0.,0.,1.));
#129522=DIRECTION('center_axis',(0.,1.,0.));
#129523=DIRECTION('ref_axis',(0.,0.,1.));
#129524=DIRECTION('center_axis',(0.,1.,0.));
#129525=DIRECTION('ref_axis',(0.,0.,1.));
#129526=DIRECTION('center_axis',(0.,-1.,0.));
#129527=DIRECTION('ref_axis',(0.,0.,1.));
#129528=DIRECTION('center_axis',(0.,-1.,0.));
#129529=DIRECTION('ref_axis',(0.,0.,1.));
#129530=DIRECTION('center_axis',(0.,-1.,0.));
#129531=DIRECTION('ref_axis',(0.,0.,1.));
#129532=DIRECTION('center_axis',(0.,-1.,0.));
#129533=DIRECTION('ref_axis',(0.,0.,1.));
#129534=DIRECTION('center_axis',(0.,-1.,0.));
#129535=DIRECTION('ref_axis',(0.,0.,1.));
#129536=DIRECTION('center_axis',(0.,-1.,0.));
#129537=DIRECTION('ref_axis',(0.,0.,1.));
#129538=DIRECTION('center_axis',(0.,1.,0.));
#129539=DIRECTION('ref_axis',(0.,0.,1.));
#129540=DIRECTION('center_axis',(0.,1.,0.));
#129541=DIRECTION('ref_axis',(0.,0.,1.));
#129542=DIRECTION('center_axis',(0.,1.,0.));
#129543=DIRECTION('ref_axis',(0.,0.,1.));
#129544=DIRECTION('center_axis',(0.,1.,0.));
#129545=DIRECTION('ref_axis',(0.,0.,1.));
#129546=DIRECTION('center_axis',(0.,1.,0.));
#129547=DIRECTION('ref_axis',(0.,0.,1.));
#129548=DIRECTION('center_axis',(0.,1.,0.));
#129549=DIRECTION('ref_axis',(0.,0.,1.));
#129550=DIRECTION('center_axis',(-1.8547604288613E-34,-1.,8.30248970910064E-18));
#129551=DIRECTION('ref_axis',(-1.,0.,-2.23398100310589E-17));
#129552=DIRECTION('center_axis',(-1.8547604288613E-34,-1.,8.30248970910064E-18));
#129553=DIRECTION('ref_axis',(-1.,0.,-2.23398100310589E-17));
#129554=DIRECTION('',(1.8547604288613E-34,1.,-8.30248970910064E-18));
#129555=DIRECTION('center_axis',(-2.90604864291398E-15,-1.,-4.10722704360696E-16));
#129556=DIRECTION('ref_axis',(-0.743877835774618,2.42999009464821E-15,-0.668315618135077));
#129557=DIRECTION('center_axis',(-1.8547604288613E-34,-1.,8.30248970910064E-18));
#129558=DIRECTION('ref_axis',(-1.,0.,-2.23398100310589E-17));
#129559=DIRECTION('',(1.8547604288613E-34,1.,-8.30248970910064E-18));
#129560=DIRECTION('center_axis',(-1.8547604288613E-34,-1.,8.30248970910064E-18));
#129561=DIRECTION('ref_axis',(-1.,0.,-2.23398100310589E-17));
#129562=DIRECTION('',(1.8547604288613E-34,1.,-8.30248970910064E-18));
#129563=DIRECTION('center_axis',(-1.8547604288613E-34,-1.,8.30248970910064E-18));
#129564=DIRECTION('ref_axis',(-1.,0.,-2.23398100310589E-17));
#129565=DIRECTION('',(1.8547604288613E-34,1.,-8.30248970910064E-18));
#129566=DIRECTION('center_axis',(-1.8547604288613E-34,-1.,8.30248970910064E-18));
#129567=DIRECTION('ref_axis',(-1.,0.,-2.23398100310589E-17));
#129568=DIRECTION('',(1.8547604288613E-34,1.,-8.30248970910064E-18));
#129569=DIRECTION('center_axis',(-1.8547604288613E-34,-1.,8.30248970910064E-18));
#129570=DIRECTION('ref_axis',(-1.,0.,-2.23398100310589E-17));
#129571=DIRECTION('',(1.8547604288613E-34,1.,-8.30248970910064E-18));
#129572=DIRECTION('center_axis',(-5.7590309055625E-16,1.,0.));
#129573=DIRECTION('ref_axis',(-1.,0.,-2.23398100310589E-17));
#129574=DIRECTION('center_axis',(5.7590309055625E-16,-1.,0.));
#129575=DIRECTION('ref_axis',(1.,5.7590309055625E-16,0.));
#129576=DIRECTION('',(5.7590309055625E-16,-1.,0.));
#129577=DIRECTION('center_axis',(-5.7590309055625E-16,1.,0.));
#129578=DIRECTION('ref_axis',(-1.,-5.7590309055625E-16,0.));
#129579=DIRECTION('center_axis',(5.7590309055625E-16,-1.,0.));
#129580=DIRECTION('ref_axis',(1.,5.7590309055625E-16,0.));
#129581=DIRECTION('',(5.7590309055625E-16,-1.,0.));
#129582=DIRECTION('center_axis',(5.7590309055625E-16,-1.,0.));
#129583=DIRECTION('ref_axis',(1.,5.7590309055625E-16,0.));
#129584=DIRECTION('',(5.7590309055625E-16,-1.,0.));
#129585=DIRECTION('center_axis',(5.7590309055625E-16,-1.,0.));
#129586=DIRECTION('ref_axis',(1.,5.7590309055625E-16,0.));
#129587=DIRECTION('',(5.7590309055625E-16,-1.,0.));
#129588=DIRECTION('center_axis',(5.7590309055625E-16,-1.,0.));
#129589=DIRECTION('ref_axis',(1.,5.7590309055625E-16,0.));
#129590=DIRECTION('',(5.7590309055625E-16,-1.,0.));
#129591=DIRECTION('center_axis',(5.7590309055625E-16,-1.,0.));
#129592=DIRECTION('ref_axis',(1.,5.7590309055625E-16,0.));
#129593=DIRECTION('',(5.7590309055625E-16,-1.,0.));
#129594=DIRECTION('center_axis',(5.7590309055625E-16,-1.,0.));
#129595=DIRECTION('ref_axis',(1.,5.7590309055625E-16,0.));
#129596=DIRECTION('',(5.7590309055625E-16,-1.,0.));
#129597=DIRECTION('center_axis',(0.,-1.,0.));
#129598=DIRECTION('ref_axis',(0.,0.,1.));
#129599=DIRECTION('center_axis',(5.7590309055625E-16,-1.,0.));
#129600=DIRECTION('ref_axis',(1.,5.7590309055625E-16,0.));
#129601=DIRECTION('center_axis',(-6.12323399573677E-17,0.,1.));
#129602=DIRECTION('ref_axis',(-1.,0.,0.));
#129603=DIRECTION('center_axis',(4.12652725799652E-17,1.,0.));
#129604=DIRECTION('ref_axis',(-1.,4.12652725799652E-17,0.));
#129605=DIRECTION('center_axis',(-6.12323399573677E-17,0.,1.));
#129606=DIRECTION('ref_axis',(-1.,0.,0.));
#129607=DIRECTION('center_axis',(4.12652725799652E-17,1.,0.));
#129608=DIRECTION('ref_axis',(-1.,4.12652725799652E-17,0.));
#129609=DIRECTION('center_axis',(0.866025403784439,0.,0.5));
#129610=DIRECTION('ref_axis',(0.5,0.,-0.866025403784439));
#129611=DIRECTION('center_axis',(-4.32612527870318E-16,0.,1.));
#129612=DIRECTION('ref_axis',(1.,0.,4.32612527870318E-16));
#129613=DIRECTION('center_axis',(-0.866025403784439,0.,0.5));
#129614=DIRECTION('ref_axis',(0.5,0.,0.866025403784439));
#129615=DIRECTION('center_axis',(-0.866025403784439,0.,-0.5));
#129616=DIRECTION('ref_axis',(-0.5,0.,0.866025403784439));
#129617=DIRECTION('center_axis',(0.,0.,-1.));
#129618=DIRECTION('ref_axis',(-1.,0.,0.));
#129619=DIRECTION('center_axis',(0.866025403784438,0.,-0.500000000000001));
#129620=DIRECTION('ref_axis',(-0.500000000000001,0.,-0.866025403784438));
#129621=DIRECTION('center_axis',(0.,-1.,0.));
#129622=DIRECTION('ref_axis',(0.,0.,1.));
#129623=DIRECTION('',(-7.02428546843655E-17,0.819152044288991,0.573576436351047));
#129624=DIRECTION('center_axis',(0.,1.,0.));
#129625=DIRECTION('ref_axis',(0.,0.,1.));
#129626=DIRECTION('center_axis',(0.,1.,0.));
#129627=DIRECTION('ref_axis',(0.,0.,1.));
#129628=DIRECTION('',(-8.659560562355E-17,0.707106781186542,-0.707106781186553));
#129629=DIRECTION('center_axis',(0.,-1.,0.));
#129630=DIRECTION('ref_axis',(0.,0.,1.));
#129631=DIRECTION('center_axis',(0.,1.,0.));
#129632=DIRECTION('ref_axis',(0.,0.,1.));
#129633=DIRECTION('center_axis',(0.866025403784439,0.,0.5));
#129634=DIRECTION('ref_axis',(0.5,0.,-0.866025403784439));
#129635=DIRECTION('',(0.,-1.,0.));
#129636=DIRECTION('',(0.,-1.,0.));
#129637=DIRECTION('center_axis',(0.866025403784438,0.,-0.500000000000001));
#129638=DIRECTION('ref_axis',(-0.500000000000001,0.,-0.866025403784438));
#129639=DIRECTION('',(0.,-1.,0.));
#129640=DIRECTION('center_axis',(0.,0.,-1.));
#129641=DIRECTION('ref_axis',(-1.,0.,0.));
#129642=DIRECTION('',(0.,-1.,0.));
#129643=DIRECTION('center_axis',(-0.866025403784439,0.,-0.5));
#129644=DIRECTION('ref_axis',(-0.5,0.,0.866025403784439));
#129645=DIRECTION('',(0.,-1.,0.));
#129646=DIRECTION('center_axis',(-0.866025403784439,0.,0.5));
#129647=DIRECTION('ref_axis',(0.5,0.,0.866025403784439));
#129648=DIRECTION('',(0.,-1.,0.));
#129649=DIRECTION('center_axis',(-4.32612527870318E-16,0.,1.));
#129650=DIRECTION('ref_axis',(1.,0.,4.32612527870318E-16));
#129651=DIRECTION('center_axis',(4.12652725799652E-17,1.,0.));
#129652=DIRECTION('ref_axis',(-1.,4.12652725799652E-17,0.));
#129653=DIRECTION('center_axis',(-5.7590309055625E-16,1.,0.));
#129654=DIRECTION('ref_axis',(-1.,-5.7590309055625E-16,0.));
#129655=DIRECTION('center_axis',(-1.8547604288613E-34,-1.,8.30248970910064E-18));
#129656=DIRECTION('ref_axis',(-1.,0.,-2.23398100310589E-17));
#129657=DIRECTION('center_axis',(-1.8547604288613E-34,-1.,8.30248970910064E-18));
#129658=DIRECTION('ref_axis',(-1.,0.,-2.23398100310589E-17));
#129659=DIRECTION('',(-1.8547604288613E-34,-1.,8.30248970910064E-18));
#129660=DIRECTION('center_axis',(-4.29158568362712E-14,-1.,1.24422947616665E-14));
#129661=DIRECTION('ref_axis',(-1.,4.32980053228238E-14,1.0804960395692E-14));
#129662=DIRECTION('center_axis',(-5.75903090556246E-16,1.,0.));
#129663=DIRECTION('ref_axis',(-1.,-5.75903090556246E-16,0.));
#129664=DIRECTION('',(0.707106781186546,0.707106781186549,-8.65956056235492E-17));
#129665=DIRECTION('center_axis',(0.,1.,0.));
#129666=DIRECTION('ref_axis',(0.,0.,-1.));
#129667=DIRECTION('center_axis',(5.75903090556246E-16,-1.,0.));
#129668=DIRECTION('ref_axis',(-1.,-5.75903090556246E-16,-8.88178419700125E-16));
#129669=DIRECTION('center_axis',(5.7590309055625E-16,-1.,0.));
#129670=DIRECTION('ref_axis',(1.,5.7590309055625E-16,0.));
#129671=DIRECTION('center_axis',(0.,-1.,0.));
#129672=DIRECTION('ref_axis',(0.,0.,-1.));
#129673=DIRECTION('center_axis',(-1.8547604288613E-34,-1.,8.30248970910064E-18));
#129674=DIRECTION('ref_axis',(-1.,0.,-2.23398100310589E-17));
#129675=DIRECTION('center_axis',(0.,-1.,0.));
#129676=DIRECTION('ref_axis',(-1.,0.,-2.23398100310589E-17));
#129677=DIRECTION('center_axis',(0.,-1.,0.));
#129678=DIRECTION('ref_axis',(0.,0.,-1.));
#129679=DIRECTION('center_axis',(-1.8547604288613E-34,-1.,8.30248970910064E-18));
#129680=DIRECTION('ref_axis',(-1.,0.,-2.23398100310589E-17));
#129681=DIRECTION('',(-1.8547604288613E-34,-1.,8.30248970910064E-18));
#129682=DIRECTION('center_axis',(-5.7590309055625E-16,1.,0.));
#129683=DIRECTION('ref_axis',(-1.,0.,-2.23398100310589E-17));
#129684=DIRECTION('center_axis',(-1.8547604288613E-34,-1.,8.30248970910064E-18));
#129685=DIRECTION('ref_axis',(-1.,0.,-2.23398100310589E-17));
#129686=DIRECTION('',(-1.8547604288613E-34,-1.,8.30248970910064E-18));
#129687=DIRECTION('center_axis',(-1.8547604288613E-34,-1.,8.30248970910064E-18));
#129688=DIRECTION('ref_axis',(-1.,0.,-2.23398100310589E-17));
#129689=DIRECTION('',(-1.8547604288613E-34,-1.,8.30248970910064E-18));
#129690=DIRECTION('center_axis',(-1.8547604288613E-34,-1.,8.30248970910064E-18));
#129691=DIRECTION('ref_axis',(-1.,0.,-2.23398100310589E-17));
#129692=DIRECTION('',(-1.8547604288613E-34,-1.,8.30248970910064E-18));
#129693=DIRECTION('center_axis',(-1.8547604288613E-34,-1.,8.30248970910064E-18));
#129694=DIRECTION('ref_axis',(-1.,0.,-2.23398100310589E-17));
#129695=DIRECTION('',(-1.8547604288613E-34,-1.,8.30248970910064E-18));
#129696=DIRECTION('center_axis',(-1.8547604288613E-34,-1.,8.30248970910064E-18));
#129697=DIRECTION('ref_axis',(-1.,0.,-2.23398100310589E-17));
#129698=DIRECTION('',(-1.8547604288613E-34,-1.,8.30248970910064E-18));
#129699=DIRECTION('center_axis',(-1.8547604288613E-34,-1.,8.30248970910064E-18));
#129700=DIRECTION('ref_axis',(-1.,0.,-2.23398100310589E-17));
#129701=DIRECTION('',(-1.8547604288613E-34,-1.,8.30248970910064E-18));
#129702=DIRECTION('center_axis',(-1.8547604288613E-34,-1.,8.30248970910064E-18));
#129703=DIRECTION('ref_axis',(-1.,0.,-2.23398100310589E-17));
#129704=DIRECTION('',(-1.8547604288613E-34,-1.,8.30248970910064E-18));
#129705=DIRECTION('center_axis',(-1.8547604288613E-34,-1.,8.30248970910064E-18));
#129706=DIRECTION('ref_axis',(-1.,0.,-2.23398100310589E-17));
#129707=DIRECTION('',(-1.8547604288613E-34,-1.,8.30248970910064E-18));
#129708=DIRECTION('center_axis',(-1.8547604288613E-34,-1.,8.30248970910064E-18));
#129709=DIRECTION('ref_axis',(-1.,0.,-2.23398100310589E-17));
#129710=DIRECTION('',(-1.8547604288613E-34,-1.,8.30248970910064E-18));
#129711=DIRECTION('center_axis',(-1.8547604288613E-34,-1.,8.30248970910064E-18));
#129712=DIRECTION('ref_axis',(-1.,0.,-2.23398100310589E-17));
#129713=DIRECTION('',(-1.8547604288613E-34,-1.,8.30248970910064E-18));
#129714=DIRECTION('center_axis',(-1.8547604288613E-34,-1.,8.30248970910064E-18));
#129715=DIRECTION('ref_axis',(-1.,0.,-2.23398100310589E-17));
#129716=DIRECTION('',(-1.8547604288613E-34,-1.,8.30248970910064E-18));
#129717=DIRECTION('center_axis',(-1.8547604288613E-34,-1.,8.30248970910064E-18));
#129718=DIRECTION('ref_axis',(-1.,0.,-2.23398100310589E-17));
#129719=DIRECTION('',(-1.8547604288613E-34,-1.,8.30248970910064E-18));
#129720=DIRECTION('center_axis',(-1.8547604288613E-34,-1.,8.30248970910064E-18));
#129721=DIRECTION('ref_axis',(-1.,0.,-2.23398100310589E-17));
#129722=DIRECTION('',(-1.8547604288613E-34,-1.,8.30248970910064E-18));
#129723=DIRECTION('center_axis',(-1.8547604288613E-34,-1.,8.30248970910064E-18));
#129724=DIRECTION('ref_axis',(-1.,0.,-2.23398100310589E-17));
#129725=DIRECTION('',(-1.8547604288613E-34,-1.,8.30248970910064E-18));
#129726=DIRECTION('center_axis',(-1.8547604288613E-34,-1.,8.30248970910064E-18));
#129727=DIRECTION('ref_axis',(-1.,0.,-2.23398100310589E-17));
#129728=DIRECTION('',(-1.8547604288613E-34,-1.,8.30248970910064E-18));
#129729=DIRECTION('center_axis',(-1.8547604288613E-34,-1.,8.30248970910064E-18));
#129730=DIRECTION('ref_axis',(-1.,0.,-2.23398100310589E-17));
#129731=DIRECTION('',(-1.8547604288613E-34,-1.,8.30248970910064E-18));
#129732=DIRECTION('center_axis',(-1.8547604288613E-34,-1.,8.30248970910064E-18));
#129733=DIRECTION('ref_axis',(-1.,0.,-2.23398100310589E-17));
#129734=DIRECTION('',(-1.8547604288613E-34,-1.,8.30248970910064E-18));
#129735=DIRECTION('center_axis',(-1.8547604288613E-34,-1.,8.30248970910064E-18));
#129736=DIRECTION('ref_axis',(-1.,0.,-2.23398100310589E-17));
#129737=DIRECTION('',(-1.8547604288613E-34,-1.,8.30248970910064E-18));
#129738=DIRECTION('center_axis',(-1.8547604288613E-34,-1.,8.30248970910064E-18));
#129739=DIRECTION('ref_axis',(-1.,0.,-2.23398100310589E-17));
#129740=DIRECTION('',(-1.8547604288613E-34,-1.,8.30248970910064E-18));
#129741=DIRECTION('center_axis',(-1.8547604288613E-34,-1.,8.30248970910064E-18));
#129742=DIRECTION('ref_axis',(-1.,0.,-2.23398100310589E-17));
#129743=DIRECTION('',(-1.8547604288613E-34,-1.,8.30248970910064E-18));
#129744=DIRECTION('center_axis',(0.,-1.,0.));
#129745=DIRECTION('ref_axis',(-1.,0.,-2.23398100310589E-17));
#129746=DIRECTION('center_axis',(-1.8547604288613E-34,-1.,8.30248970910064E-18));
#129747=DIRECTION('ref_axis',(-1.,0.,-2.23398100310589E-17));
#129748=DIRECTION('',(-1.8547604288613E-34,-1.,8.30248970910064E-18));
#129749=DIRECTION('center_axis',(-1.8547604288613E-34,-1.,8.30248970910064E-18));
#129750=DIRECTION('ref_axis',(-1.,0.,-2.23398100310589E-17));
#129751=DIRECTION('',(-1.8547604288613E-34,-1.,8.30248970910064E-18));
#129752=DIRECTION('center_axis',(-1.8547604288613E-34,-1.,8.30248970910064E-18));
#129753=DIRECTION('ref_axis',(-1.,0.,-2.23398100310589E-17));
#129754=DIRECTION('',(-1.8547604288613E-34,-1.,8.30248970910064E-18));
#129755=DIRECTION('center_axis',(-1.8547604288613E-34,-1.,8.30248970910064E-18));
#129756=DIRECTION('ref_axis',(-1.,0.,-2.23398100310589E-17));
#129757=DIRECTION('',(-1.8547604288613E-34,-1.,8.30248970910064E-18));
#129758=DIRECTION('center_axis',(-1.8547604288613E-34,-1.,8.30248970910064E-18));
#129759=DIRECTION('ref_axis',(-1.,0.,-2.23398100310589E-17));
#129760=DIRECTION('',(-1.8547604288613E-34,-1.,8.30248970910064E-18));
#129761=DIRECTION('center_axis',(-1.8547604288613E-34,-1.,8.30248970910064E-18));
#129762=DIRECTION('ref_axis',(-1.,0.,-2.23398100310589E-17));
#129763=DIRECTION('',(-1.8547604288613E-34,-1.,8.30248970910064E-18));
#129764=DIRECTION('center_axis',(-1.8547604288613E-34,-1.,8.30248970910064E-18));
#129765=DIRECTION('ref_axis',(-1.,0.,-2.23398100310589E-17));
#129766=DIRECTION('',(-1.8547604288613E-34,-1.,8.30248970910064E-18));
#129767=DIRECTION('center_axis',(-1.8547604288613E-34,-1.,8.30248970910064E-18));
#129768=DIRECTION('ref_axis',(-1.,0.,-2.23398100310589E-17));
#129769=DIRECTION('',(-1.8547604288613E-34,-1.,8.30248970910064E-18));
#129770=DIRECTION('center_axis',(-1.8547604288613E-34,-1.,8.30248970910064E-18));
#129771=DIRECTION('ref_axis',(-1.,0.,-2.23398100310589E-17));
#129772=DIRECTION('',(-1.8547604288613E-34,-1.,8.30248970910064E-18));
#129773=DIRECTION('center_axis',(-1.8547604288613E-34,-1.,8.30248970910064E-18));
#129774=DIRECTION('ref_axis',(-1.,0.,-2.23398100310589E-17));
#129775=DIRECTION('',(-1.8547604288613E-34,-1.,8.30248970910064E-18));
#129776=DIRECTION('center_axis',(-1.8547604288613E-34,-1.,8.30248970910064E-18));
#129777=DIRECTION('ref_axis',(-1.,0.,-2.23398100310589E-17));
#129778=DIRECTION('',(-1.8547604288613E-34,-1.,8.30248970910064E-18));
#129779=DIRECTION('center_axis',(-1.8547604288613E-34,-1.,8.30248970910064E-18));
#129780=DIRECTION('ref_axis',(-1.,0.,-2.23398100310589E-17));
#129781=DIRECTION('',(-1.8547604288613E-34,-1.,8.30248970910064E-18));
#129782=DIRECTION('center_axis',(5.7590309055625E-16,-1.,0.));
#129783=DIRECTION('ref_axis',(1.,5.7590309055625E-16,0.));
#129784=DIRECTION('',(-5.7590309055625E-16,1.,0.));
#129785=DIRECTION('center_axis',(5.7590309055625E-16,-1.,0.));
#129786=DIRECTION('ref_axis',(-1.,-5.7590309055625E-16,8.88178419700125E-16));
#129787=DIRECTION('center_axis',(5.7590309055625E-16,-1.,0.));
#129788=DIRECTION('ref_axis',(1.,5.7590309055625E-16,0.));
#129789=DIRECTION('',(-5.7590309055625E-16,1.,0.));
#129790=DIRECTION('center_axis',(5.7590309055625E-16,-1.,0.));
#129791=DIRECTION('ref_axis',(1.,5.7590309055625E-16,0.));
#129792=DIRECTION('',(-5.7590309055625E-16,1.,0.));
#129793=DIRECTION('center_axis',(5.7590309055625E-16,-1.,0.));
#129794=DIRECTION('ref_axis',(1.,5.7590309055625E-16,0.));
#129795=DIRECTION('',(-5.7590309055625E-16,1.,0.));
#129796=DIRECTION('center_axis',(5.7590309055625E-16,-1.,0.));
#129797=DIRECTION('ref_axis',(1.,5.7590309055625E-16,0.));
#129798=DIRECTION('',(-5.7590309055625E-16,1.,0.));
#129799=DIRECTION('center_axis',(5.7590309055625E-16,-1.,0.));
#129800=DIRECTION('ref_axis',(1.,5.7590309055625E-16,0.));
#129801=DIRECTION('',(-5.7590309055625E-16,1.,0.));
#129802=DIRECTION('center_axis',(5.7590309055625E-16,-1.,0.));
#129803=DIRECTION('ref_axis',(1.,5.7590309055625E-16,0.));
#129804=DIRECTION('',(-5.7590309055625E-16,1.,0.));
#129805=DIRECTION('center_axis',(5.7590309055625E-16,-1.,0.));
#129806=DIRECTION('ref_axis',(1.,5.7590309055625E-16,0.));
#129807=DIRECTION('',(-5.7590309055625E-16,1.,0.));
#129808=DIRECTION('center_axis',(5.7590309055625E-16,-1.,0.));
#129809=DIRECTION('ref_axis',(1.,5.7590309055625E-16,0.));
#129810=DIRECTION('',(-5.7590309055625E-16,1.,0.));
#129811=DIRECTION('center_axis',(5.7590309055625E-16,-1.,0.));
#129812=DIRECTION('ref_axis',(1.,5.7590309055625E-16,0.));
#129813=DIRECTION('',(-5.7590309055625E-16,1.,0.));
#129814=DIRECTION('center_axis',(5.7590309055625E-16,-1.,0.));
#129815=DIRECTION('ref_axis',(1.,5.7590309055625E-16,0.));
#129816=DIRECTION('',(-5.7590309055625E-16,1.,0.));
#129817=DIRECTION('center_axis',(5.7590309055625E-16,-1.,0.));
#129818=DIRECTION('ref_axis',(1.,5.7590309055625E-16,0.));
#129819=DIRECTION('',(-5.7590309055625E-16,1.,0.));
#129820=DIRECTION('center_axis',(5.7590309055625E-16,-1.,0.));
#129821=DIRECTION('ref_axis',(1.,5.7590309055625E-16,0.));
#129822=DIRECTION('',(-5.7590309055625E-16,1.,0.));
#129823=DIRECTION('center_axis',(5.7590309055625E-16,-1.,0.));
#129824=DIRECTION('ref_axis',(1.,5.7590309055625E-16,0.));
#129825=DIRECTION('',(-5.7590309055625E-16,1.,0.));
#129826=DIRECTION('center_axis',(-5.7590309055625E-16,1.,0.));
#129827=DIRECTION('ref_axis',(1.,5.7590309055625E-16,-3.5527136788005E-15));
#129828=DIRECTION('center_axis',(5.7590309055625E-16,-1.,0.));
#129829=DIRECTION('ref_axis',(1.,5.7590309055625E-16,0.));
#129830=DIRECTION('',(-5.7590309055625E-16,1.,0.));
#129831=DIRECTION('center_axis',(5.7590309055625E-16,-1.,0.));
#129832=DIRECTION('ref_axis',(1.,5.7590309055625E-16,0.));
#129833=DIRECTION('',(-5.7590309055625E-16,1.,0.));
#129834=DIRECTION('center_axis',(5.7590309055625E-16,-1.,0.));
#129835=DIRECTION('ref_axis',(1.,5.7590309055625E-16,0.));
#129836=DIRECTION('',(-5.7590309055625E-16,1.,0.));
#129837=DIRECTION('center_axis',(5.7590309055625E-16,-1.,0.));
#129838=DIRECTION('ref_axis',(1.,5.7590309055625E-16,0.));
#129839=DIRECTION('',(-5.7590309055625E-16,1.,0.));
#129840=DIRECTION('center_axis',(5.7590309055625E-16,-1.,0.));
#129841=DIRECTION('ref_axis',(1.,5.7590309055625E-16,0.));
#129842=DIRECTION('',(-5.7590309055625E-16,1.,0.));
#129843=DIRECTION('center_axis',(5.7590309055625E-16,-1.,0.));
#129844=DIRECTION('ref_axis',(1.,5.7590309055625E-16,0.));
#129845=DIRECTION('',(-5.7590309055625E-16,1.,0.));
#129846=DIRECTION('center_axis',(5.7590309055625E-16,-1.,0.));
#129847=DIRECTION('ref_axis',(1.,5.7590309055625E-16,0.));
#129848=DIRECTION('',(-5.7590309055625E-16,1.,0.));
#129849=DIRECTION('center_axis',(5.7590309055625E-16,-1.,0.));
#129850=DIRECTION('ref_axis',(1.,5.7590309055625E-16,0.));
#129851=DIRECTION('',(-5.7590309055625E-16,1.,0.));
#129852=DIRECTION('center_axis',(5.7590309055625E-16,-1.,0.));
#129853=DIRECTION('ref_axis',(1.,5.7590309055625E-16,0.));
#129854=DIRECTION('',(-5.7590309055625E-16,1.,0.));
#129855=DIRECTION('center_axis',(5.7590309055625E-16,-1.,0.));
#129856=DIRECTION('ref_axis',(1.,5.7590309055625E-16,0.));
#129857=DIRECTION('',(-5.7590309055625E-16,1.,0.));
#129858=DIRECTION('center_axis',(5.7590309055625E-16,-1.,0.));
#129859=DIRECTION('ref_axis',(1.,5.7590309055625E-16,0.));
#129860=DIRECTION('',(-5.7590309055625E-16,1.,0.));
#129861=DIRECTION('center_axis',(5.7590309055625E-16,-1.,0.));
#129862=DIRECTION('ref_axis',(1.,5.7590309055625E-16,0.));
#129863=DIRECTION('',(-5.7590309055625E-16,1.,0.));
#129864=DIRECTION('center_axis',(5.7590309055625E-16,-1.,0.));
#129865=DIRECTION('ref_axis',(1.,5.7590309055625E-16,0.));
#129866=DIRECTION('',(-5.7590309055625E-16,1.,0.));
#129867=DIRECTION('center_axis',(5.7590309055625E-16,-1.,0.));
#129868=DIRECTION('ref_axis',(1.,5.7590309055625E-16,0.));
#129869=DIRECTION('',(-5.7590309055625E-16,1.,0.));
#129870=DIRECTION('center_axis',(5.7590309055625E-16,-1.,0.));
#129871=DIRECTION('ref_axis',(1.,5.7590309055625E-16,0.));
#129872=DIRECTION('',(-5.7590309055625E-16,1.,0.));
#129873=DIRECTION('center_axis',(5.7590309055625E-16,-1.,0.));
#129874=DIRECTION('ref_axis',(1.,5.7590309055625E-16,0.));
#129875=DIRECTION('',(-5.7590309055625E-16,1.,0.));
#129876=DIRECTION('center_axis',(5.7590309055625E-16,-1.,0.));
#129877=DIRECTION('ref_axis',(1.,5.7590309055625E-16,0.));
#129878=DIRECTION('',(-5.7590309055625E-16,1.,0.));
#129879=DIRECTION('center_axis',(5.7590309055625E-16,-1.,0.));
#129880=DIRECTION('ref_axis',(1.,5.7590309055625E-16,0.));
#129881=DIRECTION('',(-5.7590309055625E-16,1.,0.));
#129882=DIRECTION('center_axis',(5.7590309055625E-16,-1.,0.));
#129883=DIRECTION('ref_axis',(1.,5.7590309055625E-16,0.));
#129884=DIRECTION('center_axis',(-5.7590309055625E-16,1.,0.));
#129885=DIRECTION('ref_axis',(-1.,-5.7590309055625E-16,0.));
#129886=DIRECTION('center_axis',(5.7590309055625E-16,-1.,0.));
#129887=DIRECTION('ref_axis',(1.,5.7590309055625E-16,0.));
#129888=DIRECTION('',(-0.707106781186543,-0.707106781186552,-8.65956056235488E-17));
#129889=DIRECTION('center_axis',(0.,1.,0.));
#129890=DIRECTION('ref_axis',(0.,0.,1.));
#129891=DIRECTION('center_axis',(-4.06800079821994E-15,1.,1.09435932434982E-14));
#129892=DIRECTION('ref_axis',(-0.0356547078254615,1.0603593140283E-14,-0.99936416876426));
#129893=DIRECTION('center_axis',(5.7590309055625E-16,-1.,0.));
#129894=DIRECTION('ref_axis',(1.,5.7590309055625E-16,0.));
#129895=DIRECTION('center_axis',(-1.00842205057537E-14,-1.,9.21063889230093E-14));
#129896=DIRECTION('ref_axis',(-0.481354876138532,8.48287451222583E-14,0.876525802938886));
#129897=DIRECTION('',(0.707106781186546,0.707106781186549,8.65956056235493E-17));
#129898=DIRECTION('center_axis',(-5.7590309055625E-16,1.,0.));
#129899=DIRECTION('ref_axis',(-1.,-5.7590309055625E-16,0.));
#129900=DIRECTION('center_axis',(5.7590309055625E-16,-1.,0.));
#129901=DIRECTION('ref_axis',(1.,5.7590309055625E-16,0.));
#129902=DIRECTION('center_axis',(0.,-1.,0.));
#129903=DIRECTION('ref_axis',(0.,0.,-1.));
#129904=DIRECTION('center_axis',(-1.8547604288613E-34,-1.,8.30248970910064E-18));
#129905=DIRECTION('ref_axis',(-1.,0.,-2.23398100310589E-17));
#129906=DIRECTION('center_axis',(-5.7590309055625E-16,1.,0.));
#129907=DIRECTION('ref_axis',(-1.,-5.7590309055625E-16,0.));
#129908=DIRECTION('center_axis',(0.,-1.,0.));
#129909=DIRECTION('ref_axis',(0.,0.,-1.));
#129910=DIRECTION('',(0.,0.,-1.));
#129911=DIRECTION('',(-1.,0.,0.));
#129912=DIRECTION('',(0.,0.,1.));
#129913=DIRECTION('',(1.,0.,0.));
#129914=DIRECTION('center_axis',(0.,-1.,0.));
#129915=DIRECTION('ref_axis',(0.,0.,-1.));
#129916=DIRECTION('',(0.,0.,-1.));
#129917=DIRECTION('',(1.,0.,0.));
#129918=DIRECTION('',(0.,0.,1.));
#129919=DIRECTION('',(-1.,0.,0.));
#129920=DIRECTION('center_axis',(0.,1.,0.));
#129921=DIRECTION('ref_axis',(0.,0.,1.));
#129922=DIRECTION('center_axis',(0.,1.,0.));
#129923=DIRECTION('ref_axis',(0.,0.,1.));
#129924=DIRECTION('center_axis',(0.,1.,0.));
#129925=DIRECTION('ref_axis',(0.,0.,1.));
#129926=DIRECTION('center_axis',(0.,1.,0.));
#129927=DIRECTION('ref_axis',(0.,0.,1.));
#129928=DIRECTION('center_axis',(0.,1.,0.));
#129929=DIRECTION('ref_axis',(0.,0.,1.));
#129930=DIRECTION('center_axis',(0.,1.,0.));
#129931=DIRECTION('ref_axis',(0.,0.,1.));
#129932=DIRECTION('center_axis',(-1.,0.,0.));
#129933=DIRECTION('ref_axis',(0.,0.,1.));
#129934=DIRECTION('',(0.,-1.,0.));
#129935=DIRECTION('',(0.,-1.,0.));
#129936=DIRECTION('center_axis',(0.,0.,1.));
#129937=DIRECTION('ref_axis',(1.,0.,0.));
#129938=DIRECTION('',(0.,-1.,0.));
#129939=DIRECTION('center_axis',(1.,0.,0.));
#129940=DIRECTION('ref_axis',(0.,0.,-1.));
#129941=DIRECTION('',(0.,-1.,0.));
#129942=DIRECTION('center_axis',(0.,0.,-1.));
#129943=DIRECTION('ref_axis',(-1.,0.,0.));
#129944=DIRECTION('center_axis',(0.866025403784439,4.98746706539683E-16,
0.5));
#129945=DIRECTION('ref_axis',(0.5,-2.05225318506028E-32,-0.866025403784439));
#129946=DIRECTION('',(-5.7590309055625E-16,1.,0.));
#129947=DIRECTION('',(-5.7590309055625E-16,1.,0.));
#129948=DIRECTION('center_axis',(0.,0.,1.));
#129949=DIRECTION('ref_axis',(1.,0.,0.));
#129950=DIRECTION('',(-5.7590309055625E-16,1.,0.));
#129951=DIRECTION('center_axis',(-0.866025403784439,-4.98746706539683E-16,
0.5));
#129952=DIRECTION('ref_axis',(0.5,-2.05225318506028E-32,0.866025403784439));
#129953=DIRECTION('',(-5.7590309055625E-16,1.,0.));
#129954=DIRECTION('center_axis',(-0.866025403784439,-4.98746706539683E-16,
-0.5));
#129955=DIRECTION('ref_axis',(-0.5,-1.07348290155056E-32,0.866025403784439));
#129956=DIRECTION('',(-5.7590309055625E-16,1.,0.));
#129957=DIRECTION('center_axis',(-1.66923844304129E-16,-9.61319578222781E-32,
-1.));
#129958=DIRECTION('ref_axis',(-1.,-9.085955592469E-64,1.66923844304129E-16));
#129959=DIRECTION('',(-5.7590309055625E-16,1.,0.));
#129960=DIRECTION('center_axis',(0.866025403784439,4.98746706539683E-16,
-0.5));
#129961=DIRECTION('ref_axis',(-0.5,-2.03743871581167E-32,-0.866025403784439));
#129962=DIRECTION('center_axis',(0.,1.,0.));
#129963=DIRECTION('ref_axis',(0.,0.,1.));
#129964=DIRECTION('center_axis',(0.,1.,0.));
#129965=DIRECTION('ref_axis',(0.,0.,1.));
#129966=DIRECTION('center_axis',(0.,-1.,0.));
#129967=DIRECTION('ref_axis',(0.,0.,1.));
#129968=DIRECTION('center_axis',(0.,-1.,0.));
#129969=DIRECTION('ref_axis',(0.,0.,1.));
#129970=DIRECTION('center_axis',(0.,-1.,0.));
#129971=DIRECTION('ref_axis',(1.77635683940025E-15,0.,1.));
#129972=DIRECTION('center_axis',(0.,-1.,0.));
#129973=DIRECTION('ref_axis',(0.,0.,1.));
#129974=DIRECTION('center_axis',(0.,-1.,0.));
#129975=DIRECTION('ref_axis',(1.77635683940025E-15,0.,1.));
#129976=DIRECTION('center_axis',(-2.16306263935159E-15,1.,3.41586791986892E-31));
#129977=DIRECTION('ref_axis',(7.38873627842809E-46,-3.41586791986892E-31,
1.));
#129978=DIRECTION('center_axis',(-2.16306263935159E-15,1.,3.41586791986892E-31));
#129979=DIRECTION('ref_axis',(7.38873627842809E-46,-3.41586791986892E-31,
1.));
#129980=DIRECTION('center_axis',(-2.16306263935159E-15,1.,3.41586791986892E-31));
#129981=DIRECTION('ref_axis',(7.38873627842809E-46,-3.41586791986892E-31,
1.));
#129982=DIRECTION('center_axis',(-2.16306263935159E-15,1.,3.41586791986892E-31));
#129983=DIRECTION('ref_axis',(7.38873627842809E-46,-3.41586791986892E-31,
1.));
#129984=DIRECTION('center_axis',(-2.16306263935159E-15,1.,3.41586791986892E-31));
#129985=DIRECTION('ref_axis',(7.38873627842809E-46,-3.41586791986892E-31,
1.));
#129986=DIRECTION('center_axis',(-2.16306263935159E-15,1.,3.41586791986892E-31));
#129987=DIRECTION('ref_axis',(7.38873627842809E-46,-3.41586791986892E-31,
1.));
#129988=DIRECTION('center_axis',(2.16306263935159E-15,-1.,-3.41586791986892E-31));
#129989=DIRECTION('ref_axis',(7.38873627842809E-46,-3.41586791986892E-31,
1.));
#129990=DIRECTION('center_axis',(2.16306263935159E-15,-1.,-3.41586791986892E-31));
#129991=DIRECTION('ref_axis',(7.38873627842809E-46,-3.41586791986892E-31,
1.));
#129992=DIRECTION('center_axis',(2.16306263935159E-15,-1.,-3.41586791986892E-31));
#129993=DIRECTION('ref_axis',(7.38873627842809E-46,-3.41586791986892E-31,
1.));
#129994=DIRECTION('center_axis',(2.16306263935159E-15,-1.,-3.41586791986892E-31));
#129995=DIRECTION('ref_axis',(7.38873627842809E-46,-3.41586791986892E-31,
1.));
#129996=DIRECTION('center_axis',(2.16306263935159E-15,-1.,-3.41586791986892E-31));
#129997=DIRECTION('ref_axis',(7.38873627842809E-46,-3.41586791986892E-31,
1.));
#129998=DIRECTION('center_axis',(2.16306263935159E-15,-1.,-3.41586791986892E-31));
#129999=DIRECTION('ref_axis',(7.38873627842809E-46,-3.41586791986892E-31,
1.));
#130000=DIRECTION('center_axis',(-5.7590309055625E-16,1.,0.));
#130001=DIRECTION('ref_axis',(-1.,-5.7590309055625E-16,0.));
#130002=DIRECTION('center_axis',(-1.8547604288613E-34,-1.,8.30248970910064E-18));
#130003=DIRECTION('ref_axis',(-1.,0.,-2.23398100310589E-17));
#130004=DIRECTION('center_axis',(0.,-1.,0.));
#130005=DIRECTION('ref_axis',(0.,0.,-1.));
#130006=DIRECTION('center_axis',(0.,-1.,0.));
#130007=DIRECTION('ref_axis',(0.,0.,-1.));
#130008=DIRECTION('',(0.,-1.,0.));
#130009=DIRECTION('center_axis',(0.,-1.,0.));
#130010=DIRECTION('ref_axis',(0.,0.,-1.));
#130011=DIRECTION('center_axis',(0.,-1.,0.));
#130012=DIRECTION('ref_axis',(0.,0.,-1.));
#130013=DIRECTION('center_axis',(0.,-1.,0.));
#130014=DIRECTION('ref_axis',(0.,0.,-1.));
#130015=DIRECTION('',(0.,-1.,0.));
#130016=DIRECTION('center_axis',(0.,-1.,0.));
#130017=DIRECTION('ref_axis',(0.,0.,-1.));
#130018=DIRECTION('center_axis',(0.,-1.,0.));
#130019=DIRECTION('ref_axis',(0.,0.,-1.));
#130020=DIRECTION('center_axis',(0.,-1.,0.));
#130021=DIRECTION('ref_axis',(0.,0.,-1.));
#130022=DIRECTION('',(0.,-1.,0.));
#130023=DIRECTION('center_axis',(0.,-1.,0.));
#130024=DIRECTION('ref_axis',(0.,0.,-1.));
#130025=DIRECTION('center_axis',(0.,-1.,0.));
#130026=DIRECTION('ref_axis',(0.,0.,-1.));
#130027=DIRECTION('center_axis',(0.,-1.,0.));
#130028=DIRECTION('ref_axis',(0.,0.,-1.));
#130029=DIRECTION('',(0.,-1.,0.));
#130030=DIRECTION('center_axis',(0.,-1.,0.));
#130031=DIRECTION('ref_axis',(0.,0.,-1.));
#130032=DIRECTION('center_axis',(0.,-1.,0.));
#130033=DIRECTION('ref_axis',(0.,0.,-1.));
#130034=DIRECTION('center_axis',(0.,-1.,0.));
#130035=DIRECTION('ref_axis',(0.,0.,-1.));
#130036=DIRECTION('',(0.,-1.,0.));
#130037=DIRECTION('center_axis',(0.,-1.,0.));
#130038=DIRECTION('ref_axis',(0.,0.,-1.));
#130039=DIRECTION('center_axis',(0.,-1.,0.));
#130040=DIRECTION('ref_axis',(0.,0.,-1.));
#130041=DIRECTION('center_axis',(0.,-1.,0.));
#130042=DIRECTION('ref_axis',(0.,0.,-1.));
#130043=DIRECTION('',(0.,-1.,0.));
#130044=DIRECTION('center_axis',(0.,-1.,0.));
#130045=DIRECTION('ref_axis',(0.,0.,-1.));
#130046=DIRECTION('center_axis',(0.,-1.,0.));
#130047=DIRECTION('ref_axis',(0.,0.,-1.));
#130048=DIRECTION('center_axis',(0.,-1.,0.));
#130049=DIRECTION('ref_axis',(0.,0.,-1.));
#130050=DIRECTION('',(0.,-1.,0.));
#130051=DIRECTION('center_axis',(0.,-1.,0.));
#130052=DIRECTION('ref_axis',(0.,0.,-1.));
#130053=DIRECTION('center_axis',(0.,-1.,0.));
#130054=DIRECTION('ref_axis',(0.,0.,-1.));
#130055=DIRECTION('center_axis',(0.,-1.,0.));
#130056=DIRECTION('ref_axis',(0.,0.,-1.));
#130057=DIRECTION('',(0.,-1.,0.));
#130058=DIRECTION('center_axis',(0.,-1.,0.));
#130059=DIRECTION('ref_axis',(0.,0.,-1.));
#130060=DIRECTION('center_axis',(0.,-1.,0.));
#130061=DIRECTION('ref_axis',(0.,0.,-1.));
#130062=DIRECTION('center_axis',(0.,-1.,0.));
#130063=DIRECTION('ref_axis',(0.,0.,-1.));
#130064=DIRECTION('',(0.,-1.,0.));
#130065=DIRECTION('center_axis',(0.,-1.,0.));
#130066=DIRECTION('ref_axis',(0.,0.,-1.));
#130067=DIRECTION('center_axis',(0.,-1.,0.));
#130068=DIRECTION('ref_axis',(0.,0.,-1.));
#130069=DIRECTION('center_axis',(0.,-1.,0.));
#130070=DIRECTION('ref_axis',(0.,0.,-1.));
#130071=DIRECTION('',(0.,1.,0.));
#130072=DIRECTION('center_axis',(0.,1.,0.));
#130073=DIRECTION('ref_axis',(0.,0.,1.));
#130074=DIRECTION('center_axis',(0.,1.,0.));
#130075=DIRECTION('ref_axis',(0.,0.,1.));
#130076=DIRECTION('center_axis',(0.,1.,0.));
#130077=DIRECTION('ref_axis',(0.,0.,1.));
#130078=DIRECTION('',(0.,1.,0.));
#130079=DIRECTION('center_axis',(0.,1.,0.));
#130080=DIRECTION('ref_axis',(0.,0.,1.));
#130081=DIRECTION('center_axis',(-6.12323399573677E-17,0.,1.));
#130082=DIRECTION('ref_axis',(-1.,0.,0.));
#130083=DIRECTION('center_axis',(1.22000879772301E-18,1.,0.));
#130084=DIRECTION('ref_axis',(-1.,1.22000879772301E-18,0.));
#130085=DIRECTION('center_axis',(1.22000879772301E-18,1.,0.));
#130086=DIRECTION('ref_axis',(-1.,1.22000879772301E-18,0.));
#130087=DIRECTION('center_axis',(0.,1.,0.));
#130088=DIRECTION('ref_axis',(0.,0.,1.));
#130089=DIRECTION('center_axis',(0.,1.,0.));
#130090=DIRECTION('ref_axis',(0.,0.,1.));
#130091=DIRECTION('center_axis',(-1.,0.,1.22464679914735E-16));
#130092=DIRECTION('ref_axis',(-1.22464679914735E-16,0.,-1.));
#130093=DIRECTION('center_axis',(0.,-1.,0.));
#130094=DIRECTION('ref_axis',(0.,0.,1.));
#130095=DIRECTION('center_axis',(0.,-1.,0.));
#130096=DIRECTION('ref_axis',(0.,0.,-1.));
#130097=DIRECTION('center_axis',(0.,-1.,0.));
#130098=DIRECTION('ref_axis',(0.,0.,-1.));
#130099=DIRECTION('center_axis',(-1.,0.,-1.22464679914735E-16));
#130100=DIRECTION('ref_axis',(-1.22464679914735E-16,0.,1.));
#130101=DIRECTION('center_axis',(0.,1.,0.));
#130102=DIRECTION('ref_axis',(0.,0.,-1.));
#130103=DIRECTION('center_axis',(0.,1.,0.));
#130104=DIRECTION('ref_axis',(0.,0.,-1.));
#130105=DIRECTION('center_axis',(0.,1.,0.));
#130106=DIRECTION('ref_axis',(0.,0.,1.));
#130107=DIRECTION('',(0.,1.,0.));
#130108=DIRECTION('center_axis',(0.,1.,0.));
#130109=DIRECTION('ref_axis',(0.,0.,1.));
#130110=DIRECTION('center_axis',(0.,1.,0.));
#130111=DIRECTION('ref_axis',(0.,0.,1.));
#130112=DIRECTION('center_axis',(1.,0.,-1.22464679914735E-16));
#130113=DIRECTION('ref_axis',(-1.22464679914735E-16,0.,-1.));
#130114=DIRECTION('center_axis',(0.,1.,0.));
#130115=DIRECTION('ref_axis',(0.,0.,1.));
#130116=DIRECTION('center_axis',(0.,1.,0.));
#130117=DIRECTION('ref_axis',(0.,0.,1.));
#130118=DIRECTION('',(0.,1.,0.));
#130119=DIRECTION('center_axis',(0.,1.,0.));
#130120=DIRECTION('ref_axis',(0.,0.,1.));
#130121=DIRECTION('center_axis',(0.,-1.,0.));
#130122=DIRECTION('ref_axis',(0.,0.,-1.));
#130123=DIRECTION('center_axis',(0.,-1.,0.));
#130124=DIRECTION('ref_axis',(0.,0.,-1.));
#130125=DIRECTION('center_axis',(0.,1.,0.));
#130126=DIRECTION('ref_axis',(0.,0.,1.));
#130127=DIRECTION('center_axis',(0.,-1.,0.));
#130128=DIRECTION('ref_axis',(0.,0.,-1.));
#130129=DIRECTION('center_axis',(0.,-1.,0.));
#130130=DIRECTION('ref_axis',(0.,0.,-1.));
#130131=DIRECTION('center_axis',(0.,-1.,0.));
#130132=DIRECTION('ref_axis',(0.,0.,-1.));
#130133=DIRECTION('center_axis',(0.,-1.,0.));
#130134=DIRECTION('ref_axis',(0.,0.,-1.));
#130135=DIRECTION('center_axis',(0.,-1.,0.));
#130136=DIRECTION('ref_axis',(0.,0.,-1.));
#130137=DIRECTION('center_axis',(0.,-1.,0.));
#130138=DIRECTION('ref_axis',(0.,0.,-1.));
#130139=DIRECTION('center_axis',(0.,-1.,0.));
#130140=DIRECTION('ref_axis',(0.,0.,-1.));
#130141=DIRECTION('center_axis',(0.,-1.,0.));
#130142=DIRECTION('ref_axis',(0.,0.,-1.));
#130143=DIRECTION('center_axis',(0.,-1.,0.));
#130144=DIRECTION('ref_axis',(0.,0.,-1.));
#130145=DIRECTION('center_axis',(0.,1.,0.));
#130146=DIRECTION('ref_axis',(0.,0.,1.));
#275559=CARTESIAN_POINT('',(0.,0.,0.));
#275560=CARTESIAN_POINT('Origin',(-3.77475828372553E-14,-1.881249999982,
2.68644078414671E-15));
#275561=CARTESIAN_POINT('',(10.0514428414941,107.431249999581,1.00171110072065E-15));
#275562=CARTESIAN_POINT('',(10.0514428414941,107.431911591494,-1.23094673026484E-15));
#275563=CARTESIAN_POINT('',(10.0514428414941,-1.881249999982,4.14193483802857E-15));
#275564=CARTESIAN_POINT('',(10.0514325246607,107.431911591494,-0.0144013199032517));
#275565=CARTESIAN_POINT('Origin',(-3.77475828372553E-14,107.431911591494,
1.77886938496422E-15));
#275566=CARTESIAN_POINT('Ctrl Pts',(10.0514428414941,107.431249999581,-1.23094673026484E-15));
#275567=CARTESIAN_POINT('Ctrl Pts',(10.0514428414941,107.431580718727,-0.00720066364701881));
#275568=CARTESIAN_POINT('Ctrl Pts',(10.0514325246607,107.431911591494,-0.0144013199032517));
#275569=CARTESIAN_POINT('Origin',(-3.77475828372553E-14,-1.881249999982,
2.68644078414671E-15));
#275570=CARTESIAN_POINT('',(10.0514428414941,104.431249999593,1.01416483528425E-15));
#275571=CARTESIAN_POINT('',(10.0514428414941,104.806249999591,1.0126081184638E-15));
#275572=CARTESIAN_POINT('',(10.0514428414941,-1.881249999982,4.14193483802857E-15));
#275573=CARTESIAN_POINT('',(7.10339095491525,107.431911591494,7.11149352368764));
#275574=CARTESIAN_POINT('Ctrl Pts',(10.0514428414941,104.806249999591,-1.23094673026484E-15));
#275575=CARTESIAN_POINT('Ctrl Pts',(10.0514428414941,104.956249999591,-3.26591175476071));
#275576=CARTESIAN_POINT('Ctrl Pts',(8.13178807675712,105.10624999959,-5.90808986649102));
#275577=CARTESIAN_POINT('Ctrl Pts',(6.21213331202014,105.256249999589,-8.55026797822134));
#275578=CARTESIAN_POINT('Ctrl Pts',(3.10606665601003,105.406249999589,-9.5594902125713));
#275579=CARTESIAN_POINT('Ctrl Pts',(-7.39149410146522E-14,105.556249999588,
-10.5687124469213));
#275580=CARTESIAN_POINT('Ctrl Pts',(-3.10606665601018,105.706249999588,
-9.5594902125713));
#275581=CARTESIAN_POINT('Ctrl Pts',(-6.21213331202029,105.856249999587,
-8.55026797822134));
#275582=CARTESIAN_POINT('Ctrl Pts',(-8.13178807675726,106.006249999586,
-5.90808986649102));
#275583=CARTESIAN_POINT('Ctrl Pts',(-10.0514428414942,106.156249999586,
-3.2659117547607));
#275584=CARTESIAN_POINT('Ctrl Pts',(-10.0514428414942,106.306249999585,
2.46189346052968E-15));
#275585=CARTESIAN_POINT('Ctrl Pts',(-10.0514428414942,106.456249999585,
3.26591175476071));
#275586=CARTESIAN_POINT('Ctrl Pts',(-8.13178807675726,106.606249999584,
5.90808986649102));
#275587=CARTESIAN_POINT('Ctrl Pts',(-6.21213331202029,106.756249999583,
8.55026797822134));
#275588=CARTESIAN_POINT('Ctrl Pts',(-3.10606665601018,106.906249999583,
9.5594902125713));
#275589=CARTESIAN_POINT('Ctrl Pts',(-7.21902076766369E-14,107.056249999582,
10.5687124469213));
#275590=CARTESIAN_POINT('Ctrl Pts',(3.10606665601003,107.206249999582,9.5594902125713));
#275591=CARTESIAN_POINT('Ctrl Pts',(5.3982158846568,107.316943819893,8.8147257814789));
#275592=CARTESIAN_POINT('Ctrl Pts',(7.10339095491525,107.431911591494,7.11149352368764));
#275593=CARTESIAN_POINT('Origin',(-3.77475828372553E-14,107.431911591494,
1.77886938496422E-15));
#275594=CARTESIAN_POINT('Ctrl Pts',(10.0514428414941,104.431249999593,-1.23094673026484E-15));
#275595=CARTESIAN_POINT('Ctrl Pts',(10.0514428414941,104.581249999592,-3.26591175476071));
#275596=CARTESIAN_POINT('Ctrl Pts',(8.13178807675712,104.731249999592,-5.90808986649102));
#275597=CARTESIAN_POINT('Ctrl Pts',(6.21213331202014,104.881249999591,-8.55026797822134));
#275598=CARTESIAN_POINT('Ctrl Pts',(3.10606665601003,105.03124999959,-9.5594902125713));
#275599=CARTESIAN_POINT('Ctrl Pts',(-7.36989773556944E-14,105.18124999959,
-10.5687124469213));
#275600=CARTESIAN_POINT('Ctrl Pts',(-3.10606665601018,105.331249999589,
-9.5594902125713));
#275601=CARTESIAN_POINT('Ctrl Pts',(-6.21213331202029,105.481249999589,
-8.55026797822134));
#275602=CARTESIAN_POINT('Ctrl Pts',(-8.13178807675726,105.631249999588,
-5.90808986649102));
#275603=CARTESIAN_POINT('Ctrl Pts',(-10.0514428414942,105.781249999587,
-3.2659117547607));
#275604=CARTESIAN_POINT('Ctrl Pts',(-10.0514428414942,105.931249999587,
2.46189346052968E-15));
#275605=CARTESIAN_POINT('Ctrl Pts',(-10.0514428414942,106.081249999586,
3.26591175476071));
#275606=CARTESIAN_POINT('Ctrl Pts',(-8.13178807675726,106.231249999586,
5.90808986649102));
#275607=CARTESIAN_POINT('Ctrl Pts',(-6.21213331202029,106.381249999585,
8.55026797822134));
#275608=CARTESIAN_POINT('Ctrl Pts',(-3.10606665601018,106.531249999584,
9.5594902125713));
#275609=CARTESIAN_POINT('Ctrl Pts',(-7.19742440176792E-14,106.681249999584,
10.5687124469213));
#275610=CARTESIAN_POINT('Ctrl Pts',(3.10606665601004,106.831249999583,9.5594902125713));
#275611=CARTESIAN_POINT('Ctrl Pts',(6.21213331202014,106.981249999583,8.55026797822134));
#275612=CARTESIAN_POINT('Ctrl Pts',(8.13178807675711,107.131249999582,5.90808986649102));
#275613=CARTESIAN_POINT('Ctrl Pts',(10.0514428414941,107.281249999581,3.2659117547607));
#275614=CARTESIAN_POINT('Ctrl Pts',(10.0514428414941,107.431249999581,-1.23094673026484E-15));
#275615=CARTESIAN_POINT('Origin',(-3.77475828372553E-14,-1.881249999982,
2.68644078414671E-15));
#275616=CARTESIAN_POINT('',(10.0514428414941,101.431249999605,1.02661856984785E-15));
#275617=CARTESIAN_POINT('',(10.0514428414941,101.806249999603,1.0250618530274E-15));
#275618=CARTESIAN_POINT('',(10.0514428414941,-1.881249999982,4.14193483802857E-15));
#275619=CARTESIAN_POINT('Ctrl Pts',(10.0514428414941,101.806249999603,-1.23094673026484E-15));
#275620=CARTESIAN_POINT('Ctrl Pts',(10.0514428414941,101.956249999603,-3.26591175476071));
#275621=CARTESIAN_POINT('Ctrl Pts',(8.13178807675712,102.106249999602,-5.90808986649102));
#275622=CARTESIAN_POINT('Ctrl Pts',(6.21213331202014,102.256249999601,-8.55026797822134));
#275623=CARTESIAN_POINT('Ctrl Pts',(3.10606665601004,102.406249999601,-9.5594902125713));
#275624=CARTESIAN_POINT('Ctrl Pts',(-7.21872317429903E-14,102.5562499996,
-10.5687124469213));
#275625=CARTESIAN_POINT('Ctrl Pts',(-3.10606665601018,102.7062499996,-9.5594902125713));
#275626=CARTESIAN_POINT('Ctrl Pts',(-6.21213331202029,102.856249999599,
-8.55026797822134));
#275627=CARTESIAN_POINT('Ctrl Pts',(-8.13178807675726,103.006249999598,
-5.90808986649102));
#275628=CARTESIAN_POINT('Ctrl Pts',(-10.0514428414942,103.156249999598,
-3.2659117547607));
#275629=CARTESIAN_POINT('Ctrl Pts',(-10.0514428414942,103.306249999597,
2.46189346052968E-15));
#275630=CARTESIAN_POINT('Ctrl Pts',(-10.0514428414942,103.456249999597,
3.26591175476071));
#275631=CARTESIAN_POINT('Ctrl Pts',(-8.13178807675726,103.606249999596,
5.90808986649102));
#275632=CARTESIAN_POINT('Ctrl Pts',(-6.21213331202029,103.756249999595,
8.55026797822134));
#275633=CARTESIAN_POINT('Ctrl Pts',(-3.10606665601018,103.906249999595,
9.5594902125713));
#275634=CARTESIAN_POINT('Ctrl Pts',(-7.0462498404975E-14,104.056249999594,
10.5687124469213));
#275635=CARTESIAN_POINT('Ctrl Pts',(3.10606665601004,104.206249999594,9.5594902125713));
#275636=CARTESIAN_POINT('Ctrl Pts',(6.21213331202014,104.356249999593,8.55026797822134));
#275637=CARTESIAN_POINT('Ctrl Pts',(8.13178807675712,104.506249999592,5.90808986649102));
#275638=CARTESIAN_POINT('Ctrl Pts',(10.0514428414941,104.656249999592,3.2659117547607));
#275639=CARTESIAN_POINT('Ctrl Pts',(10.0514428414941,104.806249999591,-1.23094673026484E-15));
#275640=CARTESIAN_POINT('Ctrl Pts',(10.0514428414941,101.431249999605,-1.23094673026484E-15));
#275641=CARTESIAN_POINT('Ctrl Pts',(10.0514428414941,101.581249999604,-3.26591175476071));
#275642=CARTESIAN_POINT('Ctrl Pts',(8.13178807675712,101.731249999604,-5.90808986649102));
#275643=CARTESIAN_POINT('Ctrl Pts',(6.21213331202014,101.881249999603,-8.55026797822134));
#275644=CARTESIAN_POINT('Ctrl Pts',(3.10606665601004,102.031249999602,-9.5594902125713));
#275645=CARTESIAN_POINT('Ctrl Pts',(-7.19712680840326E-14,102.181249999602,
-10.5687124469213));
#275646=CARTESIAN_POINT('Ctrl Pts',(-3.10606665601018,102.331249999601,
-9.5594902125713));
#275647=CARTESIAN_POINT('Ctrl Pts',(-6.21213331202029,102.481249999601,
-8.55026797822134));
#275648=CARTESIAN_POINT('Ctrl Pts',(-8.13178807675726,102.6312499996,-5.90808986649102));
#275649=CARTESIAN_POINT('Ctrl Pts',(-10.0514428414942,102.781249999599,
-3.2659117547607));
#275650=CARTESIAN_POINT('Ctrl Pts',(-10.0514428414942,102.931249999599,
2.46189346052968E-15));
#275651=CARTESIAN_POINT('Ctrl Pts',(-10.0514428414942,103.081249999598,
3.26591175476071));
#275652=CARTESIAN_POINT('Ctrl Pts',(-8.13178807675726,103.231249999598,
5.90808986649102));
#275653=CARTESIAN_POINT('Ctrl Pts',(-6.21213331202029,103.381249999597,
8.55026797822134));
#275654=CARTESIAN_POINT('Ctrl Pts',(-3.10606665601018,103.531249999596,
9.5594902125713));
#275655=CARTESIAN_POINT('Ctrl Pts',(-7.02465347460173E-14,103.681249999596,
10.5687124469213));
#275656=CARTESIAN_POINT('Ctrl Pts',(3.10606665601004,103.831249999595,9.5594902125713));
#275657=CARTESIAN_POINT('Ctrl Pts',(6.21213331202014,103.981249999595,8.55026797822134));
#275658=CARTESIAN_POINT('Ctrl Pts',(8.13178807675712,104.131249999594,5.90808986649102));
#275659=CARTESIAN_POINT('Ctrl Pts',(10.0514428414941,104.281249999593,3.2659117547607));
#275660=CARTESIAN_POINT('Ctrl Pts',(10.0514428414941,104.431249999593,-1.23094673026484E-15));
#275661=CARTESIAN_POINT('Origin',(-3.77475828372553E-14,-1.881249999982,
2.68644078414671E-15));
#275662=CARTESIAN_POINT('',(10.0514428414941,98.4312499996168,1.03907230441145E-15));
#275663=CARTESIAN_POINT('',(10.0514428414941,98.8062499996153,1.037515587591E-15));
#275664=CARTESIAN_POINT('',(10.0514428414941,-1.881249999982,4.14193483802857E-15));
#275665=CARTESIAN_POINT('Ctrl Pts',(10.0514428414941,98.8062499996153,-1.23094673026484E-15));
#275666=CARTESIAN_POINT('Ctrl Pts',(10.0514428414941,98.9562499996147,-3.26591175476071));
#275667=CARTESIAN_POINT('Ctrl Pts',(8.13178807675712,99.1062499996141,-5.90808986649102));
#275668=CARTESIAN_POINT('Ctrl Pts',(6.21213331202014,99.2562499996134,-8.55026797822134));
#275669=CARTESIAN_POINT('Ctrl Pts',(3.10606665601004,99.4062499996129,-9.5594902125713));
#275670=CARTESIAN_POINT('Ctrl Pts',(-7.04595224713285E-14,99.5562499996122,
-10.5687124469213));
#275671=CARTESIAN_POINT('Ctrl Pts',(-3.10606665601018,99.7062499996117,
-9.5594902125713));
#275672=CARTESIAN_POINT('Ctrl Pts',(-6.21213331202029,99.856249999611,-8.55026797822134));
#275673=CARTESIAN_POINT('Ctrl Pts',(-8.13178807675726,100.00624999961,-5.90808986649102));
#275674=CARTESIAN_POINT('Ctrl Pts',(-10.0514428414942,100.15624999961,-3.2659117547607));
#275675=CARTESIAN_POINT('Ctrl Pts',(-10.0514428414942,100.306249999609,
2.46189346052968E-15));
#275676=CARTESIAN_POINT('Ctrl Pts',(-10.0514428414942,100.456249999609,
3.26591175476071));
#275677=CARTESIAN_POINT('Ctrl Pts',(-8.13178807675726,100.606249999608,
5.90808986649102));
#275678=CARTESIAN_POINT('Ctrl Pts',(-6.21213331202028,100.756249999607,
8.55026797822134));
#275679=CARTESIAN_POINT('Ctrl Pts',(-3.10606665601018,100.906249999607,
9.5594902125713));
#275680=CARTESIAN_POINT('Ctrl Pts',(-6.87347891333132E-14,101.056249999606,
10.5687124469213));
#275681=CARTESIAN_POINT('Ctrl Pts',(3.10606665601004,101.206249999606,9.5594902125713));
#275682=CARTESIAN_POINT('Ctrl Pts',(6.21213331202015,101.356249999605,8.55026797822134));
#275683=CARTESIAN_POINT('Ctrl Pts',(8.13178807675712,101.506249999604,5.90808986649102));
#275684=CARTESIAN_POINT('Ctrl Pts',(10.0514428414941,101.656249999604,3.2659117547607));
#275685=CARTESIAN_POINT('Ctrl Pts',(10.0514428414941,101.806249999603,-1.23094673026484E-15));
#275686=CARTESIAN_POINT('Ctrl Pts',(10.0514428414941,98.4312499996168,-1.23094673026484E-15));
#275687=CARTESIAN_POINT('Ctrl Pts',(10.0514428414941,98.5812499996162,-3.26591175476071));
#275688=CARTESIAN_POINT('Ctrl Pts',(8.13178807675712,98.7312499996156,-5.90808986649102));
#275689=CARTESIAN_POINT('Ctrl Pts',(6.21213331202014,98.8812499996149,-8.55026797822134));
#275690=CARTESIAN_POINT('Ctrl Pts',(3.10606665601004,99.0312499996143,-9.5594902125713));
#275691=CARTESIAN_POINT('Ctrl Pts',(-7.02435588123707E-14,99.1812499996138,
-10.5687124469213));
#275692=CARTESIAN_POINT('Ctrl Pts',(-3.10606665601018,99.3312499996131,
-9.5594902125713));
#275693=CARTESIAN_POINT('Ctrl Pts',(-6.21213331202029,99.4812499996125,
-8.55026797822134));
#275694=CARTESIAN_POINT('Ctrl Pts',(-8.13178807675726,99.631249999612,-5.90808986649102));
#275695=CARTESIAN_POINT('Ctrl Pts',(-10.0514428414942,99.7812499996114,
-3.2659117547607));
#275696=CARTESIAN_POINT('Ctrl Pts',(-10.0514428414942,99.9312499996108,
2.46189346052968E-15));
#275697=CARTESIAN_POINT('Ctrl Pts',(-10.0514428414942,100.08124999961,3.26591175476071));
#275698=CARTESIAN_POINT('Ctrl Pts',(-8.13178807675726,100.23124999961,5.90808986649102));
#275699=CARTESIAN_POINT('Ctrl Pts',(-6.21213331202028,100.381249999609,
8.55026797822134));
#275700=CARTESIAN_POINT('Ctrl Pts',(-3.10606665601018,100.531249999608,
9.5594902125713));
#275701=CARTESIAN_POINT('Ctrl Pts',(-6.85188254743555E-14,100.681249999608,
10.5687124469213));
#275702=CARTESIAN_POINT('Ctrl Pts',(3.10606665601004,100.831249999607,9.5594902125713));
#275703=CARTESIAN_POINT('Ctrl Pts',(6.21213331202015,100.981249999607,8.55026797822134));
#275704=CARTESIAN_POINT('Ctrl Pts',(8.13178807675712,101.131249999606,5.90808986649102));
#275705=CARTESIAN_POINT('Ctrl Pts',(10.0514428414941,101.281249999605,3.2659117547607));
#275706=CARTESIAN_POINT('Ctrl Pts',(10.0514428414941,101.431249999605,-1.23094673026484E-15));
#275707=CARTESIAN_POINT('Origin',(-3.77475828372553E-14,-1.881249999982,
2.68644078414671E-15));
#275708=CARTESIAN_POINT('',(10.0514428414941,95.4312499996288,1.05152603897505E-15));
#275709=CARTESIAN_POINT('',(10.0514428414941,95.8062499996273,1.0499693221546E-15));
#275710=CARTESIAN_POINT('',(10.0514428414941,-1.881249999982,4.14193483802857E-15));
#275711=CARTESIAN_POINT('',(-5.07904231626403,94.4290259085059,8.67380149331447));
#275712=CARTESIAN_POINT('Ctrl Pts',(-5.07904231626403,94.4290259085059,
8.67380149331447));
#275713=CARTESIAN_POINT('Ctrl Pts',(-4.14047348819779,94.4812958157686,
9.22339105887566));
#275714=CARTESIAN_POINT('Ctrl Pts',(-3.10606665601017,94.5312499996324,
9.5594902125713));
#275715=CARTESIAN_POINT('Ctrl Pts',(-6.50634069310318E-14,94.6812499996317,
10.5687124469213));
#275716=CARTESIAN_POINT('Ctrl Pts',(3.10606665601004,94.8312499996312,9.5594902125713));
#275717=CARTESIAN_POINT('Ctrl Pts',(6.21213331202015,94.9812499996305,8.55026797822134));
#275718=CARTESIAN_POINT('Ctrl Pts',(8.13178807675712,95.13124999963,5.90808986649102));
#275719=CARTESIAN_POINT('Ctrl Pts',(10.0514428414941,95.2812499996293,3.2659117547607));
#275720=CARTESIAN_POINT('Ctrl Pts',(10.0514428414941,95.4312499996288,-1.23094673026484E-15));
#275721=CARTESIAN_POINT('',(-9.71864656122976,94.4290259085058,2.56503649364343));
#275722=CARTESIAN_POINT('Origin',(1.17683640610267E-13,94.4290259085057,
-1.79301018476963E-13));
#275723=CARTESIAN_POINT('Ctrl Pts',(-9.71864656122976,94.4290259085058,
2.56503649364343));
#275724=CARTESIAN_POINT('Ctrl Pts',(-9.23826308175394,94.5197910936883,
4.38515767416034));
#275725=CARTESIAN_POINT('Ctrl Pts',(-8.13178807675726,94.606249999632,5.90808986649102));
#275726=CARTESIAN_POINT('Ctrl Pts',(-6.21213331202028,94.7562499996315,
8.55026797822134));
#275727=CARTESIAN_POINT('Ctrl Pts',(-3.10606665601017,94.9062499996309,
9.5594902125713));
#275728=CARTESIAN_POINT('Ctrl Pts',(-6.52793705899895E-14,95.0562499996302,
10.5687124469213));
#275729=CARTESIAN_POINT('Ctrl Pts',(3.10606665601004,95.2062499996296,9.5594902125713));
#275730=CARTESIAN_POINT('Ctrl Pts',(6.21213331202015,95.3562499996291,8.55026797822134));
#275731=CARTESIAN_POINT('Ctrl Pts',(8.13178807675712,95.5062499996285,5.90808986649102));
#275732=CARTESIAN_POINT('Ctrl Pts',(10.0514428414941,95.6562499996278,3.2659117547607));
#275733=CARTESIAN_POINT('Ctrl Pts',(10.0514428414941,95.8062499996273,-1.23094673026484E-15));
#275734=CARTESIAN_POINT('Origin',(-7.54701734185159E-14,109.38046875,0.));
#275735=CARTESIAN_POINT('',(10.9371370246358,108.317605774636,-5.59181276817946E-13));
#275736=CARTESIAN_POINT('',(11.9999999999999,109.38046875,-1.46957615897682E-15));
#275737=CARTESIAN_POINT('Ctrl Pts',(7.10339095492142,107.431911591495,7.11149352368269));
#275738=CARTESIAN_POINT('Ctrl Pts',(8.21640283011763,107.591475283561,6.22527839381925));
#275739=CARTESIAN_POINT('Ctrl Pts',(8.97013365125207,107.719075998133,5.23075558842423));
#275740=CARTESIAN_POINT('Ctrl Pts',(10.1564570384933,107.968118058239,3.26634758870711));
#275741=CARTESIAN_POINT('Ctrl Pts',(10.6203336593551,108.110353403587,2.01694121932577));
#275742=CARTESIAN_POINT('Ctrl Pts',(10.8812264225221,108.269539083346,0.477180535167351));
#275743=CARTESIAN_POINT('Ctrl Pts',(10.9132812486255,108.293749998626,0.238870532520754));
#275744=CARTESIAN_POINT('Ctrl Pts',(10.9371370246358,108.317605774636,-1.22700460902792E-12));
#275745=CARTESIAN_POINT('Origin',(-6.51327129430312E-14,91.43046875,0.));
#275746=CARTESIAN_POINT('',(-10.1292796487468,94.3511891012534,-1.41514480213812E-13));
#275747=CARTESIAN_POINT('',(-11.2291932872669,93.2512754627332,4.26135578759189E-11));
#275748=CARTESIAN_POINT('',(-13.0500000000001,91.43046875,-1.5981640728873E-15));
#275749=CARTESIAN_POINT('Ctrl Pts',(-10.1292796487468,94.3511891012534,
-3.42503803096861E-13));
#275750=CARTESIAN_POINT('Ctrl Pts',(-10.1042382905,94.3762304595001,0.866661225011173));
#275751=CARTESIAN_POINT('Ctrl Pts',(-9.96696795140311,94.4023681640516,
1.72863551637103));
#275752=CARTESIAN_POINT('Ctrl Pts',(-9.71864656122976,94.4290259085059,
2.56503649364344));
#275753=CARTESIAN_POINT('Ctrl Pts',(-5.07904231626394,94.4290259085059,
8.67380149331451));
#275754=CARTESIAN_POINT('Ctrl Pts',(-5.69337143249224,94.3531311547402,
8.40202310412634));
#275755=CARTESIAN_POINT('Ctrl Pts',(-6.27907719474524,94.2775482324335,
8.06962005777155));
#275756=CARTESIAN_POINT('Ctrl Pts',(-7.39904906850036,94.1258950262357,
7.27704780513819));
#275757=CARTESIAN_POINT('Ctrl Pts',(-7.92712996465539,94.0503398117793,
6.81422983223111));
#275758=CARTESIAN_POINT('Ctrl Pts',(-9.07535528122801,93.8747927058122,
5.57538689591588));
#275759=CARTESIAN_POINT('Ctrl Pts',(-9.97387089070914,93.7211313789459,
4.40428884548453));
#275760=CARTESIAN_POINT('Ctrl Pts',(-10.9571199054006,93.4285476733796,
1.7735086098561));
#275761=CARTESIAN_POINT('Ctrl Pts',(-11.1468677668107,93.3336009831894,
0.846346921087316));
#275762=CARTESIAN_POINT('Ctrl Pts',(-11.2291932872669,93.2512754627332,
8.5342589378412E-11));
#275763=CARTESIAN_POINT('Origin',(-8.79029313101884E-14,130.96875,0.));
#275764=CARTESIAN_POINT('',(-12.0000000000001,92.80624999964,-1.44737980092247E-14));
#275765=CARTESIAN_POINT('',(-12.0000000000001,92.4804687499999,-1.46957615897682E-15));
#275766=CARTESIAN_POINT('',(-12.0000000000001,130.96875,-1.46957615897682E-15));
#275767=CARTESIAN_POINT('',(-9.3029332573012,92.4804687499999,-7.57993620093208));
#275768=CARTESIAN_POINT('Origin',(-6.57374111881153E-14,92.48046875,0.));
#275769=CARTESIAN_POINT('Ctrl Pts',(-9.3029332573012,92.4804687499999,-7.57993620093207));
#275770=CARTESIAN_POINT('Ctrl Pts',(-9.96781199016407,92.5216290384817,
-6.76392372905115));
#275771=CARTESIAN_POINT('Ctrl Pts',(-10.5224449433889,92.5621874194225,
-5.86397241395083));
#275772=CARTESIAN_POINT('Ctrl Pts',(-11.3879370382823,92.6473816274152,
-3.93068574796497));
#275773=CARTESIAN_POINT('Ctrl Pts',(-11.6918564422266,92.6906603937711,
-2.90446525895254));
#275774=CARTESIAN_POINT('Ctrl Pts',(-11.9521621005444,92.7580357386561,
-1.23771756688517));
#275775=CARTESIAN_POINT('Ctrl Pts',(-12.0000000000001,92.7824500276289,
-0.618646374098709));
#275776=CARTESIAN_POINT('Ctrl Pts',(-12.0000000000001,92.80624999964,-1.40165656858926E-14));
#275777=CARTESIAN_POINT('Origin',(-8.79029313101884E-14,130.96875,0.));
#275778=CARTESIAN_POINT('',(-12.0000000000001,95.806249999628,1.5016501082381E-14));
#275779=CARTESIAN_POINT('',(-12.0000000000001,95.431249999628,6.34288370249696E-15));
#275780=CARTESIAN_POINT('',(-12.0000000000001,130.96875,-1.46957615897682E-15));
#275781=CARTESIAN_POINT('',(-11.9338891906744,92.48046875,1.25789060919729));
#275782=CARTESIAN_POINT('Ctrl Pts',(-12.0000000000001,95.431249999628,-1.94289029309402E-15));
#275783=CARTESIAN_POINT('Ctrl Pts',(-12.0000000000001,95.3976641187748,
-0.873017136364969));
#275784=CARTESIAN_POINT('Ctrl Pts',(-11.9047347890664,95.3629119207413,
-1.74539748324885));
#275785=CARTESIAN_POINT('Ctrl Pts',(-11.3767138011809,95.2648407604998,
-4.12305319186097));
#275786=CARTESIAN_POINT('Ctrl Pts',(-10.7455985797956,95.2015050546979,
-5.56431288903644));
#275787=CARTESIAN_POINT('Ctrl Pts',(-8.95241664100026,95.0797473280993,
-8.14659144143737));
#275788=CARTESIAN_POINT('Ctrl Pts',(-7.79912443701758,95.0163880159116,
-9.25672200041033));
#275789=CARTESIAN_POINT('Ctrl Pts',(-5.16054929757683,94.8899343416185,
-10.9434853481133));
#275790=CARTESIAN_POINT('Ctrl Pts',(-3.70891226333863,94.8312786522147,
-11.5167337635027));
#275791=CARTESIAN_POINT('Ctrl Pts',(-0.642921654553635,94.7072567268602,
-12.0854313202532));
#275792=CARTESIAN_POINT('Ctrl Pts',(0.944038589215958,94.6430628365301,
-12.065646538642));
#275793=CARTESIAN_POINT('Ctrl Pts',(4.01115415839253,94.5189954055718,-11.4172439533036));
#275794=CARTESIAN_POINT('Ctrl Pts',(5.46251131982209,94.4592323691957,-10.7983224510908));
#275795=CARTESIAN_POINT('Ctrl Pts',(8.03555543718115,94.3333675962428,-9.04613168988572));
#275796=CARTESIAN_POINT('Ctrl Pts',(9.13561348468754,94.2722709092646,-7.93365723288517));
#275797=CARTESIAN_POINT('Ctrl Pts',(10.8714801211651,94.1501067125908,-5.32219019919355));
#275798=CARTESIAN_POINT('Ctrl Pts',(11.478882329683,94.0855139334344,-3.84054984568375));
#275799=CARTESIAN_POINT('Ctrl Pts',(12.075644253326,93.9596281460411,-0.762227804634905));
#275800=CARTESIAN_POINT('Ctrl Pts',(12.073058682881,93.9013041019789,0.802139162615167));
#275801=CARTESIAN_POINT('Ctrl Pts',(11.470686639618,93.7763142357512,3.85535017066264));
#275802=CARTESIAN_POINT('Ctrl Pts',(10.8719169399683,93.7127014512904,5.31432183002772));
#275803=CARTESIAN_POINT('Ctrl Pts',(9.14006629815543,93.590267568913,7.93410383523557));
#275804=CARTESIAN_POINT('Ctrl Pts',(8.01845603372403,93.5280963364804,9.06617177346286));
#275805=CARTESIAN_POINT('Ctrl Pts',(5.42793703261786,93.4017787800147,10.8133538109976));
#275806=CARTESIAN_POINT('Ctrl Pts',(3.99082685614984,93.342682337048,11.4221031877892));
#275807=CARTESIAN_POINT('Ctrl Pts',(0.936043788692094,93.2191137662634,
12.0667624748179));
#275808=CARTESIAN_POINT('Ctrl Pts',(-0.654821989464978,93.1547618937488,
12.0852847774843));
#275809=CARTESIAN_POINT('Ctrl Pts',(-3.73563892343538,93.0301402309423,
11.5097179367768));
#275810=CARTESIAN_POINT('Ctrl Pts',(-5.19718729288481,92.9709947981446,
10.9278452452945));
#275811=CARTESIAN_POINT('Ctrl Pts',(-7.81137968310086,92.8453341046328,
9.24087349583016));
#275812=CARTESIAN_POINT('Ctrl Pts',(-8.94033127393691,92.7831736812992,
8.15360822633876));
#275813=CARTESIAN_POINT('Ctrl Pts',(-10.4099330659214,92.6840372314516,
6.05419998055747));
#275814=CARTESIAN_POINT('Ctrl Pts',(-10.8823321061612,92.6436164194797,
5.15701029741631));
#275815=CARTESIAN_POINT('Ctrl Pts',(-11.5931709912404,92.5617640622437,
3.26034040809238));
#275816=CARTESIAN_POINT('Ctrl Pts',(-11.8274267264064,92.5206565619121,
2.26792378875226));
#275817=CARTESIAN_POINT('Ctrl Pts',(-11.9338891906744,92.48046875,1.25789060919715));
#275818=CARTESIAN_POINT('Origin',(-6.57374111881153E-14,92.48046875,0.));
#275819=CARTESIAN_POINT('Ctrl Pts',(-12.0000000000001,92.80624999964,9.15933995315754E-15));
#275820=CARTESIAN_POINT('Ctrl Pts',(-12.0000000000001,92.8417057528578,
0.921621805222653));
#275821=CARTESIAN_POINT('Ctrl Pts',(-11.8938313654259,92.8784483916136,
1.84219808659633));
#275822=CARTESIAN_POINT('Ctrl Pts',(-11.318208857505,92.9799433628676,4.29338421451095));
#275823=CARTESIAN_POINT('Ctrl Pts',(-10.6493327544983,93.0445577132886,
5.7556112031982));
#275824=CARTESIAN_POINT('Ctrl Pts',(-8.80169039827924,93.165673838157,8.30351697017158));
#275825=CARTESIAN_POINT('Ctrl Pts',(-7.65266103423919,93.2286729874806,
9.37313682937302));
#275826=CARTESIAN_POINT('Ctrl Pts',(-5.01001216616424,93.3541810897256,
11.0145238390819));
#275827=CARTESIAN_POINT('Ctrl Pts',(-3.54148403116243,93.4129939613117,
11.5705616108616));
#275828=CARTESIAN_POINT('Ctrl Pts',(-0.451643875509239,93.5379806211025,
12.0949290217605));
#275829=CARTESIAN_POINT('Ctrl Pts',(1.14142505877038,93.6024216131544,12.0494200828072));
#275830=CARTESIAN_POINT('Ctrl Pts',(4.18767675127626,93.7256450825729,11.3514703820219));
#275831=CARTESIAN_POINT('Ctrl Pts',(5.61447034546205,93.7851561667958,10.7177546608328));
#275832=CARTESIAN_POINT('Ctrl Pts',(8.17091909548136,93.9113660883478,8.92820590750656));
#275833=CARTESIAN_POINT('Ctrl Pts',(9.27013306719489,93.9727901849844,7.78082540002013));
#275834=CARTESIAN_POINT('Ctrl Pts',(10.9581556951928,94.0956813091259,5.1349174614681));
#275835=CARTESIAN_POINT('Ctrl Pts',(11.5336481270458,94.1594708447873,3.66378816360723));
#275836=CARTESIAN_POINT('Ctrl Pts',(12.0846225089599,94.2842356801235,0.599726400558802));
#275837=CARTESIAN_POINT('Ctrl Pts',(12.0611102430209,94.3425338274646,-0.963002346951906));
#275838=CARTESIAN_POINT('Ctrl Pts',(11.4133145370304,94.4687101029181,-4.03229333032655));
#275839=CARTESIAN_POINT('Ctrl Pts',(10.7799275253742,94.5333243696182,-5.50604924758921));
#275840=CARTESIAN_POINT('Ctrl Pts',(8.99681676547324,94.6550618151086,-8.09107294585621));
#275841=CARTESIAN_POINT('Ctrl Pts',(7.87614575620454,94.7169000396803,-9.18558476524078));
#275842=CARTESIAN_POINT('Ctrl Pts',(5.27372199527324,94.8426210955086,-10.8912933911025));
#275843=CARTESIAN_POINT('Ctrl Pts',(3.8150761730276,94.9019269266909,-11.4837995702507));
#275844=CARTESIAN_POINT('Ctrl Pts',(0.738100769421628,95.02639319633,-12.0803427809247));
#275845=CARTESIAN_POINT('Ctrl Pts',(-0.851733171522372,95.0907033301526,
-12.0728637452725));
#275846=CARTESIAN_POINT('Ctrl Pts',(-3.90985616165455,95.2144070036474,
-11.4500627845247));
#275847=CARTESIAN_POINT('Ctrl Pts',(-5.35116761717258,95.2733585740668,
-10.8515384694098));
#275848=CARTESIAN_POINT('Ctrl Pts',(-7.95557556476879,95.3997173981778,
-9.12173727191776));
#275849=CARTESIAN_POINT('Ctrl Pts',(-9.08633141264699,95.4622159086525,
-7.99596787439197));
#275850=CARTESIAN_POINT('Ctrl Pts',(-10.8359666341656,95.5844581215649,
-5.38694660416549));
#275851=CARTESIAN_POINT('Ctrl Pts',(-11.4441438879658,95.647994145039,-3.93302693695522));
#275852=CARTESIAN_POINT('Ctrl Pts',(-11.9189061176973,95.7432696367485,
-1.61073583043876));
#275853=CARTESIAN_POINT('Ctrl Pts',(-12.0000000000001,95.7752626448447,
-0.805472152264365));
#275854=CARTESIAN_POINT('Ctrl Pts',(-12.0000000000001,95.806249999628,-2.38697950294409E-14));
#275855=CARTESIAN_POINT('Origin',(-8.79029313101884E-14,130.96875,0.));
#275856=CARTESIAN_POINT('',(-12.0000000000001,98.806249999616,-2.88584518969965E-15));
#275857=CARTESIAN_POINT('',(-12.0000000000001,98.431249999616,6.19234238727939E-14));
#275858=CARTESIAN_POINT('',(-12.0000000000001,130.96875,-1.46957615897682E-15));
#275859=CARTESIAN_POINT('Ctrl Pts',(-12.0000000000001,98.431249999616,-3.44169137633799E-14));
#275860=CARTESIAN_POINT('Ctrl Pts',(-12.0000000000001,98.3903362637419,
-1.06349429056132));
#275861=CARTESIAN_POINT('Ctrl Pts',(-11.858626067169,98.3477542696158,-2.12441740297027));
#275862=CARTESIAN_POINT('Ctrl Pts',(-11.1699243170239,98.2419053899608,
-4.65203550545811));
#275863=CARTESIAN_POINT('Ctrl Pts',(-10.475302824406,98.1800666739711,-6.05608851369005));
#275864=CARTESIAN_POINT('Ctrl Pts',(-8.56783571805061,98.0583295023047,
-8.55076676634347));
#275865=CARTESIAN_POINT('Ctrl Pts',(-7.36194773443014,97.9937152278146,
-9.6085830985033));
#275866=CARTESIAN_POINT('Ctrl Pts',(-4.64307379929293,97.867538776801,-11.1731650433297));
#275867=CARTESIAN_POINT('Ctrl Pts',(-3.16410215805437,97.8092406205087,
-11.6784514411006));
#275868=CARTESIAN_POINT('Ctrl Pts',(-0.0797494407164467,97.6844759322606,
-12.1013233929251));
#275869=CARTESIAN_POINT('Ctrl Pts',(1.49721720145038,97.620686291607,-12.0086177058656));
#275870=CARTESIAN_POINT('Ctrl Pts',(4.53525976859494,97.4977948882848,-11.2208743559025));
#275871=CARTESIAN_POINT('Ctrl Pts',(5.96616398510963,97.4363712324694,-10.5300360074582));
#275872=CARTESIAN_POINT('Ctrl Pts',(8.45813053307474,97.3101613807666,-8.6517380547846));
#275873=CARTESIAN_POINT('Ctrl Pts',(9.50174622702573,97.2506500121776,-7.49061654751233));
#275874=CARTESIAN_POINT('Ctrl Pts',(11.1069091342363,97.1274267637706,-4.80915275641748));
#275875=CARTESIAN_POINT('Ctrl Pts',(11.6424924087258,97.0629857220061,-3.30812121405916));
#275876=CARTESIAN_POINT('Ctrl Pts',(12.0986344003864,96.9379988418735,-0.2074748013541));
#275877=CARTESIAN_POINT('Ctrl Pts',(12.0236277365977,96.8791861509043,1.36100270980834));
#275878=CARTESIAN_POINT('Ctrl Pts',(11.2792316172137,96.7536781456885,4.38153558319533));
#275879=CARTESIAN_POINT('Ctrl Pts',(10.617046518114,96.69067845295,5.80486658217108));
#275880=CARTESIAN_POINT('Ctrl Pts',(8.76482133190042,96.5695626085286,8.34944672988));
#275881=CARTESIAN_POINT('Ctrl Pts',(7.58086464519092,96.5049482655075,9.43745178491119));
#275882=CARTESIAN_POINT('Ctrl Pts',(4.89611881243507,96.3784052508018,11.0644241478338));
#275883=CARTESIAN_POINT('Ctrl Pts',(3.43039307442459,96.3200123143542,11.6028404232851));
#275884=CARTESIAN_POINT('Ctrl Pts',(0.354478117635857,96.19558894069,12.0968472765385));
#275885=CARTESIAN_POINT('Ctrl Pts',(-1.22777108824699,96.1315856158455,
12.0396035186058));
#275886=CARTESIAN_POINT('Ctrl Pts',(-4.2804515265945,96.0081020981951,11.3197518587139));
#275887=CARTESIAN_POINT('Ctrl Pts',(-5.72148749750293,95.9475666604573,
10.6641304978391));
#275888=CARTESIAN_POINT('Ctrl Pts',(-8.25336177812795,95.821517205652,8.84750687802869));
#275889=CARTESIAN_POINT('Ctrl Pts',(-9.32467774413927,95.7613095515572,
7.71016305346253));
#275890=CARTESIAN_POINT('Ctrl Pts',(-10.994220774471,95.6385858189331,5.06260183372988));
#275891=CARTESIAN_POINT('Ctrl Pts',(-11.5651597717373,95.5740532770615,
3.57067964711787));
#275892=CARTESIAN_POINT('Ctrl Pts',(-11.9434861476433,95.4837054996373,
1.34514354656573));
#275893=CARTESIAN_POINT('Ctrl Pts',(-12.0000000000001,95.4571183235931,
0.672410237188394));
#275894=CARTESIAN_POINT('Ctrl Pts',(-12.0000000000001,95.431249999628,8.88178419700125E-15));
#275895=CARTESIAN_POINT('Ctrl Pts',(-12.0000000000001,95.806249999628,-6.78623823802127E-14));
#275896=CARTESIAN_POINT('Ctrl Pts',(-12.0000000000001,95.8346404553987,
0.737969461197185));
#275897=CARTESIAN_POINT('Ctrl Pts',(-11.9319288660828,95.8638859980307,
1.47604803529853));
#275898=CARTESIAN_POINT('Ctrl Pts',(-11.5045591024659,95.9571893719954,
3.76247549562259));
#275899=CARTESIAN_POINT('Ctrl Pts',(-10.9077188258606,96.021768297912,5.24718753360586));
#275900=CARTESIAN_POINT('Ctrl Pts',(-9.19105849417976,96.1440992565816,
7.8692298145771));
#275901=CARTESIAN_POINT('Ctrl Pts',(-8.09934644811893,96.2049203555293,
8.98894674875177));
#275902=CARTESIAN_POINT('Ctrl Pts',(-5.53823235938179,96.3308406503862,
10.7598929530529));
#275903=CARTESIAN_POINT('Ctrl Pts',(-4.08985281277005,96.3908119781246,
11.3894873386763));
#275904=CARTESIAN_POINT('Ctrl Pts',(-1.02684768862722,96.5147131380885,
12.0587411242401));
#275905=CARTESIAN_POINT('Ctrl Pts',(0.558827698358478,96.5788550548699,
12.0894709642923));
#275906=CARTESIAN_POINT('Ctrl Pts',(3.62782455931501,96.7029985856793,11.5425525780104));
#275907=CARTESIAN_POINT('Ctrl Pts',(5.0835892948793,96.7615602696415,10.979467360577));
#275908=CARTESIAN_POINT('Ctrl Pts',(7.73583477131505,96.88804916169,9.31003841198302));
#275909=CARTESIAN_POINT('Ctrl Pts',(8.89815879494356,96.9517749723513,8.20622415256473));
#275910=CARTESIAN_POINT('Ctrl Pts',(10.7086824081936,97.0733336918042,5.63475315906449));
#275911=CARTESIAN_POINT('Ctrl Pts',(11.3488925173778,97.1365847129197,4.19864982787631));
#275912=CARTESIAN_POINT('Ctrl Pts',(12.0437715610302,97.2619262188028,1.16635579429267));
#275913=CARTESIAN_POINT('Ctrl Pts',(12.0934795422874,97.3204991868119,-0.40076067034903));
#275914=CARTESIAN_POINT('Ctrl Pts',(11.588393733587,97.4458152708407,-3.49406145928547));
#275915=CARTESIAN_POINT('Ctrl Pts',(11.0277840731536,97.5103244286932,-4.98873201661399));
#275916=CARTESIAN_POINT('Ctrl Pts',(9.37704085620864,97.6331984422303,-7.64630800428874));
#275917=CARTESIAN_POINT('Ctrl Pts',(8.31383312200354,97.693185951036,-8.79063100717509));
#275918=CARTESIAN_POINT('Ctrl Pts',(5.79361671391148,97.8192841593186,-10.6253508095566));
#275919=CARTESIAN_POINT('Ctrl Pts',(4.35552718395247,97.8800652240558,-11.2912965327819));
#275920=CARTESIAN_POINT('Ctrl Pts',(1.30705920366105,98.0033783441985,-12.0311201834856));
#275921=CARTESIAN_POINT('Ctrl Pts',(-0.273717490831138,98.067322104706,
-12.0988102824553));
#275922=CARTESIAN_POINT('Ctrl Pts',(-3.35221551586651,98.1918499656757,
-11.6257129109516));
#275923=CARTESIAN_POINT('Ctrl Pts',(-4.82185190647142,98.2501993887458,
-11.0970382348483));
#275924=CARTESIAN_POINT('Ctrl Pts',(-7.51674502260938,98.3766381746483,
-9.48841611527849));
#275925=CARTESIAN_POINT('Ctrl Pts',(-8.70724253525681,98.4412560350765,
-8.40926579798738));
#275926=CARTESIAN_POINT('Ctrl Pts',(-10.575840211191,98.5625593777037,-5.87933455790365));
#275927=CARTESIAN_POINT('Ctrl Pts',(-11.2476213291911,98.6251994919137,
-4.46168742808438));
#275928=CARTESIAN_POINT('Ctrl Pts',(-11.8763701518246,98.7282508017786,
-1.98730828071283));
#275929=CARTESIAN_POINT('Ctrl Pts',(-12.0000000000001,98.7679896997974,
-0.994521999591797));
#275930=CARTESIAN_POINT('Ctrl Pts',(-12.0000000000001,98.806249999616,1.22124532708767E-14));
#275931=CARTESIAN_POINT('Origin',(-8.79029313101884E-14,130.96875,0.));
#275932=CARTESIAN_POINT('',(-12.0000000000001,101.806249999604,1.21771383793994E-13));
#275933=CARTESIAN_POINT('',(-12.0000000000001,101.431249999604,9.59933929409784E-14));
#275934=CARTESIAN_POINT('',(-12.0000000000001,130.96875,-1.46957615897682E-15));
#275935=CARTESIAN_POINT('Ctrl Pts',(-12.0000000000001,101.431249999604,
4.35484981409218E-13));
#275936=CARTESIAN_POINT('Ctrl Pts',(-12.0000000000001,101.382732225158,
-1.26115044279506));
#275937=CARTESIAN_POINT('Ctrl Pts',(-11.8011858555912,101.3319584443,-2.51634392763927));
#275938=CARTESIAN_POINT('Ctrl Pts',(-10.9295576026251,101.218191084799,
-5.19035521167642));
#275939=CARTESIAN_POINT('Ctrl Pts',(-10.1698051033365,101.158203246843,
-6.55514968186482));
#275940=CARTESIAN_POINT('Ctrl Pts',(-8.15243145592084,101.03532946252,-8.94635876935562));
#275941=CARTESIAN_POINT('Ctrl Pts',(-6.90416210454257,100.970820266432,
-9.94142271432126));
#275942=CARTESIAN_POINT('Ctrl Pts',(-4.11835256299701,100.845503978089,
-11.3776985584927));
#275943=CARTESIAN_POINT('Ctrl Pts',(-2.61258144852507,100.786931139159,
-11.8147041098655));
#275944=CARTESIAN_POINT('Ctrl Pts',(0.48602831587838,100.661589741242,-12.090897530964));
#275945=CARTESIAN_POINT('Ctrl Pts',(2.04968283481498,100.598338587285,-11.9258176747727));
#275946=CARTESIAN_POINT('Ctrl Pts',(5.05478730302487,100.476779558053,-10.9985662576491));
#275947=CARTESIAN_POINT('Ctrl Pts',(6.46375991644632,100.413054323408,-10.2342440890019));
#275948=CARTESIAN_POINT('Ctrl Pts',(8.87108911775026,100.286565484546,-8.22771904423435));
#275949=CARTESIAN_POINT('Ctrl Pts',(9.85648401275463,100.228003666168,-7.01721833210744));
#275950=CARTESIAN_POINT('Ctrl Pts',(11.3250371392221,100.103860320699,-4.26745071991765));
#275951=CARTESIAN_POINT('Ctrl Pts',(11.785828698054,100.039718321178,-2.74989105323262));
#275952=CARTESIAN_POINT('Ctrl Pts',(12.0958838319189,99.9158169013089,0.370006863414581));
#275953=CARTESIAN_POINT('Ctrl Pts',(11.9446950421818,99.8558459067457,1.94205232576911));
#275954=CARTESIAN_POINT('Ctrl Pts',(11.0518862428444,99.7299256967796,4.92507767164746));
#275955=CARTESIAN_POINT('Ctrl Pts',(10.324344397283,99.6691041815619,6.30937792967838));
#275956=CARTESIAN_POINT('Ctrl Pts',(8.3611359667578,99.5467734787521,8.75229785457037));
#275957=CARTESIAN_POINT('Ctrl Pts',(7.13353424042131,99.4821945290531,9.77874207649069));
#275958=CARTESIAN_POINT('Ctrl Pts',(4.38054731532025,99.3564319089459,11.2789664160656));
#275959=CARTESIAN_POINT('Ctrl Pts',(2.88805958243837,99.2980744637605,11.7500374076434));
#275960=CARTESIAN_POINT('Ctrl Pts',(-0.203968503235057,99.1729993003413,
12.0994021381704));
#275961=CARTESIAN_POINT('Ctrl Pts',(-1.7746683838583,99.1094631555172,11.9702933860124));
#275962=CARTESIAN_POINT('Ctrl Pts',(-4.79666950094096,98.9872206424807,
11.1125547405502));
#275963=CARTESIAN_POINT('Ctrl Pts',(-6.21676753370284,98.9247226506023,
10.3850404492276));
#275964=CARTESIAN_POINT('Ctrl Pts',(-8.66673161054512,98.7983638894037,
8.4426681463036));
#275965=CARTESIAN_POINT('Ctrl Pts',(-9.68136490617877,98.7394121048799,
7.25686480030045));
#275966=CARTESIAN_POINT('Ctrl Pts',(-11.21872656147,98.6157086387229,4.54088847059025));
#275967=CARTESIAN_POINT('Ctrl Pts',(-11.717142100468,98.5513984376063,3.03118141519292));
#275968=CARTESIAN_POINT('Ctrl Pts',(-11.9700060674013,98.4693355863612,
0.980234962623068));
#275969=CARTESIAN_POINT('Ctrl Pts',(-12.0000000000001,98.4500953949073,
0.489859209079169));
#275970=CARTESIAN_POINT('Ctrl Pts',(-12.0000000000001,98.431249999616,-6.66133814775094E-15));
#275971=CARTESIAN_POINT('Ctrl Pts',(-12.0000000000001,98.806249999616,1.38777878078145E-16));
#275972=CARTESIAN_POINT('Ctrl Pts',(-12.0000000000001,98.8276233756076,
0.555570466773574));
#275973=CARTESIAN_POINT('Ctrl Pts',(-11.9614195863975,98.849498410001,1.11164529292389));
#275974=CARTESIAN_POINT('Ctrl Pts',(-11.6652978475081,98.9345505045725,
3.22623756605706));
#275975=CARTESIAN_POINT('Ctrl Pts',(-11.1407172499593,98.9989564945593,
4.72993297382568));
#275976=CARTESIAN_POINT('Ctrl Pts',(-9.55561030902574,99.1223266653623,
7.42173238181464));
#275977=CARTESIAN_POINT('Ctrl Pts',(-8.52058700319381,99.181654125327,8.5901921471054));
#275978=CARTESIAN_POINT('Ctrl Pts',(-6.04104625614187,99.3079101631137,
10.4875352643976));
#275979=CARTESIAN_POINT('Ctrl Pts',(-4.61332333281783,99.369637150774,11.1892657235087));
#275980=CARTESIAN_POINT('Ctrl Pts',(-1.57996080837295,99.4923392423923,
11.9978723487919));
#275981=CARTESIAN_POINT('Ctrl Pts',(-0.00477503949806751,99.5560568452079,
12.1014463532335));
#275982=CARTESIAN_POINT('Ctrl Pts',(3.08197465134809,99.6809184930712,11.700466524053));
#275983=CARTESIAN_POINT('Ctrl Pts',(4.56498990025355,99.739217703611,11.2053710962917));
#275984=CARTESIAN_POINT('Ctrl Pts',(7.29414460370894,99.8652745822897,9.65996844683288));
#275985=CARTESIAN_POINT('Ctrl Pts',(8.50659980384892,99.9298820381286,8.61147789493034));
#275986=CARTESIAN_POINT('Ctrl Pts',(10.4308090856514,100.051801075647,6.13219426693295));
#275987=CARTESIAN_POINT('Ctrl Pts',(11.1352964859028,100.113317690063,4.73404138995748));
#275988=CARTESIAN_POINT('Ctrl Pts',(11.9717301606602,100.23850541014,1.75173868711237));
#275989=CARTESIAN_POINT('Ctrl Pts',(12.0976219836414,100.297482843836,0.196170422008661));
#275990=CARTESIAN_POINT('Ctrl Pts',(11.7489890472703,100.421161649931,-2.90540627876741));
#275991=CARTESIAN_POINT('Ctrl Pts',(11.2667093682072,100.485479782146,-4.42056235048717));
#275992=CARTESIAN_POINT('Ctrl Pts',(9.75201543617218,100.60997523142,-7.16449034304141));
#275993=CARTESIAN_POINT('Ctrl Pts',(8.73947898856186,100.669250142572,-8.3697783466813));
#275994=CARTESIAN_POINT('Ctrl Pts',(6.31570132789617,100.794960060076,-10.320903774));
#275995=CARTESIAN_POINT('Ctrl Pts',(4.92925879702124,100.856857292785,-11.0503875663945));
#275996=CARTESIAN_POINT('Ctrl Pts',(1.92055461475842,100.978561933509,-11.9513820703781));
#275997=CARTESIAN_POINT('Ctrl Pts',(0.323180305856766,101.043177081623,
-12.1003857993283));
#275998=CARTESIAN_POINT('Ctrl Pts',(-2.79658640397,101.169374295959,-11.7718550594554));
#275999=CARTESIAN_POINT('Ctrl Pts',(-4.29057784217851,101.227673735964,
-11.3131971364897));
#276000=CARTESIAN_POINT('Ctrl Pts',(-7.03634923360482,101.352420926947,
-9.84574888144511));
#276001=CARTESIAN_POINT('Ctrl Pts',(-8.25902714011372,101.416222968348,
-8.84520319199907));
#276002=CARTESIAN_POINT('Ctrl Pts',(-10.2566560747344,101.539147416662,
-6.42468698789539));
#276003=CARTESIAN_POINT('Ctrl Pts',(-11.0097963852458,101.600519033734,
-5.02594677720654));
#276004=CARTESIAN_POINT('Ctrl Pts',(-11.8224652873435,101.712515064644,
-2.37882160259375));
#276005=CARTESIAN_POINT('Ctrl Pts',(-12.0000000000001,101.760401871696,
-1.19175678342724));
#276006=CARTESIAN_POINT('Ctrl Pts',(-12.0000000000001,101.806249999604,
4.51583215266282E-13));
#276007=CARTESIAN_POINT('Origin',(-8.79029313101884E-14,130.96875,0.));
#276008=CARTESIAN_POINT('',(-12.0000000000001,104.806249999592,9.27456637689777E-15));
#276009=CARTESIAN_POINT('',(-12.0000000000001,104.431249999592,6.316403021549E-16));
#276010=CARTESIAN_POINT('',(-12.0000000000001,130.96875,-1.46957615897682E-15));
#276011=CARTESIAN_POINT('Ctrl Pts',(-12.0000000000001,104.431249999592,
-1.60982338570648E-14));
#276012=CARTESIAN_POINT('Ctrl Pts',(-12.0000000000001,104.3754124827,-1.45141672215856));
#276013=CARTESIAN_POINT('Ctrl Pts',(-11.7366682504109,104.316709487413,
-2.8917558018116));
#276014=CARTESIAN_POINT('Ctrl Pts',(-10.6694625868215,104.194978937878,
-5.70921191596897));
#276015=CARTESIAN_POINT('Ctrl Pts',(-9.83791481246829,104.135668144137,
-7.04613425402326));
#276016=CARTESIAN_POINT('Ctrl Pts',(-7.6996867104163,104.011206526125,-9.3377833408248));
#276017=CARTESIAN_POINT('Ctrl Pts',(-6.40930566327384,103.946897674067,
-10.2664593419611));
#276018=CARTESIAN_POINT('Ctrl Pts',(-3.56946054311442,103.823190057369,
-11.560703293972));
#276019=CARTESIAN_POINT('Ctrl Pts',(-2.0516887747929,103.764242553893,-11.923986377946));
#276020=CARTESIAN_POINT('Ctrl Pts',(1.07210272081072,103.637882533553,-12.056038083896));
#276021=CARTESIAN_POINT('Ctrl Pts',(2.64872314137544,103.57537415047,-11.810223102415));
#276022=CARTESIAN_POINT('Ctrl Pts',(5.59798914903062,103.453137648988,-10.7284569647133));
#276023=CARTESIAN_POINT('Ctrl Pts',(6.94474352371526,103.389603935508,-9.9099733497718));
#276024=CARTESIAN_POINT('Ctrl Pts',(9.24133620388024,103.264526173037,-7.81038030019616));
#276025=CARTESIAN_POINT('Ctrl Pts',(10.1721743389527,103.206167475913,-6.55219167295185));
#276026=CARTESIAN_POINT('Ctrl Pts',(11.5181621169873,103.080408738882,-3.72061036212782));
#276027=CARTESIAN_POINT('Ctrl Pts',(11.9083049834493,103.015830266773,-2.16875006051643));
#276028=CARTESIAN_POINT('Ctrl Pts',(12.0613369283081,102.893494442124,0.961472365135507));
#276029=CARTESIAN_POINT('Ctrl Pts',(11.8366010142436,102.832681255944,2.50906255089275));
#276030=CARTESIAN_POINT('Ctrl Pts',(10.8061620462178,102.706759346794,5.44741331201057));
#276031=CARTESIAN_POINT('Ctrl Pts',(10.0047208534933,102.64678167457,6.80830477624646));
#276032=CARTESIAN_POINT('Ctrl Pts',(7.92053483803228,102.522885460395,9.15055638290675));
#276033=CARTESIAN_POINT('Ctrl Pts',(6.65597983170444,102.458745118947,10.1076915780615));
#276034=CARTESIAN_POINT('Ctrl Pts',(3.85194512226161,102.334598064039,11.4697064390822));
#276035=CARTESIAN_POINT('Ctrl Pts',(2.34331124432273,102.276038930589,11.8701513059845));
#276036=CARTESIAN_POINT('Ctrl Pts',(-0.783691128516117,102.149549027536,
12.0791548994081));
#276037=CARTESIAN_POINT('Ctrl Pts',(-2.37294220292942,102.085812253944,
11.8696540642989));
#276038=CARTESIAN_POINT('Ctrl Pts',(-5.34938384061895,101.964259428575,
10.8540463567392));
#276039=CARTESIAN_POINT('Ctrl Pts',(-6.71157120332194,101.901010935596,
10.0688003707522));
#276040=CARTESIAN_POINT('Ctrl Pts',(-9.05647978478012,101.775667377541,
8.02452949354289));
#276041=CARTESIAN_POINT('Ctrl Pts',(-10.0180799873236,101.717091948471,
6.78608948726545));
#276042=CARTESIAN_POINT('Ctrl Pts',(-11.4220280949518,101.592327134818,
3.99917625171409));
#276043=CARTESIAN_POINT('Ctrl Pts',(-11.846153848979,101.528383280513,2.4748536455238));
#276044=CARTESIAN_POINT('Ctrl Pts',(-11.9884536108764,101.454792207264,
0.608194507680637));
#276045=CARTESIAN_POINT('Ctrl Pts',(-12.0000000000001,101.442942496614,
0.303929806132952));
#276046=CARTESIAN_POINT('Ctrl Pts',(-12.0000000000001,101.431249999604,
4.79130624064794E-13));
#276047=CARTESIAN_POINT('Ctrl Pts',(-12.0000000000001,101.806249999604,
4.41591208044656E-13));
#276048=CARTESIAN_POINT('Ctrl Pts',(-12.0000000000001,101.819718521391,
0.350095040632927));
#276049=CARTESIAN_POINT('Ctrl Pts',(-11.9846796226145,101.833393558327,
0.700580256045129));
#276050=CARTESIAN_POINT('Ctrl Pts',(-11.8157459659036,101.909462883929,
2.62300415699322));
#276051=CARTESIAN_POINT('Ctrl Pts',(-11.3686032455459,101.973909767947,
4.15292363840108));
#276052=CARTESIAN_POINT('Ctrl Pts',(-9.91849965274548,102.098922706532,
6.9312897019481));
#276053=CARTESIAN_POINT('Ctrl Pts',(-8.93753485777631,102.157714218484,
8.15719532852502));
#276054=CARTESIAN_POINT('Ctrl Pts',(-6.56255730271517,102.283203504547,
10.1662089139473));
#276055=CARTESIAN_POINT('Ctrl Pts',(-5.19104211732635,102.346255274138,
10.930342364952));
#276056=CARTESIAN_POINT('Ctrl Pts',(-2.19787636457957,102.467356960704,
11.9039570865563));
#276057=CARTESIAN_POINT('Ctrl Pts',(-0.600720123462492,102.531950360164,
12.0902774525815));
#276058=CARTESIAN_POINT('Ctrl Pts',(2.5280641425565,102.658512342311,11.83225172001));
#276059=CARTESIAN_POINT('Ctrl Pts',(4.03079793476824,102.716914572037,11.4081549457105));
#276060=CARTESIAN_POINT('Ctrl Pts',(6.81147777948937,102.841318626694,10.0031858500243));
#276061=CARTESIAN_POINT('Ctrl Pts',(8.05922212204603,102.905332462921,9.02823337963791));
#276062=CARTESIAN_POINT('Ctrl Pts',(10.1085155120594,103.028846556572,6.65402760599244));
#276063=CARTESIAN_POINT('Ctrl Pts',(10.8905026907458,103.089338828686,5.27779941230339));
#276064=CARTESIAN_POINT('Ctrl Pts',(11.8746799498332,103.215379301704,2.32133541188133));
#276065=CARTESIAN_POINT('Ctrl Pts',(12.0748094649417,103.275628241651,0.771661914612208));
#276066=CARTESIAN_POINT('Ctrl Pts',(11.8731200331309,103.398324418499,-2.35211757732449));
#276067=CARTESIAN_POINT('Ctrl Pts',(11.4598969894638,103.462860891733,-3.89538697384107));
#276068=CARTESIAN_POINT('Ctrl Pts',(10.0718393722471,103.588331234776,-6.70580257434195));
#276069=CARTESIAN_POINT('Ctrl Pts',(9.12085643168401,103.646814276566,-7.95108074182539));
#276070=CARTESIAN_POINT('Ctrl Pts',(6.79254880140641,103.772070823266,-10.0145413019603));
#276071=CARTESIAN_POINT('Ctrl Pts',(5.43560345393382,103.835421547407,-10.8113019911486));
#276072=CARTESIAN_POINT('Ctrl Pts',(2.46845787887802,103.957214899215,-11.8498208098566));
#276073=CARTESIAN_POINT('Ctrl Pts',(0.883557038940081,104.020509366595,
-12.0719252313962));
#276074=CARTESIAN_POINT('Ctrl Pts',(-2.24238830252252,104.146956511831,
-11.889607902365));
#276075=CARTESIAN_POINT('Ctrl Pts',(-3.75420805423453,104.20563067194,-11.5020454222977));
#276076=CARTESIAN_POINT('Ctrl Pts',(-6.57077945978205,104.329630283488,
-10.1634870880653));
#276077=CARTESIAN_POINT('Ctrl Pts',(-7.84436963905717,104.39383322516,-9.21615487078874));
#276078=CARTESIAN_POINT('Ctrl Pts',(-9.94739883655799,104.517930272847,
-6.89139192513552));
#276079=CARTESIAN_POINT('Ctrl Pts',(-10.7593396456813,104.577657251294,
-5.53882792160448));
#276080=CARTESIAN_POINT('Ctrl Pts',(-11.759913674213,104.696968996814,-2.76259524211232));
#276081=CARTESIAN_POINT('Ctrl Pts',(-12.0000000000001,104.752933891441,
-1.38587629317705));
#276082=CARTESIAN_POINT('Ctrl Pts',(-12.0000000000001,104.806249999592,
3.52495810318487E-14));
#276083=CARTESIAN_POINT('Origin',(-8.79029313101884E-14,130.96875,0.));
#276084=CARTESIAN_POINT('',(-12.0000000000001,107.80624999958,-1.42867746987913E-15));
#276085=CARTESIAN_POINT('',(-12.0000000000001,107.43124999958,6.31640302154899E-16));
#276086=CARTESIAN_POINT('',(-12.0000000000001,130.96875,-1.46957615897682E-15));
#276087=CARTESIAN_POINT('',(11.8516579398691,109.38046875,-1.8810114503466));
#276088=CARTESIAN_POINT('Ctrl Pts',(-12.0000000000001,107.80624999958,-2.22044604925031E-15));
#276089=CARTESIAN_POINT('Ctrl Pts',(-12.0000000000001,107.866343814516,
1.56205312755359));
#276090=CARTESIAN_POINT('Ctrl Pts',(-11.6949938433683,107.92969090644,3.10956804902835));
#276091=CARTESIAN_POINT('Ctrl Pts',(-10.5145746762546,108.055118102493,
5.98632792710984));
#276092=CARTESIAN_POINT('Ctrl Pts',(-9.65626038750239,108.113582953069,
7.29034181478346));
#276093=CARTESIAN_POINT('Ctrl Pts',(-7.47603641389864,108.237872369909,
9.51694602212484));
#276094=CARTESIAN_POINT('Ctrl Pts',(-6.16853086833224,108.301945582296,
10.4121415247227));
#276095=CARTESIAN_POINT('Ctrl Pts',(-3.28613682807818,108.42563556719,11.6470803453935));
#276096=CARTESIAN_POINT('Ctrl Pts',(-1.73951548877978,108.485885119957,
11.9761130077834));
#276097=CARTESIAN_POINT('Ctrl Pts',(1.37506378162063,108.611872497961,12.021126122061));
#276098=CARTESIAN_POINT('Ctrl Pts',(2.91330421762905,108.672369841524,11.7435408531582));
#276099=CARTESIAN_POINT('Ctrl Pts',(5.83156931012537,108.794903894772,10.6065910386354));
#276100=CARTESIAN_POINT('Ctrl Pts',(7.17862656088049,108.859461370049,9.74546642258997));
#276101=CARTESIAN_POINT('Ctrl Pts',(9.4377057368,108.985065275805,7.57211167244003));
#276102=CARTESIAN_POINT('Ctrl Pts',(10.3366228846815,109.043483264628,6.28978302888967));
#276103=CARTESIAN_POINT('Ctrl Pts',(11.4376342634708,109.152590405637,3.81143858254238));
#276104=CARTESIAN_POINT('Ctrl Pts',(11.7524514429401,109.199737369538,2.68821070974933));
#276105=CARTESIAN_POINT('Ctrl Pts',(12.0478585774647,109.291407362996,0.401363391909027));
#276106=CARTESIAN_POINT('Ctrl Pts',(12.0312037663556,109.334703618332,-0.749750011370815));
#276107=CARTESIAN_POINT('Ctrl Pts',(11.8516579398691,109.38046875,-1.88101145034674));
#276108=CARTESIAN_POINT('',(7.06903888345947,109.38046875,-9.696839137788));
#276109=CARTESIAN_POINT('Origin',(-7.54701734185159E-14,109.38046875,0.));
#276110=CARTESIAN_POINT('Ctrl Pts',(7.06903888345945,109.38046875,-9.69683913778803));
#276111=CARTESIAN_POINT('Ctrl Pts',(8.02804380632041,109.332462367855,-8.99772028134388));
#276112=CARTESIAN_POINT('Ctrl Pts',(8.8780784676924,109.28473067987,-8.16016994838996));
#276113=CARTESIAN_POINT('Ctrl Pts',(10.3026613015982,109.193061552059,-6.26547500429061));
#276114=CARTESIAN_POINT('Ctrl Pts',(10.8701502580611,109.14616524121,-5.21930516734868));
#276115=CARTESIAN_POINT('Ctrl Pts',(11.8155022909111,109.034502891345,-2.62396491876396));
#276116=CARTESIAN_POINT('Ctrl Pts',(12.0578170407519,108.972322229049,-1.04882821065039));
#276117=CARTESIAN_POINT('Ctrl Pts',(11.9196530803474,108.849893935341,2.08862871745094));
#276118=CARTESIAN_POINT('Ctrl Pts',(11.5468169083728,108.786283367778,3.620953004917));
#276119=CARTESIAN_POINT('Ctrl Pts',(10.240088817047,108.661290939061,6.44537146805403));
#276120=CARTESIAN_POINT('Ctrl Pts',(9.32291011631986,108.602966100172,7.71268965593937));
#276121=CARTESIAN_POINT('Ctrl Pts',(7.03115871052508,108.477083897142,9.85277970239431));
#276122=CARTESIAN_POINT('Ctrl Pts',(5.66907121068656,108.412491483342,10.6946864168547));
#276123=CARTESIAN_POINT('Ctrl Pts',(2.73001709375482,108.290322327293,11.7876755691295));
#276124=CARTESIAN_POINT('Ctrl Pts',(1.18622866805082,108.22923395716,12.0414055389981));
#276125=CARTESIAN_POINT('Ctrl Pts',(-1.92536059284584,108.103367527582,
11.9472136780264));
#276126=CARTESIAN_POINT('Ctrl Pts',(-3.46344019184888,108.043598548278,
11.5951511074519));
#276127=CARTESIAN_POINT('Ctrl Pts',(-6.32617469954648,107.919535973427,
10.3174826910173));
#276128=CARTESIAN_POINT('Ctrl Pts',(-7.62184176508883,107.855343573278,
9.40098006137079));
#276129=CARTESIAN_POINT('Ctrl Pts',(-9.76845852360064,107.731318008446,
7.13921670750586));
#276130=CARTESIAN_POINT('Ctrl Pts',(-10.6061854625943,107.672665296767,
5.82236900617445));
#276131=CARTESIAN_POINT('Ctrl Pts',(-11.7190826474381,107.549629717902,
2.98583658854305));
#276132=CARTESIAN_POINT('Ctrl Pts',(-12.0000000000001,107.48892173526,1.49909462707177));
#276133=CARTESIAN_POINT('Ctrl Pts',(-12.0000000000001,107.43124999958,-4.10782519111308E-14));
#276134=CARTESIAN_POINT('Origin',(-8.79029313101884E-14,130.96875,0.));
#276135=CARTESIAN_POINT('Ctrl Pts',(-12.0000000000001,107.43124999958,2.73285676328662E-15));
#276136=CARTESIAN_POINT('Ctrl Pts',(-12.0000000000001,107.427995874985,
-0.0845863340034995));
#276137=CARTESIAN_POINT('Ctrl Pts',(-11.9991056463269,107.424729090763,
-0.169211143825749));
#276138=CARTESIAN_POINT('Ctrl Pts',(-11.964341287163,107.361088711466,-1.81215653557658));
#276139=CARTESIAN_POINT('Ctrl Pts',(-11.6280800167193,107.297755470126,
-3.34915602874002));
#276140=CARTESIAN_POINT('Ctrl Pts',(-10.3891578369817,107.172483440034,
-6.20287380756784));
#276141=CARTESIAN_POINT('Ctrl Pts',(-9.50039687721795,107.113985669083,
-7.49351280749634));
#276142=CARTESIAN_POINT('Ctrl Pts',(-7.25951074047479,106.988542511097,
-9.68514731953922));
#276143=CARTESIAN_POINT('Ctrl Pts',(-5.92088023027487,106.924010620768,
-10.5567942847113));
#276144=CARTESIAN_POINT('Ctrl Pts',(-3.01426889782003,106.801282393196,
-11.7179508024918));
#276145=CARTESIAN_POINT('Ctrl Pts',(-1.47911473022806,106.741081447252,
-12.0086858454301));
#276146=CARTESIAN_POINT('Ctrl Pts',(1.63703535302971,106.615030528534,-11.9908030836491));
#276147=CARTESIAN_POINT('Ctrl Pts',(3.18833183487053,106.554487995537,-11.674490635908));
#276148=CARTESIAN_POINT('Ctrl Pts',(6.08136829751295,106.431009484748,-10.4630941343253));
#276149=CARTESIAN_POINT('Ctrl Pts',(7.39522944879173,106.36700788638,-9.57965834995361));
#276150=CARTESIAN_POINT('Ctrl Pts',(9.59375419220535,106.242581366008,-7.37247662390832));
#276151=CARTESIAN_POINT('Ctrl Pts',(10.4633417627637,106.184189907485,-6.07552211554223));
#276152=CARTESIAN_POINT('Ctrl Pts',(11.6796006270252,106.057649939537,-3.18148234050514));
#276153=CARTESIAN_POINT('Ctrl Pts',(11.9982402648555,105.993035449527,-1.60545299752112));
#276154=CARTESIAN_POINT('Ctrl Pts',(12.0017042150108,105.871913988982,1.54180135026534));
#276155=CARTESIAN_POINT('Ctrl Pts',(11.7011401038563,105.808925175336,3.08255411229185));
#276156=CARTESIAN_POINT('Ctrl Pts',(10.5285614620387,105.683415227199,5.96401255403122));
#276157=CARTESIAN_POINT('Ctrl Pts',(9.66757293360446,105.624598912445,7.27723393041331));
#276158=CARTESIAN_POINT('Ctrl Pts',(7.47649463281433,105.499616447155,9.51804700867654));
#276159=CARTESIAN_POINT('Ctrl Pts',(6.16113181584196,105.435176402445,10.4178563181802));
#276160=CARTESIAN_POINT('Ctrl Pts',(3.28670360005198,105.311948728854,11.6443150407754));
#276161=CARTESIAN_POINT('Ctrl Pts',(1.75998898775683,105.252443049639,11.9705871715524));
#276162=CARTESIAN_POINT('Ctrl Pts',(-1.36012470385981,105.126231799595,
12.0260967757031));
#276163=CARTESIAN_POINT('Ctrl Pts',(-2.92392934879068,105.064799308801,
11.7442500892509));
#276164=CARTESIAN_POINT('Ctrl Pts',(-5.84503502917611,104.941913498483,
10.5964156377292));
#276165=CARTESIAN_POINT('Ctrl Pts',(-7.17546734499953,104.878125961916,
9.74479122052804));
#276166=CARTESIAN_POINT('Ctrl Pts',(-9.42264554811813,104.753358329308,
7.59022857154424));
#276167=CARTESIAN_POINT('Ctrl Pts',(-10.3224350204873,104.695060346315,
6.31230031409505));
#276168=CARTESIAN_POINT('Ctrl Pts',(-11.6029971251243,104.568887412855,
3.44869446711149));
#276169=CARTESIAN_POINT('Ctrl Pts',(-11.9571346890154,104.504273295728,
1.88420879207154));
#276170=CARTESIAN_POINT('Ctrl Pts',(-11.9987825322073,104.43886058118,0.197430649364387));
#276171=CARTESIAN_POINT('Ctrl Pts',(-12.0000000000001,104.435046718343,
0.0986902962678449));
#276172=CARTESIAN_POINT('Ctrl Pts',(-12.0000000000001,104.431249999592,
2.73285676328662E-15));
#276173=CARTESIAN_POINT('Ctrl Pts',(-12.0000000000001,104.806249999592,
-3.30291349825984E-14));
#276174=CARTESIAN_POINT('Ctrl Pts',(-12.0000000000001,104.812464713841,
0.161542645279967));
#276175=CARTESIAN_POINT('Ctrl Pts',(-11.9967380233314,104.818724869803,
0.323206602683525));
#276176=CARTESIAN_POINT('Ctrl Pts',(-11.9261120943596,104.886793472473,
2.06960522352684));
#276177=CARTESIAN_POINT('Ctrl Pts',(-11.54848852509,104.95138842782,3.62596174965847));
#276178=CARTESIAN_POINT('Ctrl Pts',(-10.2252760523671,105.077296051354,
6.46881329835151));
#276179=CARTESIAN_POINT('Ctrl Pts',(-9.30528386847831,105.135615489699,
7.7339192777929));
#276180=CARTESIAN_POINT('Ctrl Pts',(-7.0258812088237,105.260589638183,9.85281451307973));
#276181=CARTESIAN_POINT('Ctrl Pts',(-5.68474473736919,105.32421591025,10.6829233828083));
#276182=CARTESIAN_POINT('Ctrl Pts',(-2.74523390111701,105.446683865421,
11.7878509544643));
#276183=CARTESIAN_POINT('Ctrl Pts',(-1.17308397829313,105.508797755876,
12.0463228935084));
#276184=CARTESIAN_POINT('Ctrl Pts',(1.94947066697386,105.63510774457,11.9411368396299));
#276185=CARTESIAN_POINT('Ctrl Pts',(3.47039778126117,105.694231675528,11.5908386583477));
#276186=CARTESIAN_POINT('Ctrl Pts',(6.32249939755816,105.817775656283,10.3203466064808));
#276187=CARTESIAN_POINT('Ctrl Pts',(7.62173048099895,105.882134685304,9.40174126806386));
#276188=CARTESIAN_POINT('Ctrl Pts',(9.77861242901587,106.006783826509,7.12788005545473));
#276189=CARTESIAN_POINT('Ctrl Pts',(10.6205501364151,106.065902010767,5.79929321074988));
#276190=CARTESIAN_POINT('Ctrl Pts',(11.7475699929408,106.191551757011,2.89939796966487));
#276191=CARTESIAN_POINT('Ctrl Pts',(12.0237923310024,106.253771231836,1.35638022512553));
#276192=CARTESIAN_POINT('Ctrl Pts',(11.9723929312291,106.375299269845,-1.78586735302398));
#276193=CARTESIAN_POINT('Ctrl Pts',(11.6307531771349,106.43991740774,-3.35451832678343));
#276194=CARTESIAN_POINT('Ctrl Pts',(10.3728507076161,106.566224175867,-6.22896557707807));
#276195=CARTESIAN_POINT('Ctrl Pts',(9.48373849128698,106.624538019851,-7.51363935107693));
#276196=CARTESIAN_POINT('Ctrl Pts',(7.25369658646848,106.749189457153,-9.68690109223212));
#276197=CARTESIAN_POINT('Ctrl Pts',(5.92904573149467,106.813056369374,-10.5498214277077));
#276198=CARTESIAN_POINT('Ctrl Pts',(3.01778852767233,106.936156081398,-11.7202075268318));
#276199=CARTESIAN_POINT('Ctrl Pts',(1.45840227756446,106.997256388224,-12.0143038356566));
#276200=CARTESIAN_POINT('Ctrl Pts',(-1.66035201914284,107.123412649589,
-11.9848591271093));
#276201=CARTESIAN_POINT('Ctrl Pts',(-3.1900790292478,107.183147372144,-11.6712020474588));
#276202=CARTESIAN_POINT('Ctrl Pts',(-6.0760466845703,107.306202024025,-10.4679030324817));
#276203=CARTESIAN_POINT('Ctrl Pts',(-7.39975098695485,107.370678482113,
-9.57804330102746));
#276204=CARTESIAN_POINT('Ctrl Pts',(-9.6086165723654,107.495828889602,-7.35464892462781));
#276205=CARTESIAN_POINT('Ctrl Pts',(-10.4795187353534,107.554514780734,
-6.04946415648028));
#276206=CARTESIAN_POINT('Ctrl Pts',(-11.6757493718232,107.679940049496,
-3.17789183339809));
#276207=CARTESIAN_POINT('Ctrl Pts',(-11.989082469283,107.743082695574,-1.63839677759871));
#276208=CARTESIAN_POINT('Ctrl Pts',(-11.9999066094214,107.804145561296,
-0.054671531396247));
#276209=CARTESIAN_POINT('Ctrl Pts',(-12.0000000000001,107.805198448039,
-0.0273335845947108));
#276210=CARTESIAN_POINT('Ctrl Pts',(-12.0000000000001,107.80624999958,2.17774546598592E-15));
#276211=CARTESIAN_POINT('Origin',(-6.51327129430312E-14,91.43046875,0.));
#276212=CARTESIAN_POINT('Ctrl Pts',(-11.2291932872669,93.2512754627332,
8.5342589378412E-11));
#276213=CARTESIAN_POINT('Ctrl Pts',(-11.2847945964217,93.1956741535784,
-0.57160885882348));
#276214=CARTESIAN_POINT('Ctrl Pts',(-11.2935934610398,93.143158872129,-1.10587788332065));
#276215=CARTESIAN_POINT('Ctrl Pts',(-11.2307768438364,92.9923394153088,
-2.6300800192019));
#276216=CARTESIAN_POINT('Ctrl Pts',(-11.0476053526866,92.8890071879839,
-3.65836031572687));
#276217=CARTESIAN_POINT('Ctrl Pts',(-10.3932827518185,92.6811478925007,
-5.6915126996453));
#276218=CARTESIAN_POINT('Ctrl Pts',(-9.9151798225123,92.5816333031356,-6.66836341355856));
#276219=CARTESIAN_POINT('Ctrl Pts',(-9.30293325730102,92.4804687499998,
-7.57993620093262));
#276220=CARTESIAN_POINT('',(-13.0500000000001,91.43046875,-1.5981640728873E-15));
#276221=CARTESIAN_POINT('',(-13.0500000000001,91.43046875,-1.5981640728873E-15));
#276222=CARTESIAN_POINT('Origin',(-6.51327129430312E-14,91.43046875,0.));
#276223=CARTESIAN_POINT('Ctrl Pts',(-11.9338891906744,92.48046875,1.25789060919728));
#276224=CARTESIAN_POINT('Ctrl Pts',(-11.770923660508,92.511971325493,2.50345334854318));
#276225=CARTESIAN_POINT('Ctrl Pts',(-11.4122992544335,92.5444554192473,
3.71547200511176));
#276226=CARTESIAN_POINT('Ctrl Pts',(-10.3244245330618,92.6093697694792,
5.99501809473401));
#276227=CARTESIAN_POINT('Ctrl Pts',(-9.59484510342232,92.6404645939112,
7.05327596796796));
#276228=CARTESIAN_POINT('Ctrl Pts',(-7.6557591345177,92.7118196954419,9.06644546422308));
#276229=CARTESIAN_POINT('Ctrl Pts',(-6.39836926084137,92.7519983328108,
9.94624499765885));
#276230=CARTESIAN_POINT('Ctrl Pts',(-4.3200113853284,92.8107939361435,10.8666927631942));
#276231=CARTESIAN_POINT('Ctrl Pts',(-3.59982559121635,92.8296305703617,
11.1064875492582));
#276232=CARTESIAN_POINT('Ctrl Pts',(-1.39093647983724,92.8876938258724,
11.6075000465635));
#276233=CARTESIAN_POINT('Ctrl Pts',(0.132137348818577,92.9281282121338,
11.6496887621334));
#276234=CARTESIAN_POINT('Ctrl Pts',(3.02010897419524,93.0056179478086,11.1608980046078));
#276235=CARTESIAN_POINT('Ctrl Pts',(4.46788175864068,93.0435700320912,10.6515406785813));
#276236=CARTESIAN_POINT('Ctrl Pts',(7.05209221412667,93.1258189120352,9.01507985911188));
#276237=CARTESIAN_POINT('Ctrl Pts',(8.11193039348105,93.165100379407,8.01934582510662));
#276238=CARTESIAN_POINT('Ctrl Pts',(9.9463038250971,93.2468518201986,5.48682671511057));
#276239=CARTESIAN_POINT('Ctrl Pts',(10.4991557746749,93.2874302123591,4.08411044948916));
#276240=CARTESIAN_POINT('Ctrl Pts',(11.1192237564845,93.3623130546168,1.43522933079907));
#276241=CARTESIAN_POINT('Ctrl Pts',(11.1747094657362,93.4000738876541,-0.0302329141322163));
#276242=CARTESIAN_POINT('Ctrl Pts',(10.7175467303705,93.4786371807489,-2.86025213866675));
#276243=CARTESIAN_POINT('Ctrl Pts',(10.2229105328389,93.518696977927,-4.20226784190578));
#276244=CARTESIAN_POINT('Ctrl Pts',(8.74706554744609,93.5970629058072,-6.63063803679562));
#276245=CARTESIAN_POINT('Ctrl Pts',(7.77752378047288,93.6351162741571,-7.69213698519598));
#276246=CARTESIAN_POINT('Ctrl Pts',(6.05893990234535,93.6957097996795,-8.94941269430666));
#276247=CARTESIAN_POINT('Ctrl Pts',(5.45372378818858,93.7157422931018,-9.30741418619836));
#276248=CARTESIAN_POINT('Ctrl Pts',(3.61704124833991,93.7729986214116,-10.1647555333684));
#276249=CARTESIAN_POINT('Ctrl Pts',(2.23967766451721,93.8109335955831,-10.5392880962719));
#276250=CARTESIAN_POINT('Ctrl Pts',(-0.814433850702704,93.8992040341989,
-10.6637298323807));
#276251=CARTESIAN_POINT('Ctrl Pts',(-2.205161618853,93.9397832479048,-10.3781035460965));
#276252=CARTESIAN_POINT('Ctrl Pts',(-4.56420121931845,94.0099587092093,
-9.51297076079011));
#276253=CARTESIAN_POINT('Ctrl Pts',(-5.69260107256812,94.0483614325352,
-8.83854113951805));
#276254=CARTESIAN_POINT('Ctrl Pts',(-7.63861966215954,94.1251920550018,
-7.11118943227298));
#276255=CARTESIAN_POINT('Ctrl Pts',(-8.50510758937149,94.163586056503,-6.0180431767386));
#276256=CARTESIAN_POINT('Ctrl Pts',(-9.66899795618243,94.2432885837152,
-3.58491338927264));
#276257=CARTESIAN_POINT('Ctrl Pts',(-9.99624123320409,94.2809774299658,
-2.37613833619406));
#276258=CARTESIAN_POINT('Ctrl Pts',(-10.1300916521385,94.3290886022729,
-0.759197386330359));
#276259=CARTESIAN_POINT('Ctrl Pts',(-10.1402351895106,94.3402335604895,
-0.379162435421409));
#276260=CARTESIAN_POINT('Ctrl Pts',(-10.1292796487468,94.3511891012534,
-3.61308205576449E-13));
#276261=CARTESIAN_POINT('Origin',(-7.54701734185159E-14,109.38046875,0.));
#276262=CARTESIAN_POINT('Ctrl Pts',(10.9371370246358,108.317605774636,-1.20722876140178E-12));
#276263=CARTESIAN_POINT('Ctrl Pts',(10.9828089962346,108.363277746235,-0.457318519945779));
#276264=CARTESIAN_POINT('Ctrl Pts',(11.0000648203508,108.409479285711,-0.916344195964511));
#276265=CARTESIAN_POINT('Ctrl Pts',(10.9568199431785,108.605400899729,-2.84979780113602));
#276266=CARTESIAN_POINT('Ctrl Pts',(10.6307901096444,108.756544688372,-4.31034356862055));
#276267=CARTESIAN_POINT('Ctrl Pts',(9.63928557161438,108.994702486232,-6.54978660282652));
#276268=CARTESIAN_POINT('Ctrl Pts',(9.18158964065412,109.07307336719,-7.27431422591661));
#276269=CARTESIAN_POINT('Ctrl Pts',(8.26278618214127,109.220237796992,-8.52069965894701));
#276270=CARTESIAN_POINT('Ctrl Pts',(7.69604270790284,109.300636569957,-9.14095690657997));
#276271=CARTESIAN_POINT('Ctrl Pts',(7.06903888345942,109.38046875,-9.69683913778806));
#276272=CARTESIAN_POINT('',(11.952947197667,109.333415947667,-1.48178615512317E-14));
#276273=CARTESIAN_POINT('Ctrl Pts',(11.8516579398691,109.38046875,-1.88101145034666));
#276274=CARTESIAN_POINT('Ctrl Pts',(11.9344344341192,109.364552105091,-1.25792197685612));
#276275=CARTESIAN_POINT('Ctrl Pts',(11.9683416601056,109.348810410106,-0.628713018278117));
#276276=CARTESIAN_POINT('Ctrl Pts',(11.952947197667,109.333415947667,-3.24740234702858E-14));
#276277=CARTESIAN_POINT('',(13.0499999999999,110.43046875,-1.5981640728873E-15));
#276278=CARTESIAN_POINT('',(11.9999999999999,109.38046875,-1.46957615897682E-15));
#276279=CARTESIAN_POINT('Origin',(-7.60748716635999E-14,110.43046875,0.));
#276280=CARTESIAN_POINT('Ctrl Pts',(11.952947197667,109.333415947667,3.13638004456607E-14));
#276281=CARTESIAN_POINT('Ctrl Pts',(11.9361764328271,109.316645182827,0.684921491956612));
#276282=CARTESIAN_POINT('Ctrl Pts',(11.8599674216354,109.29935041853,1.36919665137744));
#276283=CARTESIAN_POINT('Ctrl Pts',(11.4730011189775,109.249063059047,3.29578789917538));
#276284=CARTESIAN_POINT('Ctrl Pts',(11.0211144208823,109.215720290848,4.4985163450752));
#276285=CARTESIAN_POINT('Ctrl Pts',(10.0086823313146,109.163528707969,6.26438058673198));
#276286=CARTESIAN_POINT('Ctrl Pts',(9.56664237078174,109.144696058498,6.88882718671992));
#276287=CARTESIAN_POINT('Ctrl Pts',(8.06901266781109,109.086716018239,8.6169708190365));
#276288=CARTESIAN_POINT('Ctrl Pts',(6.85368625009054,109.046260158232,9.56255164669703));
#276289=CARTESIAN_POINT('Ctrl Pts',(4.21079500114126,108.968719165965,10.890719112925));
#276290=CARTESIAN_POINT('Ctrl Pts',(2.72850500147909,108.930794662696,11.3415417579546));
#276291=CARTESIAN_POINT('Ctrl Pts',(-0.353974635331329,108.848567400121,
11.5547589716743));
#276292=CARTESIAN_POINT('Ctrl Pts',(-1.81312200817527,108.809238555222,
11.377609085633));
#276293=CARTESIAN_POINT('Ctrl Pts',(-4.7766980905649,108.72856277097,10.426047251413));
#276294=CARTESIAN_POINT('Ctrl Pts',(-6.06885139591756,108.688381621656,
9.63585458101247));
#276295=CARTESIAN_POINT('Ctrl Pts',(-8.19920523793862,108.611961202264,
7.81291676199372));
#276296=CARTESIAN_POINT('Ctrl Pts',(-9.11924339429115,108.57419762057,6.65404377338028));
#276297=CARTESIAN_POINT('Ctrl Pts',(-10.439195517319,108.49573029401,4.07719125689671));
#276298=CARTESIAN_POINT('Ctrl Pts',(-10.8391889019031,108.455639008447,
2.6874865390273));
#276299=CARTESIAN_POINT('Ctrl Pts',(-11.0891692155128,108.377141915412,
-0.174830130587083));
#276300=CARTESIAN_POINT('Ctrl Pts',(-10.9338206948192,108.339099105353,
-1.62092318083063));
#276301=CARTESIAN_POINT('Ctrl Pts',(-10.0428368869227,108.255905747577,
-4.43801234683806));
#276302=CARTESIAN_POINT('Ctrl Pts',(-9.31543510841679,108.216187512317,
-5.6993707846993));
#276303=CARTESIAN_POINT('Ctrl Pts',(-7.566753328723,108.141749268725,-7.76993416685136));
#276304=CARTESIAN_POINT('Ctrl Pts',(-6.50812173253096,108.102871888907,
-8.62766004041432));
#276305=CARTESIAN_POINT('Ctrl Pts',(-4.16308966090255,108.026690485365,
-9.88571225891757));
#276306=CARTESIAN_POINT('Ctrl Pts',(-2.80350980033859,107.988483056552,
-10.3421060224423));
#276307=CARTESIAN_POINT('Ctrl Pts',(0.0619227332583308,107.905310295235,
-10.6126892031837));
#276308=CARTESIAN_POINT('Ctrl Pts',(1.43257949959365,107.865068333532,-10.4754648420145));
#276309=CARTESIAN_POINT('Ctrl Pts',(3.38998859143884,107.806953429599,-9.88342127397056));
#276310=CARTESIAN_POINT('Ctrl Pts',(4.01942385278669,107.787935859554,-9.62411150470083));
#276311=CARTESIAN_POINT('Ctrl Pts',(5.79234492729014,107.729258630109,-8.67805514103696));
#276312=CARTESIAN_POINT('Ctrl Pts',(6.83259006553437,107.689352061935,-7.8327023884626));
#276313=CARTESIAN_POINT('Ctrl Pts',(8.48087656920956,107.614172913412,-5.86047188401398));
#276314=CARTESIAN_POINT('Ctrl Pts',(9.0983171567984,107.578847249204,-4.77235854786256));
#276315=CARTESIAN_POINT('Ctrl Pts',(9.89948065809396,107.504398305741,-2.44433261748365));
#276316=CARTESIAN_POINT('Ctrl Pts',(10.0851375233499,107.467360083825,-1.23130189093642));
#276317=CARTESIAN_POINT('Ctrl Pts',(10.0514325246607,107.431911591494,-0.0144013199032733));
#276318=CARTESIAN_POINT('Origin',(2.27702183671572E-14,91.43046875,0.));
#276319=CARTESIAN_POINT('',(-1.38777878078145E-14,91.43046875,18.));
#276320=CARTESIAN_POINT('',(15.5884572681199,91.43046875,9.));
#276321=CARTESIAN_POINT('Origin',(-1.38777878078145E-14,91.43046875,0.));
#276322=CARTESIAN_POINT('',(-15.5884572681199,91.43046875,9.));
#276323=CARTESIAN_POINT('Origin',(-1.38777878078145E-14,91.43046875,0.));
#276324=CARTESIAN_POINT('',(-15.5884572681199,91.43046875,-9.));
#276325=CARTESIAN_POINT('Origin',(-1.38777878078145E-14,91.43046875,0.));
#276326=CARTESIAN_POINT('',(-1.38777878078145E-14,91.43046875,-18.));
#276327=CARTESIAN_POINT('Origin',(-1.38777878078145E-14,91.43046875,0.));
#276328=CARTESIAN_POINT('',(15.5884572681199,91.43046875,-9.));
#276329=CARTESIAN_POINT('Origin',(-1.38777878078145E-14,91.43046875,0.));
#276330=CARTESIAN_POINT('Origin',(-1.38777878078145E-14,91.43046875,0.));
#276331=CARTESIAN_POINT('Origin',(-20.7846096908266,91.43046875,-6.94962355144037E-15));
#276332=CARTESIAN_POINT('',(-10.3923048454133,93.0381639045868,18.));
#276333=CARTESIAN_POINT('Ctrl Pts',(-10.39230484538,93.038163904606,18.0000000000577));
#276334=CARTESIAN_POINT('Ctrl Pts',(-13.1769145362265,91.43046875,13.176914536263));
#276335=CARTESIAN_POINT('Ctrl Pts',(-15.5884572681199,91.43046875,9.00000000000001));
#276336=CARTESIAN_POINT('',(-10.3923048454133,108.822773595413,18.));
#276337=CARTESIAN_POINT('',(-10.3923048454133,91.43046875,18.));
#276338=CARTESIAN_POINT('',(-15.5884572681199,110.43046875,9.));
#276339=CARTESIAN_POINT('Ctrl Pts',(-10.3923048453801,108.822773595394,
18.0000000000576));
#276340=CARTESIAN_POINT('Ctrl Pts',(-13.1769145362265,110.43046875,13.176914536263));
#276341=CARTESIAN_POINT('Ctrl Pts',(-15.5884572681199,110.43046875,9.00000000000004));
#276342=CARTESIAN_POINT('',(-20.7846096908266,108.822773595413,-4.36661259642003E-15));
#276343=CARTESIAN_POINT('Ctrl Pts',(-15.5884572681199,110.43046875,9.00000000000004));
#276344=CARTESIAN_POINT('Ctrl Pts',(-18.0000000000134,110.43046875,4.82308546373706));
#276345=CARTESIAN_POINT('Ctrl Pts',(-20.7846096908599,108.822773595394,
-5.76492496878966E-11));
#276346=CARTESIAN_POINT('',(-20.7846096908266,93.0381639045868,-6.10030560343973E-15));
#276347=CARTESIAN_POINT('',(-20.7846096908266,91.43046875,-6.94962355144037E-15));
#276348=CARTESIAN_POINT('Ctrl Pts',(-15.5884572681199,91.43046875,9.00000000000001));
#276349=CARTESIAN_POINT('Ctrl Pts',(-18.0000000000134,91.43046875,4.82308546373705));
#276350=CARTESIAN_POINT('Ctrl Pts',(-20.7846096908599,93.038163904606,-5.76355956615792E-11));
#276351=CARTESIAN_POINT('Origin',(-10.3923048454133,91.43046875,-18.));
#276352=CARTESIAN_POINT('Ctrl Pts',(-20.7846096908598,93.038163904606,5.75936582950325E-11));
#276353=CARTESIAN_POINT('Ctrl Pts',(-18.0000000000134,91.4304687500001,
-4.82308546373707));
#276354=CARTESIAN_POINT('Ctrl Pts',(-15.58845726812,91.4304687500001,-9.00000000000002));
#276355=CARTESIAN_POINT('',(-15.5884572681199,110.43046875,-9.));
#276356=CARTESIAN_POINT('Ctrl Pts',(-20.7846096908599,108.822773595394,
5.7616089909697E-11));
#276357=CARTESIAN_POINT('Ctrl Pts',(-18.0000000000135,110.43046875,-4.82308546373705));
#276358=CARTESIAN_POINT('Ctrl Pts',(-15.58845726812,110.43046875,-9.00000000000001));
#276359=CARTESIAN_POINT('',(-10.3923048454133,108.822773595413,-18.));
#276360=CARTESIAN_POINT('Ctrl Pts',(-15.58845726812,110.43046875,-9.00000000000001));
#276361=CARTESIAN_POINT('Ctrl Pts',(-13.1769145362265,110.43046875,-13.176914536263));
#276362=CARTESIAN_POINT('Ctrl Pts',(-10.3923048453801,108.822773595394,
-18.0000000000577));
#276363=CARTESIAN_POINT('',(-10.3923048454133,93.0381639045868,-18.));
#276364=CARTESIAN_POINT('',(-10.3923048454133,91.43046875,-18.));
#276365=CARTESIAN_POINT('Ctrl Pts',(-15.58845726812,91.4304687500001,-9.00000000000002));
#276366=CARTESIAN_POINT('Ctrl Pts',(-13.1769145362265,91.43046875,-13.176914536263));
#276367=CARTESIAN_POINT('Ctrl Pts',(-10.3923048453801,93.038163904606,-18.0000000000576));
#276368=CARTESIAN_POINT('Origin',(10.3923048454132,91.43046875,-18.));
#276369=CARTESIAN_POINT('Ctrl Pts',(-10.3923048454799,93.038163904606,-18.));
#276370=CARTESIAN_POINT('Ctrl Pts',(-4.82308546378702,91.43046875,-18.));
#276371=CARTESIAN_POINT('Ctrl Pts',(-3.2589543430822E-14,91.43046875,-18.));
#276372=CARTESIAN_POINT('',(-1.38777878078145E-14,110.43046875,-18.));
#276373=CARTESIAN_POINT('Ctrl Pts',(-10.3923048454799,108.822773595394,
-18.));
#276374=CARTESIAN_POINT('Ctrl Pts',(-4.82308546378693,110.43046875,-18.));
#276375=CARTESIAN_POINT('Ctrl Pts',(9.0526509530061E-14,110.43046875,-18.));
#276376=CARTESIAN_POINT('',(10.3923048454132,108.822773595413,-18.));
#276377=CARTESIAN_POINT('Ctrl Pts',(9.0526509530061E-14,110.43046875,-18.));
#276378=CARTESIAN_POINT('Ctrl Pts',(4.82308546378697,110.43046875,-18.));
#276379=CARTESIAN_POINT('Ctrl Pts',(10.3923048454797,108.822773595394,-18.));
#276380=CARTESIAN_POINT('',(10.3923048454132,93.0381639045867,-18.));
#276381=CARTESIAN_POINT('',(10.3923048454132,91.43046875,-18.));
#276382=CARTESIAN_POINT('Ctrl Pts',(-3.2589543430822E-14,91.43046875,-18.));
#276383=CARTESIAN_POINT('Ctrl Pts',(4.8230854637869,91.43046875,-18.));
#276384=CARTESIAN_POINT('Ctrl Pts',(10.3923048454797,93.0381639046059,-18.));
#276385=CARTESIAN_POINT('Origin',(20.7846096908265,91.43046875,-3.86306572340787E-15));
#276386=CARTESIAN_POINT('Ctrl Pts',(10.3923048453799,93.0381639046059,-18.0000000000576));
#276387=CARTESIAN_POINT('Ctrl Pts',(13.1769145362264,91.43046875,-13.176914536263));
#276388=CARTESIAN_POINT('Ctrl Pts',(15.5884572681198,91.43046875,-8.99999999999999));
#276389=CARTESIAN_POINT('',(15.5884572681199,110.43046875,-9.));
#276390=CARTESIAN_POINT('Ctrl Pts',(10.3923048453799,108.822773595394,-18.0000000000576));
#276391=CARTESIAN_POINT('Ctrl Pts',(13.1769145362264,110.43046875,-13.1769145362629));
#276392=CARTESIAN_POINT('Ctrl Pts',(15.5884572681199,110.43046875,-8.99999999999993));
#276393=CARTESIAN_POINT('',(20.7846096908264,108.822773595413,-3.76180926347169E-15));
#276394=CARTESIAN_POINT('Ctrl Pts',(15.5884572681199,110.43046875,-8.99999999999993));
#276395=CARTESIAN_POINT('Ctrl Pts',(18.0000000000133,110.43046875,-4.82308546373703));
#276396=CARTESIAN_POINT('Ctrl Pts',(20.7846096908597,108.822773595394,5.75790289811204E-11));
#276397=CARTESIAN_POINT('',(20.7846096908265,93.0381639045867,-2.6733106584905E-15));
#276398=CARTESIAN_POINT('',(20.7846096908265,91.43046875,-3.86306572340787E-15));
#276399=CARTESIAN_POINT('Ctrl Pts',(15.5884572681198,91.43046875,-8.99999999999999));
#276400=CARTESIAN_POINT('Ctrl Pts',(18.0000000000133,91.43046875,-4.82308546373704));
#276401=CARTESIAN_POINT('Ctrl Pts',(20.7846096908597,93.0381639046059,5.76336450863906E-11));
#276402=CARTESIAN_POINT('Origin',(10.3923048454132,91.43046875,18.));
#276403=CARTESIAN_POINT('Ctrl Pts',(20.7846096908597,93.0381639046059,-5.76141393345085E-11));
#276404=CARTESIAN_POINT('Ctrl Pts',(18.0000000000133,91.43046875,4.82308546373704));
#276405=CARTESIAN_POINT('Ctrl Pts',(15.5884572681198,91.43046875,8.99999999999998));
#276406=CARTESIAN_POINT('',(15.5884572681199,110.43046875,9.));
#276407=CARTESIAN_POINT('Ctrl Pts',(20.7846096908597,108.822773595394,-5.76531508382729E-11));
#276408=CARTESIAN_POINT('Ctrl Pts',(18.0000000000133,110.43046875,4.82308546373702));
#276409=CARTESIAN_POINT('Ctrl Pts',(15.5884572681198,110.43046875,8.99999999999998));
#276410=CARTESIAN_POINT('',(10.3923048454132,108.822773595413,18.));
#276411=CARTESIAN_POINT('Ctrl Pts',(15.5884572681198,110.43046875,8.99999999999998));
#276412=CARTESIAN_POINT('Ctrl Pts',(13.1769145362263,110.43046875,13.176914536263));
#276413=CARTESIAN_POINT('Ctrl Pts',(10.3923048453799,108.822773595394,18.0000000000577));
#276414=CARTESIAN_POINT('',(10.3923048454132,93.0381639045867,18.));
#276415=CARTESIAN_POINT('',(10.3923048454132,91.43046875,18.));
#276416=CARTESIAN_POINT('Ctrl Pts',(15.5884572681198,91.43046875,8.99999999999998));
#276417=CARTESIAN_POINT('Ctrl Pts',(13.1769145362264,91.43046875,13.1769145362629));
#276418=CARTESIAN_POINT('Ctrl Pts',(10.3923048453799,93.0381639046059,18.0000000000576));
#276419=CARTESIAN_POINT('Origin',(-10.3923048454133,91.43046875,18.));
#276420=CARTESIAN_POINT('Ctrl Pts',(10.3923048454797,93.0381639046059,18.));
#276421=CARTESIAN_POINT('Ctrl Pts',(4.8230854637869,91.43046875,18.));
#276422=CARTESIAN_POINT('Ctrl Pts',(-2.17263622872146E-14,91.43046875,18.));
#276423=CARTESIAN_POINT('',(-1.38777878078145E-14,110.43046875,18.));
#276424=CARTESIAN_POINT('Ctrl Pts',(10.3923048454797,108.822773595394,18.));
#276425=CARTESIAN_POINT('Ctrl Pts',(4.82308546378686,110.43046875,18.));
#276426=CARTESIAN_POINT('Ctrl Pts',(-1.14063402007877E-13,110.43046875,
18.));
#276427=CARTESIAN_POINT('Ctrl Pts',(-1.14063402007877E-13,110.43046875,
18.));
#276428=CARTESIAN_POINT('Ctrl Pts',(-4.82308546378701,110.43046875,18.));
#276429=CARTESIAN_POINT('Ctrl Pts',(-10.3923048454798,108.822773595394,
18.));
#276430=CARTESIAN_POINT('Ctrl Pts',(-1.44842415248098E-14,91.43046875,18.));
#276431=CARTESIAN_POINT('Ctrl Pts',(-4.82308546378699,91.43046875,18.));
#276432=CARTESIAN_POINT('Ctrl Pts',(-10.3923048454799,93.038163904606,18.));
#276433=CARTESIAN_POINT('Origin',(1.18280596465885E-14,110.43046875,0.));
#276434=CARTESIAN_POINT('Origin',(-1.38777878078145E-14,110.43046875,0.));
#276435=CARTESIAN_POINT('Origin',(-1.38777878078145E-14,110.43046875,0.));
#276436=CARTESIAN_POINT('Origin',(-1.38777878078145E-14,110.43046875,0.));
#276437=CARTESIAN_POINT('Origin',(-1.38777878078145E-14,110.43046875,0.));
#276438=CARTESIAN_POINT('Origin',(-1.38777878078145E-14,110.43046875,0.));
#276439=CARTESIAN_POINT('Origin',(-1.38777878078145E-14,110.43046875,0.));
#276440=CARTESIAN_POINT('Origin',(-1.38777878078145E-14,110.43046875,0.));
#276441=CARTESIAN_POINT('Origin',(-1.38777878078145E-14,110.43046875,0.));
#276442=CARTESIAN_POINT('Origin',(-1.38777878078145E-14,110.43046875,0.));
#276443=CARTESIAN_POINT('Origin',(-1.38777878078145E-14,110.43046875,0.));
#276444=CARTESIAN_POINT('Origin',(-1.38777878078145E-14,110.43046875,0.));
#276445=CARTESIAN_POINT('Origin',(-1.38777878078145E-14,110.43046875,0.));
#276446=CARTESIAN_POINT('Origin',(-1.38777878078145E-14,91.43046875,0.));
#276447=CARTESIAN_POINT('Origin',(-1.38777878078145E-14,91.43046875,0.));
#276448=CARTESIAN_POINT('Origin',(-1.38777878078145E-14,91.43046875,0.));
#276449=CARTESIAN_POINT('Origin',(-1.38777878078145E-14,91.43046875,0.));
#276450=CARTESIAN_POINT('Origin',(-1.38777878078145E-14,91.43046875,0.));
#276451=CARTESIAN_POINT('Origin',(-1.38777878078145E-14,91.43046875,0.));
#276452=CARTESIAN_POINT('Ctrl Pts',(-10.0514385264422,-1.69375249127916,
2.46189240364677E-15));
#276453=CARTESIAN_POINT('Ctrl Pts',(-10.0514385264422,-1.54375249127976,
3.26591035271534));
#276454=CARTESIAN_POINT('Ctrl Pts',(-8.13178458580685,-1.39375249128036,
5.90808733016713));
#276455=CARTESIAN_POINT('Ctrl Pts',(-6.21213064517146,-1.24375249128095,
8.55026430761891));
#276456=CARTESIAN_POINT('Ctrl Pts',(-3.10606532258574,-1.09375249128155,
9.55948610871303));
#276457=CARTESIAN_POINT('Ctrl Pts',(-9.99267329551972E-15,-0.943752491282151,
10.5687079098071));
#276458=CARTESIAN_POINT('Ctrl Pts',(3.10606532258571,-0.79375249128275,
9.55948610871303));
#276459=CARTESIAN_POINT('Ctrl Pts',(6.21213064517144,-0.643752491283348,
8.55026430761891));
#276460=CARTESIAN_POINT('Ctrl Pts',(8.13178458580682,-0.493752491283947,
5.90808733016712));
#276461=CARTESIAN_POINT('Ctrl Pts',(10.0514385264422,-0.343752491284545,
3.26591035271534));
#276462=CARTESIAN_POINT('Ctrl Pts',(10.0514385264422,-0.193752491285145,
-1.23094620182339E-15));
#276463=CARTESIAN_POINT('Ctrl Pts',(10.0514385264422,-0.0437524912857454,
-3.26591035271534));
#276464=CARTESIAN_POINT('Ctrl Pts',(8.13178458580682,0.106247508713654,
-5.90808733016713));
#276465=CARTESIAN_POINT('Ctrl Pts',(6.21213064517144,0.256247508713052,
-8.55026430761891));
#276466=CARTESIAN_POINT('Ctrl Pts',(3.10606532258571,0.40624750871245,-9.55948610871303));
#276467=CARTESIAN_POINT('Ctrl Pts',(-1.34451147939244E-14,0.556247508711849,
-10.5687079098071));
#276468=CARTESIAN_POINT('Ctrl Pts',(-3.10606532258574,0.706247508711247,
-9.55948610871303));
#276469=CARTESIAN_POINT('Ctrl Pts',(-6.21213064517146,0.856247508710645,
-8.55026430761891));
#276470=CARTESIAN_POINT('Ctrl Pts',(-8.13178458580685,1.00624750871004,
-5.90808733016712));
#276471=CARTESIAN_POINT('Ctrl Pts',(-10.0514385264422,1.15624750870944,
-3.26591035271534));
#276472=CARTESIAN_POINT('Ctrl Pts',(-10.0514385264422,1.30624750870884,
2.46189240364677E-15));
#276473=CARTESIAN_POINT('Ctrl Pts',(-10.0514385264422,1.45624750870824,
3.26591035271534));
#276474=CARTESIAN_POINT('Ctrl Pts',(-8.13178458580685,1.60624750870764,
5.90808733016713));
#276475=CARTESIAN_POINT('Ctrl Pts',(-6.21213064517146,1.75624750870705,
8.55026430761891));
#276476=CARTESIAN_POINT('Ctrl Pts',(-3.10606532258574,1.90624750870645,
9.55948610871303));
#276477=CARTESIAN_POINT('Ctrl Pts',(-1.17203825671816E-14,2.05624750870585,
10.5687079098071));
#276478=CARTESIAN_POINT('Ctrl Pts',(3.10606532258571,2.20624750870525,9.55948610871303));
#276479=CARTESIAN_POINT('Ctrl Pts',(6.21213064517144,2.35624750870465,8.55026430761891));
#276480=CARTESIAN_POINT('Ctrl Pts',(8.13178458580682,2.50624750870405,5.90808733016712));
#276481=CARTESIAN_POINT('Ctrl Pts',(10.0514385264422,2.65624750870345,3.26591035271534));
#276482=CARTESIAN_POINT('Ctrl Pts',(10.0514385264422,2.80624750870286,-1.23094620182339E-15));
#276483=CARTESIAN_POINT('Ctrl Pts',(10.0514385264422,2.95624750870225,-3.26591035271534));
#276484=CARTESIAN_POINT('Ctrl Pts',(8.13178458580682,3.10624750870165,-5.90808733016713));
#276485=CARTESIAN_POINT('Ctrl Pts',(6.21213064517143,3.25624750870105,-8.55026430761891));
#276486=CARTESIAN_POINT('Ctrl Pts',(3.10606532258571,3.40624750870045,-9.55948610871303));
#276487=CARTESIAN_POINT('Ctrl Pts',(-1.51728240655862E-14,3.55624750869985,
-10.5687079098071));
#276488=CARTESIAN_POINT('Ctrl Pts',(-3.10606532258574,3.70624750869925,
-9.55948610871303));
#276489=CARTESIAN_POINT('Ctrl Pts',(-6.21213064517146,3.85624750869865,
-8.55026430761891));
#276490=CARTESIAN_POINT('Ctrl Pts',(-8.13178458580685,4.00624750869804,
-5.90808733016712));
#276491=CARTESIAN_POINT('Ctrl Pts',(-10.0514385264422,4.15624750869744,
-3.26591035271534));
#276492=CARTESIAN_POINT('Ctrl Pts',(-10.0514385264422,4.30624750869684,
2.46189240364677E-15));
#276493=CARTESIAN_POINT('Ctrl Pts',(-10.0514385264422,4.45624750869624,
3.26591035271534));
#276494=CARTESIAN_POINT('Ctrl Pts',(-8.13178458580685,4.60624750869564,
5.90808733016713));
#276495=CARTESIAN_POINT('Ctrl Pts',(-6.21213064517146,4.75624750869505,
8.55026430761891));
#276496=CARTESIAN_POINT('Ctrl Pts',(-3.10606532258574,4.90624750869445,
9.55948610871303));
#276497=CARTESIAN_POINT('Ctrl Pts',(-1.34480918388434E-14,5.05624750869385,
10.5687079098071));
#276498=CARTESIAN_POINT('Ctrl Pts',(3.10606532258571,5.20624750869325,9.55948610871303));
#276499=CARTESIAN_POINT('Ctrl Pts',(6.21213064517144,5.35624750869265,8.55026430761891));
#276500=CARTESIAN_POINT('Ctrl Pts',(8.13178458580682,5.50624750869205,5.90808733016712));
#276501=CARTESIAN_POINT('Ctrl Pts',(10.0514385264422,5.65624750869145,3.26591035271534));
#276502=CARTESIAN_POINT('Ctrl Pts',(10.0514385264422,5.80624750869085,-1.23094620182339E-15));
#276503=CARTESIAN_POINT('Ctrl Pts',(10.0514385264422,5.95624750869025,-3.26591035271534));
#276504=CARTESIAN_POINT('Ctrl Pts',(8.13178458580682,6.10624750868966,-5.90808733016713));
#276505=CARTESIAN_POINT('Ctrl Pts',(6.21213064517143,6.25624750868905,-8.55026430761891));
#276506=CARTESIAN_POINT('Ctrl Pts',(3.10606532258571,6.40624750868845,-9.55948610871303));
#276507=CARTESIAN_POINT('Ctrl Pts',(-1.6900533337248E-14,6.55624750868785,
-10.5687079098071));
#276508=CARTESIAN_POINT('Ctrl Pts',(-3.10606532258574,6.70624750868725,
-9.55948610871303));
#276509=CARTESIAN_POINT('Ctrl Pts',(-6.21213064517146,6.85624750868664,
-8.55026430761891));
#276510=CARTESIAN_POINT('Ctrl Pts',(-8.13178458580685,7.00624750868604,
-5.90808733016712));
#276511=CARTESIAN_POINT('Ctrl Pts',(-10.0514385264422,7.15624750868544,
-3.26591035271534));
#276512=CARTESIAN_POINT('Ctrl Pts',(-10.0514385264422,7.30624750868484,
2.46189240364677E-15));
#276513=CARTESIAN_POINT('Ctrl Pts',(-10.0514385264422,7.45624750868424,
3.26591035271534));
#276514=CARTESIAN_POINT('Ctrl Pts',(-8.13178458580685,7.60624750868365,
5.90808733016713));
#276515=CARTESIAN_POINT('Ctrl Pts',(-6.21213064517146,7.75624750868305,
8.55026430761891));
#276516=CARTESIAN_POINT('Ctrl Pts',(-3.10606532258574,7.90624750868245,
9.55948610871303));
#276517=CARTESIAN_POINT('Ctrl Pts',(-1.51758011105052E-14,8.05624750868185,
10.5687079098071));
#276518=CARTESIAN_POINT('Ctrl Pts',(3.10606532258571,8.20624750868125,9.55948610871303));
#276519=CARTESIAN_POINT('Ctrl Pts',(6.21213064517143,8.35624750868065,8.55026430761891));
#276520=CARTESIAN_POINT('Ctrl Pts',(8.13178458580682,8.50624750868005,5.90808733016712));
#276521=CARTESIAN_POINT('Ctrl Pts',(10.0514385264422,8.65624750867945,3.26591035271534));
#276522=CARTESIAN_POINT('Ctrl Pts',(10.0514385264422,8.80624750867885,-1.23094620182339E-15));
#276523=CARTESIAN_POINT('Ctrl Pts',(10.0514385264422,8.95624750867826,-3.26591035271534));
#276524=CARTESIAN_POINT('Ctrl Pts',(8.13178458580681,9.10624750867765,-5.90808733016713));
#276525=CARTESIAN_POINT('Ctrl Pts',(6.21213064517143,9.25624750867705,-8.55026430761891));
#276526=CARTESIAN_POINT('Ctrl Pts',(3.10606532258571,9.40624750867645,-9.55948610871303));
#276527=CARTESIAN_POINT('Ctrl Pts',(-1.86282426089099E-14,9.55624750867585,
-10.5687079098071));
#276528=CARTESIAN_POINT('Ctrl Pts',(-3.10606532258574,9.70624750867525,
-9.55948610871303));
#276529=CARTESIAN_POINT('Ctrl Pts',(-6.21213064517147,9.85624750867465,
-8.55026430761891));
#276530=CARTESIAN_POINT('Ctrl Pts',(-8.13178458580685,10.006247508674,-5.90808733016712));
#276531=CARTESIAN_POINT('Ctrl Pts',(-10.0514385264422,10.1562475086734,
-3.26591035271534));
#276532=CARTESIAN_POINT('Ctrl Pts',(-10.0514385264422,10.3062475086728,
2.46189240364677E-15));
#276533=CARTESIAN_POINT('Ctrl Pts',(-10.0514385264422,10.4562475086722,
3.26591035271534));
#276534=CARTESIAN_POINT('Ctrl Pts',(-8.13178458580685,10.6062475086716,
5.90808733016713));
#276535=CARTESIAN_POINT('Ctrl Pts',(-6.21213064517146,10.756247508671,8.55026430761891));
#276536=CARTESIAN_POINT('Ctrl Pts',(-3.10606532258574,10.9062475086704,
9.55948610871303));
#276537=CARTESIAN_POINT('Ctrl Pts',(-1.69035103821671E-14,11.0562475086699,
10.5687079098071));
#276538=CARTESIAN_POINT('Ctrl Pts',(3.10606532258571,11.2062475086693,9.55948610871303));
#276539=CARTESIAN_POINT('Ctrl Pts',(6.21213064517143,11.3562475086687,8.55026430761891));
#276540=CARTESIAN_POINT('Ctrl Pts',(8.13178458580681,11.5062475086681,5.90808733016712));
#276541=CARTESIAN_POINT('Ctrl Pts',(10.0514385264422,11.6562475086675,3.26591035271534));
#276542=CARTESIAN_POINT('Ctrl Pts',(10.0514385264422,11.8062475086669,-1.23094620182339E-15));
#276543=CARTESIAN_POINT('Ctrl Pts',(10.0514385264422,11.9562475086663,-3.26591035271534));
#276544=CARTESIAN_POINT('Ctrl Pts',(8.13178458580681,12.1062475086657,-5.90808733016713));
#276545=CARTESIAN_POINT('Ctrl Pts',(6.21213064517143,12.2562475086651,-8.55026430761891));
#276546=CARTESIAN_POINT('Ctrl Pts',(3.1060653225857,12.4062475086645,-9.55948610871303));
#276547=CARTESIAN_POINT('Ctrl Pts',(-2.03559518805717E-14,12.5562475086638,
-10.5687079098071));
#276548=CARTESIAN_POINT('Ctrl Pts',(-3.10606532258575,12.7062475086632,
-9.55948610871303));
#276549=CARTESIAN_POINT('Ctrl Pts',(-6.21213064517147,12.8562475086626,
-8.55026430761891));
#276550=CARTESIAN_POINT('Ctrl Pts',(-8.13178458580686,13.006247508662,-5.90808733016712));
#276551=CARTESIAN_POINT('Ctrl Pts',(-10.0514385264422,13.1562475086614,
-3.26591035271534));
#276552=CARTESIAN_POINT('Ctrl Pts',(-10.0514385264422,13.3062475086608,
2.46189240364677E-15));
#276553=CARTESIAN_POINT('Ctrl Pts',(-10.0514385264422,13.4562475086602,
3.26591035271534));
#276554=CARTESIAN_POINT('Ctrl Pts',(-8.13178458580686,13.6062475086596,
5.90808733016713));
#276555=CARTESIAN_POINT('Ctrl Pts',(-6.21213064517146,13.756247508659,8.55026430761891));
#276556=CARTESIAN_POINT('Ctrl Pts',(-3.10606532258574,13.9062475086584,
9.55948610871303));
#276557=CARTESIAN_POINT('Ctrl Pts',(-1.86312196538289E-14,14.0562475086578,
10.5687079098071));
#276558=CARTESIAN_POINT('Ctrl Pts',(3.10606532258571,14.2062475086573,9.55948610871303));
#276559=CARTESIAN_POINT('Ctrl Pts',(6.21213064517143,14.3562475086567,8.55026430761891));
#276560=CARTESIAN_POINT('Ctrl Pts',(8.13178458580681,14.5062475086561,5.90808733016712));
#276561=CARTESIAN_POINT('Ctrl Pts',(10.0514385264422,14.6562475086555,3.26591035271534));
#276562=CARTESIAN_POINT('Ctrl Pts',(10.0514385264422,14.8062475086549,-1.23094620182339E-15));
#276563=CARTESIAN_POINT('Ctrl Pts',(10.0514385264422,14.9562475086543,-3.26591035271534));
#276564=CARTESIAN_POINT('Ctrl Pts',(8.13178458580681,15.1062475086537,-5.90808733016713));
#276565=CARTESIAN_POINT('Ctrl Pts',(6.21213064517143,15.2562475086531,-8.55026430761891));
#276566=CARTESIAN_POINT('Ctrl Pts',(3.1060653225857,15.4062475086525,-9.55948610871303));
#276567=CARTESIAN_POINT('Ctrl Pts',(-2.20836611522336E-14,15.5562475086518,
-10.5687079098071));
#276568=CARTESIAN_POINT('Ctrl Pts',(-3.10606532258575,15.7062475086513,
-9.55948610871303));
#276569=CARTESIAN_POINT('Ctrl Pts',(-6.21213064517147,15.8562475086506,
-8.55026430761891));
#276570=CARTESIAN_POINT('Ctrl Pts',(-8.13178458580686,16.00624750865,-5.90808733016712));
#276571=CARTESIAN_POINT('Ctrl Pts',(-10.0514385264422,16.1562475086494,
-3.26591035271534));
#276572=CARTESIAN_POINT('Ctrl Pts',(-10.0514385264422,16.3062475086488,
2.46189240364677E-15));
#276573=CARTESIAN_POINT('Ctrl Pts',(-10.0514385264422,16.4562475086482,
3.26591035271534));
#276574=CARTESIAN_POINT('Ctrl Pts',(-8.13178458580686,16.6062475086476,
5.90808733016713));
#276575=CARTESIAN_POINT('Ctrl Pts',(-6.21213064517147,16.756247508647,8.55026430761891));
#276576=CARTESIAN_POINT('Ctrl Pts',(-3.10606532258575,16.9062475086464,
9.55948610871303));
#276577=CARTESIAN_POINT('Ctrl Pts',(-2.03589289254908E-14,17.0562475086458,
10.5687079098071));
#276578=CARTESIAN_POINT('Ctrl Pts',(3.1060653225857,17.2062475086453,9.55948610871303));
#276579=CARTESIAN_POINT('Ctrl Pts',(6.21213064517143,17.3562475086446,8.55026430761891));
#276580=CARTESIAN_POINT('Ctrl Pts',(8.13178458580681,17.5062475086441,5.90808733016712));
#276581=CARTESIAN_POINT('Ctrl Pts',(10.0514385264422,17.6562475086435,3.26591035271534));
#276582=CARTESIAN_POINT('Ctrl Pts',(10.0514385264422,17.8062475086429,-1.23094620182339E-15));
#276583=CARTESIAN_POINT('Ctrl Pts',(10.0514385264422,17.9562475086423,-3.26591035271534));
#276584=CARTESIAN_POINT('Ctrl Pts',(8.13178458580681,18.1062475086417,-5.90808733016713));
#276585=CARTESIAN_POINT('Ctrl Pts',(6.21213064517142,18.2562475086411,-8.55026430761891));
#276586=CARTESIAN_POINT('Ctrl Pts',(3.1060653225857,18.4062475086405,-9.55948610871303));
#276587=CARTESIAN_POINT('Ctrl Pts',(-2.38113704238954E-14,18.5562475086398,
-10.5687079098071));
#276588=CARTESIAN_POINT('Ctrl Pts',(-3.10606532258575,18.7062475086392,
-9.55948610871303));
#276589=CARTESIAN_POINT('Ctrl Pts',(-6.21213064517147,18.8562475086386,
-8.55026430761891));
#276590=CARTESIAN_POINT('Ctrl Pts',(-8.13178458580686,19.006247508638,-5.90808733016712));
#276591=CARTESIAN_POINT('Ctrl Pts',(-10.0514385264422,19.1562475086374,
-3.26591035271534));
#276592=CARTESIAN_POINT('Ctrl Pts',(-10.0514385264422,19.3062475086368,
2.46189240364677E-15));
#276593=CARTESIAN_POINT('Ctrl Pts',(-10.0514385264422,19.4562475086362,
3.26591035271534));
#276594=CARTESIAN_POINT('Ctrl Pts',(-8.13178458580686,19.6062475086356,
5.90808733016713));
#276595=CARTESIAN_POINT('Ctrl Pts',(-6.21213064517147,19.756247508635,8.55026430761891));
#276596=CARTESIAN_POINT('Ctrl Pts',(-3.10606532258575,19.9062475086345,
9.55948610871303));
#276597=CARTESIAN_POINT('Ctrl Pts',(-2.20866381971526E-14,20.0562475086338,
10.5687079098071));
#276598=CARTESIAN_POINT('Ctrl Pts',(3.1060653225857,20.2062475086333,9.55948610871303));
#276599=CARTESIAN_POINT('Ctrl Pts',(6.21213064517142,20.3562475086326,8.55026430761891));
#276600=CARTESIAN_POINT('Ctrl Pts',(8.13178458580681,20.5062475086321,5.90808733016712));
#276601=CARTESIAN_POINT('Ctrl Pts',(10.0514385264422,20.6562475086315,3.26591035271534));
#276602=CARTESIAN_POINT('Ctrl Pts',(10.0514385264422,20.8062475086309,-1.23094620182339E-15));
#276603=CARTESIAN_POINT('Ctrl Pts',(10.0514385264422,20.9562475086302,-3.26591035271534));
#276604=CARTESIAN_POINT('Ctrl Pts',(8.13178458580681,21.1062475086297,-5.90808733016713));
#276605=CARTESIAN_POINT('Ctrl Pts',(6.21213064517142,21.256247508629,-8.55026430761891));
#276606=CARTESIAN_POINT('Ctrl Pts',(3.1060653225857,21.4062475086285,-9.55948610871303));
#276607=CARTESIAN_POINT('Ctrl Pts',(-2.55390796955572E-14,21.5562475086278,
-10.5687079098071));
#276608=CARTESIAN_POINT('Ctrl Pts',(-3.10606532258575,21.7062475086273,
-9.55948610871303));
#276609=CARTESIAN_POINT('Ctrl Pts',(-6.21213064517148,21.8562475086266,
-8.55026430761891));
#276610=CARTESIAN_POINT('Ctrl Pts',(-8.13178458580686,22.006247508626,-5.90808733016712));
#276611=CARTESIAN_POINT('Ctrl Pts',(-10.0514385264422,22.1562475086254,
-3.26591035271534));
#276612=CARTESIAN_POINT('Ctrl Pts',(-10.0514385264422,22.3062475086248,
2.46189240364677E-15));
#276613=CARTESIAN_POINT('Ctrl Pts',(-10.0514385264422,22.4562475086242,
3.26591035271534));
#276614=CARTESIAN_POINT('Ctrl Pts',(-8.13178458580686,22.6062475086236,
5.90808733016713));
#276615=CARTESIAN_POINT('Ctrl Pts',(-6.21213064517147,22.756247508623,8.55026430761891));
#276616=CARTESIAN_POINT('Ctrl Pts',(-3.10606532258575,22.9062475086224,
9.55948610871303));
#276617=CARTESIAN_POINT('Ctrl Pts',(-2.38143474688144E-14,23.0562475086218,
10.5687079098071));
#276618=CARTESIAN_POINT('Ctrl Pts',(3.1060653225857,23.2062475086213,9.55948610871303));
#276619=CARTESIAN_POINT('Ctrl Pts',(6.21213064517142,23.3562475086206,8.55026430761891));
#276620=CARTESIAN_POINT('Ctrl Pts',(8.13178458580681,23.5062475086201,5.90808733016712));
#276621=CARTESIAN_POINT('Ctrl Pts',(10.0514385264422,23.6562475086195,3.26591035271534));
#276622=CARTESIAN_POINT('Ctrl Pts',(10.0514385264422,23.8062475086189,-1.23094620182339E-15));
#276623=CARTESIAN_POINT('Ctrl Pts',(10.0514385264422,23.9562475086183,-3.26591035271534));
#276624=CARTESIAN_POINT('Ctrl Pts',(8.13178458580681,24.1062475086177,-5.90808733016713));
#276625=CARTESIAN_POINT('Ctrl Pts',(6.21213064517142,24.256247508617,-8.55026430761891));
#276626=CARTESIAN_POINT('Ctrl Pts',(3.1060653225857,24.4062475086165,-9.55948610871303));
#276627=CARTESIAN_POINT('Ctrl Pts',(-2.72667889672191E-14,24.5562475086158,
-10.5687079098071));
#276628=CARTESIAN_POINT('Ctrl Pts',(-3.10606532258575,24.7062475086152,
-9.55948610871303));
#276629=CARTESIAN_POINT('Ctrl Pts',(-6.21213064517148,24.8562475086146,
-8.55026430761891));
#276630=CARTESIAN_POINT('Ctrl Pts',(-8.13178458580686,25.006247508614,-5.90808733016712));
#276631=CARTESIAN_POINT('Ctrl Pts',(-10.0514385264422,25.1562475086134,
-3.26591035271534));
#276632=CARTESIAN_POINT('Ctrl Pts',(-10.0514385264422,25.3062475086128,
2.46189240364677E-15));
#276633=CARTESIAN_POINT('Ctrl Pts',(-10.0514385264422,25.4562475086122,
3.26591035271534));
#276634=CARTESIAN_POINT('Ctrl Pts',(-8.13178458580686,25.6062475086116,
5.90808733016713));
#276635=CARTESIAN_POINT('Ctrl Pts',(-6.21213064517148,25.756247508611,8.55026430761891));
#276636=CARTESIAN_POINT('Ctrl Pts',(-3.10606532258575,25.9062475086105,
9.55948610871303));
#276637=CARTESIAN_POINT('Ctrl Pts',(-2.55420567404763E-14,26.0562475086098,
10.5687079098071));
#276638=CARTESIAN_POINT('Ctrl Pts',(3.1060653225857,26.2062475086093,9.55948610871303));
#276639=CARTESIAN_POINT('Ctrl Pts',(6.21213064517142,26.3562475086086,8.55026430761891));
#276640=CARTESIAN_POINT('Ctrl Pts',(8.13178458580681,26.5062475086081,5.90808733016712));
#276641=CARTESIAN_POINT('Ctrl Pts',(10.0514385264422,26.6562475086075,3.26591035271534));
#276642=CARTESIAN_POINT('Ctrl Pts',(10.0514385264422,26.8062475086069,-1.23094620182339E-15));
#276643=CARTESIAN_POINT('Ctrl Pts',(10.0514385264422,26.9562475086063,-3.26591035271534));
#276644=CARTESIAN_POINT('Ctrl Pts',(8.13178458580681,27.1062475086057,-5.90808733016713));
#276645=CARTESIAN_POINT('Ctrl Pts',(6.21213064517142,27.256247508605,-8.55026430761891));
#276646=CARTESIAN_POINT('Ctrl Pts',(3.1060653225857,27.4062475086045,-9.55948610871303));
#276647=CARTESIAN_POINT('Ctrl Pts',(-2.89944982388809E-14,27.5562475086038,
-10.5687079098071));
#276648=CARTESIAN_POINT('Ctrl Pts',(-3.10606532258575,27.7062475086032,
-9.55948610871303));
#276649=CARTESIAN_POINT('Ctrl Pts',(-6.21213064517148,27.8562475086026,
-8.55026430761891));
#276650=CARTESIAN_POINT('Ctrl Pts',(-8.13178458580686,28.006247508602,-5.90808733016712));
#276651=CARTESIAN_POINT('Ctrl Pts',(-10.0514385264422,28.1562475086014,
-3.26591035271534));
#276652=CARTESIAN_POINT('Ctrl Pts',(-10.0514385264423,28.3062475086009,
2.46189240364677E-15));
#276653=CARTESIAN_POINT('Ctrl Pts',(-10.0514385264422,28.4562475086002,
3.26591035271534));
#276654=CARTESIAN_POINT('Ctrl Pts',(-8.13178458580686,28.6062475085996,
5.90808733016713));
#276655=CARTESIAN_POINT('Ctrl Pts',(-6.21213064517148,28.756247508599,8.55026430761891));
#276656=CARTESIAN_POINT('Ctrl Pts',(-3.10606532258575,28.9062475085985,
9.55948610871303));
#276657=CARTESIAN_POINT('Ctrl Pts',(-2.72697660121381E-14,29.0562475085978,
10.5687079098071));
#276658=CARTESIAN_POINT('Ctrl Pts',(3.1060653225857,29.2062475085973,9.55948610871303));
#276659=CARTESIAN_POINT('Ctrl Pts',(6.21213064517142,29.3562475085966,8.55026430761891));
#276660=CARTESIAN_POINT('Ctrl Pts',(8.13178458580681,29.5062475085961,5.90808733016712));
#276661=CARTESIAN_POINT('Ctrl Pts',(10.0514385264422,29.6562475085955,3.26591035271534));
#276662=CARTESIAN_POINT('Ctrl Pts',(10.0514385264422,29.8062475085949,-1.23094620182339E-15));
#276663=CARTESIAN_POINT('Ctrl Pts',(10.0514385264422,29.9562475085943,-3.26591035271534));
#276664=CARTESIAN_POINT('Ctrl Pts',(8.1317845858068,30.1062475085937,-5.90808733016713));
#276665=CARTESIAN_POINT('Ctrl Pts',(6.21213064517142,30.256247508593,-8.55026430761891));
#276666=CARTESIAN_POINT('Ctrl Pts',(3.10606532258569,30.4062475085925,-9.55948610871303));
#276667=CARTESIAN_POINT('Ctrl Pts',(-3.07222075105427E-14,30.5562475085918,
-10.5687079098071));
#276668=CARTESIAN_POINT('Ctrl Pts',(-3.10606532258576,30.7062475085912,
-9.55948610871303));
#276669=CARTESIAN_POINT('Ctrl Pts',(-6.21213064517148,30.8562475085907,
-8.55026430761891));
#276670=CARTESIAN_POINT('Ctrl Pts',(-8.13178458580687,31.00624750859,-5.90808733016712));
#276671=CARTESIAN_POINT('Ctrl Pts',(-10.0514385264422,31.1562475085894,
-3.26591035271534));
#276672=CARTESIAN_POINT('Ctrl Pts',(-10.0514385264423,31.3062475085889,
2.46189240364677E-15));
#276673=CARTESIAN_POINT('Ctrl Pts',(-10.0514385264422,31.4562475085882,
3.26591035271534));
#276674=CARTESIAN_POINT('Ctrl Pts',(-8.13178458580687,31.6062475085876,
5.90808733016713));
#276675=CARTESIAN_POINT('Ctrl Pts',(-6.21213064517148,31.756247508587,8.55026430761891));
#276676=CARTESIAN_POINT('Ctrl Pts',(-3.10606532258575,31.9062475085864,
9.55948610871303));
#276677=CARTESIAN_POINT('Ctrl Pts',(-2.89974752837999E-14,32.0562475085858,
10.5687079098071));
#276678=CARTESIAN_POINT('Ctrl Pts',(3.1060653225857,32.2062475085852,9.55948610871303));
#276679=CARTESIAN_POINT('Ctrl Pts',(6.21213064517142,32.3562475085847,8.55026430761891));
#276680=CARTESIAN_POINT('Ctrl Pts',(8.1317845858068,32.5062475085841,5.90808733016712));
#276681=CARTESIAN_POINT('Ctrl Pts',(10.0514385264422,32.6562475085834,3.26591035271534));
#276682=CARTESIAN_POINT('Ctrl Pts',(10.0514385264422,32.8062475085829,-1.23094620182339E-15));
#276683=CARTESIAN_POINT('Ctrl Pts',(10.0514385264422,32.9562475085823,-3.26591035271534));
#276684=CARTESIAN_POINT('Ctrl Pts',(8.1317845858068,33.1062475085817,-5.90808733016713));
#276685=CARTESIAN_POINT('Ctrl Pts',(6.21213064517142,33.256247508581,-8.55026430761891));
#276686=CARTESIAN_POINT('Ctrl Pts',(3.10606532258569,33.4062475085805,-9.55948610871303));
#276687=CARTESIAN_POINT('Ctrl Pts',(-3.24499167822046E-14,33.5562475085799,
-10.5687079098071));
#276688=CARTESIAN_POINT('Ctrl Pts',(-3.10606532258576,33.7062475085792,
-9.55948610871303));
#276689=CARTESIAN_POINT('Ctrl Pts',(-6.21213064517148,33.8562475085787,
-8.55026430761891));
#276690=CARTESIAN_POINT('Ctrl Pts',(-8.13178458580687,34.006247508578,-5.90808733016712));
#276691=CARTESIAN_POINT('Ctrl Pts',(-10.0514385264423,34.1562475085774,
-3.26591035271534));
#276692=CARTESIAN_POINT('Ctrl Pts',(-10.0514385264423,34.3062475085768,
2.46189240364677E-15));
#276693=CARTESIAN_POINT('Ctrl Pts',(-10.0514385264423,34.4562475085762,
3.26591035271534));
#276694=CARTESIAN_POINT('Ctrl Pts',(-8.13178458580687,34.6062475085756,
5.90808733016713));
#276695=CARTESIAN_POINT('Ctrl Pts',(-6.21213064517148,34.7562475085751,
8.55026430761891));
#276696=CARTESIAN_POINT('Ctrl Pts',(-3.10606532258576,34.9062475085744,
9.55948610871303));
#276697=CARTESIAN_POINT('Ctrl Pts',(-3.07251845554618E-14,35.0562475085739,
10.5687079098071));
#276698=CARTESIAN_POINT('Ctrl Pts',(3.10606532258569,35.2062475085733,9.55948610871303));
#276699=CARTESIAN_POINT('Ctrl Pts',(6.21213064517142,35.3562475085727,8.55026430761891));
#276700=CARTESIAN_POINT('Ctrl Pts',(8.1317845858068,35.5062475085721,5.90808733016712));
#276701=CARTESIAN_POINT('Ctrl Pts',(10.0514385264422,35.6562475085715,3.26591035271534));
#276702=CARTESIAN_POINT('Ctrl Pts',(10.0514385264422,35.8062475085709,-1.23094620182339E-15));
#276703=CARTESIAN_POINT('Ctrl Pts',(10.0514385264422,35.9562475085703,-3.26591035271534));
#276704=CARTESIAN_POINT('Ctrl Pts',(8.1317845858068,36.1062475085696,-5.90808733016713));
#276705=CARTESIAN_POINT('Ctrl Pts',(6.21213064517142,36.256247508569,-8.55026430761891));
#276706=CARTESIAN_POINT('Ctrl Pts',(3.10606532258569,36.4062475085685,-9.55948610871303));
#276707=CARTESIAN_POINT('Ctrl Pts',(-3.41776260538664E-14,36.5562475085678,
-10.5687079098071));
#276708=CARTESIAN_POINT('Ctrl Pts',(-3.10606532258576,36.7062475085672,
-9.55948610871303));
#276709=CARTESIAN_POINT('Ctrl Pts',(-6.21213064517148,36.8562475085666,
-8.55026430761891));
#276710=CARTESIAN_POINT('Ctrl Pts',(-8.13178458580687,37.006247508566,-5.90808733016712));
#276711=CARTESIAN_POINT('Ctrl Pts',(-10.0514385264423,37.1562475085654,
-3.26591035271534));
#276712=CARTESIAN_POINT('Ctrl Pts',(-10.0514385264423,37.3062475085648,
2.46189240364677E-15));
#276713=CARTESIAN_POINT('Ctrl Pts',(-10.0514385264423,37.4562475085642,
3.26591035271534));
#276714=CARTESIAN_POINT('Ctrl Pts',(-8.13178458580687,37.6062475085636,
5.90808733016713));
#276715=CARTESIAN_POINT('Ctrl Pts',(-6.21213064517148,37.756247508563,8.55026430761891));
#276716=CARTESIAN_POINT('Ctrl Pts',(-3.10606532258576,37.9062475085624,
9.55948610871303));
#276717=CARTESIAN_POINT('Ctrl Pts',(-3.24528938271236E-14,38.0562475085619,
10.5687079098071));
#276718=CARTESIAN_POINT('Ctrl Pts',(3.10606532258569,38.2062475085613,9.55948610871303));
#276719=CARTESIAN_POINT('Ctrl Pts',(6.21213064517142,38.3562475085607,8.55026430761891));
#276720=CARTESIAN_POINT('Ctrl Pts',(8.1317845858068,38.5062475085601,5.90808733016712));
#276721=CARTESIAN_POINT('Ctrl Pts',(10.0514385264422,38.6562475085595,3.26591035271534));
#276722=CARTESIAN_POINT('Ctrl Pts',(10.0514385264422,38.8062475085589,-1.23094620182339E-15));
#276723=CARTESIAN_POINT('Ctrl Pts',(10.0514385264422,38.9562475085582,-3.26591035271534));
#276724=CARTESIAN_POINT('Ctrl Pts',(8.1317845858068,39.1062475085576,-5.90808733016713));
#276725=CARTESIAN_POINT('Ctrl Pts',(6.21213064517141,39.2562475085571,-8.55026430761891));
#276726=CARTESIAN_POINT('Ctrl Pts',(3.10606532258569,39.4062475085565,-9.55948610871303));
#276727=CARTESIAN_POINT('Ctrl Pts',(-3.59053353255283E-14,39.5562475085559,
-10.5687079098071));
#276728=CARTESIAN_POINT('Ctrl Pts',(-3.10606532258576,39.7062475085552,
-9.55948610871303));
#276729=CARTESIAN_POINT('Ctrl Pts',(-6.21213064517148,39.8562475085546,
-8.55026430761891));
#276730=CARTESIAN_POINT('Ctrl Pts',(-8.13178458580687,40.0062475085541,
-5.90808733016712));
#276731=CARTESIAN_POINT('Ctrl Pts',(-10.0514385264423,40.1562475085534,
-3.26591035271534));
#276732=CARTESIAN_POINT('Ctrl Pts',(-10.0514385264423,40.3062475085529,
2.46189240364677E-15));
#276733=CARTESIAN_POINT('Ctrl Pts',(-10.0514385264423,40.4562475085523,
3.26591035271534));
#276734=CARTESIAN_POINT('Ctrl Pts',(-8.13178458580687,40.6062475085516,
5.90808733016713));
#276735=CARTESIAN_POINT('Ctrl Pts',(-6.21213064517148,40.756247508551,8.55026430761891));
#276736=CARTESIAN_POINT('Ctrl Pts',(-3.10606532258576,40.9062475085505,
9.55948610871303));
#276737=CARTESIAN_POINT('Ctrl Pts',(-3.41806030987855E-14,41.0562475085499,
10.5687079098071));
#276738=CARTESIAN_POINT('Ctrl Pts',(3.10606532258569,41.2062475085493,9.55948610871303));
#276739=CARTESIAN_POINT('Ctrl Pts',(6.21213064517141,41.3562475085487,8.55026430761891));
#276740=CARTESIAN_POINT('Ctrl Pts',(8.1317845858068,41.5062475085481,5.90808733016712));
#276741=CARTESIAN_POINT('Ctrl Pts',(10.0514385264422,41.6562475085475,3.26591035271534));
#276742=CARTESIAN_POINT('Ctrl Pts',(10.0514385264422,41.8062475085469,-1.23094620182339E-15));
#276743=CARTESIAN_POINT('Ctrl Pts',(10.0514385264422,41.9562475085463,-3.26591035271534));
#276744=CARTESIAN_POINT('Ctrl Pts',(8.1317845858068,42.1062475085457,-5.90808733016713));
#276745=CARTESIAN_POINT('Ctrl Pts',(6.21213064517141,42.256247508545,-8.55026430761891));
#276746=CARTESIAN_POINT('Ctrl Pts',(3.10606532258569,42.4062475085444,-9.55948610871303));
#276747=CARTESIAN_POINT('Ctrl Pts',(-3.76330445971901E-14,42.5562475085438,
-10.5687079098071));
#276748=CARTESIAN_POINT('Ctrl Pts',(-3.10606532258576,42.7062475085432,
-9.55948610871303));
#276749=CARTESIAN_POINT('Ctrl Pts',(-6.21213064517149,42.8562475085426,
-8.55026430761891));
#276750=CARTESIAN_POINT('Ctrl Pts',(-8.13178458580687,43.006247508542,-5.90808733016712));
#276751=CARTESIAN_POINT('Ctrl Pts',(-10.0514385264423,43.1562475085414,
-3.26591035271534));
#276752=CARTESIAN_POINT('Ctrl Pts',(-10.0514385264423,43.3062475085409,
2.46189240364677E-15));
#276753=CARTESIAN_POINT('Ctrl Pts',(-10.0514385264423,43.4562475085402,
3.26591035271534));
#276754=CARTESIAN_POINT('Ctrl Pts',(-8.13178458580687,43.6062475085397,
5.90808733016713));
#276755=CARTESIAN_POINT('Ctrl Pts',(-6.21213064517148,43.756247508539,8.55026430761891));
#276756=CARTESIAN_POINT('Ctrl Pts',(-3.10606532258576,43.9062475085384,
9.55948610871303));
#276757=CARTESIAN_POINT('Ctrl Pts',(-3.59083123704473E-14,44.0562475085379,
10.5687079098071));
#276758=CARTESIAN_POINT('Ctrl Pts',(3.10606532258569,44.2062475085373,9.55948610871303));
#276759=CARTESIAN_POINT('Ctrl Pts',(6.21213064517141,44.3562475085367,8.55026430761891));
#276760=CARTESIAN_POINT('Ctrl Pts',(8.1317845858068,44.5062475085361,5.90808733016712));
#276761=CARTESIAN_POINT('Ctrl Pts',(10.0514385264422,44.6562475085355,3.26591035271534));
#276762=CARTESIAN_POINT('Ctrl Pts',(10.0514385264422,44.8062475085349,-1.23094620182339E-15));
#276763=CARTESIAN_POINT('Ctrl Pts',(10.0514385264422,44.9562475085342,-3.26591035271534));
#276764=CARTESIAN_POINT('Ctrl Pts',(8.13178458580679,45.1062475085337,-5.90808733016713));
#276765=CARTESIAN_POINT('Ctrl Pts',(6.21213064517141,45.2562475085331,-8.55026430761891));
#276766=CARTESIAN_POINT('Ctrl Pts',(3.10606532258569,45.4062475085325,-9.55948610871303));
#276767=CARTESIAN_POINT('Ctrl Pts',(-3.93607538688519E-14,45.5562475085318,
-10.5687079098071));
#276768=CARTESIAN_POINT('Ctrl Pts',(-3.10606532258576,45.7062475085312,
-9.55948610871303));
#276769=CARTESIAN_POINT('Ctrl Pts',(-6.21213064517149,45.8562475085306,
-8.55026430761891));
#276770=CARTESIAN_POINT('Ctrl Pts',(-8.13178458580687,46.0062475085301,
-5.90808733016712));
#276771=CARTESIAN_POINT('Ctrl Pts',(-10.0514385264423,46.1562475085295,
-3.26591035271534));
#276772=CARTESIAN_POINT('Ctrl Pts',(-10.0514385264423,46.3062475085288,
2.46189240364677E-15));
#276773=CARTESIAN_POINT('Ctrl Pts',(-10.0514385264423,46.4562475085283,
3.26591035271534));
#276774=CARTESIAN_POINT('Ctrl Pts',(-8.13178458580687,46.6062475085277,
5.90808733016713));
#276775=CARTESIAN_POINT('Ctrl Pts',(-6.21213064517149,46.756247508527,8.55026430761891));
#276776=CARTESIAN_POINT('Ctrl Pts',(-3.10606532258576,46.9062475085265,
9.55948610871303));
#276777=CARTESIAN_POINT('Ctrl Pts',(-3.76360216421092E-14,47.0562475085259,
10.5687079098071));
#276778=CARTESIAN_POINT('Ctrl Pts',(3.10606532258569,47.2062475085253,9.55948610871303));
#276779=CARTESIAN_POINT('Ctrl Pts',(6.21213064517141,47.3562475085247,8.55026430761891));
#276780=CARTESIAN_POINT('Ctrl Pts',(8.13178458580679,47.5062475085241,5.90808733016712));
#276781=CARTESIAN_POINT('Ctrl Pts',(10.0514385264422,47.6562475085235,3.26591035271534));
#276782=CARTESIAN_POINT('Ctrl Pts',(10.0514385264422,47.8062475085229,-1.23094620182339E-15));
#276783=CARTESIAN_POINT('Ctrl Pts',(10.0514385264422,47.9562475085222,-3.26591035271534));
#276784=CARTESIAN_POINT('Ctrl Pts',(8.13178458580679,48.1062475085216,-5.90808733016713));
#276785=CARTESIAN_POINT('Ctrl Pts',(6.21213064517141,48.256247508521,-8.55026430761891));
#276786=CARTESIAN_POINT('Ctrl Pts',(3.10606532258568,48.4062475085205,-9.55948610871303));
#276787=CARTESIAN_POINT('Ctrl Pts',(-4.10884631405138E-14,48.5562475085198,
-10.5687079098071));
#276788=CARTESIAN_POINT('Ctrl Pts',(-3.10606532258577,48.7062475085193,
-9.55948610871303));
#276789=CARTESIAN_POINT('Ctrl Pts',(-6.21213064517149,48.8562475085186,
-8.55026430761891));
#276790=CARTESIAN_POINT('Ctrl Pts',(-8.13178458580688,49.006247508518,-5.90808733016712));
#276791=CARTESIAN_POINT('Ctrl Pts',(-10.0514385264423,49.1562475085174,
-3.26591035271534));
#276792=CARTESIAN_POINT('Ctrl Pts',(-10.0514385264423,49.3062475085168,
2.46189240364677E-15));
#276793=CARTESIAN_POINT('Ctrl Pts',(-10.0514385264423,49.4562475085162,
3.26591035271534));
#276794=CARTESIAN_POINT('Ctrl Pts',(-8.13178458580688,49.6062475085157,
5.90808733016713));
#276795=CARTESIAN_POINT('Ctrl Pts',(-6.21213064517149,49.7562475085151,
8.55026430761891));
#276796=CARTESIAN_POINT('Ctrl Pts',(-3.10606532258576,49.9062475085144,
9.55948610871303));
#276797=CARTESIAN_POINT('Ctrl Pts',(-3.9363730913771E-14,50.0562475085139,
10.5687079098071));
#276798=CARTESIAN_POINT('Ctrl Pts',(3.10606532258568,50.2062475085133,9.55948610871303));
#276799=CARTESIAN_POINT('Ctrl Pts',(6.21213064517141,50.3562475085127,8.55026430761891));
#276800=CARTESIAN_POINT('Ctrl Pts',(8.13178458580679,50.5062475085121,5.90808733016712));
#276801=CARTESIAN_POINT('Ctrl Pts',(10.0514385264422,50.6562475085115,3.26591035271534));
#276802=CARTESIAN_POINT('Ctrl Pts',(10.0514385264422,50.8062475085109,-1.23094620182339E-15));
#276803=CARTESIAN_POINT('Ctrl Pts',(10.0514385264422,50.9562475085102,-3.26591035271534));
#276804=CARTESIAN_POINT('Ctrl Pts',(8.13178458580679,51.1062475085097,-5.90808733016713));
#276805=CARTESIAN_POINT('Ctrl Pts',(6.21213064517141,51.256247508509,-8.55026430761891));
#276806=CARTESIAN_POINT('Ctrl Pts',(3.10606532258568,51.4062475085084,-9.55948610871303));
#276807=CARTESIAN_POINT('Ctrl Pts',(-4.28161724121756E-14,51.5562475085078,
-10.5687079098071));
#276808=CARTESIAN_POINT('Ctrl Pts',(-3.10606532258577,51.7062475085073,
-9.55948610871303));
#276809=CARTESIAN_POINT('Ctrl Pts',(-6.21213064517149,51.8562475085066,
-8.55026430761891));
#276810=CARTESIAN_POINT('Ctrl Pts',(-8.13178458580688,52.0062475085061,
-5.90808733016712));
#276811=CARTESIAN_POINT('Ctrl Pts',(-10.0514385264423,52.1562475085055,
-3.26591035271534));
#276812=CARTESIAN_POINT('Ctrl Pts',(-10.0514385264423,52.3062475085048,
2.46189240364677E-15));
#276813=CARTESIAN_POINT('Ctrl Pts',(-10.0514385264423,52.4562475085042,
3.26591035271534));
#276814=CARTESIAN_POINT('Ctrl Pts',(-8.13178458580688,52.6062475085036,
5.90808733016713));
#276815=CARTESIAN_POINT('Ctrl Pts',(-6.21213064517149,52.7562475085031,
8.55026430761891));
#276816=CARTESIAN_POINT('Ctrl Pts',(-3.10606532258577,52.9062475085025,
9.55948610871303));
#276817=CARTESIAN_POINT('Ctrl Pts',(-4.10914401854328E-14,53.0562475085018,
10.5687079098071));
#276818=CARTESIAN_POINT('Ctrl Pts',(3.10606532258568,53.2062475085012,9.55948610871303));
#276819=CARTESIAN_POINT('Ctrl Pts',(6.21213064517141,53.3562475085007,8.55026430761891));
#276820=CARTESIAN_POINT('Ctrl Pts',(8.13178458580679,53.5062475085001,5.90808733016712));
#276821=CARTESIAN_POINT('Ctrl Pts',(10.0514385264422,53.6562475084995,3.26591035271534));
#276822=CARTESIAN_POINT('Ctrl Pts',(10.0514385264422,53.8062475084989,-1.23094620182339E-15));
#276823=CARTESIAN_POINT('Ctrl Pts',(10.0514385264422,53.9562475084982,-3.26591035271534));
#276824=CARTESIAN_POINT('Ctrl Pts',(8.13178458580679,54.1062475084976,-5.90808733016713));
#276825=CARTESIAN_POINT('Ctrl Pts',(6.21213064517141,54.2562475084971,-8.55026430761891));
#276826=CARTESIAN_POINT('Ctrl Pts',(3.10606532258568,54.4062475084964,-9.55948610871303));
#276827=CARTESIAN_POINT('Ctrl Pts',(-4.45438816838375E-14,54.5562475084958,
-10.5687079098071));
#276828=CARTESIAN_POINT('Ctrl Pts',(-3.10606532258577,54.7062475084953,
-9.55948610871303));
#276829=CARTESIAN_POINT('Ctrl Pts',(-6.2121306451715,54.8562475084946,-8.55026430761891));
#276830=CARTESIAN_POINT('Ctrl Pts',(-8.13178458580688,55.0062475084941,
-5.90808733016712));
#276831=CARTESIAN_POINT('Ctrl Pts',(-10.0514385264423,55.1562475084934,
-3.26591035271534));
#276832=CARTESIAN_POINT('Ctrl Pts',(-10.0514385264423,55.3062475084929,
2.46189240364677E-15));
#276833=CARTESIAN_POINT('Ctrl Pts',(-10.0514385264423,55.4562475084922,
3.26591035271534));
#276834=CARTESIAN_POINT('Ctrl Pts',(-8.13178458580688,55.6062475084916,
5.90808733016713));
#276835=CARTESIAN_POINT('Ctrl Pts',(-6.21213064517149,55.756247508491,8.55026430761891));
#276836=CARTESIAN_POINT('Ctrl Pts',(-3.10606532258577,55.9062475084905,
9.55948610871303));
#276837=CARTESIAN_POINT('Ctrl Pts',(-4.28191494570947E-14,56.0562475084898,
10.5687079098071));
#276838=CARTESIAN_POINT('Ctrl Pts',(3.10606532258568,56.2062475084893,9.55948610871303));
#276839=CARTESIAN_POINT('Ctrl Pts',(6.21213064517141,56.3562475084887,8.55026430761891));
#276840=CARTESIAN_POINT('Ctrl Pts',(8.13178458580679,56.5062475084881,5.90808733016712));
#276841=CARTESIAN_POINT('Ctrl Pts',(10.0514385264422,56.6562475084875,3.26591035271534));
#276842=CARTESIAN_POINT('Ctrl Pts',(10.0514385264422,56.8062475084869,-1.23094620182339E-15));
#276843=CARTESIAN_POINT('Ctrl Pts',(10.0514385264422,56.9562475084863,-3.26591035271534));
#276844=CARTESIAN_POINT('Ctrl Pts',(8.13178458580679,57.1062475084857,-5.90808733016713));
#276845=CARTESIAN_POINT('Ctrl Pts',(6.2121306451714,57.256247508485,-8.55026430761891));
#276846=CARTESIAN_POINT('Ctrl Pts',(3.10606532258568,57.4062475084844,-9.55948610871303));
#276847=CARTESIAN_POINT('Ctrl Pts',(-4.62715909554993E-14,57.5562475084838,
-10.5687079098071));
#276848=CARTESIAN_POINT('Ctrl Pts',(-3.10606532258577,57.7062475084833,
-9.55948610871303));
#276849=CARTESIAN_POINT('Ctrl Pts',(-6.2121306451715,57.8562475084826,-8.55026430761891));
#276850=CARTESIAN_POINT('Ctrl Pts',(-8.13178458580688,58.006247508482,-5.90808733016712));
#276851=CARTESIAN_POINT('Ctrl Pts',(-10.0514385264423,58.1562475084814,
-3.26591035271534));
#276852=CARTESIAN_POINT('Ctrl Pts',(-10.0514385264423,58.3062475084808,
2.46189240364677E-15));
#276853=CARTESIAN_POINT('Ctrl Pts',(-10.0514385264423,58.4562475084802,
3.26591035271534));
#276854=CARTESIAN_POINT('Ctrl Pts',(-8.13178458580688,58.6062475084797,
5.90808733016713));
#276855=CARTESIAN_POINT('Ctrl Pts',(-6.21213064517149,58.756247508479,8.55026430761891));
#276856=CARTESIAN_POINT('Ctrl Pts',(-3.10606532258577,58.9062475084785,
9.55948610871303));
#276857=CARTESIAN_POINT('Ctrl Pts',(-4.45468587287565E-14,59.0562475084778,
10.5687079098071));
#276858=CARTESIAN_POINT('Ctrl Pts',(3.10606532258568,59.2062475084773,9.55948610871303));
#276859=CARTESIAN_POINT('Ctrl Pts',(6.2121306451714,59.3562475084766,8.55026430761891));
#276860=CARTESIAN_POINT('Ctrl Pts',(8.13178458580679,59.5062475084761,5.90808733016712));
#276861=CARTESIAN_POINT('Ctrl Pts',(10.0514385264422,59.6562475084754,3.26591035271534));
#276862=CARTESIAN_POINT('Ctrl Pts',(10.0514385264422,59.8062475084749,-1.23094620182339E-15));
#276863=CARTESIAN_POINT('Ctrl Pts',(10.0514385264422,59.9562475084742,-3.26591035271534));
#276864=CARTESIAN_POINT('Ctrl Pts',(8.13178458580678,60.1062475084737,-5.90808733016713));
#276865=CARTESIAN_POINT('Ctrl Pts',(6.2121306451714,60.2562475084731,-8.55026430761891));
#276866=CARTESIAN_POINT('Ctrl Pts',(3.10606532258568,60.4062475084725,-9.55948610871303));
#276867=CARTESIAN_POINT('Ctrl Pts',(-4.79993002271612E-14,60.5562475084718,
-10.5687079098071));
#276868=CARTESIAN_POINT('Ctrl Pts',(-3.10606532258577,60.7062475084712,
-9.55948610871303));
#276869=CARTESIAN_POINT('Ctrl Pts',(-6.2121306451715,60.8562475084706,-8.55026430761891));
#276870=CARTESIAN_POINT('Ctrl Pts',(-8.13178458580688,61.00624750847,-5.90808733016712));
#276871=CARTESIAN_POINT('Ctrl Pts',(-10.0514385264423,61.1562475084694,
-3.26591035271534));
#276872=CARTESIAN_POINT('Ctrl Pts',(-10.0514385264423,61.3062475084689,
2.46189240364677E-15));
#276873=CARTESIAN_POINT('Ctrl Pts',(-10.0514385264423,61.4562475084682,
3.26591035271534));
#276874=CARTESIAN_POINT('Ctrl Pts',(-8.13178458580688,61.6062475084676,
5.90808733016713));
#276875=CARTESIAN_POINT('Ctrl Pts',(-6.2121306451715,61.756247508467,8.55026430761891));
#276876=CARTESIAN_POINT('Ctrl Pts',(-3.10606532258577,61.9062475084664,
9.55948610871303));
#276877=CARTESIAN_POINT('Ctrl Pts',(-4.62745680004183E-14,62.0562475084658,
10.5687079098071));
#276878=CARTESIAN_POINT('Ctrl Pts',(3.10606532258568,62.2062475084653,9.55948610871303));
#276879=CARTESIAN_POINT('Ctrl Pts',(6.2121306451714,62.3562475084646,8.55026430761891));
#276880=CARTESIAN_POINT('Ctrl Pts',(8.13178458580678,62.5062475084641,5.90808733016712));
#276881=CARTESIAN_POINT('Ctrl Pts',(10.0514385264422,62.6562475084635,3.26591035271534));
#276882=CARTESIAN_POINT('Ctrl Pts',(10.0514385264422,62.8062475084629,-1.23094620182339E-15));
#276883=CARTESIAN_POINT('Ctrl Pts',(10.0514385264422,62.9562475084623,-3.26591035271534));
#276884=CARTESIAN_POINT('Ctrl Pts',(8.13178458580678,63.1062475084617,-5.90808733016713));
#276885=CARTESIAN_POINT('Ctrl Pts',(6.2121306451714,63.2562475084611,-8.55026430761891));
#276886=CARTESIAN_POINT('Ctrl Pts',(3.10606532258567,63.4062475084604,-9.55948610871303));
#276887=CARTESIAN_POINT('Ctrl Pts',(-4.9727009498823E-14,63.5562475084598,
-10.5687079098071));
#276888=CARTESIAN_POINT('Ctrl Pts',(-3.10606532258578,63.7062475084593,
-9.55948610871303));
#276889=CARTESIAN_POINT('Ctrl Pts',(-6.2121306451715,63.8562475084587,-8.55026430761891));
#276890=CARTESIAN_POINT('Ctrl Pts',(-8.13178458580689,64.006247508458,-5.90808733016712));
#276891=CARTESIAN_POINT('Ctrl Pts',(-10.0514385264423,64.1562475084574,
-3.26591035271534));
#276892=CARTESIAN_POINT('Ctrl Pts',(-10.0514385264423,64.3062475084568,
2.46189240364677E-15));
#276893=CARTESIAN_POINT('Ctrl Pts',(-10.0514385264423,64.4562475084562,
3.26591035271534));
#276894=CARTESIAN_POINT('Ctrl Pts',(-8.13178458580689,64.6062475084557,
5.90808733016713));
#276895=CARTESIAN_POINT('Ctrl Pts',(-6.2121306451715,64.7562475084551,8.55026430761891));
#276896=CARTESIAN_POINT('Ctrl Pts',(-3.10606532258577,64.9062475084545,
9.55948610871303));
#276897=CARTESIAN_POINT('Ctrl Pts',(-4.80022772720802E-14,65.0562475084539,
10.5687079098071));
#276898=CARTESIAN_POINT('Ctrl Pts',(3.10606532258568,65.2062475084533,9.55948610871303));
#276899=CARTESIAN_POINT('Ctrl Pts',(6.2121306451714,65.3562475084527,8.55026430761891));
#276900=CARTESIAN_POINT('Ctrl Pts',(8.13178458580678,65.506247508452,5.90808733016712));
#276901=CARTESIAN_POINT('Ctrl Pts',(10.0514385264422,65.6562475084515,3.26591035271534));
#276902=CARTESIAN_POINT('Ctrl Pts',(10.0514385264422,65.8062475084509,-1.23094620182339E-15));
#276903=CARTESIAN_POINT('Ctrl Pts',(10.0514385264422,65.9562475084503,-3.26591035271534));
#276904=CARTESIAN_POINT('Ctrl Pts',(8.13178458580678,66.1062475084497,-5.90808733016713));
#276905=CARTESIAN_POINT('Ctrl Pts',(6.2121306451714,66.2562475084491,-8.55026430761891));
#276906=CARTESIAN_POINT('Ctrl Pts',(3.10606532258567,66.4062475084485,-9.55948610871303));
#276907=CARTESIAN_POINT('Ctrl Pts',(-5.14547187704848E-14,66.5562475084479,
-10.5687079098071));
#276908=CARTESIAN_POINT('Ctrl Pts',(-3.10606532258578,66.7062475084472,
-9.55948610871303));
#276909=CARTESIAN_POINT('Ctrl Pts',(-6.2121306451715,66.8562475084467,-8.55026430761891));
#276910=CARTESIAN_POINT('Ctrl Pts',(-8.13178458580689,67.0062475084461,
-5.90808733016712));
#276911=CARTESIAN_POINT('Ctrl Pts',(-10.0514385264423,67.1562475084454,
-3.26591035271534));
#276912=CARTESIAN_POINT('Ctrl Pts',(-10.0514385264423,67.3062475084448,
2.46189240364677E-15));
#276913=CARTESIAN_POINT('Ctrl Pts',(-10.0514385264423,67.4562475084442,
3.26591035271534));
#276914=CARTESIAN_POINT('Ctrl Pts',(-8.13178458580689,67.6062475084436,
5.90808733016713));
#276915=CARTESIAN_POINT('Ctrl Pts',(-6.2121306451715,67.7562475084431,8.55026430761891));
#276916=CARTESIAN_POINT('Ctrl Pts',(-3.10606532258578,67.9062475084425,
9.55948610871303));
#276917=CARTESIAN_POINT('Ctrl Pts',(-4.9729986543742E-14,68.0562475084418,
10.5687079098071));
#276918=CARTESIAN_POINT('Ctrl Pts',(3.10606532258567,68.2062475084413,9.55948610871303));
#276919=CARTESIAN_POINT('Ctrl Pts',(6.2121306451714,68.3562475084406,8.55026430761891));
#276920=CARTESIAN_POINT('Ctrl Pts',(8.13178458580678,68.5062475084401,5.90808733016712));
#276921=CARTESIAN_POINT('Ctrl Pts',(10.0514385264422,68.6562475084394,3.26591035271534));
#276922=CARTESIAN_POINT('Ctrl Pts',(10.0514385264422,68.8062475084389,-1.23094620182339E-15));
#276923=CARTESIAN_POINT('Ctrl Pts',(10.0514385264422,68.9562475084383,-3.26591035271534));
#276924=CARTESIAN_POINT('Ctrl Pts',(8.13178458580678,69.1062475084377,-5.90808733016713));
#276925=CARTESIAN_POINT('Ctrl Pts',(6.2121306451714,69.2562475084371,-8.55026430761891));
#276926=CARTESIAN_POINT('Ctrl Pts',(3.10606532258567,69.4062475084365,-9.55948610871303));
#276927=CARTESIAN_POINT('Ctrl Pts',(-5.31824280421467E-14,69.5562475084359,
-10.5687079098071));
#276928=CARTESIAN_POINT('Ctrl Pts',(-3.10606532258578,69.7062475084353,
-9.55948610871303));
#276929=CARTESIAN_POINT('Ctrl Pts',(-6.2121306451715,69.8562475084346,-8.55026430761891));
#276930=CARTESIAN_POINT('Ctrl Pts',(-8.13178458580689,70.006247508434,-5.90808733016712));
#276931=CARTESIAN_POINT('Ctrl Pts',(-10.0514385264423,70.1562475084334,
-3.26591035271534));
#276932=CARTESIAN_POINT('Ctrl Pts',(-10.0514385264423,70.3062475084328,
2.46189240364677E-15));
#276933=CARTESIAN_POINT('Ctrl Pts',(-10.0514385264423,70.4562475084322,
3.26591035271534));
#276934=CARTESIAN_POINT('Ctrl Pts',(-8.13178458580689,70.6062475084316,
5.90808733016713));
#276935=CARTESIAN_POINT('Ctrl Pts',(-6.2121306451715,70.756247508431,8.55026430761891));
#276936=CARTESIAN_POINT('Ctrl Pts',(-3.10606532258578,70.9062475084305,
9.55948610871303));
#276937=CARTESIAN_POINT('Ctrl Pts',(-5.14576958154038E-14,71.0562475084299,
10.5687079098071));
#276938=CARTESIAN_POINT('Ctrl Pts',(3.10606532258567,71.2062475084292,9.55948610871303));
#276939=CARTESIAN_POINT('Ctrl Pts',(6.2121306451714,71.3562475084287,8.55026430761891));
#276940=CARTESIAN_POINT('Ctrl Pts',(8.13178458580678,71.506247508428,5.90808733016712));
#276941=CARTESIAN_POINT('Ctrl Pts',(10.0514385264422,71.6562475084275,3.26591035271534));
#276942=CARTESIAN_POINT('Ctrl Pts',(10.0514385264422,71.8062475084268,-1.23094620182339E-15));
#276943=CARTESIAN_POINT('Ctrl Pts',(10.0514385264422,71.9562475084263,-3.26591035271534));
#276944=CARTESIAN_POINT('Ctrl Pts',(8.13178458580678,72.1062475084257,-5.90808733016713));
#276945=CARTESIAN_POINT('Ctrl Pts',(6.21213064517139,72.2562475084251,-8.55026430761891));
#276946=CARTESIAN_POINT('Ctrl Pts',(3.10606532258567,72.4062475084245,-9.55948610871303));
#276947=CARTESIAN_POINT('Ctrl Pts',(-5.49101373138085E-14,72.5562475084239,
-10.5687079098071));
#276948=CARTESIAN_POINT('Ctrl Pts',(-3.10606532258578,72.7062475084233,
-9.55948610871303));
#276949=CARTESIAN_POINT('Ctrl Pts',(-6.2121306451715,72.8562475084227,-8.55026430761891));
#276950=CARTESIAN_POINT('Ctrl Pts',(-8.13178458580689,73.006247508422,-5.90808733016712));
#276951=CARTESIAN_POINT('Ctrl Pts',(-10.0514385264423,73.1562475084214,
-3.26591035271534));
#276952=CARTESIAN_POINT('Ctrl Pts',(-10.0514385264423,73.3062475084208,
2.46189240364677E-15));
#276953=CARTESIAN_POINT('Ctrl Pts',(-10.0514385264423,73.4562475084202,
3.26591035271534));
#276954=CARTESIAN_POINT('Ctrl Pts',(-8.13178458580689,73.6062475084196,
5.90808733016713));
#276955=CARTESIAN_POINT('Ctrl Pts',(-6.2121306451715,73.7562475084191,8.55026430761891));
#276956=CARTESIAN_POINT('Ctrl Pts',(-3.10606532258578,73.9062475084185,
9.55948610871303));
#276957=CARTESIAN_POINT('Ctrl Pts',(-5.31854050870657E-14,74.0562475084179,
10.5687079098071));
#276958=CARTESIAN_POINT('Ctrl Pts',(3.10606532258567,74.2062475084172,9.55948610871303));
#276959=CARTESIAN_POINT('Ctrl Pts',(6.21213064517139,74.3562475084167,8.55026430761891));
#276960=CARTESIAN_POINT('Ctrl Pts',(8.13178458580678,74.5062475084161,5.90808733016712));
#276961=CARTESIAN_POINT('Ctrl Pts',(10.0514385264422,74.6562475084154,3.26591035271534));
#276962=CARTESIAN_POINT('Ctrl Pts',(10.0514385264422,74.8062475084149,-1.23094620182339E-15));
#276963=CARTESIAN_POINT('Ctrl Pts',(10.0514385264422,74.9562475084143,-3.26591035271534));
#276964=CARTESIAN_POINT('Ctrl Pts',(8.13178458580678,75.1062475084136,-5.90808733016713));
#276965=CARTESIAN_POINT('Ctrl Pts',(6.21213064517139,75.256247508413,-8.55026430761891));
#276966=CARTESIAN_POINT('Ctrl Pts',(3.10606532258567,75.4062475084124,-9.55948610871303));
#276967=CARTESIAN_POINT('Ctrl Pts',(-5.66378465854703E-14,75.5562475084119,
-10.5687079098071));
#276968=CARTESIAN_POINT('Ctrl Pts',(-3.10606532258578,75.7062475084113,
-9.55948610871303));
#276969=CARTESIAN_POINT('Ctrl Pts',(-6.21213064517151,75.8562475084106,
-8.55026430761891));
#276970=CARTESIAN_POINT('Ctrl Pts',(-8.13178458580689,76.00624750841,-5.90808733016712));
#276971=CARTESIAN_POINT('Ctrl Pts',(-10.0514385264423,76.1562475084095,
-3.26591035271534));
#276972=CARTESIAN_POINT('Ctrl Pts',(-10.0514385264423,76.3062475084089,
2.46189240364677E-15));
#276973=CARTESIAN_POINT('Ctrl Pts',(-10.0514385264423,76.4562475084082,
3.26591035271534));
#276974=CARTESIAN_POINT('Ctrl Pts',(-8.13178458580689,76.6062475084076,
5.90808733016713));
#276975=CARTESIAN_POINT('Ctrl Pts',(-6.2121306451715,76.7562475084071,8.55026430761891));
#276976=CARTESIAN_POINT('Ctrl Pts',(-3.10606532258578,76.9062475084065,
9.55948610871303));
#276977=CARTESIAN_POINT('Ctrl Pts',(-5.49131143587276E-14,77.0562475084058,
10.5687079098071));
#276978=CARTESIAN_POINT('Ctrl Pts',(3.10606532258567,77.2062475084053,9.55948610871303));
#276979=CARTESIAN_POINT('Ctrl Pts',(6.21213064517139,77.3562475084047,8.55026430761891));
#276980=CARTESIAN_POINT('Ctrl Pts',(8.13178458580678,77.506247508404,5.90808733016712));
#276981=CARTESIAN_POINT('Ctrl Pts',(10.0514385264422,77.6562475084034,3.26591035271534));
#276982=CARTESIAN_POINT('Ctrl Pts',(10.0514385264422,77.8062475084029,-1.23094620182339E-15));
#276983=CARTESIAN_POINT('Ctrl Pts',(10.0514385264422,77.9562475084023,-3.26591035271534));
#276984=CARTESIAN_POINT('Ctrl Pts',(8.13178458580678,78.1062475084017,-5.90808733016713));
#276985=CARTESIAN_POINT('Ctrl Pts',(6.21213064517139,78.256247508401,-8.55026430761891));
#276986=CARTESIAN_POINT('Ctrl Pts',(3.10606532258567,78.4062475084005,-9.55948610871303));
#276987=CARTESIAN_POINT('Ctrl Pts',(-5.83655558571322E-14,78.5562475083999,
-10.5687079098071));
#276988=CARTESIAN_POINT('Ctrl Pts',(-3.10606532258578,78.7062475083993,
-9.55948610871303));
#276989=CARTESIAN_POINT('Ctrl Pts',(-6.21213064517151,78.8562475083986,
-8.55026430761891));
#276990=CARTESIAN_POINT('Ctrl Pts',(-8.13178458580689,79.006247508398,-5.90808733016712));
#276991=CARTESIAN_POINT('Ctrl Pts',(-10.0514385264423,79.1562475083975,
-3.26591035271534));
#276992=CARTESIAN_POINT('Ctrl Pts',(-10.0514385264423,79.3062475083968,
2.46189240364677E-15));
#276993=CARTESIAN_POINT('Ctrl Pts',(-10.0514385264423,79.4562475083962,
3.26591035271534));
#276994=CARTESIAN_POINT('Ctrl Pts',(-8.13178458580689,79.6062475083957,
5.90808733016713));
#276995=CARTESIAN_POINT('Ctrl Pts',(-6.21213064517151,79.7562475083951,
8.55026430761891));
#276996=CARTESIAN_POINT('Ctrl Pts',(-3.10606532258578,79.9062475083944,
9.55948610871303));
#276997=CARTESIAN_POINT('Ctrl Pts',(-5.66408236303894E-14,80.0562475083938,
10.5687079098071));
#276998=CARTESIAN_POINT('Ctrl Pts',(3.10606532258567,80.2062475083933,9.55948610871303));
#276999=CARTESIAN_POINT('Ctrl Pts',(6.21213064517139,80.3562475083926,8.55026430761891));
#277000=CARTESIAN_POINT('Ctrl Pts',(8.13178458580678,80.5062475083921,5.90808733016712));
#277001=CARTESIAN_POINT('Ctrl Pts',(10.0514385264422,80.6562475083914,3.26591035271534));
#277002=CARTESIAN_POINT('Ctrl Pts',(10.0514385264422,80.8062475083909,-1.23094620182339E-15));
#277003=CARTESIAN_POINT('Ctrl Pts',(10.0514385264422,80.9562475083902,-3.26591035271534));
#277004=CARTESIAN_POINT('Ctrl Pts',(8.13178458580678,81.1062475083897,-5.90808733016713));
#277005=CARTESIAN_POINT('Ctrl Pts',(6.21213064517139,81.256247508389,-8.55026430761891));
#277006=CARTESIAN_POINT('Ctrl Pts',(3.10606532258566,81.4062475083885,-9.55948610871303));
#277007=CARTESIAN_POINT('Ctrl Pts',(-6.0093265128794E-14,81.5562475083879,
-10.5687079098071));
#277008=CARTESIAN_POINT('Ctrl Pts',(-3.10606532258579,81.7062475083873,
-9.55948610871303));
#277009=CARTESIAN_POINT('Ctrl Pts',(-6.21213064517151,81.8562475083866,
-8.55026430761891));
#277010=CARTESIAN_POINT('Ctrl Pts',(-8.13178458580689,82.0062475083861,
-5.90808733016712));
#277011=CARTESIAN_POINT('Ctrl Pts',(-10.0514385264423,82.1562475083854,
-3.26591035271534));
#277012=CARTESIAN_POINT('Ctrl Pts',(-10.0514385264423,82.3062475083849,
2.46189240364677E-15));
#277013=CARTESIAN_POINT('Ctrl Pts',(-10.0514385264423,82.4562475083842,
3.26591035271534));
#277014=CARTESIAN_POINT('Ctrl Pts',(-8.13178458580689,82.6062475083837,
5.90808733016713));
#277015=CARTESIAN_POINT('Ctrl Pts',(-6.21213064517151,82.7562475083831,
8.55026430761891));
#277016=CARTESIAN_POINT('Ctrl Pts',(-3.10606532258578,82.9062475083825,
9.55948610871303));
#277017=CARTESIAN_POINT('Ctrl Pts',(-5.83685329020512E-14,83.0562475083818,
10.5687079098071));
#277018=CARTESIAN_POINT('Ctrl Pts',(3.10606532258567,83.2062475083812,9.55948610871303));
#277019=CARTESIAN_POINT('Ctrl Pts',(6.21213064517139,83.3562475083806,8.55026430761891));
#277020=CARTESIAN_POINT('Ctrl Pts',(8.13178458580677,83.5062475083801,5.90808733016712));
#277021=CARTESIAN_POINT('Ctrl Pts',(10.0514385264422,83.6562475083795,3.26591035271534));
#277022=CARTESIAN_POINT('Ctrl Pts',(10.0514385264422,83.8062475083788,-1.23094620182339E-15));
#277023=CARTESIAN_POINT('Ctrl Pts',(10.0514385264422,83.9562475083783,-3.26591035271534));
#277024=CARTESIAN_POINT('Ctrl Pts',(8.13178458580677,84.1062475083777,-5.90808733016713));
#277025=CARTESIAN_POINT('Ctrl Pts',(6.21213064517139,84.256247508377,-8.55026430761891));
#277026=CARTESIAN_POINT('Ctrl Pts',(3.10606532258566,84.4062475083765,-9.55948610871303));
#277027=CARTESIAN_POINT('Ctrl Pts',(-6.18209744004559E-14,84.5562475083758,
-10.5687079098071));
#277028=CARTESIAN_POINT('Ctrl Pts',(-3.10606532258579,84.7062475083753,
-9.55948610871303));
#277029=CARTESIAN_POINT('Ctrl Pts',(-6.21213064517151,84.8562475083747,
-8.55026430761891));
#277030=CARTESIAN_POINT('Ctrl Pts',(-8.1317845858069,85.006247508374,-5.90808733016712));
#277031=CARTESIAN_POINT('Ctrl Pts',(-10.0514385264423,85.1562475083734,
-3.26591035271534));
#277032=CARTESIAN_POINT('Ctrl Pts',(-10.0514385264423,85.3062475083728,
2.46189240364677E-15));
#277033=CARTESIAN_POINT('Ctrl Pts',(-10.0514385264423,85.4562475083722,
3.26591035271534));
#277034=CARTESIAN_POINT('Ctrl Pts',(-8.1317845858069,85.6062475083716,5.90808733016713));
#277035=CARTESIAN_POINT('Ctrl Pts',(-6.21213064517151,85.7562475083711,
8.55026430761891));
#277036=CARTESIAN_POINT('Ctrl Pts',(-3.10606532258578,85.9062475083705,
9.55948610871303));
#277037=CARTESIAN_POINT('Ctrl Pts',(-6.00962421737131E-14,86.0562475083699,
10.5687079098071));
#277038=CARTESIAN_POINT('Ctrl Pts',(3.10606532258566,86.2062475083693,9.55948610871303));
#277039=CARTESIAN_POINT('Ctrl Pts',(6.21213064517139,86.3562475083687,8.55026430761891));
#277040=CARTESIAN_POINT('Ctrl Pts',(8.13178458580677,86.506247508368,5.90808733016712));
#277041=CARTESIAN_POINT('Ctrl Pts',(10.0514385264422,86.6562475083674,3.26591035271534));
#277042=CARTESIAN_POINT('Ctrl Pts',(10.0514385264422,86.8062475083669,-1.23094620182339E-15));
#277043=CARTESIAN_POINT('Ctrl Pts',(10.0514385264422,86.9562475083663,-3.26591035271534));
#277044=CARTESIAN_POINT('Ctrl Pts',(8.13178458580677,87.1062475083657,-5.90808733016713));
#277045=CARTESIAN_POINT('Ctrl Pts',(6.21213064517139,87.256247508365,-8.55026430761891));
#277046=CARTESIAN_POINT('Ctrl Pts',(3.10606532258566,87.4062475083645,-9.55948610871303));
#277047=CARTESIAN_POINT('Ctrl Pts',(-6.35486836721177E-14,87.5562475083638,
-10.5687079098071));
#277048=CARTESIAN_POINT('Ctrl Pts',(-3.10606532258579,87.7062475083633,
-9.55948610871303));
#277049=CARTESIAN_POINT('Ctrl Pts',(-6.21213064517151,87.8562475083626,
-8.55026430761891));
#277050=CARTESIAN_POINT('Ctrl Pts',(-8.1317845858069,88.0062475083621,-5.90808733016712));
#277051=CARTESIAN_POINT('Ctrl Pts',(-10.0514385264423,88.1562475083614,
-3.26591035271534));
#277052=CARTESIAN_POINT('Ctrl Pts',(-10.0514385264423,88.3062475083609,
2.46189240364677E-15));
#277053=CARTESIAN_POINT('Ctrl Pts',(-10.0514385264423,88.4562475083602,
3.26591035271534));
#277054=CARTESIAN_POINT('Ctrl Pts',(-8.1317845858069,88.6062475083597,5.90808733016713));
#277055=CARTESIAN_POINT('Ctrl Pts',(-6.21213064517151,88.7562475083591,
8.55026430761891));
#277056=CARTESIAN_POINT('Ctrl Pts',(-3.10606532258579,88.9062475083585,
9.55948610871303));
#277057=CARTESIAN_POINT('Ctrl Pts',(-6.18239514453749E-14,89.0562475083578,
10.5687079098071));
#277058=CARTESIAN_POINT('Ctrl Pts',(3.10606532258566,89.2062475083573,9.55948610871303));
#277059=CARTESIAN_POINT('Ctrl Pts',(6.21213064517139,89.3562475083567,8.55026430761891));
#277060=CARTESIAN_POINT('Ctrl Pts',(8.13178458580677,89.5062475083561,5.90808733016712));
#277061=CARTESIAN_POINT('Ctrl Pts',(10.0514385264422,89.6562475083554,3.26591035271534));
#277062=CARTESIAN_POINT('Ctrl Pts',(10.0514385264422,89.8062475083549,-1.23094620182339E-15));
#277063=CARTESIAN_POINT('Ctrl Pts',(10.0514385264422,89.9562475083543,-3.26591035271534));
#277064=CARTESIAN_POINT('Ctrl Pts',(8.13178458580677,90.1062475083536,-5.90808733016713));
#277065=CARTESIAN_POINT('Ctrl Pts',(6.21213064517138,90.256247508353,-8.55026430761891));
#277066=CARTESIAN_POINT('Ctrl Pts',(3.10606532258566,90.4062475083525,-9.55948610871303));
#277067=CARTESIAN_POINT('Ctrl Pts',(-6.52763929437795E-14,90.5562475083518,
-10.5687079098071));
#277068=CARTESIAN_POINT('Ctrl Pts',(-3.10606532258579,90.7062475083512,
-9.55948610871303));
#277069=CARTESIAN_POINT('Ctrl Pts',(-6.21213064517151,90.8562475083506,
-8.55026430761891));
#277070=CARTESIAN_POINT('Ctrl Pts',(-8.1317845858069,91.00624750835,-5.90808733016712));
#277071=CARTESIAN_POINT('Ctrl Pts',(-10.0514385264423,91.1562475083494,
-3.26591035271534));
#277072=CARTESIAN_POINT('Ctrl Pts',(-10.0514385264423,91.3062475083488,
2.46189240364677E-15));
#277073=CARTESIAN_POINT('Ctrl Pts',(-10.0514385264423,91.4562475083482,
3.26591035271534));
#277074=CARTESIAN_POINT('Ctrl Pts',(-8.1317845858069,91.6062475083476,5.90808733016713));
#277075=CARTESIAN_POINT('Ctrl Pts',(-6.21213064517151,91.7562475083471,
8.55026430761891));
#277076=CARTESIAN_POINT('Ctrl Pts',(-3.10606532258579,91.9062475083465,
9.55948610871303));
#277077=CARTESIAN_POINT('Ctrl Pts',(-6.35516607170367E-14,92.0562475083459,
10.5687079098071));
#277078=CARTESIAN_POINT('Ctrl Pts',(3.10606532258566,92.2062475083453,9.55948610871303));
#277079=CARTESIAN_POINT('Ctrl Pts',(6.21213064517139,92.3562475083446,8.55026430761891));
#277080=CARTESIAN_POINT('Ctrl Pts',(8.13178458580677,92.506247508344,5.90808733016712));
#277081=CARTESIAN_POINT('Ctrl Pts',(10.0514385264422,92.6562475083435,3.26591035271534));
#277082=CARTESIAN_POINT('Ctrl Pts',(10.0514385264422,92.8062475083428,-1.23094620182339E-15));
#277083=CARTESIAN_POINT('Ctrl Pts',(10.0514385264422,92.9562475083423,-3.26591035271534));
#277084=CARTESIAN_POINT('Ctrl Pts',(8.13178458580677,93.1062475083417,-5.90808733016713));
#277085=CARTESIAN_POINT('Ctrl Pts',(6.21213064517138,93.256247508341,-8.55026430761891));
#277086=CARTESIAN_POINT('Ctrl Pts',(3.10606532258566,93.4062475083405,-9.55948610871303));
#277087=CARTESIAN_POINT('Ctrl Pts',(-6.70041022154414E-14,93.5562475083398,
-10.5687079098071));
#277088=CARTESIAN_POINT('Ctrl Pts',(-3.10606532258579,93.7062475083393,
-9.55948610871303));
#277089=CARTESIAN_POINT('Ctrl Pts',(-6.21213064517151,93.8562475083386,
-8.55026430761891));
#277090=CARTESIAN_POINT('Ctrl Pts',(-8.1317845858069,94.006247508338,-5.90808733016712));
#277091=CARTESIAN_POINT('Ctrl Pts',(-10.0514385264423,94.1562475083374,
-3.26591035271534));
#277092=CARTESIAN_POINT('Ctrl Pts',(-10.0514385264423,94.3062475083369,
2.46189240364677E-15));
#277093=CARTESIAN_POINT('Ctrl Pts',(-10.0514385264423,94.4562475083362,
3.26591035271534));
#277094=CARTESIAN_POINT('Ctrl Pts',(-8.1317845858069,94.6062475083356,5.90808733016713));
#277095=CARTESIAN_POINT('Ctrl Pts',(-6.21213064517151,94.7562475083351,
8.55026430761891));
#277096=CARTESIAN_POINT('Ctrl Pts',(-3.10606532258579,94.9062475083345,
9.55948610871303));
#277097=CARTESIAN_POINT('Ctrl Pts',(-6.52793699886986E-14,95.0562475083338,
10.5687079098071));
#277098=CARTESIAN_POINT('Ctrl Pts',(3.10606532258566,95.2062475083333,9.55948610871303));
#277099=CARTESIAN_POINT('Ctrl Pts',(6.21213064517138,95.3562475083327,8.55026430761891));
#277100=CARTESIAN_POINT('Ctrl Pts',(8.13178458580677,95.5062475083321,5.90808733016712));
#277101=CARTESIAN_POINT('Ctrl Pts',(10.0514385264422,95.6562475083314,3.26591035271534));
#277102=CARTESIAN_POINT('Ctrl Pts',(10.0514385264422,95.8062475083309,-1.23094620182339E-15));
#277103=CARTESIAN_POINT('Ctrl Pts',(10.0514385264422,95.9562475083303,-3.26591035271534));
#277104=CARTESIAN_POINT('Ctrl Pts',(8.13178458580677,96.1062475083297,-5.90808733016713));
#277105=CARTESIAN_POINT('Ctrl Pts',(6.21213064517138,96.2562475083291,-8.55026430761891));
#277106=CARTESIAN_POINT('Ctrl Pts',(3.10606532258566,96.4062475083284,-9.55948610871303));
#277107=CARTESIAN_POINT('Ctrl Pts',(-6.87318114871032E-14,96.5562475083278,
-10.5687079098071));
#277108=CARTESIAN_POINT('Ctrl Pts',(-3.10606532258579,96.7062475083272,
-9.55948610871303));
#277109=CARTESIAN_POINT('Ctrl Pts',(-6.21213064517152,96.8562475083267,
-8.55026430761891));
#277110=CARTESIAN_POINT('Ctrl Pts',(-8.1317845858069,97.0062475083261,-5.90808733016712));
#277111=CARTESIAN_POINT('Ctrl Pts',(-10.0514385264423,97.1562475083254,
-3.26591035271534));
#277112=CARTESIAN_POINT('Ctrl Pts',(-10.0514385264423,97.3062475083248,
2.46189240364677E-15));
#277113=CARTESIAN_POINT('Ctrl Pts',(-10.0514385264423,97.4562475083242,
3.26591035271534));
#277114=CARTESIAN_POINT('Ctrl Pts',(-8.1317845858069,97.6062475083236,5.90808733016713));
#277115=CARTESIAN_POINT('Ctrl Pts',(-6.21213064517151,97.7562475083231,
8.55026430761891));
#277116=CARTESIAN_POINT('Ctrl Pts',(-3.10606532258579,97.9062475083225,
9.55948610871303));
#277117=CARTESIAN_POINT('Ctrl Pts',(-6.70070792603604E-14,98.0562475083219,
10.5687079098071));
#277118=CARTESIAN_POINT('Ctrl Pts',(3.10606532258566,98.2062475083213,9.55948610871303));
#277119=CARTESIAN_POINT('Ctrl Pts',(6.21213064517138,98.3562475083206,8.55026430761891));
#277120=CARTESIAN_POINT('Ctrl Pts',(8.13178458580676,98.5062475083201,5.90808733016712));
#277121=CARTESIAN_POINT('Ctrl Pts',(10.0514385264422,98.6562475083194,3.26591035271534));
#277122=CARTESIAN_POINT('Ctrl Pts',(10.0514385264422,98.8062475083189,-1.23094620182339E-15));
#277123=CARTESIAN_POINT('Ctrl Pts',(10.0514385264421,98.9562475083183,-3.26591035271534));
#277124=CARTESIAN_POINT('Ctrl Pts',(8.13178458580676,99.1062475083177,-5.90808733016713));
#277125=CARTESIAN_POINT('Ctrl Pts',(6.21213064517138,99.256247508317,-8.55026430761891));
#277126=CARTESIAN_POINT('Ctrl Pts',(3.10606532258565,99.4062475083165,-9.55948610871303));
#277127=CARTESIAN_POINT('Ctrl Pts',(-7.0459520758765E-14,99.5562475083159,
-10.5687079098071));
#277128=CARTESIAN_POINT('Ctrl Pts',(-3.1060653225858,99.7062475083153,-9.55948610871303));
#277129=CARTESIAN_POINT('Ctrl Pts',(-6.21213064517152,99.8562475083146,
-8.55026430761891));
#277130=CARTESIAN_POINT('Ctrl Pts',(-8.1317845858069,100.006247508314,-5.90808733016712));
#277131=CARTESIAN_POINT('Ctrl Pts',(-10.0514385264423,100.156247508313,
-3.26591035271534));
#277132=CARTESIAN_POINT('Ctrl Pts',(-10.0514385264423,100.306247508313,
2.46189240364677E-15));
#277133=CARTESIAN_POINT('Ctrl Pts',(-10.0514385264423,100.456247508312,
3.26591035271534));
#277134=CARTESIAN_POINT('Ctrl Pts',(-8.1317845858069,100.606247508312,5.90808733016713));
#277135=CARTESIAN_POINT('Ctrl Pts',(-6.21213064517152,100.756247508311,
8.55026430761891));
#277136=CARTESIAN_POINT('Ctrl Pts',(-3.10606532258579,100.90624750831,9.55948610871303));
#277137=CARTESIAN_POINT('Ctrl Pts',(-6.87347885320222E-14,101.05624750831,
10.5687079098071));
#277138=CARTESIAN_POINT('Ctrl Pts',(3.10606532258566,101.206247508309,9.55948610871303));
#277139=CARTESIAN_POINT('Ctrl Pts',(6.21213064517138,101.356247508309,8.55026430761891));
#277140=CARTESIAN_POINT('Ctrl Pts',(8.13178458580676,101.506247508308,5.90808733016712));
#277141=CARTESIAN_POINT('Ctrl Pts',(10.0514385264421,101.656247508307,3.26591035271534));
#277142=CARTESIAN_POINT('Ctrl Pts',(10.0514385264421,101.806247508307,-1.23094620182339E-15));
#277143=CARTESIAN_POINT('Ctrl Pts',(10.0514385264421,101.956247508306,-3.26591035271534));
#277144=CARTESIAN_POINT('Ctrl Pts',(8.13178458580676,102.106247508306,-5.90808733016713));
#277145=CARTESIAN_POINT('Ctrl Pts',(6.21213064517138,102.256247508305,-8.55026430761891));
#277146=CARTESIAN_POINT('Ctrl Pts',(3.10606532258565,102.406247508304,-9.55948610871303));
#277147=CARTESIAN_POINT('Ctrl Pts',(-7.21872300304269E-14,102.556247508304,
-10.5687079098071));
#277148=CARTESIAN_POINT('Ctrl Pts',(-3.1060653225858,102.706247508303,-9.55948610871303));
#277149=CARTESIAN_POINT('Ctrl Pts',(-6.21213064517152,102.856247508303,
-8.55026430761891));
#277150=CARTESIAN_POINT('Ctrl Pts',(-8.13178458580691,103.006247508302,
-5.90808733016712));
#277151=CARTESIAN_POINT('Ctrl Pts',(-10.0514385264423,103.156247508301,
-3.26591035271534));
#277152=CARTESIAN_POINT('Ctrl Pts',(-10.0514385264423,103.306247508301,
2.46189240364677E-15));
#277153=CARTESIAN_POINT('Ctrl Pts',(-10.0514385264423,103.4562475083,3.26591035271534));
#277154=CARTESIAN_POINT('Ctrl Pts',(-8.13178458580691,103.6062475083,5.90808733016713));
#277155=CARTESIAN_POINT('Ctrl Pts',(-6.21213064517152,103.756247508299,
8.55026430761891));
#277156=CARTESIAN_POINT('Ctrl Pts',(-3.1060653225858,103.906247508298,9.55948610871303));
#277157=CARTESIAN_POINT('Ctrl Pts',(-7.04624978036841E-14,104.056247508298,
10.5687079098071));
#277158=CARTESIAN_POINT('Ctrl Pts',(3.10606532258565,104.206247508297,9.55948610871303));
#277159=CARTESIAN_POINT('Ctrl Pts',(6.21213064517138,104.356247508297,8.55026430761891));
#277160=CARTESIAN_POINT('Ctrl Pts',(8.13178458580676,104.506247508296,5.90808733016712));
#277161=CARTESIAN_POINT('Ctrl Pts',(10.0514385264421,104.656247508295,3.26591035271534));
#277162=CARTESIAN_POINT('Ctrl Pts',(10.0514385264421,104.806247508295,-1.23094620182339E-15));
#277163=CARTESIAN_POINT('Ctrl Pts',(10.0514385264421,104.956247508294,-3.26591035271534));
#277164=CARTESIAN_POINT('Ctrl Pts',(8.13178458580676,105.106247508294,-5.90808733016713));
#277165=CARTESIAN_POINT('Ctrl Pts',(6.21213064517137,105.256247508293,-8.55026430761891));
#277166=CARTESIAN_POINT('Ctrl Pts',(3.10606532258565,105.406247508292,-9.55948610871303));
#277167=CARTESIAN_POINT('Ctrl Pts',(-7.39149393020888E-14,105.556247508292,
-10.5687079098071));
#277168=CARTESIAN_POINT('Ctrl Pts',(-3.1060653225858,105.706247508291,-9.55948610871303));
#277169=CARTESIAN_POINT('Ctrl Pts',(-6.21213064517152,105.856247508291,
-8.55026430761891));
#277170=CARTESIAN_POINT('Ctrl Pts',(-8.13178458580691,106.00624750829,-5.90808733016712));
#277171=CARTESIAN_POINT('Ctrl Pts',(-10.0514385264423,106.156247508289,
-3.26591035271534));
#277172=CARTESIAN_POINT('Ctrl Pts',(-10.0514385264423,106.306247508289,
2.46189240364677E-15));
#277173=CARTESIAN_POINT('Ctrl Pts',(-10.0514385264423,106.456247508288,
3.26591035271534));
#277174=CARTESIAN_POINT('Ctrl Pts',(-8.13178458580691,106.606247508288,
5.90808733016713));
#277175=CARTESIAN_POINT('Ctrl Pts',(-6.21213064517152,106.756247508287,
8.55026430761891));
#277176=CARTESIAN_POINT('Ctrl Pts',(-3.1060653225858,106.906247508286,9.55948610871303));
#277177=CARTESIAN_POINT('Ctrl Pts',(-7.21902070753459E-14,107.056247508286,
10.5687079098071));
#277178=CARTESIAN_POINT('Ctrl Pts',(3.10606532258565,107.206247508285,9.55948610871303));
#277179=CARTESIAN_POINT('Ctrl Pts',(6.21213064517138,107.356247508285,8.55026430761891));
#277180=CARTESIAN_POINT('Ctrl Pts',(8.13178458580676,107.506247508284,5.90808733016712));
#277181=CARTESIAN_POINT('Ctrl Pts',(10.0514385264421,107.656247508283,3.26591035271534));
#277182=CARTESIAN_POINT('Ctrl Pts',(10.0514385264421,107.806247508283,-1.23094620182339E-15));
#277183=CARTESIAN_POINT('Ctrl Pts',(10.0514385264421,107.956247508282,-3.26591035271534));
#277184=CARTESIAN_POINT('Ctrl Pts',(8.13178458580676,108.106247508282,-5.90808733016713));
#277185=CARTESIAN_POINT('Ctrl Pts',(6.21213064517137,108.256247508281,-8.55026430761891));
#277186=CARTESIAN_POINT('Ctrl Pts',(3.10606532258565,108.40624750828,-9.55948610871303));
#277187=CARTESIAN_POINT('Ctrl Pts',(-7.56426485737506E-14,108.55624750828,
-10.5687079098071));
#277188=CARTESIAN_POINT('Ctrl Pts',(-3.1060653225858,108.706247508279,-9.55948610871303));
#277189=CARTESIAN_POINT('Ctrl Pts',(-6.21213064517153,108.856247508279,
-8.55026430761891));
#277190=CARTESIAN_POINT('Ctrl Pts',(-8.13178458580691,109.006247508278,
-5.90808733016712));
#277191=CARTESIAN_POINT('Ctrl Pts',(-10.0514385264423,109.156247508277,
-3.26591035271534));
#277192=CARTESIAN_POINT('Ctrl Pts',(-10.0514385264423,109.306247508277,
2.46189240364677E-15));
#277193=CARTESIAN_POINT('Ctrl Pts',(-10.0514385264423,109.456247508276,
3.26591035271534));
#277194=CARTESIAN_POINT('Ctrl Pts',(-8.13178458580691,109.606247508276,
5.90808733016713));
#277195=CARTESIAN_POINT('Ctrl Pts',(-6.21213064517152,109.756247508275,
8.55026430761891));
#277196=CARTESIAN_POINT('Ctrl Pts',(-3.1060653225858,109.906247508274,9.55948610871303));
#277197=CARTESIAN_POINT('Ctrl Pts',(-7.39179163470078E-14,110.056247508274,
10.5687079098071));
#277198=CARTESIAN_POINT('Ctrl Pts',(3.10606532258565,110.206247508273,9.55948610871303));
#277199=CARTESIAN_POINT('Ctrl Pts',(6.21213064517137,110.356247508273,8.55026430761891));
#277200=CARTESIAN_POINT('Ctrl Pts',(8.13178458580676,110.506247508272,5.90808733016712));
#277201=CARTESIAN_POINT('Ctrl Pts',(10.0514385264421,110.656247508271,3.26591035271534));
#277202=CARTESIAN_POINT('Ctrl Pts',(10.0514385264421,110.806247508271,-1.23094620182339E-15));
#277203=CARTESIAN_POINT('Ctrl Pts',(10.0514385264421,110.95624750827,-3.26591035271534));
#277204=CARTESIAN_POINT('Ctrl Pts',(8.13178458580676,111.10624750827,-5.90808733016713));
#277205=CARTESIAN_POINT('Ctrl Pts',(6.21213064517137,111.256247508269,-8.55026430761891));
#277206=CARTESIAN_POINT('Ctrl Pts',(3.10606532258565,111.406247508268,-9.55948610871303));
#277207=CARTESIAN_POINT('Ctrl Pts',(-7.73703578454124E-14,111.556247508268,
-10.5687079098071));
#277208=CARTESIAN_POINT('Ctrl Pts',(-3.1060653225858,111.706247508267,-9.55948610871303));
#277209=CARTESIAN_POINT('Ctrl Pts',(-6.21213064517153,111.856247508267,
-8.55026430761891));
#277210=CARTESIAN_POINT('Ctrl Pts',(-8.13178458580691,112.006247508266,
-5.90808733016712));
#277211=CARTESIAN_POINT('Ctrl Pts',(-10.0514385264423,112.156247508265,
-3.26591035271534));
#277212=CARTESIAN_POINT('Ctrl Pts',(-10.0514385264423,112.306247508265,
2.46189240364677E-15));
#277213=CARTESIAN_POINT('Ctrl Pts',(-10.0514385264423,112.456247508264,
3.26591035271534));
#277214=CARTESIAN_POINT('Ctrl Pts',(-8.13178458580691,112.606247508264,
5.90808733016713));
#277215=CARTESIAN_POINT('Ctrl Pts',(-6.21213064517153,112.756247508263,
8.55026430761891));
#277216=CARTESIAN_POINT('Ctrl Pts',(-3.1060653225858,112.906247508262,9.55948610871303));
#277217=CARTESIAN_POINT('Ctrl Pts',(-7.56456256186696E-14,113.056247508262,
10.5687079098071));
#277218=CARTESIAN_POINT('Ctrl Pts',(3.10606532258565,113.206247508261,9.55948610871303));
#277219=CARTESIAN_POINT('Ctrl Pts',(6.21213064517137,113.356247508261,8.55026430761891));
#277220=CARTESIAN_POINT('Ctrl Pts',(8.13178458580676,113.50624750826,5.90808733016712));
#277221=CARTESIAN_POINT('Ctrl Pts',(10.0514385264421,113.656247508259,3.26591035271534));
#277222=CARTESIAN_POINT('Ctrl Pts',(10.0514385264421,113.806247508259,-1.23094620182339E-15));
#277223=CARTESIAN_POINT('Ctrl Pts',(10.0514385264421,113.956247508258,-3.26591035271534));
#277224=CARTESIAN_POINT('Ctrl Pts',(8.13178458580676,114.106247508258,-5.90808733016713));
#277225=CARTESIAN_POINT('Ctrl Pts',(6.21213064517137,114.256247508257,-8.55026430761891));
#277226=CARTESIAN_POINT('Ctrl Pts',(3.10606532258565,114.406247508256,-9.55948610871303));
#277227=CARTESIAN_POINT('Ctrl Pts',(-7.90980671170742E-14,114.556247508256,
-10.5687079098071));
#277228=CARTESIAN_POINT('Ctrl Pts',(-3.1060653225858,114.706247508255,-9.55948610871303));
#277229=CARTESIAN_POINT('Ctrl Pts',(-6.21213064517153,114.856247508255,
-8.55026430761891));
#277230=CARTESIAN_POINT('Ctrl Pts',(-8.13178458580691,115.006247508254,
-5.90808733016712));
#277231=CARTESIAN_POINT('Ctrl Pts',(-10.0514385264423,115.156247508253,
-3.26591035271534));
#277232=CARTESIAN_POINT('Ctrl Pts',(-10.0514385264423,115.306247508253,
2.46189240364677E-15));
#277233=CARTESIAN_POINT('Ctrl Pts',(-10.0514385264423,115.456247508252,
3.26591035271534));
#277234=CARTESIAN_POINT('Ctrl Pts',(-8.13178458580691,115.606247508252,
5.90808733016713));
#277235=CARTESIAN_POINT('Ctrl Pts',(-6.21213064517153,115.756247508251,
8.55026430761891));
#277236=CARTESIAN_POINT('Ctrl Pts',(-3.1060653225858,115.90624750825,9.55948610871303));
#277237=CARTESIAN_POINT('Ctrl Pts',(-7.73733348903315E-14,116.05624750825,
10.5687079098071));
#277238=CARTESIAN_POINT('Ctrl Pts',(3.10606532258565,116.206247508249,9.55948610871303));
#277239=CARTESIAN_POINT('Ctrl Pts',(6.21213064517137,116.356247508249,8.55026430761891));
#277240=CARTESIAN_POINT('Ctrl Pts',(8.13178458580676,116.506247508248,5.90808733016712));
#277241=CARTESIAN_POINT('Ctrl Pts',(10.0514385264421,116.656247508247,3.26591035271534));
#277242=CARTESIAN_POINT('Ctrl Pts',(10.0514385264421,116.806247508247,-1.23094620182339E-15));
#277243=CARTESIAN_POINT('Ctrl Pts',(10.0514385264421,116.956247508246,-3.26591035271534));
#277244=CARTESIAN_POINT('Ctrl Pts',(8.13178458580676,117.106247508246,-5.90808733016713));
#277245=CARTESIAN_POINT('Ctrl Pts',(6.21213064517137,117.256247508245,-8.55026430761891));
#277246=CARTESIAN_POINT('Ctrl Pts',(3.10606532258564,117.406247508244,-9.55948610871303));
#277247=CARTESIAN_POINT('Ctrl Pts',(-8.08257763887361E-14,117.556247508244,
-10.5687079098071));
#277248=CARTESIAN_POINT('Ctrl Pts',(-3.10606532258581,117.706247508243,
-9.55948610871303));
#277249=CARTESIAN_POINT('Ctrl Pts',(-6.21213064517153,117.856247508243,
-8.55026430761891));
#277250=CARTESIAN_POINT('Ctrl Pts',(-8.13178458580692,118.006247508242,
-5.90808733016712));
#277251=CARTESIAN_POINT('Ctrl Pts',(-10.0514385264423,118.156247508241,
-3.26591035271534));
#277252=CARTESIAN_POINT('Ctrl Pts',(-10.0514385264423,118.306247508241,
2.46189240364677E-15));
#277253=CARTESIAN_POINT('Ctrl Pts',(-10.0514385264423,118.45624750824,3.26591035271534));
#277254=CARTESIAN_POINT('Ctrl Pts',(-8.13178458580692,118.60624750824,5.90808733016713));
#277255=CARTESIAN_POINT('Ctrl Pts',(-6.21213064517153,118.756247508239,
8.55026430761891));
#277256=CARTESIAN_POINT('Ctrl Pts',(-3.1060653225858,118.906247508238,9.55948610871303));
#277257=CARTESIAN_POINT('Ctrl Pts',(-7.91010441619933E-14,119.056247508238,
10.5687079098071));
#277258=CARTESIAN_POINT('Ctrl Pts',(3.10606532258564,119.206247508237,9.55948610871303));
#277259=CARTESIAN_POINT('Ctrl Pts',(6.21213064517137,119.356247508237,8.55026430761891));
#277260=CARTESIAN_POINT('Ctrl Pts',(8.13178458580675,119.506247508236,5.90808733016712));
#277261=CARTESIAN_POINT('Ctrl Pts',(10.0514385264421,119.656247508235,3.26591035271534));
#277262=CARTESIAN_POINT('Ctrl Pts',(10.0514385264421,119.806247508235,-1.23094620182339E-15));
#277263=CARTESIAN_POINT('Ctrl Pts',(10.0514385264421,119.956247508234,-3.26591035271534));
#277264=CARTESIAN_POINT('Ctrl Pts',(8.13178458580675,120.106247508234,-5.90808733016713));
#277265=CARTESIAN_POINT('Ctrl Pts',(6.21213064517137,120.256247508233,-8.55026430761891));
#277266=CARTESIAN_POINT('Ctrl Pts',(3.10606532258564,120.406247508232,-9.55948610871303));
#277267=CARTESIAN_POINT('Ctrl Pts',(-8.25534856603979E-14,120.556247508232,
-10.5687079098071));
#277268=CARTESIAN_POINT('Ctrl Pts',(-3.10606532258581,120.706247508231,
-9.55948610871303));
#277269=CARTESIAN_POINT('Ctrl Pts',(-6.21213064517153,120.856247508231,
-8.55026430761891));
#277270=CARTESIAN_POINT('Ctrl Pts',(-8.13178458580692,121.00624750823,-5.90808733016712));
#277271=CARTESIAN_POINT('Ctrl Pts',(-10.0514385264423,121.156247508229,
-3.26591035271534));
#277272=CARTESIAN_POINT('Ctrl Pts',(-10.0514385264423,121.306247508229,
2.46189240364677E-15));
#277273=CARTESIAN_POINT('Ctrl Pts',(-10.0514385264423,121.456247508228,
3.26591035271534));
#277274=CARTESIAN_POINT('Ctrl Pts',(-8.13178458580692,121.606247508228,
5.90808733016713));
#277275=CARTESIAN_POINT('Ctrl Pts',(-6.21213064517153,121.756247508227,
8.55026430761891));
#277276=CARTESIAN_POINT('Ctrl Pts',(-3.10606532258581,121.906247508226,
9.55948610871303));
#277277=CARTESIAN_POINT('Ctrl Pts',(-8.08287534336551E-14,122.056247508226,
10.5687079098071));
#277278=CARTESIAN_POINT('Ctrl Pts',(3.10606532258564,122.206247508225,9.55948610871303));
#277279=CARTESIAN_POINT('Ctrl Pts',(6.21213064517137,122.356247508225,8.55026430761891));
#277280=CARTESIAN_POINT('Ctrl Pts',(8.13178458580675,122.506247508224,5.90808733016712));
#277281=CARTESIAN_POINT('Ctrl Pts',(10.0514385264421,122.656247508223,3.26591035271534));
#277282=CARTESIAN_POINT('Ctrl Pts',(10.0514385264421,122.806247508223,-1.23094620182339E-15));
#277283=CARTESIAN_POINT('Ctrl Pts',(10.0514385264421,122.956247508222,-3.26591035271534));
#277284=CARTESIAN_POINT('Ctrl Pts',(8.13178458580675,123.106247508222,-5.90808733016713));
#277285=CARTESIAN_POINT('Ctrl Pts',(6.21213064517137,123.256247508221,-8.55026430761891));
#277286=CARTESIAN_POINT('Ctrl Pts',(3.10606532258564,123.40624750822,-9.55948610871303));
#277287=CARTESIAN_POINT('Ctrl Pts',(-8.42811949320597E-14,123.55624750822,
-10.5687079098071));
#277288=CARTESIAN_POINT('Ctrl Pts',(-3.10606532258581,123.706247508219,
-9.55948610871303));
#277289=CARTESIAN_POINT('Ctrl Pts',(-6.21213064517153,123.856247508219,
-8.55026430761891));
#277290=CARTESIAN_POINT('Ctrl Pts',(-8.13178458580692,124.006247508218,
-5.90808733016712));
#277291=CARTESIAN_POINT('Ctrl Pts',(-10.0514385264423,124.156247508217,
-3.26591035271534));
#277292=CARTESIAN_POINT('Ctrl Pts',(-10.0514385264423,124.306247508217,
2.46189240364677E-15));
#277293=CARTESIAN_POINT('Ctrl Pts',(-10.0514385264423,124.456247508216,
3.26591035271534));
#277294=CARTESIAN_POINT('Ctrl Pts',(-8.13178458580692,124.606247508216,
5.90808733016713));
#277295=CARTESIAN_POINT('Ctrl Pts',(-6.21213064517153,124.756247508215,
8.55026430761891));
#277296=CARTESIAN_POINT('Ctrl Pts',(-3.10606532258581,124.906247508214,
9.55948610871303));
#277297=CARTESIAN_POINT('Ctrl Pts',(-8.25564627053169E-14,125.056247508214,
10.5687079098071));
#277298=CARTESIAN_POINT('Ctrl Pts',(3.10606532258564,125.206247508213,9.55948610871303));
#277299=CARTESIAN_POINT('Ctrl Pts',(6.21213064517137,125.356247508213,8.55026430761891));
#277300=CARTESIAN_POINT('Ctrl Pts',(8.13178458580675,125.506247508212,5.90808733016712));
#277301=CARTESIAN_POINT('Ctrl Pts',(10.0514385264421,125.656247508211,3.26591035271534));
#277302=CARTESIAN_POINT('Ctrl Pts',(10.0514385264421,125.806247508211,-1.23094620182339E-15));
#277303=CARTESIAN_POINT('Ctrl Pts',(10.0514385264421,125.95624750821,-3.26591035271534));
#277304=CARTESIAN_POINT('Ctrl Pts',(8.13178458580675,126.10624750821,-5.90808733016713));
#277305=CARTESIAN_POINT('Ctrl Pts',(6.21213064517136,126.256247508209,-8.55026430761891));
#277306=CARTESIAN_POINT('Ctrl Pts',(3.10606532258564,126.406247508208,-9.55948610871303));
#277307=CARTESIAN_POINT('Ctrl Pts',(-8.60089042037216E-14,126.556247508208,
-10.5687079098071));
#277308=CARTESIAN_POINT('Ctrl Pts',(-3.10606532258581,126.706247508207,
-9.55948610871303));
#277309=CARTESIAN_POINT('Ctrl Pts',(-6.21213064517153,126.856247508207,
-8.55026430761891));
#277310=CARTESIAN_POINT('Ctrl Pts',(-8.13178458580692,127.006247508206,
-5.90808733016712));
#277311=CARTESIAN_POINT('Ctrl Pts',(-10.0514385264423,127.156247508205,
-3.26591035271534));
#277312=CARTESIAN_POINT('Ctrl Pts',(-10.0514385264423,127.306247508205,
2.46189240364677E-15));
#277313=CARTESIAN_POINT('Ctrl Pts',(-10.0514385264423,127.456247508204,
3.26591035271534));
#277314=CARTESIAN_POINT('Ctrl Pts',(-8.13178458580692,127.606247508204,
5.90808733016713));
#277315=CARTESIAN_POINT('Ctrl Pts',(-6.21213064517153,127.756247508203,
8.55026430761891));
#277316=CARTESIAN_POINT('Ctrl Pts',(-3.10606532258581,127.906247508202,
9.55948610871303));
#277317=CARTESIAN_POINT('Ctrl Pts',(-8.42841719769788E-14,128.056247508202,
10.5687079098071));
#277318=CARTESIAN_POINT('Ctrl Pts',(3.10606532258564,128.206247508201,9.55948610871303));
#277319=CARTESIAN_POINT('Ctrl Pts',(6.21213064517137,128.356247508201,8.55026430761891));
#277320=CARTESIAN_POINT('Ctrl Pts',(8.13178458580675,128.5062475082,5.90808733016712));
#277321=CARTESIAN_POINT('Ctrl Pts',(10.0514385264421,128.656247508199,3.26591035271534));
#277322=CARTESIAN_POINT('Ctrl Pts',(10.0514385264421,128.806247508199,-1.23094620182339E-15));
#277323=CARTESIAN_POINT('Ctrl Pts',(10.0514385264421,128.956247508198,-3.26591035271534));
#277324=CARTESIAN_POINT('Ctrl Pts',(8.13178458580675,129.106247508198,-5.90808733016713));
#277325=CARTESIAN_POINT('Ctrl Pts',(6.21213064517136,129.256247508197,-8.55026430761891));
#277326=CARTESIAN_POINT('Ctrl Pts',(3.10606532258564,129.406247508196,-9.55948610871303));
#277327=CARTESIAN_POINT('Ctrl Pts',(-8.77366134753835E-14,129.556247508196,
-10.5687079098071));
#277328=CARTESIAN_POINT('Ctrl Pts',(-3.10606532258581,129.706247508195,
-9.55948610871303));
#277329=CARTESIAN_POINT('Ctrl Pts',(-6.21213064517154,129.856247508195,
-8.55026430761891));
#277330=CARTESIAN_POINT('Ctrl Pts',(-8.13178458580692,130.006247508194,
-5.90808733016712));
#277331=CARTESIAN_POINT('Ctrl Pts',(-10.0514385264423,130.156247508193,
-3.26591035271534));
#277332=CARTESIAN_POINT('Ctrl Pts',(-10.0514385264423,130.306247508193,
2.46189240364677E-15));
#277333=CARTESIAN_POINT('Ctrl Pts',(-10.0514385264423,130.456247508192,
3.26591035271534));
#277334=CARTESIAN_POINT('Ctrl Pts',(-8.13178458580692,130.606247508192,
5.90808733016713));
#277335=CARTESIAN_POINT('Ctrl Pts',(-6.21213064517153,130.756247508191,
8.55026430761891));
#277336=CARTESIAN_POINT('Ctrl Pts',(-3.10606532258581,130.90624750819,9.55948610871303));
#277337=CARTESIAN_POINT('Ctrl Pts',(-8.60118812486407E-14,131.05624750819,
10.5687079098071));
#277338=CARTESIAN_POINT('Ctrl Pts',(3.10606532258564,131.206247508189,9.55948610871303));
#277339=CARTESIAN_POINT('Ctrl Pts',(6.21213064517136,131.356247508189,8.55026430761891));
#277340=CARTESIAN_POINT('Ctrl Pts',(8.13178458580675,131.506247508188,5.90808733016712));
#277341=CARTESIAN_POINT('Ctrl Pts',(10.0514385264421,131.656247508187,3.26591035271534));
#277342=CARTESIAN_POINT('Ctrl Pts',(10.0514385264421,131.806247508187,-1.23094620182339E-15));
#277343=CARTESIAN_POINT('Ctrl Pts',(10.0514385264421,131.956247508186,-3.26591035271534));
#277344=CARTESIAN_POINT('Ctrl Pts',(8.13178458580675,132.106247508186,-5.90808733016713));
#277345=CARTESIAN_POINT('Ctrl Pts',(6.21213064517136,132.256247508185,-8.55026430761891));
#277346=CARTESIAN_POINT('Ctrl Pts',(3.10606532258563,132.406247508184,-9.55948610871303));
#277347=CARTESIAN_POINT('Ctrl Pts',(-8.94643227470453E-14,132.556247508184,
-10.5687079098071));
#277348=CARTESIAN_POINT('Ctrl Pts',(-3.10606532258582,132.706247508183,
-9.55948610871303));
#277349=CARTESIAN_POINT('Ctrl Pts',(-6.21213064517154,132.856247508183,
-8.55026430761891));
#277350=CARTESIAN_POINT('Ctrl Pts',(-8.13178458580692,133.006247508182,
-5.90808733016712));
#277351=CARTESIAN_POINT('Ctrl Pts',(-10.0514385264423,133.156247508181,
-3.26591035271534));
#277352=CARTESIAN_POINT('Ctrl Pts',(-10.0514385264423,133.306247508181,
2.46189240364677E-15));
#277353=CARTESIAN_POINT('Ctrl Pts',(-10.0514385264423,133.45624750818,3.26591035271534));
#277354=CARTESIAN_POINT('Ctrl Pts',(-8.13178458580692,133.60624750818,5.90808733016713));
#277355=CARTESIAN_POINT('Ctrl Pts',(-6.21213064517154,133.756247508179,
8.55026430761891));
#277356=CARTESIAN_POINT('Ctrl Pts',(-3.10606532258581,133.906247508178,
9.55948610871303));
#277357=CARTESIAN_POINT('Ctrl Pts',(-8.77395905203025E-14,134.056247508178,
10.5687079098071));
#277358=CARTESIAN_POINT('Ctrl Pts',(3.10606532258564,134.206247508177,9.55948610871303));
#277359=CARTESIAN_POINT('Ctrl Pts',(6.21213064517136,134.356247508177,8.55026430761891));
#277360=CARTESIAN_POINT('Ctrl Pts',(8.13178458580674,134.506247508176,5.90808733016712));
#277361=CARTESIAN_POINT('Ctrl Pts',(10.0514385264421,134.656247508175,3.26591035271534));
#277362=CARTESIAN_POINT('Ctrl Pts',(10.0514385264421,134.806247508175,-1.23094620182339E-15));
#277363=CARTESIAN_POINT('Ctrl Pts',(10.0514385264421,134.956247508174,-3.26591035271534));
#277364=CARTESIAN_POINT('Ctrl Pts',(8.13178458580674,135.106247508174,-5.90808733016713));
#277365=CARTESIAN_POINT('Ctrl Pts',(6.21213064517136,135.256247508173,-8.55026430761891));
#277366=CARTESIAN_POINT('Ctrl Pts',(3.10606532258563,135.406247508172,-9.55948610871303));
#277367=CARTESIAN_POINT('Ctrl Pts',(-9.11920320187072E-14,135.556247508172,
-10.5687079098071));
#277368=CARTESIAN_POINT('Ctrl Pts',(-3.10606532258582,135.706247508171,
-9.55948610871303));
#277369=CARTESIAN_POINT('Ctrl Pts',(-6.21213064517154,135.856247508171,
-8.55026430761891));
#277370=CARTESIAN_POINT('Ctrl Pts',(-8.13178458580693,136.00624750817,-5.90808733016712));
#277371=CARTESIAN_POINT('Ctrl Pts',(-10.0514385264423,136.156247508169,
-3.26591035271534));
#277372=CARTESIAN_POINT('Ctrl Pts',(-10.0514385264423,136.306247508169,
2.46189240364677E-15));
#277373=CARTESIAN_POINT('Ctrl Pts',(-10.0514385264423,136.456247508168,
3.26591035271534));
#277374=CARTESIAN_POINT('Ctrl Pts',(-8.13178458580693,136.606247508168,
5.90808733016713));
#277375=CARTESIAN_POINT('Ctrl Pts',(-6.21213064517154,136.756247508167,
8.55026430761891));
#277376=CARTESIAN_POINT('Ctrl Pts',(-3.10606532258582,136.906247508166,
9.55948610871303));
#277377=CARTESIAN_POINT('Ctrl Pts',(-8.94672997919643E-14,137.056247508166,
10.5687079098071));
#277378=CARTESIAN_POINT('Ctrl Pts',(3.10606532258563,137.206247508165,9.55948610871303));
#277379=CARTESIAN_POINT('Ctrl Pts',(6.21213064517136,137.356247508165,8.55026430761891));
#277380=CARTESIAN_POINT('Ctrl Pts',(8.13178458580674,137.506247508164,5.90808733016712));
#277381=CARTESIAN_POINT('Ctrl Pts',(10.0514385264421,137.656247508163,3.26591035271534));
#277382=CARTESIAN_POINT('Ctrl Pts',(10.0514385264421,137.806247508163,-1.23094620182339E-15));
#277383=CARTESIAN_POINT('Ctrl Pts',(10.0514385264421,137.956247508162,-3.26591035271534));
#277384=CARTESIAN_POINT('Ctrl Pts',(8.13178458580674,138.106247508162,-5.90808733016713));
#277385=CARTESIAN_POINT('Ctrl Pts',(6.21213064517135,138.256247508161,-8.55026430761891));
#277386=CARTESIAN_POINT('Ctrl Pts',(3.10606532258563,138.40624750816,-9.55948610871303));
#277387=CARTESIAN_POINT('Ctrl Pts',(-9.2919741290369E-14,138.55624750816,
-10.5687079098071));
#277388=CARTESIAN_POINT('Ctrl Pts',(-3.10606532258582,138.706247508159,
-9.55948610871303));
#277389=CARTESIAN_POINT('Ctrl Pts',(-6.21213064517154,138.856247508159,
-8.55026430761891));
#277390=CARTESIAN_POINT('Ctrl Pts',(-8.13178458580693,139.006247508158,
-5.90808733016712));
#277391=CARTESIAN_POINT('Ctrl Pts',(-10.0514385264423,139.156247508157,
-3.26591035271534));
#277392=CARTESIAN_POINT('Ctrl Pts',(-10.0514385264423,139.306247508157,
2.46189240364677E-15));
#277393=CARTESIAN_POINT('Ctrl Pts',(-10.0514385264423,139.456247508156,
3.26591035271534));
#277394=CARTESIAN_POINT('Ctrl Pts',(-8.13178458580693,139.606247508156,
5.90808733016713));
#277395=CARTESIAN_POINT('Ctrl Pts',(-6.21213064517154,139.756247508155,
8.55026430761891));
#277396=CARTESIAN_POINT('Ctrl Pts',(-3.10606532258582,139.906247508154,
9.55948610871303));
#277397=CARTESIAN_POINT('Ctrl Pts',(-9.11950090636262E-14,140.056247508154,
10.5687079098071));
#277398=CARTESIAN_POINT('Ctrl Pts',(3.10606532258563,140.206247508153,9.55948610871303));
#277399=CARTESIAN_POINT('Ctrl Pts',(6.21213064517136,140.356247508153,8.55026430761891));
#277400=CARTESIAN_POINT('Ctrl Pts',(8.13178458580674,140.506247508152,5.90808733016712));
#277401=CARTESIAN_POINT('Ctrl Pts',(10.0514385264421,140.656247508151,3.26591035271534));
#277402=CARTESIAN_POINT('Ctrl Pts',(10.0514385264421,140.806247508151,-1.23094620182339E-15));
#277403=CARTESIAN_POINT('Ctrl Pts',(10.0514385264421,140.95624750815,-3.26591035271534));
#277404=CARTESIAN_POINT('Ctrl Pts',(8.13178458580674,141.10624750815,-5.90808733016713));
#277405=CARTESIAN_POINT('Ctrl Pts',(6.21213064517135,141.256247508149,-8.55026430761891));
#277406=CARTESIAN_POINT('Ctrl Pts',(3.10606532258563,141.406247508148,-9.55948610871303));
#277407=CARTESIAN_POINT('Ctrl Pts',(-9.46474505620308E-14,141.556247508148,
-10.5687079098071));
#277408=CARTESIAN_POINT('Ctrl Pts',(-3.10606532258582,141.706247508147,
-9.55948610871303));
#277409=CARTESIAN_POINT('Ctrl Pts',(-6.21213064517154,141.856247508147,
-8.55026430761891));
#277410=CARTESIAN_POINT('Ctrl Pts',(-8.13178458580693,142.006247508146,
-5.90808733016712));
#277411=CARTESIAN_POINT('Ctrl Pts',(-10.0514385264423,142.156247508145,
-3.26591035271534));
#277412=CARTESIAN_POINT('Ctrl Pts',(-10.0514385264423,142.306247508145,
2.46189240364677E-15));
#277413=CARTESIAN_POINT('Ctrl Pts',(-10.0514385264423,142.456247508144,
3.26591035271534));
#277414=CARTESIAN_POINT('Ctrl Pts',(-8.13178458580693,142.606247508144,
5.90808733016713));
#277415=CARTESIAN_POINT('Ctrl Pts',(-6.21213064517154,142.756247508143,
8.55026430761891));
#277416=CARTESIAN_POINT('Ctrl Pts',(-3.10606532258582,142.906247508142,
9.55948610871303));
#277417=CARTESIAN_POINT('Ctrl Pts',(-9.2922718335288E-14,143.056247508142,
10.5687079098071));
#277418=CARTESIAN_POINT('Ctrl Pts',(3.10606532258563,143.206247508141,9.55948610871303));
#277419=CARTESIAN_POINT('Ctrl Pts',(6.21213064517135,143.356247508141,8.55026430761891));
#277420=CARTESIAN_POINT('Ctrl Pts',(8.13178458580674,143.50624750814,5.90808733016712));
#277421=CARTESIAN_POINT('Ctrl Pts',(10.0514385264421,143.656247508139,3.26591035271534));
#277422=CARTESIAN_POINT('Ctrl Pts',(10.0514385264421,143.806247508139,-1.23094620182339E-15));
#277423=CARTESIAN_POINT('Ctrl Pts',(10.0514385264421,143.956247508138,-3.26591035271534));
#277424=CARTESIAN_POINT('Ctrl Pts',(8.13178458580674,144.106247508138,-5.90808733016713));
#277425=CARTESIAN_POINT('Ctrl Pts',(6.21213064517135,144.256247508137,-8.55026430761891));
#277426=CARTESIAN_POINT('Ctrl Pts',(3.10606532258563,144.406247508136,-9.55948610871303));
#277427=CARTESIAN_POINT('Ctrl Pts',(-9.63751598336927E-14,144.556247508136,
-10.5687079098071));
#277428=CARTESIAN_POINT('Ctrl Pts',(-3.10606532258582,144.706247508135,
-9.55948610871303));
#277429=CARTESIAN_POINT('Ctrl Pts',(-6.21213064517155,144.856247508135,
-8.55026430761891));
#277430=CARTESIAN_POINT('Ctrl Pts',(-8.13178458580693,145.006247508134,
-5.90808733016712));
#277431=CARTESIAN_POINT('Ctrl Pts',(-10.0514385264423,145.156247508133,
-3.26591035271534));
#277432=CARTESIAN_POINT('Ctrl Pts',(-10.0514385264423,145.306247508133,
2.46189240364677E-15));
#277433=CARTESIAN_POINT('Ctrl Pts',(-10.0514385264423,145.456247508132,
3.26591035271534));
#277434=CARTESIAN_POINT('Ctrl Pts',(-8.13178458580693,145.606247508132,
5.90808733016713));
#277435=CARTESIAN_POINT('Ctrl Pts',(-6.21213064517154,145.756247508131,
8.55026430761891));
#277436=CARTESIAN_POINT('Ctrl Pts',(-3.10606532258582,145.90624750813,9.55948610871303));
#277437=CARTESIAN_POINT('Ctrl Pts',(-9.46504276069498E-14,146.05624750813,
10.5687079098071));
#277438=CARTESIAN_POINT('Ctrl Pts',(3.10606532258563,146.206247508129,9.55948610871303));
#277439=CARTESIAN_POINT('Ctrl Pts',(6.21213064517135,146.356247508129,8.55026430761891));
#277440=CARTESIAN_POINT('Ctrl Pts',(8.13178458580674,146.506247508128,5.90808733016712));
#277441=CARTESIAN_POINT('Ctrl Pts',(10.0514385264421,146.656247508127,3.26591035271534));
#277442=CARTESIAN_POINT('Ctrl Pts',(10.0514385264421,146.806247508127,-1.23094620182339E-15));
#277443=CARTESIAN_POINT('Ctrl Pts',(10.0514385264421,146.956247508126,-3.26591035271534));
#277444=CARTESIAN_POINT('Ctrl Pts',(8.13178458580674,147.106247508126,-5.90808733016713));
#277445=CARTESIAN_POINT('Ctrl Pts',(6.21213064517135,147.256247508125,-8.55026430761891));
#277446=CARTESIAN_POINT('Ctrl Pts',(3.10606532258563,147.406247508124,-9.55948610871303));
#277447=CARTESIAN_POINT('Ctrl Pts',(-9.81028691053545E-14,147.556247508124,
-10.5687079098071));
#277448=CARTESIAN_POINT('Ctrl Pts',(-3.10606532258582,147.706247508123,
-9.55948610871303));
#277449=CARTESIAN_POINT('Ctrl Pts',(-6.21213064517155,147.856247508123,
-8.55026430761891));
#277450=CARTESIAN_POINT('Ctrl Pts',(-8.13178458580693,148.006247508122,
-5.90808733016712));
#277451=CARTESIAN_POINT('Ctrl Pts',(-10.0514385264423,148.156247508121,
-3.26591035271534));
#277452=CARTESIAN_POINT('Ctrl Pts',(-10.0514385264423,148.306247508121,
2.46189240364677E-15));
#277453=CARTESIAN_POINT('Ctrl Pts',(-10.0514385264423,148.45624750812,3.26591035271534));
#277454=CARTESIAN_POINT('Ctrl Pts',(-8.13178458580693,148.60624750812,5.90808733016713));
#277455=CARTESIAN_POINT('Ctrl Pts',(-6.21213064517155,148.756247508119,
8.55026430761891));
#277456=CARTESIAN_POINT('Ctrl Pts',(-3.10606532258582,148.906247508118,
9.55948610871303));
#277457=CARTESIAN_POINT('Ctrl Pts',(-9.63781368786116E-14,149.056247508118,
10.5687079098071));
#277458=CARTESIAN_POINT('Ctrl Pts',(3.10606532258563,149.206247508117,9.55948610871303));
#277459=CARTESIAN_POINT('Ctrl Pts',(6.21213064517135,149.356247508117,8.55026430761891));
#277460=CARTESIAN_POINT('Ctrl Pts',(8.13178458580673,149.506247508116,5.90808733016712));
#277461=CARTESIAN_POINT('Ctrl Pts',(10.0514385264421,149.656247508115,3.26591035271534));
#277462=CARTESIAN_POINT('Ctrl Pts',(10.0514385264421,149.806247508115,-1.23094620182339E-15));
#277463=CARTESIAN_POINT('Ctrl Pts',(10.0514385264421,149.956247508114,-3.26591035271534));
#277464=CARTESIAN_POINT('Ctrl Pts',(8.13178458580673,150.106247508114,-5.90808733016713));
#277465=CARTESIAN_POINT('Ctrl Pts',(6.21213064517135,150.256247508113,-8.55026430761891));
#277466=CARTESIAN_POINT('Ctrl Pts',(3.10606532258562,150.406247508112,-9.55948610871303));
#277467=CARTESIAN_POINT('Ctrl Pts',(-9.98305783770163E-14,150.556247508112,
-10.5687079098071));
#277468=CARTESIAN_POINT('Ctrl Pts',(-3.10606532258582,150.706247508111,
-9.55948610871303));
#277469=CARTESIAN_POINT('Ctrl Pts',(-6.21213064517155,150.856247508111,
-8.55026430761891));
#277470=CARTESIAN_POINT('Ctrl Pts',(-8.13178458580694,151.00624750811,-5.90808733016712));
#277471=CARTESIAN_POINT('Ctrl Pts',(-10.0514385264423,151.156247508109,
-3.26591035271534));
#277472=CARTESIAN_POINT('Ctrl Pts',(-10.0514385264423,151.306247508109,
2.46189240364677E-15));
#277473=CARTESIAN_POINT('Ctrl Pts',(-10.0514385264423,151.456247508108,
3.26591035271534));
#277474=CARTESIAN_POINT('Ctrl Pts',(-8.13178458580694,151.606247508108,
5.90808733016713));
#277475=CARTESIAN_POINT('Ctrl Pts',(-6.21213064517155,151.756247508107,
8.55026430761891));
#277476=CARTESIAN_POINT('Ctrl Pts',(-3.10606532258582,151.906247508106,
9.55948610871303));
#277477=CARTESIAN_POINT('Ctrl Pts',(-9.81058461502735E-14,152.056247508106,
10.5687079098071));
#277478=CARTESIAN_POINT('Ctrl Pts',(3.10606532258563,152.206247508105,9.55948610871303));
#277479=CARTESIAN_POINT('Ctrl Pts',(6.21213064517135,152.356247508105,8.55026430761891));
#277480=CARTESIAN_POINT('Ctrl Pts',(8.13178458580673,152.506247508104,5.90808733016712));
#277481=CARTESIAN_POINT('Ctrl Pts',(10.0514385264421,152.656247508103,3.26591035271534));
#277482=CARTESIAN_POINT('Ctrl Pts',(10.0514385264421,152.806247508103,-1.23094620182339E-15));
#277483=CARTESIAN_POINT('Ctrl Pts',(10.0514385264421,152.956247508102,-3.26591035271534));
#277484=CARTESIAN_POINT('Ctrl Pts',(8.13178458580673,153.106247508102,-5.90808733016713));
#277485=CARTESIAN_POINT('Ctrl Pts',(6.21213064517135,153.256247508101,-8.55026430761891));
#277486=CARTESIAN_POINT('Ctrl Pts',(3.10606532258562,153.4062475081,-9.55948610871303));
#277487=CARTESIAN_POINT('Ctrl Pts',(-1.01558287648678E-13,153.5562475081,
-10.5687079098071));
#277488=CARTESIAN_POINT('Ctrl Pts',(-3.10606532258583,153.706247508099,
-9.55948610871303));
#277489=CARTESIAN_POINT('Ctrl Pts',(-12.1623797632097,-0.474999999988005,
2.97892388940585E-15));
#277490=CARTESIAN_POINT('Ctrl Pts',(-12.1623797632096,-0.324999999988605,
3.95179673813133));
#277491=CARTESIAN_POINT('Ctrl Pts',(-9.83957192047856,-0.174999999989203,
7.14886745759505));
#277492=CARTESIAN_POINT('Ctrl Pts',(-7.51676407774747,-0.0249999999898023,
10.3459381770588));
#277493=CARTESIAN_POINT('Ctrl Pts',(-3.75838203887374,0.1250000000096,11.5671105274568));
#277494=CARTESIAN_POINT('Ctrl Pts',(-1.02868273148643E-14,0.275000000009002,
12.7882828778549));
#277495=CARTESIAN_POINT('Ctrl Pts',(3.75838203887372,0.425000000008404,
11.5671105274568));
#277496=CARTESIAN_POINT('Ctrl Pts',(7.51676407774745,0.575000000007806,
10.3459381770588));
#277497=CARTESIAN_POINT('Ctrl Pts',(9.83957192047854,0.725000000007208,
7.14886745759505));
#277498=CARTESIAN_POINT('Ctrl Pts',(12.1623797632096,0.875000000006609,
3.95179673813132));
#277499=CARTESIAN_POINT('Ctrl Pts',(12.1623797632096,1.02500000000601,-1.48946194470292E-15));
#277500=CARTESIAN_POINT('Ctrl Pts',(12.1623797632096,1.17500000000541,-3.95179673813132));
#277501=CARTESIAN_POINT('Ctrl Pts',(9.83957192047853,1.32500000000481,-7.14886745759505));
#277502=CARTESIAN_POINT('Ctrl Pts',(7.51676407774744,1.47500000000421,-10.3459381770588));
#277503=CARTESIAN_POINT('Ctrl Pts',(3.75838203887371,1.6250000000036,-11.5671105274568));
#277504=CARTESIAN_POINT('Ctrl Pts',(-1.42829078892864E-14,1.775000000003,
-12.7882828778549));
#277505=CARTESIAN_POINT('Ctrl Pts',(-3.75838203887374,1.9250000000024,-11.5671105274568));
#277506=CARTESIAN_POINT('Ctrl Pts',(-7.51676407774747,2.0750000000018,-10.3459381770588));
#277507=CARTESIAN_POINT('Ctrl Pts',(-9.83957192047856,2.2250000000012,-7.14886745759505));
#277508=CARTESIAN_POINT('Ctrl Pts',(-12.1623797632097,2.37500000000059,
-3.95179673813132));
#277509=CARTESIAN_POINT('Ctrl Pts',(-12.1623797632097,2.525,2.97892388940585E-15));
#277510=CARTESIAN_POINT('Ctrl Pts',(-12.1623797632097,2.6749999999994,3.95179673813133));
#277511=CARTESIAN_POINT('Ctrl Pts',(-9.83957192047856,2.8249999999988,7.14886745759505));
#277512=CARTESIAN_POINT('Ctrl Pts',(-7.51676407774747,2.9749999999982,10.3459381770588));
#277513=CARTESIAN_POINT('Ctrl Pts',(-3.75838203887374,3.1249999999976,11.5671105274568));
#277514=CARTESIAN_POINT('Ctrl Pts',(-1.20145365865262E-14,3.274999999997,
12.7882828778549));
#277515=CARTESIAN_POINT('Ctrl Pts',(3.75838203887372,3.4249999999964,11.5671105274568));
#277516=CARTESIAN_POINT('Ctrl Pts',(7.51676407774744,3.57499999999581,10.3459381770588));
#277517=CARTESIAN_POINT('Ctrl Pts',(9.83957192047853,3.72499999999521,7.14886745759505));
#277518=CARTESIAN_POINT('Ctrl Pts',(12.1623797632096,3.87499999999461,3.95179673813132));
#277519=CARTESIAN_POINT('Ctrl Pts',(12.1623797632096,4.02499999999401,-1.48946194470292E-15));
#277520=CARTESIAN_POINT('Ctrl Pts',(12.1623797632096,4.17499999999341,-3.95179673813132));
#277521=CARTESIAN_POINT('Ctrl Pts',(9.83957192047853,4.32499999999281,-7.14886745759505));
#277522=CARTESIAN_POINT('Ctrl Pts',(7.51676407774744,4.47499999999221,-10.3459381770588));
#277523=CARTESIAN_POINT('Ctrl Pts',(3.75838203887371,4.6249999999916,-11.5671105274568));
#277524=CARTESIAN_POINT('Ctrl Pts',(-1.60106171609483E-14,4.774999999991,
-12.7882828778549));
#277525=CARTESIAN_POINT('Ctrl Pts',(-3.75838203887374,4.9249999999904,-11.5671105274568));
#277526=CARTESIAN_POINT('Ctrl Pts',(-7.51676407774747,5.0749999999898,-10.3459381770588));
#277527=CARTESIAN_POINT('Ctrl Pts',(-9.83957192047857,5.2249999999892,-7.14886745759505));
#277528=CARTESIAN_POINT('Ctrl Pts',(-12.1623797632097,5.3749999999886,-3.95179673813132));
#277529=CARTESIAN_POINT('Ctrl Pts',(-12.1623797632097,5.52499999998799,
2.97892388940585E-15));
#277530=CARTESIAN_POINT('Ctrl Pts',(-12.1623797632097,5.67499999998739,
3.95179673813133));
#277531=CARTESIAN_POINT('Ctrl Pts',(-9.83957192047857,5.8249999999868,7.14886745759505));
#277532=CARTESIAN_POINT('Ctrl Pts',(-7.51676407774747,5.9749999999862,10.3459381770588));
#277533=CARTESIAN_POINT('Ctrl Pts',(-3.75838203887374,6.1249999999856,11.5671105274568));
#277534=CARTESIAN_POINT('Ctrl Pts',(-1.3742245858188E-14,6.274999999985,
12.7882828778549));
#277535=CARTESIAN_POINT('Ctrl Pts',(3.75838203887371,6.4249999999844,11.5671105274568));
#277536=CARTESIAN_POINT('Ctrl Pts',(7.51676407774744,6.57499999998381,10.3459381770588));
#277537=CARTESIAN_POINT('Ctrl Pts',(9.83957192047853,6.72499999998321,7.14886745759505));
#277538=CARTESIAN_POINT('Ctrl Pts',(12.1623797632096,6.87499999998261,3.95179673813132));
#277539=CARTESIAN_POINT('Ctrl Pts',(12.1623797632096,7.02499999998201,-1.48946194470292E-15));
#277540=CARTESIAN_POINT('Ctrl Pts',(12.1623797632096,7.17499999998141,-3.95179673813132));
#277541=CARTESIAN_POINT('Ctrl Pts',(9.83957192047853,7.32499999998081,-7.14886745759505));
#277542=CARTESIAN_POINT('Ctrl Pts',(7.51676407774744,7.47499999998021,-10.3459381770588));
#277543=CARTESIAN_POINT('Ctrl Pts',(3.75838203887371,7.6249999999796,-11.5671105274568));
#277544=CARTESIAN_POINT('Ctrl Pts',(-1.77383264326101E-14,7.774999999979,
-12.7882828778549));
#277545=CARTESIAN_POINT('Ctrl Pts',(-3.75838203887375,7.9249999999784,-11.5671105274568));
#277546=CARTESIAN_POINT('Ctrl Pts',(-7.51676407774747,8.0749999999778,-10.3459381770588));
#277547=CARTESIAN_POINT('Ctrl Pts',(-9.83957192047857,8.2249999999772,-7.14886745759505));
#277548=CARTESIAN_POINT('Ctrl Pts',(-12.1623797632097,8.3749999999766,-3.95179673813132));
#277549=CARTESIAN_POINT('Ctrl Pts',(-12.1623797632097,8.52499999997599,
2.97892388940585E-15));
#277550=CARTESIAN_POINT('Ctrl Pts',(-12.1623797632097,8.6749999999754,3.95179673813133));
#277551=CARTESIAN_POINT('Ctrl Pts',(-9.83957192047857,8.8249999999748,7.14886745759505));
#277552=CARTESIAN_POINT('Ctrl Pts',(-7.51676407774747,8.9749999999742,10.3459381770588));
#277553=CARTESIAN_POINT('Ctrl Pts',(-3.75838203887374,9.1249999999736,11.5671105274568));
#277554=CARTESIAN_POINT('Ctrl Pts',(-1.54699551298498E-14,9.274999999973,
12.7882828778549));
#277555=CARTESIAN_POINT('Ctrl Pts',(3.75838203887371,9.4249999999724,11.5671105274568));
#277556=CARTESIAN_POINT('Ctrl Pts',(7.51676407774744,9.57499999997181,10.3459381770588));
#277557=CARTESIAN_POINT('Ctrl Pts',(9.83957192047853,9.72499999997121,7.14886745759505));
#277558=CARTESIAN_POINT('Ctrl Pts',(12.1623797632096,9.87499999997061,3.95179673813132));
#277559=CARTESIAN_POINT('Ctrl Pts',(12.1623797632096,10.02499999997,-1.48946194470292E-15));
#277560=CARTESIAN_POINT('Ctrl Pts',(12.1623797632096,10.1749999999694,-3.95179673813132));
#277561=CARTESIAN_POINT('Ctrl Pts',(9.83957192047853,10.3249999999688,-7.14886745759505));
#277562=CARTESIAN_POINT('Ctrl Pts',(7.51676407774744,10.4749999999682,-10.3459381770588));
#277563=CARTESIAN_POINT('Ctrl Pts',(3.75838203887371,10.6249999999676,-11.5671105274568));
#277564=CARTESIAN_POINT('Ctrl Pts',(-1.9466035704272E-14,10.774999999967,
-12.7882828778549));
#277565=CARTESIAN_POINT('Ctrl Pts',(-3.75838203887375,10.9249999999664,
-11.5671105274568));
#277566=CARTESIAN_POINT('Ctrl Pts',(-7.51676407774748,11.0749999999658,
-10.3459381770588));
#277567=CARTESIAN_POINT('Ctrl Pts',(-9.83957192047857,11.2249999999652,
-7.14886745759505));
#277568=CARTESIAN_POINT('Ctrl Pts',(-12.1623797632097,11.3749999999646,
-3.95179673813132));
#277569=CARTESIAN_POINT('Ctrl Pts',(-12.1623797632097,11.524999999964,2.97892388940585E-15));
#277570=CARTESIAN_POINT('Ctrl Pts',(-12.1623797632097,11.6749999999634,
3.95179673813133));
#277571=CARTESIAN_POINT('Ctrl Pts',(-9.83957192047857,11.8249999999628,
7.14886745759505));
#277572=CARTESIAN_POINT('Ctrl Pts',(-7.51676407774747,11.9749999999622,
10.3459381770588));
#277573=CARTESIAN_POINT('Ctrl Pts',(-3.75838203887375,12.1249999999616,
11.5671105274568));
#277574=CARTESIAN_POINT('Ctrl Pts',(-1.71976644015117E-14,12.274999999961,
12.7882828778549));
#277575=CARTESIAN_POINT('Ctrl Pts',(3.75838203887371,12.4249999999604,11.5671105274568));
#277576=CARTESIAN_POINT('Ctrl Pts',(7.51676407774744,12.5749999999598,10.3459381770588));
#277577=CARTESIAN_POINT('Ctrl Pts',(9.83957192047853,12.7249999999592,7.14886745759505));
#277578=CARTESIAN_POINT('Ctrl Pts',(12.1623797632096,12.8749999999586,3.95179673813132));
#277579=CARTESIAN_POINT('Ctrl Pts',(12.1623797632096,13.024999999958,-1.48946194470292E-15));
#277580=CARTESIAN_POINT('Ctrl Pts',(12.1623797632096,13.1749999999574,-3.95179673813132));
#277581=CARTESIAN_POINT('Ctrl Pts',(9.83957192047853,13.3249999999568,-7.14886745759505));
#277582=CARTESIAN_POINT('Ctrl Pts',(7.51676407774743,13.4749999999562,-10.3459381770588));
#277583=CARTESIAN_POINT('Ctrl Pts',(3.75838203887371,13.6249999999556,-11.5671105274568));
#277584=CARTESIAN_POINT('Ctrl Pts',(-2.11937449759338E-14,13.774999999955,
-12.7882828778549));
#277585=CARTESIAN_POINT('Ctrl Pts',(-3.75838203887375,13.9249999999544,
-11.5671105274568));
#277586=CARTESIAN_POINT('Ctrl Pts',(-7.51676407774748,14.0749999999538,
-10.3459381770588));
#277587=CARTESIAN_POINT('Ctrl Pts',(-9.83957192047857,14.2249999999532,
-7.14886745759505));
#277588=CARTESIAN_POINT('Ctrl Pts',(-12.1623797632097,14.3749999999526,
-3.95179673813132));
#277589=CARTESIAN_POINT('Ctrl Pts',(-12.1623797632097,14.524999999952,2.97892388940585E-15));
#277590=CARTESIAN_POINT('Ctrl Pts',(-12.1623797632097,14.6749999999514,
3.95179673813133));
#277591=CARTESIAN_POINT('Ctrl Pts',(-9.83957192047857,14.8249999999508,
7.14886745759505));
#277592=CARTESIAN_POINT('Ctrl Pts',(-7.51676407774747,14.9749999999502,
10.3459381770588));
#277593=CARTESIAN_POINT('Ctrl Pts',(-3.75838203887375,15.1249999999496,
11.5671105274568));
#277594=CARTESIAN_POINT('Ctrl Pts',(-1.89253736731735E-14,15.274999999949,
12.7882828778549));
#277595=CARTESIAN_POINT('Ctrl Pts',(3.75838203887371,15.4249999999484,11.5671105274568));
#277596=CARTESIAN_POINT('Ctrl Pts',(7.51676407774744,15.5749999999478,10.3459381770588));
#277597=CARTESIAN_POINT('Ctrl Pts',(9.83957192047853,15.7249999999472,7.14886745759505));
#277598=CARTESIAN_POINT('Ctrl Pts',(12.1623797632096,15.8749999999466,3.95179673813132));
#277599=CARTESIAN_POINT('Ctrl Pts',(12.1623797632096,16.024999999946,-1.48946194470292E-15));
#277600=CARTESIAN_POINT('Ctrl Pts',(12.1623797632096,16.1749999999454,-3.95179673813132));
#277601=CARTESIAN_POINT('Ctrl Pts',(9.83957192047852,16.3249999999448,-7.14886745759505));
#277602=CARTESIAN_POINT('Ctrl Pts',(7.51676407774743,16.4749999999442,-10.3459381770588));
#277603=CARTESIAN_POINT('Ctrl Pts',(3.7583820388737,16.6249999999436,-11.5671105274568));
#277604=CARTESIAN_POINT('Ctrl Pts',(-2.29214542475956E-14,16.774999999943,
-12.7882828778549));
#277605=CARTESIAN_POINT('Ctrl Pts',(-3.75838203887375,16.9249999999424,
-11.5671105274568));
#277606=CARTESIAN_POINT('Ctrl Pts',(-7.51676407774748,17.0749999999418,
-10.3459381770588));
#277607=CARTESIAN_POINT('Ctrl Pts',(-9.83957192047857,17.2249999999412,
-7.14886745759505));
#277608=CARTESIAN_POINT('Ctrl Pts',(-12.1623797632097,17.3749999999406,
-3.95179673813132));
#277609=CARTESIAN_POINT('Ctrl Pts',(-12.1623797632097,17.52499999994,2.97892388940585E-15));
#277610=CARTESIAN_POINT('Ctrl Pts',(-12.1623797632097,17.6749999999394,
3.95179673813133));
#277611=CARTESIAN_POINT('Ctrl Pts',(-9.83957192047857,17.8249999999388,
7.14886745759505));
#277612=CARTESIAN_POINT('Ctrl Pts',(-7.51676407774748,17.9749999999382,
10.3459381770588));
#277613=CARTESIAN_POINT('Ctrl Pts',(-3.75838203887375,18.1249999999376,
11.5671105274568));
#277614=CARTESIAN_POINT('Ctrl Pts',(-2.06530829448354E-14,18.274999999937,
12.7882828778549));
#277615=CARTESIAN_POINT('Ctrl Pts',(3.75838203887371,18.4249999999364,11.5671105274568));
#277616=CARTESIAN_POINT('Ctrl Pts',(7.51676407774743,18.5749999999358,10.3459381770588));
#277617=CARTESIAN_POINT('Ctrl Pts',(9.83957192047852,18.7249999999352,7.14886745759505));
#277618=CARTESIAN_POINT('Ctrl Pts',(12.1623797632096,18.8749999999346,3.95179673813132));
#277619=CARTESIAN_POINT('Ctrl Pts',(12.1623797632096,19.024999999934,-1.48946194470292E-15));
#277620=CARTESIAN_POINT('Ctrl Pts',(12.1623797632096,19.1749999999334,-3.95179673813132));
#277621=CARTESIAN_POINT('Ctrl Pts',(9.83957192047852,19.3249999999328,-7.14886745759505));
#277622=CARTESIAN_POINT('Ctrl Pts',(7.51676407774743,19.4749999999322,-10.3459381770588));
#277623=CARTESIAN_POINT('Ctrl Pts',(3.7583820388737,19.6249999999316,-11.5671105274568));
#277624=CARTESIAN_POINT('Ctrl Pts',(-2.46491635192575E-14,19.774999999931,
-12.7882828778549));
#277625=CARTESIAN_POINT('Ctrl Pts',(-3.75838203887375,19.9249999999304,
-11.5671105274568));
#277626=CARTESIAN_POINT('Ctrl Pts',(-7.51676407774748,20.0749999999298,
-10.3459381770588));
#277627=CARTESIAN_POINT('Ctrl Pts',(-9.83957192047857,20.2249999999292,
-7.14886745759505));
#277628=CARTESIAN_POINT('Ctrl Pts',(-12.1623797632097,20.3749999999286,
-3.95179673813132));
#277629=CARTESIAN_POINT('Ctrl Pts',(-12.1623797632097,20.524999999928,2.97892388940585E-15));
#277630=CARTESIAN_POINT('Ctrl Pts',(-12.1623797632097,20.6749999999274,
3.95179673813133));
#277631=CARTESIAN_POINT('Ctrl Pts',(-9.83957192047857,20.8249999999268,
7.14886745759505));
#277632=CARTESIAN_POINT('Ctrl Pts',(-7.51676407774748,20.9749999999262,
10.3459381770588));
#277633=CARTESIAN_POINT('Ctrl Pts',(-3.75838203887375,21.1249999999256,
11.5671105274568));
#277634=CARTESIAN_POINT('Ctrl Pts',(-2.23807922164972E-14,21.274999999925,
12.7882828778549));
#277635=CARTESIAN_POINT('Ctrl Pts',(3.7583820388737,21.4249999999244,11.5671105274568));
#277636=CARTESIAN_POINT('Ctrl Pts',(7.51676407774743,21.5749999999238,10.3459381770588));
#277637=CARTESIAN_POINT('Ctrl Pts',(9.83957192047852,21.7249999999232,7.14886745759505));
#277638=CARTESIAN_POINT('Ctrl Pts',(12.1623797632096,21.8749999999226,3.95179673813132));
#277639=CARTESIAN_POINT('Ctrl Pts',(12.1623797632096,22.024999999922,-1.48946194470292E-15));
#277640=CARTESIAN_POINT('Ctrl Pts',(12.1623797632096,22.1749999999214,-3.95179673813132));
#277641=CARTESIAN_POINT('Ctrl Pts',(9.83957192047852,22.3249999999208,-7.14886745759505));
#277642=CARTESIAN_POINT('Ctrl Pts',(7.51676407774743,22.4749999999202,-10.3459381770588));
#277643=CARTESIAN_POINT('Ctrl Pts',(3.7583820388737,22.6249999999196,-11.5671105274568));
#277644=CARTESIAN_POINT('Ctrl Pts',(-2.63768727909193E-14,22.774999999919,
-12.7882828778549));
#277645=CARTESIAN_POINT('Ctrl Pts',(-3.75838203887375,22.9249999999184,
-11.5671105274568));
#277646=CARTESIAN_POINT('Ctrl Pts',(-7.51676407774748,23.0749999999178,
-10.3459381770588));
#277647=CARTESIAN_POINT('Ctrl Pts',(-9.83957192047857,23.2249999999172,
-7.14886745759505));
#277648=CARTESIAN_POINT('Ctrl Pts',(-12.1623797632097,23.3749999999166,
-3.95179673813132));
#277649=CARTESIAN_POINT('Ctrl Pts',(-12.1623797632097,23.524999999916,2.97892388940585E-15));
#277650=CARTESIAN_POINT('Ctrl Pts',(-12.1623797632097,23.6749999999154,
3.95179673813133));
#277651=CARTESIAN_POINT('Ctrl Pts',(-9.83957192047857,23.8249999999148,
7.14886745759505));
#277652=CARTESIAN_POINT('Ctrl Pts',(-7.51676407774748,23.9749999999142,
10.3459381770588));
#277653=CARTESIAN_POINT('Ctrl Pts',(-3.75838203887375,24.1249999999136,
11.5671105274568));
#277654=CARTESIAN_POINT('Ctrl Pts',(-2.4108501488159E-14,24.274999999913,
12.7882828778549));
#277655=CARTESIAN_POINT('Ctrl Pts',(3.7583820388737,24.4249999999124,11.5671105274568));
#277656=CARTESIAN_POINT('Ctrl Pts',(7.51676407774743,24.5749999999118,10.3459381770588));
#277657=CARTESIAN_POINT('Ctrl Pts',(9.83957192047852,24.7249999999112,7.14886745759505));
#277658=CARTESIAN_POINT('Ctrl Pts',(12.1623797632096,24.8749999999106,3.95179673813132));
#277659=CARTESIAN_POINT('Ctrl Pts',(12.1623797632096,25.02499999991,-1.48946194470292E-15));
#277660=CARTESIAN_POINT('Ctrl Pts',(12.1623797632096,25.1749999999094,-3.95179673813132));
#277661=CARTESIAN_POINT('Ctrl Pts',(9.83957192047852,25.3249999999088,-7.14886745759505));
#277662=CARTESIAN_POINT('Ctrl Pts',(7.51676407774743,25.4749999999082,-10.3459381770588));
#277663=CARTESIAN_POINT('Ctrl Pts',(3.7583820388737,25.6249999999076,-11.5671105274568));
#277664=CARTESIAN_POINT('Ctrl Pts',(-2.81045820625811E-14,25.774999999907,
-12.7882828778549));
#277665=CARTESIAN_POINT('Ctrl Pts',(-3.75838203887376,25.9249999999064,
-11.5671105274568));
#277666=CARTESIAN_POINT('Ctrl Pts',(-7.51676407774749,26.0749999999058,
-10.3459381770588));
#277667=CARTESIAN_POINT('Ctrl Pts',(-9.83957192047857,26.2249999999052,
-7.14886745759505));
#277668=CARTESIAN_POINT('Ctrl Pts',(-12.1623797632097,26.3749999999046,
-3.95179673813132));
#277669=CARTESIAN_POINT('Ctrl Pts',(-12.1623797632097,26.524999999904,2.97892388940585E-15));
#277670=CARTESIAN_POINT('Ctrl Pts',(-12.1623797632097,26.6749999999034,
3.95179673813133));
#277671=CARTESIAN_POINT('Ctrl Pts',(-9.83957192047857,26.8249999999028,
7.14886745759505));
#277672=CARTESIAN_POINT('Ctrl Pts',(-7.51676407774748,26.9749999999022,
10.3459381770588));
#277673=CARTESIAN_POINT('Ctrl Pts',(-3.75838203887375,27.1249999999016,
11.5671105274568));
#277674=CARTESIAN_POINT('Ctrl Pts',(-2.58362107598209E-14,27.274999999901,
12.7882828778549));
#277675=CARTESIAN_POINT('Ctrl Pts',(3.7583820388737,27.4249999999004,11.5671105274568));
#277676=CARTESIAN_POINT('Ctrl Pts',(7.51676407774743,27.5749999998998,10.3459381770588));
#277677=CARTESIAN_POINT('Ctrl Pts',(9.83957192047852,27.7249999998992,7.14886745759505));
#277678=CARTESIAN_POINT('Ctrl Pts',(12.1623797632096,27.8749999998986,3.95179673813132));
#277679=CARTESIAN_POINT('Ctrl Pts',(12.1623797632096,28.024999999898,-1.48946194470292E-15));
#277680=CARTESIAN_POINT('Ctrl Pts',(12.1623797632096,28.1749999998974,-3.95179673813132));
#277681=CARTESIAN_POINT('Ctrl Pts',(9.83957192047852,28.3249999998968,-7.14886745759505));
#277682=CARTESIAN_POINT('Ctrl Pts',(7.51676407774743,28.4749999998962,-10.3459381770588));
#277683=CARTESIAN_POINT('Ctrl Pts',(3.7583820388737,28.6249999998956,-11.5671105274568));
#277684=CARTESIAN_POINT('Ctrl Pts',(-2.9832291334243E-14,28.774999999895,
-12.7882828778549));
#277685=CARTESIAN_POINT('Ctrl Pts',(-3.75838203887376,28.9249999998944,
-11.5671105274568));
#277686=CARTESIAN_POINT('Ctrl Pts',(-7.51676407774749,29.0749999998938,
-10.3459381770588));
#277687=CARTESIAN_POINT('Ctrl Pts',(-9.83957192047858,29.2249999998932,
-7.14886745759505));
#277688=CARTESIAN_POINT('Ctrl Pts',(-12.1623797632097,29.3749999998926,
-3.95179673813132));
#277689=CARTESIAN_POINT('Ctrl Pts',(-12.1623797632097,29.524999999892,2.97892388940585E-15));
#277690=CARTESIAN_POINT('Ctrl Pts',(-12.1623797632097,29.6749999998914,
3.95179673813133));
#277691=CARTESIAN_POINT('Ctrl Pts',(-9.83957192047858,29.8249999998908,
7.14886745759505));
#277692=CARTESIAN_POINT('Ctrl Pts',(-7.51676407774748,29.9749999998902,
10.3459381770588));
#277693=CARTESIAN_POINT('Ctrl Pts',(-3.75838203887376,30.1249999998896,
11.5671105274568));
#277694=CARTESIAN_POINT('Ctrl Pts',(-2.75639200314827E-14,30.274999999889,
12.7882828778549));
#277695=CARTESIAN_POINT('Ctrl Pts',(3.7583820388737,30.4249999998884,11.5671105274568));
#277696=CARTESIAN_POINT('Ctrl Pts',(7.51676407774743,30.5749999998878,10.3459381770588));
#277697=CARTESIAN_POINT('Ctrl Pts',(9.83957192047852,30.7249999998872,7.14886745759505));
#277698=CARTESIAN_POINT('Ctrl Pts',(12.1623797632096,30.8749999998866,3.95179673813132));
#277699=CARTESIAN_POINT('Ctrl Pts',(12.1623797632096,31.024999999886,-1.48946194470292E-15));
#277700=CARTESIAN_POINT('Ctrl Pts',(12.1623797632096,31.1749999998854,-3.95179673813132));
#277701=CARTESIAN_POINT('Ctrl Pts',(9.83957192047852,31.3249999998848,-7.14886745759505));
#277702=CARTESIAN_POINT('Ctrl Pts',(7.51676407774742,31.4749999998842,-10.3459381770588));
#277703=CARTESIAN_POINT('Ctrl Pts',(3.7583820388737,31.6249999998836,-11.5671105274568));
#277704=CARTESIAN_POINT('Ctrl Pts',(-3.15600006059048E-14,31.774999999883,
-12.7882828778549));
#277705=CARTESIAN_POINT('Ctrl Pts',(-3.75838203887376,31.9249999998824,
-11.5671105274568));
#277706=CARTESIAN_POINT('Ctrl Pts',(-7.51676407774749,32.0749999998818,
-10.3459381770588));
#277707=CARTESIAN_POINT('Ctrl Pts',(-9.83957192047858,32.2249999998812,
-7.14886745759505));
#277708=CARTESIAN_POINT('Ctrl Pts',(-12.1623797632097,32.3749999998806,
-3.95179673813132));
#277709=CARTESIAN_POINT('Ctrl Pts',(-12.1623797632097,32.52499999988,2.97892388940585E-15));
#277710=CARTESIAN_POINT('Ctrl Pts',(-12.1623797632097,32.6749999998794,
3.95179673813133));
#277711=CARTESIAN_POINT('Ctrl Pts',(-9.83957192047858,32.8249999998788,
7.14886745759505));
#277712=CARTESIAN_POINT('Ctrl Pts',(-7.51676407774749,32.9749999998782,
10.3459381770588));
#277713=CARTESIAN_POINT('Ctrl Pts',(-3.75838203887376,33.1249999998776,
11.5671105274568));
#277714=CARTESIAN_POINT('Ctrl Pts',(-2.92916293031446E-14,33.274999999877,
12.7882828778549));
#277715=CARTESIAN_POINT('Ctrl Pts',(3.7583820388737,33.4249999998764,11.5671105274568));
#277716=CARTESIAN_POINT('Ctrl Pts',(7.51676407774743,33.5749999998758,10.3459381770588));
#277717=CARTESIAN_POINT('Ctrl Pts',(9.83957192047852,33.7249999998752,7.14886745759505));
#277718=CARTESIAN_POINT('Ctrl Pts',(12.1623797632096,33.8749999998746,3.95179673813132));
#277719=CARTESIAN_POINT('Ctrl Pts',(12.1623797632096,34.024999999874,-1.48946194470292E-15));
#277720=CARTESIAN_POINT('Ctrl Pts',(12.1623797632096,34.1749999998734,-3.95179673813132));
#277721=CARTESIAN_POINT('Ctrl Pts',(9.83957192047851,34.3249999998728,-7.14886745759505));
#277722=CARTESIAN_POINT('Ctrl Pts',(7.51676407774742,34.4749999998722,-10.3459381770588));
#277723=CARTESIAN_POINT('Ctrl Pts',(3.7583820388737,34.6249999998716,-11.5671105274568));
#277724=CARTESIAN_POINT('Ctrl Pts',(-3.32877098775667E-14,34.774999999871,
-12.7882828778549));
#277725=CARTESIAN_POINT('Ctrl Pts',(-3.75838203887376,34.9249999998704,
-11.5671105274568));
#277726=CARTESIAN_POINT('Ctrl Pts',(-7.51676407774749,35.0749999998698,
-10.3459381770588));
#277727=CARTESIAN_POINT('Ctrl Pts',(-9.83957192047858,35.2249999998692,
-7.14886745759505));
#277728=CARTESIAN_POINT('Ctrl Pts',(-12.1623797632097,35.3749999998686,
-3.95179673813132));
#277729=CARTESIAN_POINT('Ctrl Pts',(-12.1623797632097,35.524999999868,2.97892388940585E-15));
#277730=CARTESIAN_POINT('Ctrl Pts',(-12.1623797632097,35.6749999998674,
3.95179673813133));
#277731=CARTESIAN_POINT('Ctrl Pts',(-9.83957192047858,35.8249999998668,
7.14886745759505));
#277732=CARTESIAN_POINT('Ctrl Pts',(-7.51676407774749,35.9749999998662,
10.3459381770588));
#277733=CARTESIAN_POINT('Ctrl Pts',(-3.75838203887376,36.1249999998656,
11.5671105274568));
#277734=CARTESIAN_POINT('Ctrl Pts',(-3.10193385748064E-14,36.274999999865,
12.7882828778549));
#277735=CARTESIAN_POINT('Ctrl Pts',(3.7583820388737,36.4249999998644,11.5671105274568));
#277736=CARTESIAN_POINT('Ctrl Pts',(7.51676407774742,36.5749999998638,10.3459381770588));
#277737=CARTESIAN_POINT('Ctrl Pts',(9.83957192047851,36.7249999998632,7.14886745759505));
#277738=CARTESIAN_POINT('Ctrl Pts',(12.1623797632096,36.8749999998626,3.95179673813132));
#277739=CARTESIAN_POINT('Ctrl Pts',(12.1623797632096,37.024999999862,-1.48946194470292E-15));
#277740=CARTESIAN_POINT('Ctrl Pts',(12.1623797632096,37.1749999998614,-3.95179673813132));
#277741=CARTESIAN_POINT('Ctrl Pts',(9.83957192047851,37.3249999998608,-7.14886745759505));
#277742=CARTESIAN_POINT('Ctrl Pts',(7.51676407774742,37.4749999998602,-10.3459381770588));
#277743=CARTESIAN_POINT('Ctrl Pts',(3.75838203887369,37.6249999998596,-11.5671105274568));
#277744=CARTESIAN_POINT('Ctrl Pts',(-3.50154191492285E-14,37.774999999859,
-12.7882828778549));
#277745=CARTESIAN_POINT('Ctrl Pts',(-3.75838203887376,37.9249999998584,
-11.5671105274568));
#277746=CARTESIAN_POINT('Ctrl Pts',(-7.51676407774749,38.0749999998578,
-10.3459381770588));
#277747=CARTESIAN_POINT('Ctrl Pts',(-9.83957192047858,38.2249999998572,
-7.14886745759505));
#277748=CARTESIAN_POINT('Ctrl Pts',(-12.1623797632097,38.3749999998566,
-3.95179673813132));
#277749=CARTESIAN_POINT('Ctrl Pts',(-12.1623797632097,38.524999999856,2.97892388940585E-15));
#277750=CARTESIAN_POINT('Ctrl Pts',(-12.1623797632097,38.6749999998554,
3.95179673813133));
#277751=CARTESIAN_POINT('Ctrl Pts',(-9.83957192047858,38.8249999998548,
7.14886745759505));
#277752=CARTESIAN_POINT('Ctrl Pts',(-7.51676407774749,38.9749999998542,
10.3459381770588));
#277753=CARTESIAN_POINT('Ctrl Pts',(-3.75838203887376,39.1249999998536,
11.5671105274568));
#277754=CARTESIAN_POINT('Ctrl Pts',(-3.27470478464682E-14,39.274999999853,
12.7882828778549));
#277755=CARTESIAN_POINT('Ctrl Pts',(3.7583820388737,39.4249999998524,11.5671105274568));
#277756=CARTESIAN_POINT('Ctrl Pts',(7.51676407774742,39.5749999998518,10.3459381770588));
#277757=CARTESIAN_POINT('Ctrl Pts',(9.83957192047851,39.7249999998512,7.14886745759505));
#277758=CARTESIAN_POINT('Ctrl Pts',(12.1623797632096,39.8749999998506,3.95179673813132));
#277759=CARTESIAN_POINT('Ctrl Pts',(12.1623797632096,40.02499999985,-1.48946194470292E-15));
#277760=CARTESIAN_POINT('Ctrl Pts',(12.1623797632096,40.1749999998494,-3.95179673813132));
#277761=CARTESIAN_POINT('Ctrl Pts',(9.83957192047851,40.3249999998488,-7.14886745759505));
#277762=CARTESIAN_POINT('Ctrl Pts',(7.51676407774742,40.4749999998482,-10.3459381770588));
#277763=CARTESIAN_POINT('Ctrl Pts',(3.75838203887369,40.6249999998476,-11.5671105274568));
#277764=CARTESIAN_POINT('Ctrl Pts',(-3.67431284208903E-14,40.774999999847,
-12.7882828778549));
#277765=CARTESIAN_POINT('Ctrl Pts',(-3.75838203887376,40.9249999998464,
-11.5671105274568));
#277766=CARTESIAN_POINT('Ctrl Pts',(-7.51676407774749,41.0749999998458,
-10.3459381770588));
#277767=CARTESIAN_POINT('Ctrl Pts',(-9.83957192047858,41.2249999998452,
-7.14886745759505));
#277768=CARTESIAN_POINT('Ctrl Pts',(-12.1623797632097,41.3749999998446,
-3.95179673813132));
#277769=CARTESIAN_POINT('Ctrl Pts',(-12.1623797632097,41.524999999844,2.97892388940585E-15));
#277770=CARTESIAN_POINT('Ctrl Pts',(-12.1623797632097,41.6749999998434,
3.95179673813133));
#277771=CARTESIAN_POINT('Ctrl Pts',(-9.83957192047858,41.8249999998428,
7.14886745759505));
#277772=CARTESIAN_POINT('Ctrl Pts',(-7.51676407774749,41.9749999998422,
10.3459381770588));
#277773=CARTESIAN_POINT('Ctrl Pts',(-3.75838203887376,42.1249999998416,
11.5671105274568));
#277774=CARTESIAN_POINT('Ctrl Pts',(-3.44747571181301E-14,42.274999999841,
12.7882828778549));
#277775=CARTESIAN_POINT('Ctrl Pts',(3.75838203887369,42.4249999998404,11.5671105274568));
#277776=CARTESIAN_POINT('Ctrl Pts',(7.51676407774742,42.5749999998398,10.3459381770588));
#277777=CARTESIAN_POINT('Ctrl Pts',(9.83957192047851,42.7249999998392,7.14886745759505));
#277778=CARTESIAN_POINT('Ctrl Pts',(12.1623797632096,42.8749999998386,3.95179673813132));
#277779=CARTESIAN_POINT('Ctrl Pts',(12.1623797632096,43.024999999838,-1.48946194470292E-15));
#277780=CARTESIAN_POINT('Ctrl Pts',(12.1623797632096,43.1749999998374,-3.95179673813132));
#277781=CARTESIAN_POINT('Ctrl Pts',(9.83957192047851,43.3249999998368,-7.14886745759505));
#277782=CARTESIAN_POINT('Ctrl Pts',(7.51676407774742,43.4749999998362,-10.3459381770588));
#277783=CARTESIAN_POINT('Ctrl Pts',(3.75838203887369,43.6249999998356,-11.5671105274568));
#277784=CARTESIAN_POINT('Ctrl Pts',(-3.84708376925522E-14,43.774999999835,
-12.7882828778549));
#277785=CARTESIAN_POINT('Ctrl Pts',(-3.75838203887377,43.9249999998344,
-11.5671105274568));
#277786=CARTESIAN_POINT('Ctrl Pts',(-7.51676407774749,44.0749999998338,
-10.3459381770588));
#277787=CARTESIAN_POINT('Ctrl Pts',(-9.83957192047859,44.2249999998332,
-7.14886745759505));
#277788=CARTESIAN_POINT('Ctrl Pts',(-12.1623797632097,44.3749999998326,
-3.95179673813132));
#277789=CARTESIAN_POINT('Ctrl Pts',(-12.1623797632097,44.524999999832,2.97892388940585E-15));
#277790=CARTESIAN_POINT('Ctrl Pts',(-12.1623797632097,44.6749999998314,
3.95179673813133));
#277791=CARTESIAN_POINT('Ctrl Pts',(-9.83957192047859,44.8249999998308,
7.14886745759505));
#277792=CARTESIAN_POINT('Ctrl Pts',(-7.51676407774749,44.9749999998302,
10.3459381770588));
#277793=CARTESIAN_POINT('Ctrl Pts',(-3.75838203887376,45.1249999998296,
11.5671105274568));
#277794=CARTESIAN_POINT('Ctrl Pts',(-3.62024663897919E-14,45.274999999829,
12.7882828778549));
#277795=CARTESIAN_POINT('Ctrl Pts',(3.75838203887369,45.4249999998284,11.5671105274568));
#277796=CARTESIAN_POINT('Ctrl Pts',(7.51676407774742,45.5749999998278,10.3459381770588));
#277797=CARTESIAN_POINT('Ctrl Pts',(9.83957192047851,45.7249999998272,7.14886745759505));
#277798=CARTESIAN_POINT('Ctrl Pts',(12.1623797632096,45.8749999998266,3.95179673813132));
#277799=CARTESIAN_POINT('Ctrl Pts',(12.1623797632096,46.024999999826,-1.48946194470292E-15));
#277800=CARTESIAN_POINT('Ctrl Pts',(12.1623797632096,46.1749999998254,-3.95179673813132));
#277801=CARTESIAN_POINT('Ctrl Pts',(9.83957192047851,46.3249999998248,-7.14886745759505));
#277802=CARTESIAN_POINT('Ctrl Pts',(7.51676407774742,46.4749999998242,-10.3459381770588));
#277803=CARTESIAN_POINT('Ctrl Pts',(3.75838203887369,46.6249999998236,-11.5671105274568));
#277804=CARTESIAN_POINT('Ctrl Pts',(-4.0198546964214E-14,46.774999999823,
-12.7882828778549));
#277805=CARTESIAN_POINT('Ctrl Pts',(-3.75838203887377,46.9249999998224,
-11.5671105274568));
#277806=CARTESIAN_POINT('Ctrl Pts',(-7.5167640777475,47.0749999998218,-10.3459381770588));
#277807=CARTESIAN_POINT('Ctrl Pts',(-9.83957192047859,47.2249999998212,
-7.14886745759505));
#277808=CARTESIAN_POINT('Ctrl Pts',(-12.1623797632097,47.3749999998206,
-3.95179673813132));
#277809=CARTESIAN_POINT('Ctrl Pts',(-12.1623797632097,47.52499999982,2.97892388940585E-15));
#277810=CARTESIAN_POINT('Ctrl Pts',(-12.1623797632097,47.6749999998194,
3.95179673813133));
#277811=CARTESIAN_POINT('Ctrl Pts',(-9.83957192047859,47.8249999998188,
7.14886745759505));
#277812=CARTESIAN_POINT('Ctrl Pts',(-7.51676407774749,47.9749999998182,
10.3459381770588));
#277813=CARTESIAN_POINT('Ctrl Pts',(-3.75838203887377,48.1249999998176,
11.5671105274568));
#277814=CARTESIAN_POINT('Ctrl Pts',(-3.79301756614538E-14,48.274999999817,
12.7882828778549));
#277815=CARTESIAN_POINT('Ctrl Pts',(3.75838203887369,48.4249999998164,11.5671105274568));
#277816=CARTESIAN_POINT('Ctrl Pts',(7.51676407774742,48.5749999998158,10.3459381770588));
#277817=CARTESIAN_POINT('Ctrl Pts',(9.83957192047851,48.7249999998152,7.14886745759505));
#277818=CARTESIAN_POINT('Ctrl Pts',(12.1623797632096,48.8749999998146,3.95179673813132));
#277819=CARTESIAN_POINT('Ctrl Pts',(12.1623797632096,49.024999999814,-1.48946194470292E-15));
#277820=CARTESIAN_POINT('Ctrl Pts',(12.1623797632096,49.1749999998134,-3.95179673813132));
#277821=CARTESIAN_POINT('Ctrl Pts',(9.83957192047851,49.3249999998128,-7.14886745759505));
#277822=CARTESIAN_POINT('Ctrl Pts',(7.51676407774741,49.4749999998122,-10.3459381770588));
#277823=CARTESIAN_POINT('Ctrl Pts',(3.75838203887369,49.6249999998116,-11.5671105274568));
#277824=CARTESIAN_POINT('Ctrl Pts',(-4.19262562358759E-14,49.774999999811,
-12.7882828778549));
#277825=CARTESIAN_POINT('Ctrl Pts',(-3.75838203887377,49.9249999998104,
-11.5671105274568));
#277826=CARTESIAN_POINT('Ctrl Pts',(-7.5167640777475,50.0749999998098,-10.3459381770588));
#277827=CARTESIAN_POINT('Ctrl Pts',(-9.83957192047859,50.2249999998092,
-7.14886745759505));
#277828=CARTESIAN_POINT('Ctrl Pts',(-12.1623797632097,50.3749999998086,
-3.95179673813132));
#277829=CARTESIAN_POINT('Ctrl Pts',(-12.1623797632097,50.524999999808,2.97892388940585E-15));
#277830=CARTESIAN_POINT('Ctrl Pts',(-12.1623797632097,50.6749999998074,
3.95179673813133));
#277831=CARTESIAN_POINT('Ctrl Pts',(-9.83957192047859,50.8249999998068,
7.14886745759505));
#277832=CARTESIAN_POINT('Ctrl Pts',(-7.51676407774749,50.9749999998062,
10.3459381770588));
#277833=CARTESIAN_POINT('Ctrl Pts',(-3.75838203887377,51.1249999998056,
11.5671105274568));
#277834=CARTESIAN_POINT('Ctrl Pts',(-3.96578849331156E-14,51.274999999805,
12.7882828778549));
#277835=CARTESIAN_POINT('Ctrl Pts',(3.75838203887369,51.4249999998044,11.5671105274568));
#277836=CARTESIAN_POINT('Ctrl Pts',(7.51676407774742,51.5749999998038,10.3459381770588));
#277837=CARTESIAN_POINT('Ctrl Pts',(9.83957192047851,51.7249999998032,7.14886745759505));
#277838=CARTESIAN_POINT('Ctrl Pts',(12.1623797632096,51.8749999998026,3.95179673813132));
#277839=CARTESIAN_POINT('Ctrl Pts',(12.1623797632096,52.024999999802,-1.48946194470292E-15));
#277840=CARTESIAN_POINT('Ctrl Pts',(12.1623797632096,52.1749999998014,-3.95179673813132));
#277841=CARTESIAN_POINT('Ctrl Pts',(9.8395719204785,52.3249999998008,-7.14886745759505));
#277842=CARTESIAN_POINT('Ctrl Pts',(7.51676407774741,52.4749999998002,-10.3459381770588));
#277843=CARTESIAN_POINT('Ctrl Pts',(3.75838203887368,52.6249999997996,-11.5671105274568));
#277844=CARTESIAN_POINT('Ctrl Pts',(-4.36539655075377E-14,52.774999999799,
-12.7882828778549));
#277845=CARTESIAN_POINT('Ctrl Pts',(-3.75838203887377,52.9249999997984,
-11.5671105274568));
#277846=CARTESIAN_POINT('Ctrl Pts',(-7.5167640777475,53.0749999997978,-10.3459381770588));
#277847=CARTESIAN_POINT('Ctrl Pts',(-9.83957192047859,53.2249999997972,
-7.14886745759505));
#277848=CARTESIAN_POINT('Ctrl Pts',(-12.1623797632097,53.3749999997966,
-3.95179673813132));
#277849=CARTESIAN_POINT('Ctrl Pts',(-12.1623797632097,53.524999999796,2.97892388940585E-15));
#277850=CARTESIAN_POINT('Ctrl Pts',(-12.1623797632097,53.6749999997954,
3.95179673813133));
#277851=CARTESIAN_POINT('Ctrl Pts',(-9.83957192047859,53.8249999997948,
7.14886745759505));
#277852=CARTESIAN_POINT('Ctrl Pts',(-7.5167640777475,53.9749999997942,10.3459381770588));
#277853=CARTESIAN_POINT('Ctrl Pts',(-3.75838203887377,54.1249999997936,
11.5671105274568));
#277854=CARTESIAN_POINT('Ctrl Pts',(-4.13855942047774E-14,54.274999999793,
12.7882828778549));
#277855=CARTESIAN_POINT('Ctrl Pts',(3.75838203887369,54.4249999997924,11.5671105274568));
#277856=CARTESIAN_POINT('Ctrl Pts',(7.51676407774741,54.5749999997918,10.3459381770588));
#277857=CARTESIAN_POINT('Ctrl Pts',(9.8395719204785,54.7249999997912,7.14886745759505));
#277858=CARTESIAN_POINT('Ctrl Pts',(12.1623797632096,54.8749999997906,3.95179673813132));
#277859=CARTESIAN_POINT('Ctrl Pts',(12.1623797632096,55.02499999979,-1.48946194470292E-15));
#277860=CARTESIAN_POINT('Ctrl Pts',(12.1623797632096,55.1749999997894,-3.95179673813132));
#277861=CARTESIAN_POINT('Ctrl Pts',(9.8395719204785,55.3249999997888,-7.14886745759505));
#277862=CARTESIAN_POINT('Ctrl Pts',(7.51676407774741,55.4749999997882,-10.3459381770588));
#277863=CARTESIAN_POINT('Ctrl Pts',(3.75838203887368,55.6249999997876,-11.5671105274568));
#277864=CARTESIAN_POINT('Ctrl Pts',(-4.53816747791995E-14,55.774999999787,
-12.7882828778549));
#277865=CARTESIAN_POINT('Ctrl Pts',(-3.75838203887377,55.9249999997864,
-11.5671105274568));
#277866=CARTESIAN_POINT('Ctrl Pts',(-7.5167640777475,56.0749999997858,-10.3459381770588));
#277867=CARTESIAN_POINT('Ctrl Pts',(-9.83957192047859,56.2249999997852,
-7.14886745759505));
#277868=CARTESIAN_POINT('Ctrl Pts',(-12.1623797632097,56.3749999997846,
-3.95179673813132));
#277869=CARTESIAN_POINT('Ctrl Pts',(-12.1623797632097,56.524999999784,2.97892388940585E-15));
#277870=CARTESIAN_POINT('Ctrl Pts',(-12.1623797632097,56.6749999997834,
3.95179673813133));
#277871=CARTESIAN_POINT('Ctrl Pts',(-9.83957192047859,56.8249999997828,
7.14886745759505));
#277872=CARTESIAN_POINT('Ctrl Pts',(-7.5167640777475,56.9749999997822,10.3459381770588));
#277873=CARTESIAN_POINT('Ctrl Pts',(-3.75838203887377,57.1249999997816,
11.5671105274568));
#277874=CARTESIAN_POINT('Ctrl Pts',(-4.31133034764393E-14,57.274999999781,
12.7882828778549));
#277875=CARTESIAN_POINT('Ctrl Pts',(3.75838203887368,57.4249999997804,11.5671105274568));
#277876=CARTESIAN_POINT('Ctrl Pts',(7.51676407774741,57.5749999997798,10.3459381770588));
#277877=CARTESIAN_POINT('Ctrl Pts',(9.8395719204785,57.7249999997792,7.14886745759505));
#277878=CARTESIAN_POINT('Ctrl Pts',(12.1623797632096,57.8749999997786,3.95179673813132));
#277879=CARTESIAN_POINT('Ctrl Pts',(12.1623797632096,58.024999999778,-1.48946194470292E-15));
#277880=CARTESIAN_POINT('Ctrl Pts',(12.1623797632096,58.1749999997774,-3.95179673813132));
#277881=CARTESIAN_POINT('Ctrl Pts',(9.8395719204785,58.3249999997768,-7.14886745759505));
#277882=CARTESIAN_POINT('Ctrl Pts',(7.51676407774741,58.4749999997762,-10.3459381770588));
#277883=CARTESIAN_POINT('Ctrl Pts',(3.75838203887368,58.6249999997756,-11.5671105274568));
#277884=CARTESIAN_POINT('Ctrl Pts',(-4.71093840508614E-14,58.774999999775,
-12.7882828778549));
#277885=CARTESIAN_POINT('Ctrl Pts',(-3.75838203887377,58.9249999997744,
-11.5671105274568));
#277886=CARTESIAN_POINT('Ctrl Pts',(-7.5167640777475,59.0749999997738,-10.3459381770588));
#277887=CARTESIAN_POINT('Ctrl Pts',(-9.83957192047859,59.2249999997732,
-7.14886745759505));
#277888=CARTESIAN_POINT('Ctrl Pts',(-12.1623797632097,59.3749999997726,
-3.95179673813132));
#277889=CARTESIAN_POINT('Ctrl Pts',(-12.1623797632097,59.524999999772,2.97892388940585E-15));
#277890=CARTESIAN_POINT('Ctrl Pts',(-12.1623797632097,59.6749999997714,
3.95179673813133));
#277891=CARTESIAN_POINT('Ctrl Pts',(-9.83957192047859,59.8249999997708,
7.14886745759505));
#277892=CARTESIAN_POINT('Ctrl Pts',(-7.5167640777475,59.9749999997702,10.3459381770588));
#277893=CARTESIAN_POINT('Ctrl Pts',(-3.75838203887377,60.1249999997696,
11.5671105274568));
#277894=CARTESIAN_POINT('Ctrl Pts',(-4.48410127481011E-14,60.274999999769,
12.7882828778549));
#277895=CARTESIAN_POINT('Ctrl Pts',(3.75838203887368,60.4249999997684,11.5671105274568));
#277896=CARTESIAN_POINT('Ctrl Pts',(7.51676407774741,60.5749999997678,10.3459381770588));
#277897=CARTESIAN_POINT('Ctrl Pts',(9.8395719204785,60.7249999997672,7.14886745759505));
#277898=CARTESIAN_POINT('Ctrl Pts',(12.1623797632096,60.8749999997666,3.95179673813132));
#277899=CARTESIAN_POINT('Ctrl Pts',(12.1623797632096,61.024999999766,-1.48946194470292E-15));
#277900=CARTESIAN_POINT('Ctrl Pts',(12.1623797632096,61.1749999997654,-3.95179673813132));
#277901=CARTESIAN_POINT('Ctrl Pts',(9.8395719204785,61.3249999997648,-7.14886745759505));
#277902=CARTESIAN_POINT('Ctrl Pts',(7.51676407774741,61.4749999997642,-10.3459381770588));
#277903=CARTESIAN_POINT('Ctrl Pts',(3.75838203887368,61.6249999997636,-11.5671105274568));
#277904=CARTESIAN_POINT('Ctrl Pts',(-4.88370933225232E-14,61.774999999763,
-12.7882828778549));
#277905=CARTESIAN_POINT('Ctrl Pts',(-3.75838203887378,61.9249999997624,
-11.5671105274568));
#277906=CARTESIAN_POINT('Ctrl Pts',(-7.5167640777475,62.0749999997618,-10.3459381770588));
#277907=CARTESIAN_POINT('Ctrl Pts',(-9.8395719204786,62.2249999997612,-7.14886745759505));
#277908=CARTESIAN_POINT('Ctrl Pts',(-12.1623797632097,62.3749999997606,
-3.95179673813132));
#277909=CARTESIAN_POINT('Ctrl Pts',(-12.1623797632097,62.52499999976,2.97892388940585E-15));
#277910=CARTESIAN_POINT('Ctrl Pts',(-12.1623797632097,62.6749999997594,
3.95179673813133));
#277911=CARTESIAN_POINT('Ctrl Pts',(-9.8395719204786,62.8249999997588,7.14886745759505));
#277912=CARTESIAN_POINT('Ctrl Pts',(-7.5167640777475,62.9749999997582,10.3459381770588));
#277913=CARTESIAN_POINT('Ctrl Pts',(-3.75838203887377,63.1249999997576,
11.5671105274568));
#277914=CARTESIAN_POINT('Ctrl Pts',(-4.6568722019763E-14,63.274999999757,
12.7882828778549));
#277915=CARTESIAN_POINT('Ctrl Pts',(3.75838203887368,63.4249999997564,11.5671105274568));
#277916=CARTESIAN_POINT('Ctrl Pts',(7.51676407774741,63.5749999997558,10.3459381770588));
#277917=CARTESIAN_POINT('Ctrl Pts',(9.8395719204785,63.7249999997552,7.14886745759505));
#277918=CARTESIAN_POINT('Ctrl Pts',(12.1623797632096,63.8749999997546,3.95179673813132));
#277919=CARTESIAN_POINT('Ctrl Pts',(12.1623797632096,64.024999999754,-1.48946194470292E-15));
#277920=CARTESIAN_POINT('Ctrl Pts',(12.1623797632096,64.1749999997534,-3.95179673813132));
#277921=CARTESIAN_POINT('Ctrl Pts',(9.8395719204785,64.3249999997528,-7.14886745759505));
#277922=CARTESIAN_POINT('Ctrl Pts',(7.5167640777474,64.4749999997522,-10.3459381770588));
#277923=CARTESIAN_POINT('Ctrl Pts',(3.75838203887368,64.6249999997516,-11.5671105274568));
#277924=CARTESIAN_POINT('Ctrl Pts',(-5.05648025941851E-14,64.774999999751,
-12.7882828778549));
#277925=CARTESIAN_POINT('Ctrl Pts',(-3.75838203887378,64.9249999997504,
-11.5671105274568));
#277926=CARTESIAN_POINT('Ctrl Pts',(-7.51676407774751,65.0749999997498,
-10.3459381770588));
#277927=CARTESIAN_POINT('Ctrl Pts',(-9.8395719204786,65.2249999997492,-7.14886745759505));
#277928=CARTESIAN_POINT('Ctrl Pts',(-12.1623797632097,65.3749999997486,
-3.95179673813132));
#277929=CARTESIAN_POINT('Ctrl Pts',(-12.1623797632097,65.524999999748,2.97892388940585E-15));
#277930=CARTESIAN_POINT('Ctrl Pts',(-12.1623797632097,65.6749999997474,
3.95179673813133));
#277931=CARTESIAN_POINT('Ctrl Pts',(-9.8395719204786,65.8249999997468,7.14886745759505));
#277932=CARTESIAN_POINT('Ctrl Pts',(-7.5167640777475,65.9749999997462,10.3459381770588));
#277933=CARTESIAN_POINT('Ctrl Pts',(-3.75838203887378,66.1249999997456,
11.5671105274568));
#277934=CARTESIAN_POINT('Ctrl Pts',(-4.82964312914248E-14,66.274999999745,
12.7882828778549));
#277935=CARTESIAN_POINT('Ctrl Pts',(3.75838203887368,66.4249999997444,11.5671105274568));
#277936=CARTESIAN_POINT('Ctrl Pts',(7.51676407774741,66.5749999997438,10.3459381770588));
#277937=CARTESIAN_POINT('Ctrl Pts',(9.8395719204785,66.7249999997432,7.14886745759505));
#277938=CARTESIAN_POINT('Ctrl Pts',(12.1623797632096,66.8749999997426,3.95179673813132));
#277939=CARTESIAN_POINT('Ctrl Pts',(12.1623797632096,67.024999999742,-1.48946194470292E-15));
#277940=CARTESIAN_POINT('Ctrl Pts',(12.1623797632096,67.1749999997414,-3.95179673813132));
#277941=CARTESIAN_POINT('Ctrl Pts',(9.8395719204785,67.3249999997408,-7.14886745759505));
#277942=CARTESIAN_POINT('Ctrl Pts',(7.5167640777474,67.4749999997402,-10.3459381770588));
#277943=CARTESIAN_POINT('Ctrl Pts',(3.75838203887368,67.6249999997396,-11.5671105274568));
#277944=CARTESIAN_POINT('Ctrl Pts',(-5.22925118658469E-14,67.774999999739,
-12.7882828778549));
#277945=CARTESIAN_POINT('Ctrl Pts',(-3.75838203887378,67.9249999997384,
-11.5671105274568));
#277946=CARTESIAN_POINT('Ctrl Pts',(-7.51676407774751,68.0749999997378,
-10.3459381770588));
#277947=CARTESIAN_POINT('Ctrl Pts',(-9.8395719204786,68.2249999997372,-7.14886745759505));
#277948=CARTESIAN_POINT('Ctrl Pts',(-12.1623797632097,68.3749999997366,
-3.95179673813132));
#277949=CARTESIAN_POINT('Ctrl Pts',(-12.1623797632097,68.524999999736,2.97892388940585E-15));
#277950=CARTESIAN_POINT('Ctrl Pts',(-12.1623797632097,68.6749999997354,
3.95179673813133));
#277951=CARTESIAN_POINT('Ctrl Pts',(-9.8395719204786,68.8249999997348,7.14886745759505));
#277952=CARTESIAN_POINT('Ctrl Pts',(-7.51676407774751,68.9749999997342,
10.3459381770588));
#277953=CARTESIAN_POINT('Ctrl Pts',(-3.75838203887378,69.1249999997336,
11.5671105274568));
#277954=CARTESIAN_POINT('Ctrl Pts',(-5.00241405630866E-14,69.274999999733,
12.7882828778549));
#277955=CARTESIAN_POINT('Ctrl Pts',(3.75838203887368,69.4249999997324,11.5671105274568));
#277956=CARTESIAN_POINT('Ctrl Pts',(7.5167640777474,69.5749999997318,10.3459381770588));
#277957=CARTESIAN_POINT('Ctrl Pts',(9.8395719204785,69.7249999997312,7.14886745759505));
#277958=CARTESIAN_POINT('Ctrl Pts',(12.1623797632096,69.8749999997306,3.95179673813132));
#277959=CARTESIAN_POINT('Ctrl Pts',(12.1623797632096,70.02499999973,-1.48946194470292E-15));
#277960=CARTESIAN_POINT('Ctrl Pts',(12.1623797632096,70.1749999997294,-3.95179673813132));
#277961=CARTESIAN_POINT('Ctrl Pts',(9.83957192047849,70.3249999997288,-7.14886745759505));
#277962=CARTESIAN_POINT('Ctrl Pts',(7.5167640777474,70.4749999997282,-10.3459381770588));
#277963=CARTESIAN_POINT('Ctrl Pts',(3.75838203887367,70.6249999997276,-11.5671105274568));
#277964=CARTESIAN_POINT('Ctrl Pts',(-5.40202211375087E-14,70.774999999727,
-12.7882828778549));
#277965=CARTESIAN_POINT('Ctrl Pts',(-3.75838203887378,70.9249999997264,
-11.5671105274568));
#277966=CARTESIAN_POINT('Ctrl Pts',(-7.51676407774751,71.0749999997258,
-10.3459381770588));
#277967=CARTESIAN_POINT('Ctrl Pts',(-9.8395719204786,71.2249999997252,-7.14886745759505));
#277968=CARTESIAN_POINT('Ctrl Pts',(-12.1623797632097,71.3749999997246,
-3.95179673813132));
#277969=CARTESIAN_POINT('Ctrl Pts',(-12.1623797632097,71.524999999724,2.97892388940585E-15));
#277970=CARTESIAN_POINT('Ctrl Pts',(-12.1623797632097,71.6749999997234,
3.95179673813133));
#277971=CARTESIAN_POINT('Ctrl Pts',(-9.8395719204786,71.8249999997228,7.14886745759505));
#277972=CARTESIAN_POINT('Ctrl Pts',(-7.51676407774751,71.9749999997222,
10.3459381770588));
#277973=CARTESIAN_POINT('Ctrl Pts',(-3.75838203887378,72.1249999997216,
11.5671105274568));
#277974=CARTESIAN_POINT('Ctrl Pts',(-5.17518498347485E-14,72.274999999721,
12.7882828778549));
#277975=CARTESIAN_POINT('Ctrl Pts',(3.75838203887368,72.4249999997204,11.5671105274568));
#277976=CARTESIAN_POINT('Ctrl Pts',(7.5167640777474,72.5749999997198,10.3459381770588));
#277977=CARTESIAN_POINT('Ctrl Pts',(9.83957192047849,72.7249999997192,7.14886745759505));
#277978=CARTESIAN_POINT('Ctrl Pts',(12.1623797632096,72.8749999997186,3.95179673813132));
#277979=CARTESIAN_POINT('Ctrl Pts',(12.1623797632096,73.024999999718,-1.48946194470292E-15));
#277980=CARTESIAN_POINT('Ctrl Pts',(12.1623797632096,73.1749999997174,-3.95179673813132));
#277981=CARTESIAN_POINT('Ctrl Pts',(9.83957192047849,73.3249999997168,-7.14886745759505));
#277982=CARTESIAN_POINT('Ctrl Pts',(7.5167640777474,73.4749999997162,-10.3459381770588));
#277983=CARTESIAN_POINT('Ctrl Pts',(3.75838203887367,73.6249999997156,-11.5671105274568));
#277984=CARTESIAN_POINT('Ctrl Pts',(-5.57479304091706E-14,73.774999999715,
-12.7882828778549));
#277985=CARTESIAN_POINT('Ctrl Pts',(-3.75838203887378,73.9249999997144,
-11.5671105274568));
#277986=CARTESIAN_POINT('Ctrl Pts',(-7.51676407774751,74.0749999997138,
-10.3459381770588));
#277987=CARTESIAN_POINT('Ctrl Pts',(-9.8395719204786,74.2249999997132,-7.14886745759505));
#277988=CARTESIAN_POINT('Ctrl Pts',(-12.1623797632097,74.3749999997126,
-3.95179673813132));
#277989=CARTESIAN_POINT('Ctrl Pts',(-12.1623797632097,74.524999999712,2.97892388940585E-15));
#277990=CARTESIAN_POINT('Ctrl Pts',(-12.1623797632097,74.6749999997114,
3.95179673813133));
#277991=CARTESIAN_POINT('Ctrl Pts',(-9.8395719204786,74.8249999997108,7.14886745759505));
#277992=CARTESIAN_POINT('Ctrl Pts',(-7.51676407774751,74.9749999997102,
10.3459381770588));
#277993=CARTESIAN_POINT('Ctrl Pts',(-3.75838203887378,75.1249999997096,
11.5671105274568));
#277994=CARTESIAN_POINT('Ctrl Pts',(-5.34795591064103E-14,75.274999999709,
12.7882828778549));
#277995=CARTESIAN_POINT('Ctrl Pts',(3.75838203887367,75.4249999997084,11.5671105274568));
#277996=CARTESIAN_POINT('Ctrl Pts',(7.5167640777474,75.5749999997078,10.3459381770588));
#277997=CARTESIAN_POINT('Ctrl Pts',(9.83957192047849,75.7249999997072,7.14886745759505));
#277998=CARTESIAN_POINT('Ctrl Pts',(12.1623797632096,75.8749999997066,3.95179673813132));
#277999=CARTESIAN_POINT('Ctrl Pts',(12.1623797632096,76.024999999706,-1.48946194470292E-15));
#278000=CARTESIAN_POINT('Ctrl Pts',(12.1623797632096,76.1749999997054,-3.95179673813132));
#278001=CARTESIAN_POINT('Ctrl Pts',(9.83957192047849,76.3249999997048,-7.14886745759505));
#278002=CARTESIAN_POINT('Ctrl Pts',(7.5167640777474,76.4749999997042,-10.3459381770588));
#278003=CARTESIAN_POINT('Ctrl Pts',(3.75838203887367,76.6249999997036,-11.5671105274568));
#278004=CARTESIAN_POINT('Ctrl Pts',(-5.74756396808324E-14,76.774999999703,
-12.7882828778549));
#278005=CARTESIAN_POINT('Ctrl Pts',(-3.75838203887379,76.9249999997024,
-11.5671105274568));
#278006=CARTESIAN_POINT('Ctrl Pts',(-7.51676407774751,77.0749999997018,
-10.3459381770588));
#278007=CARTESIAN_POINT('Ctrl Pts',(-9.8395719204786,77.2249999997012,-7.14886745759505));
#278008=CARTESIAN_POINT('Ctrl Pts',(-12.1623797632097,77.3749999997006,
-3.95179673813132));
#278009=CARTESIAN_POINT('Ctrl Pts',(-12.1623797632097,77.5249999997,2.97892388940585E-15));
#278010=CARTESIAN_POINT('Ctrl Pts',(-12.1623797632097,77.6749999996994,
3.95179673813133));
#278011=CARTESIAN_POINT('Ctrl Pts',(-9.8395719204786,77.8249999996988,7.14886745759505));
#278012=CARTESIAN_POINT('Ctrl Pts',(-7.51676407774751,77.9749999996982,
10.3459381770588));
#278013=CARTESIAN_POINT('Ctrl Pts',(-3.75838203887378,78.1249999996976,
11.5671105274568));
#278014=CARTESIAN_POINT('Ctrl Pts',(-5.52072683780721E-14,78.274999999697,
12.7882828778549));
#278015=CARTESIAN_POINT('Ctrl Pts',(3.75838203887367,78.4249999996964,11.5671105274568));
#278016=CARTESIAN_POINT('Ctrl Pts',(7.5167640777474,78.5749999996958,10.3459381770588));
#278017=CARTESIAN_POINT('Ctrl Pts',(9.83957192047849,78.7249999996952,7.14886745759505));
#278018=CARTESIAN_POINT('Ctrl Pts',(12.1623797632096,78.8749999996946,3.95179673813132));
#278019=CARTESIAN_POINT('Ctrl Pts',(12.1623797632096,79.024999999694,-1.48946194470292E-15));
#278020=CARTESIAN_POINT('Ctrl Pts',(12.1623797632096,79.1749999996934,-3.95179673813132));
#278021=CARTESIAN_POINT('Ctrl Pts',(9.83957192047849,79.3249999996928,-7.14886745759505));
#278022=CARTESIAN_POINT('Ctrl Pts',(7.5167640777474,79.4749999996922,-10.3459381770588));
#278023=CARTESIAN_POINT('Ctrl Pts',(3.75838203887367,79.6249999996916,-11.5671105274568));
#278024=CARTESIAN_POINT('Ctrl Pts',(-5.92033489524943E-14,79.774999999691,
-12.7882828778549));
#278025=CARTESIAN_POINT('Ctrl Pts',(-3.75838203887379,79.9249999996904,
-11.5671105274568));
#278026=CARTESIAN_POINT('Ctrl Pts',(-7.51676407774751,80.0749999996898,
-10.3459381770588));
#278027=CARTESIAN_POINT('Ctrl Pts',(-9.83957192047861,80.2249999996892,
-7.14886745759505));
#278028=CARTESIAN_POINT('Ctrl Pts',(-12.1623797632097,80.3749999996886,
-3.95179673813132));
#278029=CARTESIAN_POINT('Ctrl Pts',(-12.1623797632097,80.524999999688,2.97892388940585E-15));
#278030=CARTESIAN_POINT('Ctrl Pts',(-12.1623797632097,80.6749999996874,
3.95179673813133));
#278031=CARTESIAN_POINT('Ctrl Pts',(-9.83957192047861,80.8249999996868,
7.14886745759505));
#278032=CARTESIAN_POINT('Ctrl Pts',(-7.51676407774751,80.9749999996862,
10.3459381770588));
#278033=CARTESIAN_POINT('Ctrl Pts',(-3.75838203887378,81.1249999996856,
11.5671105274568));
#278034=CARTESIAN_POINT('Ctrl Pts',(-5.6934977649734E-14,81.274999999685,
12.7882828778549));
#278035=CARTESIAN_POINT('Ctrl Pts',(3.75838203887367,81.4249999996844,11.5671105274568));
#278036=CARTESIAN_POINT('Ctrl Pts',(7.5167640777474,81.5749999996838,10.3459381770588));
#278037=CARTESIAN_POINT('Ctrl Pts',(9.83957192047849,81.7249999996832,7.14886745759505));
#278038=CARTESIAN_POINT('Ctrl Pts',(12.1623797632096,81.8749999996826,3.95179673813132));
#278039=CARTESIAN_POINT('Ctrl Pts',(12.1623797632096,82.024999999682,-1.48946194470292E-15));
#278040=CARTESIAN_POINT('Ctrl Pts',(12.1623797632096,82.1749999996814,-3.95179673813132));
#278041=CARTESIAN_POINT('Ctrl Pts',(9.83957192047849,82.3249999996808,-7.14886745759505));
#278042=CARTESIAN_POINT('Ctrl Pts',(7.5167640777474,82.4749999996802,-10.3459381770588));
#278043=CARTESIAN_POINT('Ctrl Pts',(3.75838203887367,82.6249999996796,-11.5671105274568));
#278044=CARTESIAN_POINT('Ctrl Pts',(-6.09310582241561E-14,82.774999999679,
-12.7882828778549));
#278045=CARTESIAN_POINT('Ctrl Pts',(-3.75838203887379,82.9249999996784,
-11.5671105274568));
#278046=CARTESIAN_POINT('Ctrl Pts',(-7.51676407774752,83.0749999996778,
-10.3459381770588));
#278047=CARTESIAN_POINT('Ctrl Pts',(-9.83957192047861,83.2249999996772,
-7.14886745759505));
#278048=CARTESIAN_POINT('Ctrl Pts',(-12.1623797632097,83.3749999996766,
-3.95179673813132));
#278049=CARTESIAN_POINT('Ctrl Pts',(-12.1623797632097,83.524999999676,2.97892388940585E-15));
#278050=CARTESIAN_POINT('Ctrl Pts',(-12.1623797632097,83.6749999996754,
3.95179673813133));
#278051=CARTESIAN_POINT('Ctrl Pts',(-9.83957192047861,83.8249999996748,
7.14886745759505));
#278052=CARTESIAN_POINT('Ctrl Pts',(-7.51676407774751,83.9749999996742,
10.3459381770588));
#278053=CARTESIAN_POINT('Ctrl Pts',(-3.75838203887379,84.1249999996736,
11.5671105274568));
#278054=CARTESIAN_POINT('Ctrl Pts',(-5.86626869213958E-14,84.274999999673,
12.7882828778549));
#278055=CARTESIAN_POINT('Ctrl Pts',(3.75838203887367,84.4249999996724,11.5671105274568));
#278056=CARTESIAN_POINT('Ctrl Pts',(7.5167640777474,84.5749999996718,10.3459381770588));
#278057=CARTESIAN_POINT('Ctrl Pts',(9.83957192047849,84.7249999996712,7.14886745759505));
#278058=CARTESIAN_POINT('Ctrl Pts',(12.1623797632096,84.8749999996706,3.95179673813132));
#278059=CARTESIAN_POINT('Ctrl Pts',(12.1623797632096,85.02499999967,-1.48946194470292E-15));
#278060=CARTESIAN_POINT('Ctrl Pts',(12.1623797632096,85.1749999996694,-3.95179673813132));
#278061=CARTESIAN_POINT('Ctrl Pts',(9.83957192047849,85.3249999996688,-7.14886745759505));
#278062=CARTESIAN_POINT('Ctrl Pts',(7.51676407774739,85.4749999996682,-10.3459381770588));
#278063=CARTESIAN_POINT('Ctrl Pts',(3.75838203887367,85.6249999996676,-11.5671105274568));
#278064=CARTESIAN_POINT('Ctrl Pts',(-6.26587674958179E-14,85.774999999667,
-12.7882828778549));
#278065=CARTESIAN_POINT('Ctrl Pts',(-3.75838203887379,85.9249999996664,
-11.5671105274568));
#278066=CARTESIAN_POINT('Ctrl Pts',(-7.51676407774752,86.0749999996658,
-10.3459381770588));
#278067=CARTESIAN_POINT('Ctrl Pts',(-9.83957192047861,86.2249999996652,
-7.14886745759505));
#278068=CARTESIAN_POINT('Ctrl Pts',(-12.1623797632097,86.3749999996646,
-3.95179673813132));
#278069=CARTESIAN_POINT('Ctrl Pts',(-12.1623797632097,86.524999999664,2.97892388940585E-15));
#278070=CARTESIAN_POINT('Ctrl Pts',(-12.1623797632097,86.6749999996634,
3.95179673813133));
#278071=CARTESIAN_POINT('Ctrl Pts',(-9.83957192047861,86.8249999996628,
7.14886745759505));
#278072=CARTESIAN_POINT('Ctrl Pts',(-7.51676407774752,86.9749999996622,
10.3459381770588));
#278073=CARTESIAN_POINT('Ctrl Pts',(-3.75838203887379,87.1249999996616,
11.5671105274568));
#278074=CARTESIAN_POINT('Ctrl Pts',(-6.03903961930577E-14,87.274999999661,
12.7882828778549));
#278075=CARTESIAN_POINT('Ctrl Pts',(3.75838203887367,87.4249999996604,11.5671105274568));
#278076=CARTESIAN_POINT('Ctrl Pts',(7.5167640777474,87.5749999996598,10.3459381770588));
#278077=CARTESIAN_POINT('Ctrl Pts',(9.83957192047849,87.7249999996592,7.14886745759505));
#278078=CARTESIAN_POINT('Ctrl Pts',(12.1623797632096,87.8749999996586,3.95179673813132));
#278079=CARTESIAN_POINT('Ctrl Pts',(12.1623797632096,88.024999999658,-1.48946194470292E-15));
#278080=CARTESIAN_POINT('Ctrl Pts',(12.1623797632096,88.1749999996574,-3.95179673813132));
#278081=CARTESIAN_POINT('Ctrl Pts',(9.83957192047849,88.3249999996568,-7.14886745759505));
#278082=CARTESIAN_POINT('Ctrl Pts',(7.51676407774739,88.4749999996562,-10.3459381770588));
#278083=CARTESIAN_POINT('Ctrl Pts',(3.75838203887366,88.6249999996556,-11.5671105274568));
#278084=CARTESIAN_POINT('Ctrl Pts',(-6.43864767674798E-14,88.774999999655,
-12.7882828778549));
#278085=CARTESIAN_POINT('Ctrl Pts',(-3.75838203887379,88.9249999996544,
-11.5671105274568));
#278086=CARTESIAN_POINT('Ctrl Pts',(-7.51676407774752,89.0749999996538,
-10.3459381770588));
#278087=CARTESIAN_POINT('Ctrl Pts',(-9.83957192047861,89.2249999996532,
-7.14886745759505));
#278088=CARTESIAN_POINT('Ctrl Pts',(-12.1623797632097,89.3749999996526,
-3.95179673813132));
#278089=CARTESIAN_POINT('Ctrl Pts',(-12.1623797632097,89.524999999652,2.97892388940585E-15));
#278090=CARTESIAN_POINT('Ctrl Pts',(-12.1623797632097,89.6749999996514,
3.95179673813133));
#278091=CARTESIAN_POINT('Ctrl Pts',(-9.83957192047861,89.8249999996508,
7.14886745759505));
#278092=CARTESIAN_POINT('Ctrl Pts',(-7.51676407774752,89.9749999996502,
10.3459381770588));
#278093=CARTESIAN_POINT('Ctrl Pts',(-3.75838203887379,90.1249999996496,
11.5671105274568));
#278094=CARTESIAN_POINT('Ctrl Pts',(-6.21181054647195E-14,90.274999999649,
12.7882828778549));
#278095=CARTESIAN_POINT('Ctrl Pts',(3.75838203887366,90.4249999996484,11.5671105274568));
#278096=CARTESIAN_POINT('Ctrl Pts',(7.51676407774739,90.5749999996478,10.3459381770588));
#278097=CARTESIAN_POINT('Ctrl Pts',(9.83957192047848,90.7249999996472,7.14886745759505));
#278098=CARTESIAN_POINT('Ctrl Pts',(12.1623797632096,90.8749999996466,3.95179673813132));
#278099=CARTESIAN_POINT('Ctrl Pts',(12.1623797632096,91.024999999646,-1.48946194470292E-15));
#278100=CARTESIAN_POINT('Ctrl Pts',(12.1623797632096,91.1749999996454,-3.95179673813132));
#278101=CARTESIAN_POINT('Ctrl Pts',(9.83957192047848,91.3249999996448,-7.14886745759505));
#278102=CARTESIAN_POINT('Ctrl Pts',(7.51676407774739,91.4749999996442,-10.3459381770588));
#278103=CARTESIAN_POINT('Ctrl Pts',(3.75838203887366,91.6249999996436,-11.5671105274568));
#278104=CARTESIAN_POINT('Ctrl Pts',(-6.61141860391416E-14,91.774999999643,
-12.7882828778549));
#278105=CARTESIAN_POINT('Ctrl Pts',(-3.75838203887379,91.9249999996424,
-11.5671105274568));
#278106=CARTESIAN_POINT('Ctrl Pts',(-7.51676407774752,92.0749999996418,
-10.3459381770588));
#278107=CARTESIAN_POINT('Ctrl Pts',(-9.83957192047861,92.2249999996412,
-7.14886745759505));
#278108=CARTESIAN_POINT('Ctrl Pts',(-12.1623797632097,92.3749999996406,
-3.95179673813132));
#278109=CARTESIAN_POINT('Ctrl Pts',(-12.1623797632097,92.52499999964,2.97892388940585E-15));
#278110=CARTESIAN_POINT('Ctrl Pts',(-12.1623797632097,92.6749999996394,
3.95179673813133));
#278111=CARTESIAN_POINT('Ctrl Pts',(-9.83957192047861,92.8249999996388,
7.14886745759505));
#278112=CARTESIAN_POINT('Ctrl Pts',(-7.51676407774752,92.9749999996382,
10.3459381770588));
#278113=CARTESIAN_POINT('Ctrl Pts',(-3.75838203887379,93.1249999996376,
11.5671105274568));
#278114=CARTESIAN_POINT('Ctrl Pts',(-6.38458147363813E-14,93.274999999637,
12.7882828778549));
#278115=CARTESIAN_POINT('Ctrl Pts',(3.75838203887366,93.4249999996364,11.5671105274568));
#278116=CARTESIAN_POINT('Ctrl Pts',(7.51676407774739,93.5749999996358,10.3459381770588));
#278117=CARTESIAN_POINT('Ctrl Pts',(9.83957192047848,93.7249999996352,7.14886745759505));
#278118=CARTESIAN_POINT('Ctrl Pts',(12.1623797632096,93.8749999996346,3.95179673813132));
#278119=CARTESIAN_POINT('Ctrl Pts',(12.1623797632096,94.024999999634,-1.48946194470292E-15));
#278120=CARTESIAN_POINT('Ctrl Pts',(12.1623797632096,94.1749999996334,-3.95179673813132));
#278121=CARTESIAN_POINT('Ctrl Pts',(9.83957192047848,94.3249999996328,-7.14886745759505));
#278122=CARTESIAN_POINT('Ctrl Pts',(7.51676407774739,94.4749999996322,-10.3459381770588));
#278123=CARTESIAN_POINT('Ctrl Pts',(3.75838203887366,94.6249999996316,-11.5671105274568));
#278124=CARTESIAN_POINT('Ctrl Pts',(-6.78418953108034E-14,94.774999999631,
-12.7882828778549));
#278125=CARTESIAN_POINT('Ctrl Pts',(-3.7583820388738,94.9249999996304,-11.5671105274568));
#278126=CARTESIAN_POINT('Ctrl Pts',(-7.51676407774752,95.0749999996298,
-10.3459381770588));
#278127=CARTESIAN_POINT('Ctrl Pts',(-9.83957192047862,95.2249999996292,
-7.14886745759505));
#278128=CARTESIAN_POINT('Ctrl Pts',(-12.1623797632097,95.3749999996286,
-3.95179673813132));
#278129=CARTESIAN_POINT('Ctrl Pts',(-12.1623797632097,95.524999999628,2.97892388940585E-15));
#278130=CARTESIAN_POINT('Ctrl Pts',(-12.1623797632097,95.6749999996274,
3.95179673813133));
#278131=CARTESIAN_POINT('Ctrl Pts',(-9.83957192047862,95.8249999996268,
7.14886745759505));
#278132=CARTESIAN_POINT('Ctrl Pts',(-7.51676407774752,95.9749999996262,
10.3459381770588));
#278133=CARTESIAN_POINT('Ctrl Pts',(-3.75838203887379,96.1249999996256,
11.5671105274568));
#278134=CARTESIAN_POINT('Ctrl Pts',(-6.55735240080432E-14,96.274999999625,
12.7882828778549));
#278135=CARTESIAN_POINT('Ctrl Pts',(3.75838203887366,96.4249999996244,11.5671105274568));
#278136=CARTESIAN_POINT('Ctrl Pts',(7.51676407774739,96.5749999996238,10.3459381770588));
#278137=CARTESIAN_POINT('Ctrl Pts',(9.83957192047848,96.7249999996232,7.14886745759505));
#278138=CARTESIAN_POINT('Ctrl Pts',(12.1623797632096,96.8749999996226,3.95179673813132));
#278139=CARTESIAN_POINT('Ctrl Pts',(12.1623797632096,97.024999999622,-1.48946194470292E-15));
#278140=CARTESIAN_POINT('Ctrl Pts',(12.1623797632096,97.1749999996214,-3.95179673813132));
#278141=CARTESIAN_POINT('Ctrl Pts',(9.83957192047848,97.3249999996208,-7.14886745759505));
#278142=CARTESIAN_POINT('Ctrl Pts',(7.51676407774739,97.4749999996202,-10.3459381770588));
#278143=CARTESIAN_POINT('Ctrl Pts',(3.75838203887366,97.6249999996196,-11.5671105274568));
#278144=CARTESIAN_POINT('Ctrl Pts',(-6.95696045824653E-14,97.774999999619,
-12.7882828778549));
#278145=CARTESIAN_POINT('Ctrl Pts',(-3.7583820388738,97.9249999996184,-11.5671105274568));
#278146=CARTESIAN_POINT('Ctrl Pts',(-7.51676407774752,98.0749999996178,
-10.3459381770588));
#278147=CARTESIAN_POINT('Ctrl Pts',(-9.83957192047862,98.2249999996172,
-7.14886745759505));
#278148=CARTESIAN_POINT('Ctrl Pts',(-12.1623797632097,98.3749999996166,
-3.95179673813132));
#278149=CARTESIAN_POINT('Ctrl Pts',(-12.1623797632097,98.524999999616,2.97892388940585E-15));
#278150=CARTESIAN_POINT('Ctrl Pts',(-12.1623797632097,98.6749999996154,
3.95179673813133));
#278151=CARTESIAN_POINT('Ctrl Pts',(-9.83957192047862,98.8249999996148,
7.14886745759505));
#278152=CARTESIAN_POINT('Ctrl Pts',(-7.51676407774752,98.9749999996142,
10.3459381770588));
#278153=CARTESIAN_POINT('Ctrl Pts',(-3.7583820388738,99.1249999996136,11.5671105274568));
#278154=CARTESIAN_POINT('Ctrl Pts',(-6.7301233279705E-14,99.274999999613,
12.7882828778549));
#278155=CARTESIAN_POINT('Ctrl Pts',(3.75838203887366,99.4249999996124,11.5671105274568));
#278156=CARTESIAN_POINT('Ctrl Pts',(7.51676407774739,99.5749999996118,10.3459381770588));
#278157=CARTESIAN_POINT('Ctrl Pts',(9.83957192047848,99.7249999996112,7.14886745759505));
#278158=CARTESIAN_POINT('Ctrl Pts',(12.1623797632096,99.8749999996106,3.95179673813132));
#278159=CARTESIAN_POINT('Ctrl Pts',(12.1623797632096,100.02499999961,-1.48946194470292E-15));
#278160=CARTESIAN_POINT('Ctrl Pts',(12.1623797632096,100.174999999609,-3.95179673813132));
#278161=CARTESIAN_POINT('Ctrl Pts',(9.83957192047848,100.324999999609,-7.14886745759505));
#278162=CARTESIAN_POINT('Ctrl Pts',(7.51676407774738,100.474999999608,-10.3459381770588));
#278163=CARTESIAN_POINT('Ctrl Pts',(3.75838203887366,100.624999999608,-11.5671105274568));
#278164=CARTESIAN_POINT('Ctrl Pts',(-7.12973138541271E-14,100.774999999607,
-12.7882828778549));
#278165=CARTESIAN_POINT('Ctrl Pts',(-3.7583820388738,100.924999999606,-11.5671105274568));
#278166=CARTESIAN_POINT('Ctrl Pts',(-7.51676407774753,101.074999999606,
-10.3459381770588));
#278167=CARTESIAN_POINT('Ctrl Pts',(-9.83957192047862,101.224999999605,
-7.14886745759505));
#278168=CARTESIAN_POINT('Ctrl Pts',(-12.1623797632097,101.374999999605,
-3.95179673813132));
#278169=CARTESIAN_POINT('Ctrl Pts',(-12.1623797632097,101.524999999604,
2.97892388940585E-15));
#278170=CARTESIAN_POINT('Ctrl Pts',(-12.1623797632097,101.674999999603,
3.95179673813133));
#278171=CARTESIAN_POINT('Ctrl Pts',(-9.83957192047862,101.824999999603,
7.14886745759505));
#278172=CARTESIAN_POINT('Ctrl Pts',(-7.51676407774752,101.974999999602,
10.3459381770588));
#278173=CARTESIAN_POINT('Ctrl Pts',(-3.7583820388738,102.124999999602,11.5671105274568));
#278174=CARTESIAN_POINT('Ctrl Pts',(-6.90289425513669E-14,102.274999999601,
12.7882828778549));
#278175=CARTESIAN_POINT('Ctrl Pts',(3.75838203887366,102.4249999996,11.5671105274568));
#278176=CARTESIAN_POINT('Ctrl Pts',(7.51676407774739,102.5749999996,10.3459381770588));
#278177=CARTESIAN_POINT('Ctrl Pts',(9.83957192047848,102.724999999599,7.14886745759505));
#278178=CARTESIAN_POINT('Ctrl Pts',(12.1623797632096,102.874999999599,3.95179673813132));
#278179=CARTESIAN_POINT('Ctrl Pts',(12.1623797632096,103.024999999598,-1.48946194470292E-15));
#278180=CARTESIAN_POINT('Ctrl Pts',(12.1623797632096,103.174999999597,-3.95179673813132));
#278181=CARTESIAN_POINT('Ctrl Pts',(9.83957192047848,103.324999999597,-7.14886745759505));
#278182=CARTESIAN_POINT('Ctrl Pts',(7.51676407774738,103.474999999596,-10.3459381770588));
#278183=CARTESIAN_POINT('Ctrl Pts',(3.75838203887366,103.624999999596,-11.5671105274568));
#278184=CARTESIAN_POINT('Ctrl Pts',(-7.3025023125789E-14,103.774999999595,
-12.7882828778549));
#278185=CARTESIAN_POINT('Ctrl Pts',(-3.7583820388738,103.924999999594,-11.5671105274568));
#278186=CARTESIAN_POINT('Ctrl Pts',(-7.51676407774753,104.074999999594,
-10.3459381770588));
#278187=CARTESIAN_POINT('Ctrl Pts',(-9.83957192047862,104.224999999593,
-7.14886745759505));
#278188=CARTESIAN_POINT('Ctrl Pts',(-12.1623797632097,104.374999999593,
-3.95179673813132));
#278189=CARTESIAN_POINT('Ctrl Pts',(-12.1623797632097,104.524999999592,
2.97892388940585E-15));
#278190=CARTESIAN_POINT('Ctrl Pts',(-12.1623797632097,104.674999999591,
3.95179673813133));
#278191=CARTESIAN_POINT('Ctrl Pts',(-9.83957192047862,104.824999999591,
7.14886745759505));
#278192=CARTESIAN_POINT('Ctrl Pts',(-7.51676407774753,104.97499999959,10.3459381770588));
#278193=CARTESIAN_POINT('Ctrl Pts',(-3.7583820388738,105.12499999959,11.5671105274568));
#278194=CARTESIAN_POINT('Ctrl Pts',(-7.07566518230287E-14,105.274999999589,
12.7882828778549));
#278195=CARTESIAN_POINT('Ctrl Pts',(3.75838203887366,105.424999999588,11.5671105274568));
#278196=CARTESIAN_POINT('Ctrl Pts',(7.51676407774738,105.574999999588,10.3459381770588));
#278197=CARTESIAN_POINT('Ctrl Pts',(9.83957192047848,105.724999999587,7.14886745759505));
#278198=CARTESIAN_POINT('Ctrl Pts',(12.1623797632096,105.874999999587,3.95179673813132));
#278199=CARTESIAN_POINT('Ctrl Pts',(12.1623797632096,106.024999999586,-1.48946194470292E-15));
#278200=CARTESIAN_POINT('Ctrl Pts',(12.1623797632096,106.174999999585,-3.95179673813132));
#278201=CARTESIAN_POINT('Ctrl Pts',(9.83957192047848,106.324999999585,-7.14886745759505));
#278202=CARTESIAN_POINT('Ctrl Pts',(7.51676407774738,106.474999999584,-10.3459381770588));
#278203=CARTESIAN_POINT('Ctrl Pts',(3.75838203887365,106.624999999584,-11.5671105274568));
#278204=CARTESIAN_POINT('Ctrl Pts',(-7.47527323974508E-14,106.774999999583,
-12.7882828778549));
#278205=CARTESIAN_POINT('Ctrl Pts',(-3.7583820388738,106.924999999582,-11.5671105274568));
#278206=CARTESIAN_POINT('Ctrl Pts',(-7.51676407774753,107.074999999582,
-10.3459381770588));
#278207=CARTESIAN_POINT('Ctrl Pts',(-9.83957192047862,107.224999999581,
-7.14886745759505));
#278208=CARTESIAN_POINT('Ctrl Pts',(-12.1623797632097,107.374999999581,
-3.95179673813132));
#278209=CARTESIAN_POINT('Ctrl Pts',(-12.1623797632097,107.52499999958,2.97892388940585E-15));
#278210=CARTESIAN_POINT('Ctrl Pts',(-12.1623797632097,107.674999999579,
3.95179673813133));
#278211=CARTESIAN_POINT('Ctrl Pts',(-9.83957192047862,107.824999999579,
7.14886745759505));
#278212=CARTESIAN_POINT('Ctrl Pts',(-7.51676407774753,107.974999999578,
10.3459381770588));
#278213=CARTESIAN_POINT('Ctrl Pts',(-3.7583820388738,108.124999999578,11.5671105274568));
#278214=CARTESIAN_POINT('Ctrl Pts',(-7.24843610946905E-14,108.274999999577,
12.7882828778549));
#278215=CARTESIAN_POINT('Ctrl Pts',(3.75838203887366,108.424999999576,11.5671105274568));
#278216=CARTESIAN_POINT('Ctrl Pts',(7.51676407774738,108.574999999576,10.3459381770588));
#278217=CARTESIAN_POINT('Ctrl Pts',(9.83957192047847,108.724999999575,7.14886745759505));
#278218=CARTESIAN_POINT('Ctrl Pts',(12.1623797632096,108.874999999575,3.95179673813132));
#278219=CARTESIAN_POINT('Ctrl Pts',(12.1623797632096,109.024999999574,-1.48946194470292E-15));
#278220=CARTESIAN_POINT('Ctrl Pts',(12.1623797632096,109.174999999573,-3.95179673813132));
#278221=CARTESIAN_POINT('Ctrl Pts',(9.83957192047847,109.324999999573,-7.14886745759505));
#278222=CARTESIAN_POINT('Ctrl Pts',(7.51676407774738,109.474999999572,-10.3459381770588));
#278223=CARTESIAN_POINT('Ctrl Pts',(3.75838203887365,109.624999999572,-11.5671105274568));
#278224=CARTESIAN_POINT('Ctrl Pts',(-7.64804416691126E-14,109.774999999571,
-12.7882828778549));
#278225=CARTESIAN_POINT('Ctrl Pts',(-3.7583820388738,109.92499999957,-11.5671105274568));
#278226=CARTESIAN_POINT('Ctrl Pts',(-7.51676407774753,110.07499999957,-10.3459381770588));
#278227=CARTESIAN_POINT('Ctrl Pts',(-9.83957192047862,110.224999999569,
-7.14886745759505));
#278228=CARTESIAN_POINT('Ctrl Pts',(-12.1623797632097,110.374999999569,
-3.95179673813132));
#278229=CARTESIAN_POINT('Ctrl Pts',(-12.1623797632097,110.524999999568,
2.97892388940585E-15));
#278230=CARTESIAN_POINT('Ctrl Pts',(-12.1623797632097,110.674999999567,
3.95179673813133));
#278231=CARTESIAN_POINT('Ctrl Pts',(-9.83957192047862,110.824999999567,
7.14886745759505));
#278232=CARTESIAN_POINT('Ctrl Pts',(-7.51676407774753,110.974999999566,
10.3459381770588));
#278233=CARTESIAN_POINT('Ctrl Pts',(-3.7583820388738,111.124999999566,11.5671105274568));
#278234=CARTESIAN_POINT('Ctrl Pts',(-7.42120703663524E-14,111.274999999565,
12.7882828778549));
#278235=CARTESIAN_POINT('Ctrl Pts',(3.75838203887365,111.424999999564,11.5671105274568));
#278236=CARTESIAN_POINT('Ctrl Pts',(7.51676407774738,111.574999999564,10.3459381770588));
#278237=CARTESIAN_POINT('Ctrl Pts',(9.83957192047847,111.724999999563,7.14886745759505));
#278238=CARTESIAN_POINT('Ctrl Pts',(12.1623797632096,111.874999999563,3.95179673813132));
#278239=CARTESIAN_POINT('Ctrl Pts',(12.1623797632096,112.024999999562,-1.48946194470292E-15));
#278240=CARTESIAN_POINT('Ctrl Pts',(12.1623797632096,112.174999999561,-3.95179673813132));
#278241=CARTESIAN_POINT('Ctrl Pts',(9.83957192047847,112.324999999561,-7.14886745759505));
#278242=CARTESIAN_POINT('Ctrl Pts',(7.51676407774738,112.47499999956,-10.3459381770588));
#278243=CARTESIAN_POINT('Ctrl Pts',(3.75838203887365,112.62499999956,-11.5671105274568));
#278244=CARTESIAN_POINT('Ctrl Pts',(-7.82081509407745E-14,112.774999999559,
-12.7882828778549));
#278245=CARTESIAN_POINT('Ctrl Pts',(-3.75838203887381,112.924999999558,
-11.5671105274568));
#278246=CARTESIAN_POINT('Ctrl Pts',(-7.51676407774753,113.074999999558,
-10.3459381770588));
#278247=CARTESIAN_POINT('Ctrl Pts',(-9.83957192047863,113.224999999557,
-7.14886745759505));
#278248=CARTESIAN_POINT('Ctrl Pts',(-12.1623797632097,113.374999999557,
-3.95179673813132));
#278249=CARTESIAN_POINT('Ctrl Pts',(-12.1623797632097,113.524999999556,
2.97892388940585E-15));
#278250=CARTESIAN_POINT('Ctrl Pts',(-12.1623797632097,113.674999999555,
3.95179673813133));
#278251=CARTESIAN_POINT('Ctrl Pts',(-9.83957192047863,113.824999999555,
7.14886745759505));
#278252=CARTESIAN_POINT('Ctrl Pts',(-7.51676407774753,113.974999999554,
10.3459381770588));
#278253=CARTESIAN_POINT('Ctrl Pts',(-3.7583820388738,114.124999999554,11.5671105274568));
#278254=CARTESIAN_POINT('Ctrl Pts',(-7.59397796380142E-14,114.274999999553,
12.7882828778549));
#278255=CARTESIAN_POINT('Ctrl Pts',(3.75838203887365,114.424999999552,11.5671105274568));
#278256=CARTESIAN_POINT('Ctrl Pts',(7.51676407774738,114.574999999552,10.3459381770588));
#278257=CARTESIAN_POINT('Ctrl Pts',(9.83957192047847,114.724999999551,7.14886745759505));
#278258=CARTESIAN_POINT('Ctrl Pts',(12.1623797632096,114.874999999551,3.95179673813132));
#278259=CARTESIAN_POINT('Ctrl Pts',(12.1623797632096,115.02499999955,-1.48946194470292E-15));
#278260=CARTESIAN_POINT('Ctrl Pts',(12.1623797632096,115.174999999549,-3.95179673813132));
#278261=CARTESIAN_POINT('Ctrl Pts',(9.83957192047847,115.324999999549,-7.14886745759505));
#278262=CARTESIAN_POINT('Ctrl Pts',(7.51676407774738,115.474999999548,-10.3459381770588));
#278263=CARTESIAN_POINT('Ctrl Pts',(3.75838203887365,115.624999999548,-11.5671105274568));
#278264=CARTESIAN_POINT('Ctrl Pts',(-7.99358602124363E-14,115.774999999547,
-12.7882828778549));
#278265=CARTESIAN_POINT('Ctrl Pts',(-3.75838203887381,115.924999999546,
-11.5671105274568));
#278266=CARTESIAN_POINT('Ctrl Pts',(-7.51676407774754,116.074999999546,
-10.3459381770588));
#278267=CARTESIAN_POINT('Ctrl Pts',(-9.83957192047863,116.224999999545,
-7.14886745759505));
#278268=CARTESIAN_POINT('Ctrl Pts',(-12.1623797632097,116.374999999545,
-3.95179673813132));
#278269=CARTESIAN_POINT('Ctrl Pts',(-12.1623797632097,116.524999999544,
2.97892388940585E-15));
#278270=CARTESIAN_POINT('Ctrl Pts',(-12.1623797632097,116.674999999543,
3.95179673813133));
#278271=CARTESIAN_POINT('Ctrl Pts',(-9.83957192047863,116.824999999543,
7.14886745759505));
#278272=CARTESIAN_POINT('Ctrl Pts',(-7.51676407774753,116.974999999542,
10.3459381770588));
#278273=CARTESIAN_POINT('Ctrl Pts',(-3.75838203887381,117.124999999542,
11.5671105274568));
#278274=CARTESIAN_POINT('Ctrl Pts',(-7.76674889096761E-14,117.274999999541,
12.7882828778549));
#278275=CARTESIAN_POINT('Ctrl Pts',(3.75838203887365,117.42499999954,11.5671105274568));
#278276=CARTESIAN_POINT('Ctrl Pts',(7.51676407774738,117.57499999954,10.3459381770588));
#278277=CARTESIAN_POINT('Ctrl Pts',(9.83957192047847,117.724999999539,7.14886745759505));
#278278=CARTESIAN_POINT('Ctrl Pts',(12.1623797632096,117.874999999539,3.95179673813132));
#278279=CARTESIAN_POINT('Ctrl Pts',(12.1623797632096,118.024999999538,-1.48946194470292E-15));
#278280=CARTESIAN_POINT('Ctrl Pts',(12.1623797632096,118.174999999537,-3.95179673813132));
#278281=CARTESIAN_POINT('Ctrl Pts',(9.83957192047847,118.324999999537,-7.14886745759505));
#278282=CARTESIAN_POINT('Ctrl Pts',(7.51676407774737,118.474999999536,-10.3459381770588));
#278283=CARTESIAN_POINT('Ctrl Pts',(3.75838203887365,118.624999999536,-11.5671105274568));
#278284=CARTESIAN_POINT('Ctrl Pts',(-8.16635694840981E-14,118.774999999535,
-12.7882828778549));
#278285=CARTESIAN_POINT('Ctrl Pts',(-3.75838203887381,118.924999999534,
-11.5671105274568));
#278286=CARTESIAN_POINT('Ctrl Pts',(-7.51676407774754,119.074999999534,
-10.3459381770588));
#278287=CARTESIAN_POINT('Ctrl Pts',(-9.83957192047863,119.224999999533,
-7.14886745759505));
#278288=CARTESIAN_POINT('Ctrl Pts',(-12.1623797632097,119.374999999533,
-3.95179673813132));
#278289=CARTESIAN_POINT('Ctrl Pts',(-12.1623797632097,119.524999999532,
2.97892388940585E-15));
#278290=CARTESIAN_POINT('Ctrl Pts',(-12.1623797632097,119.674999999531,
3.95179673813133));
#278291=CARTESIAN_POINT('Ctrl Pts',(-9.83957192047863,119.824999999531,
7.14886745759505));
#278292=CARTESIAN_POINT('Ctrl Pts',(-7.51676407774754,119.97499999953,10.3459381770588));
#278293=CARTESIAN_POINT('Ctrl Pts',(-3.75838203887381,120.12499999953,11.5671105274568));
#278294=CARTESIAN_POINT('Ctrl Pts',(-7.93951981813379E-14,120.274999999529,
12.7882828778549));
#278295=CARTESIAN_POINT('Ctrl Pts',(3.75838203887365,120.424999999528,11.5671105274568));
#278296=CARTESIAN_POINT('Ctrl Pts',(7.51676407774738,120.574999999528,10.3459381770588));
#278297=CARTESIAN_POINT('Ctrl Pts',(9.83957192047847,120.724999999527,7.14886745759505));
#278298=CARTESIAN_POINT('Ctrl Pts',(12.1623797632096,120.874999999527,3.95179673813132));
#278299=CARTESIAN_POINT('Ctrl Pts',(12.1623797632096,121.024999999526,-1.48946194470292E-15));
#278300=CARTESIAN_POINT('Ctrl Pts',(12.1623797632096,121.174999999525,-3.95179673813132));
#278301=CARTESIAN_POINT('Ctrl Pts',(9.83957192047847,121.324999999525,-7.14886745759505));
#278302=CARTESIAN_POINT('Ctrl Pts',(7.51676407774737,121.474999999524,-10.3459381770588));
#278303=CARTESIAN_POINT('Ctrl Pts',(3.75838203887364,121.624999999524,-11.5671105274568));
#278304=CARTESIAN_POINT('Ctrl Pts',(-8.339127875576E-14,121.774999999523,
-12.7882828778549));
#278305=CARTESIAN_POINT('Ctrl Pts',(-3.75838203887381,121.924999999522,
-11.5671105274568));
#278306=CARTESIAN_POINT('Ctrl Pts',(-7.51676407774754,122.074999999522,
-10.3459381770588));
#278307=CARTESIAN_POINT('Ctrl Pts',(-9.83957192047863,122.224999999521,
-7.14886745759505));
#278308=CARTESIAN_POINT('Ctrl Pts',(-12.1623797632097,122.374999999521,
-3.95179673813132));
#278309=CARTESIAN_POINT('Ctrl Pts',(-12.1623797632097,122.52499999952,2.97892388940585E-15));
#278310=CARTESIAN_POINT('Ctrl Pts',(-12.1623797632097,122.674999999519,
3.95179673813133));
#278311=CARTESIAN_POINT('Ctrl Pts',(-9.83957192047863,122.824999999519,
7.14886745759505));
#278312=CARTESIAN_POINT('Ctrl Pts',(-7.51676407774754,122.974999999518,
10.3459381770588));
#278313=CARTESIAN_POINT('Ctrl Pts',(-3.75838203887381,123.124999999518,
11.5671105274568));
#278314=CARTESIAN_POINT('Ctrl Pts',(-8.11229074529997E-14,123.274999999517,
12.7882828778549));
#278315=CARTESIAN_POINT('Ctrl Pts',(3.75838203887365,123.424999999516,11.5671105274568));
#278316=CARTESIAN_POINT('Ctrl Pts',(7.51676407774737,123.574999999516,10.3459381770588));
#278317=CARTESIAN_POINT('Ctrl Pts',(9.83957192047846,123.724999999515,7.14886745759505));
#278318=CARTESIAN_POINT('Ctrl Pts',(12.1623797632096,123.874999999515,3.95179673813132));
#278319=CARTESIAN_POINT('Ctrl Pts',(12.1623797632096,124.024999999514,-1.48946194470292E-15));
#278320=CARTESIAN_POINT('Ctrl Pts',(12.1623797632096,124.174999999513,-3.95179673813132));
#278321=CARTESIAN_POINT('Ctrl Pts',(9.83957192047846,124.324999999513,-7.14886745759505));
#278322=CARTESIAN_POINT('Ctrl Pts',(7.51676407774737,124.474999999512,-10.3459381770588));
#278323=CARTESIAN_POINT('Ctrl Pts',(3.75838203887364,124.624999999512,-11.5671105274568));
#278324=CARTESIAN_POINT('Ctrl Pts',(-8.51189880274219E-14,124.774999999511,
-12.7882828778549));
#278325=CARTESIAN_POINT('Ctrl Pts',(-3.75838203887381,124.92499999951,-11.5671105274568));
#278326=CARTESIAN_POINT('Ctrl Pts',(-7.51676407774754,125.07499999951,-10.3459381770588));
#278327=CARTESIAN_POINT('Ctrl Pts',(-9.83957192047863,125.224999999509,
-7.14886745759505));
#278328=CARTESIAN_POINT('Ctrl Pts',(-12.1623797632097,125.374999999509,
-3.95179673813132));
#278329=CARTESIAN_POINT('Ctrl Pts',(-12.1623797632097,125.524999999508,
2.97892388940585E-15));
#278330=CARTESIAN_POINT('Ctrl Pts',(-12.1623797632097,125.674999999507,
3.95179673813133));
#278331=CARTESIAN_POINT('Ctrl Pts',(-9.83957192047863,125.824999999507,
7.14886745759505));
#278332=CARTESIAN_POINT('Ctrl Pts',(-7.51676407774754,125.974999999506,
10.3459381770588));
#278333=CARTESIAN_POINT('Ctrl Pts',(-3.75838203887381,126.124999999506,
11.5671105274568));
#278334=CARTESIAN_POINT('Ctrl Pts',(-8.28506167246616E-14,126.274999999505,
12.7882828778549));
#278335=CARTESIAN_POINT('Ctrl Pts',(3.75838203887364,126.424999999504,11.5671105274568));
#278336=CARTESIAN_POINT('Ctrl Pts',(7.51676407774737,126.574999999504,10.3459381770588));
#278337=CARTESIAN_POINT('Ctrl Pts',(9.83957192047846,126.724999999503,7.14886745759505));
#278338=CARTESIAN_POINT('Ctrl Pts',(12.1623797632096,126.874999999503,3.95179673813132));
#278339=CARTESIAN_POINT('Ctrl Pts',(12.1623797632096,127.024999999502,-1.48946194470292E-15));
#278340=CARTESIAN_POINT('Ctrl Pts',(12.1623797632096,127.174999999501,-3.95179673813132));
#278341=CARTESIAN_POINT('Ctrl Pts',(9.83957192047846,127.324999999501,-7.14886745759505));
#278342=CARTESIAN_POINT('Ctrl Pts',(7.51676407774737,127.4749999995,-10.3459381770588));
#278343=CARTESIAN_POINT('Ctrl Pts',(3.75838203887364,127.6249999995,-11.5671105274568));
#278344=CARTESIAN_POINT('Ctrl Pts',(-8.68466972990837E-14,127.774999999499,
-12.7882828778549));
#278345=CARTESIAN_POINT('Ctrl Pts',(-3.75838203887381,127.924999999498,
-11.5671105274568));
#278346=CARTESIAN_POINT('Ctrl Pts',(-7.51676407774754,128.074999999498,
-10.3459381770588));
#278347=CARTESIAN_POINT('Ctrl Pts',(-9.83957192047864,128.224999999497,
-7.14886745759505));
#278348=CARTESIAN_POINT('Ctrl Pts',(-12.1623797632097,128.374999999497,
-3.95179673813132));
#278349=CARTESIAN_POINT('Ctrl Pts',(-12.1623797632097,128.524999999496,
2.97892388940585E-15));
#278350=CARTESIAN_POINT('Ctrl Pts',(-12.1623797632097,128.674999999495,
3.95179673813133));
#278351=CARTESIAN_POINT('Ctrl Pts',(-9.83957192047864,128.824999999495,
7.14886745759505));
#278352=CARTESIAN_POINT('Ctrl Pts',(-7.51676407774754,128.974999999494,
10.3459381770588));
#278353=CARTESIAN_POINT('Ctrl Pts',(-3.75838203887381,129.124999999494,
11.5671105274568));
#278354=CARTESIAN_POINT('Ctrl Pts',(-8.45783259963234E-14,129.274999999493,
12.7882828778549));
#278355=CARTESIAN_POINT('Ctrl Pts',(3.75838203887364,129.424999999492,11.5671105274568));
#278356=CARTESIAN_POINT('Ctrl Pts',(7.51676407774737,129.574999999492,10.3459381770588));
#278357=CARTESIAN_POINT('Ctrl Pts',(9.83957192047846,129.724999999491,7.14886745759505));
#278358=CARTESIAN_POINT('Ctrl Pts',(12.1623797632096,129.874999999491,3.95179673813132));
#278359=CARTESIAN_POINT('Ctrl Pts',(12.1623797632096,130.02499999949,-1.48946194470292E-15));
#278360=CARTESIAN_POINT('Ctrl Pts',(12.1623797632096,130.174999999489,-3.95179673813132));
#278361=CARTESIAN_POINT('Ctrl Pts',(9.83957192047846,130.324999999489,-7.14886745759505));
#278362=CARTESIAN_POINT('Ctrl Pts',(7.51676407774737,130.474999999488,-10.3459381770588));
#278363=CARTESIAN_POINT('Ctrl Pts',(3.75838203887364,130.624999999488,-11.5671105274568));
#278364=CARTESIAN_POINT('Ctrl Pts',(-8.85744065707455E-14,130.774999999487,
-12.7882828778549));
#278365=CARTESIAN_POINT('Ctrl Pts',(-3.75838203887382,130.924999999486,
-11.5671105274568));
#278366=CARTESIAN_POINT('Ctrl Pts',(-7.51676407774754,131.074999999486,
-10.3459381770588));
#278367=CARTESIAN_POINT('Ctrl Pts',(-9.83957192047864,131.224999999485,
-7.14886745759505));
#278368=CARTESIAN_POINT('Ctrl Pts',(-12.1623797632097,131.374999999485,
-3.95179673813132));
#278369=CARTESIAN_POINT('Ctrl Pts',(-12.1623797632097,131.524999999484,
2.97892388940585E-15));
#278370=CARTESIAN_POINT('Ctrl Pts',(-12.1623797632097,131.674999999483,
3.95179673813133));
#278371=CARTESIAN_POINT('Ctrl Pts',(-9.83957192047864,131.824999999483,
7.14886745759505));
#278372=CARTESIAN_POINT('Ctrl Pts',(-7.51676407774754,131.974999999482,
10.3459381770588));
#278373=CARTESIAN_POINT('Ctrl Pts',(-3.75838203887381,132.124999999482,
11.5671105274568));
#278374=CARTESIAN_POINT('Ctrl Pts',(-8.63060352679853E-14,132.274999999481,
12.7882828778549));
#278375=CARTESIAN_POINT('Ctrl Pts',(3.75838203887364,132.42499999948,11.5671105274568));
#278376=CARTESIAN_POINT('Ctrl Pts',(7.51676407774737,132.57499999948,10.3459381770588));
#278377=CARTESIAN_POINT('Ctrl Pts',(9.83957192047846,132.724999999479,7.14886745759505));
#278378=CARTESIAN_POINT('Ctrl Pts',(12.1623797632096,132.874999999479,3.95179673813132));
#278379=CARTESIAN_POINT('Ctrl Pts',(12.1623797632096,133.024999999478,-1.48946194470292E-15));
#278380=CARTESIAN_POINT('Ctrl Pts',(12.1623797632096,133.174999999477,-3.95179673813132));
#278381=CARTESIAN_POINT('Ctrl Pts',(9.83957192047846,133.324999999477,-7.14886745759505));
#278382=CARTESIAN_POINT('Ctrl Pts',(7.51676407774736,133.474999999476,-10.3459381770588));
#278383=CARTESIAN_POINT('Ctrl Pts',(3.75838203887364,133.624999999476,-11.5671105274568));
#278384=CARTESIAN_POINT('Ctrl Pts',(-9.03021158424074E-14,133.774999999475,
-12.7882828778549));
#278385=CARTESIAN_POINT('Ctrl Pts',(-3.75838203887382,133.924999999474,
-11.5671105274568));
#278386=CARTESIAN_POINT('Ctrl Pts',(-7.51676407774755,134.074999999474,
-10.3459381770588));
#278387=CARTESIAN_POINT('Ctrl Pts',(-9.83957192047864,134.224999999473,
-7.14886745759505));
#278388=CARTESIAN_POINT('Ctrl Pts',(-12.1623797632097,134.374999999473,
-3.95179673813132));
#278389=CARTESIAN_POINT('Ctrl Pts',(-12.1623797632097,134.524999999472,
2.97892388940585E-15));
#278390=CARTESIAN_POINT('Ctrl Pts',(-12.1623797632097,134.674999999471,
3.95179673813133));
#278391=CARTESIAN_POINT('Ctrl Pts',(-9.83957192047864,134.824999999471,
7.14886745759505));
#278392=CARTESIAN_POINT('Ctrl Pts',(-7.51676407774754,134.97499999947,10.3459381770588));
#278393=CARTESIAN_POINT('Ctrl Pts',(-3.75838203887382,135.12499999947,11.5671105274568));
#278394=CARTESIAN_POINT('Ctrl Pts',(-8.80337445396471E-14,135.274999999469,
12.7882828778549));
#278395=CARTESIAN_POINT('Ctrl Pts',(3.75838203887364,135.424999999468,11.5671105274568));
#278396=CARTESIAN_POINT('Ctrl Pts',(7.51676407774737,135.574999999468,10.3459381770588));
#278397=CARTESIAN_POINT('Ctrl Pts',(9.83957192047846,135.724999999467,7.14886745759505));
#278398=CARTESIAN_POINT('Ctrl Pts',(12.1623797632096,135.874999999467,3.95179673813132));
#278399=CARTESIAN_POINT('Ctrl Pts',(12.1623797632096,136.024999999466,-1.48946194470292E-15));
#278400=CARTESIAN_POINT('Ctrl Pts',(12.1623797632095,136.174999999465,-3.95179673813132));
#278401=CARTESIAN_POINT('Ctrl Pts',(9.83957192047846,136.324999999465,-7.14886745759505));
#278402=CARTESIAN_POINT('Ctrl Pts',(7.51676407774736,136.474999999464,-10.3459381770588));
#278403=CARTESIAN_POINT('Ctrl Pts',(3.75838203887364,136.624999999464,-11.5671105274568));
#278404=CARTESIAN_POINT('Ctrl Pts',(-9.20298251140692E-14,136.774999999463,
-12.7882828778549));
#278405=CARTESIAN_POINT('Ctrl Pts',(-3.75838203887382,136.924999999462,
-11.5671105274568));
#278406=CARTESIAN_POINT('Ctrl Pts',(-7.51676407774755,137.074999999462,
-10.3459381770588));
#278407=CARTESIAN_POINT('Ctrl Pts',(-9.83957192047864,137.224999999461,
-7.14886745759505));
#278408=CARTESIAN_POINT('Ctrl Pts',(-12.1623797632097,137.374999999461,
-3.95179673813132));
#278409=CARTESIAN_POINT('Ctrl Pts',(-12.1623797632097,137.52499999946,2.97892388940585E-15));
#278410=CARTESIAN_POINT('Ctrl Pts',(-12.1623797632097,137.674999999459,
3.95179673813133));
#278411=CARTESIAN_POINT('Ctrl Pts',(-9.83957192047864,137.824999999459,
7.14886745759505));
#278412=CARTESIAN_POINT('Ctrl Pts',(-7.51676407774755,137.974999999458,
10.3459381770588));
#278413=CARTESIAN_POINT('Ctrl Pts',(-3.75838203887382,138.124999999458,
11.5671105274568));
#278414=CARTESIAN_POINT('Ctrl Pts',(-8.97614538113089E-14,138.274999999457,
12.7882828778549));
#278415=CARTESIAN_POINT('Ctrl Pts',(3.75838203887364,138.424999999456,11.5671105274568));
#278416=CARTESIAN_POINT('Ctrl Pts',(7.51676407774736,138.574999999456,10.3459381770588));
#278417=CARTESIAN_POINT('Ctrl Pts',(9.83957192047846,138.724999999455,7.14886745759505));
#278418=CARTESIAN_POINT('Ctrl Pts',(12.1623797632096,138.874999999455,3.95179673813132));
#278419=CARTESIAN_POINT('Ctrl Pts',(12.1623797632096,139.024999999454,-1.48946194470292E-15));
#278420=CARTESIAN_POINT('Ctrl Pts',(12.1623797632095,139.174999999453,-3.95179673813132));
#278421=CARTESIAN_POINT('Ctrl Pts',(9.83957192047846,139.324999999453,-7.14886745759505));
#278422=CARTESIAN_POINT('Ctrl Pts',(7.51676407774736,139.474999999452,-10.3459381770588));
#278423=CARTESIAN_POINT('Ctrl Pts',(3.75838203887363,139.624999999452,-11.5671105274568));
#278424=CARTESIAN_POINT('Ctrl Pts',(-9.3757534385731E-14,139.774999999451,
-12.7882828778549));
#278425=CARTESIAN_POINT('Ctrl Pts',(-3.75838203887382,139.92499999945,-11.5671105274568));
#278426=CARTESIAN_POINT('Ctrl Pts',(-7.51676407774755,140.07499999945,-10.3459381770588));
#278427=CARTESIAN_POINT('Ctrl Pts',(-9.83957192047864,140.224999999449,
-7.14886745759505));
#278428=CARTESIAN_POINT('Ctrl Pts',(-12.1623797632097,140.374999999449,
-3.95179673813132));
#278429=CARTESIAN_POINT('Ctrl Pts',(-12.1623797632097,140.524999999448,
2.97892388940585E-15));
#278430=CARTESIAN_POINT('Ctrl Pts',(-12.1623797632097,140.674999999447,
3.95179673813133));
#278431=CARTESIAN_POINT('Ctrl Pts',(-9.83957192047864,140.824999999447,
7.14886745759505));
#278432=CARTESIAN_POINT('Ctrl Pts',(-7.51676407774755,140.974999999446,
10.3459381770588));
#278433=CARTESIAN_POINT('Ctrl Pts',(-3.75838203887382,141.124999999446,
11.5671105274568));
#278434=CARTESIAN_POINT('Ctrl Pts',(-9.14891630829708E-14,141.274999999445,
12.7882828778549));
#278435=CARTESIAN_POINT('Ctrl Pts',(3.75838203887364,141.424999999444,11.5671105274568));
#278436=CARTESIAN_POINT('Ctrl Pts',(7.51676407774736,141.574999999444,10.3459381770588));
#278437=CARTESIAN_POINT('Ctrl Pts',(9.83957192047845,141.724999999443,7.14886745759505));
#278438=CARTESIAN_POINT('Ctrl Pts',(12.1623797632095,141.874999999443,3.95179673813132));
#278439=CARTESIAN_POINT('Ctrl Pts',(12.1623797632095,142.024999999442,-1.48946194470292E-15));
#278440=CARTESIAN_POINT('Ctrl Pts',(12.1623797632095,142.174999999441,-3.95179673813132));
#278441=CARTESIAN_POINT('Ctrl Pts',(9.83957192047845,142.324999999441,-7.14886745759505));
#278442=CARTESIAN_POINT('Ctrl Pts',(7.51676407774736,142.47499999944,-10.3459381770588));
#278443=CARTESIAN_POINT('Ctrl Pts',(3.75838203887363,142.62499999944,-11.5671105274568));
#278444=CARTESIAN_POINT('Ctrl Pts',(-9.54852436573929E-14,142.774999999439,
-12.7882828778549));
#278445=CARTESIAN_POINT('Ctrl Pts',(-3.75838203887382,142.924999999438,
-11.5671105274568));
#278446=CARTESIAN_POINT('Ctrl Pts',(-7.51676407774755,143.074999999438,
-10.3459381770588));
#278447=CARTESIAN_POINT('Ctrl Pts',(-9.83957192047864,143.224999999437,
-7.14886745759505));
#278448=CARTESIAN_POINT('Ctrl Pts',(-12.1623797632097,143.374999999437,
-3.95179673813132));
#278449=CARTESIAN_POINT('Ctrl Pts',(-12.1623797632097,143.524999999436,
2.97892388940585E-15));
#278450=CARTESIAN_POINT('Ctrl Pts',(-12.1623797632097,143.674999999435,
3.95179673813133));
#278451=CARTESIAN_POINT('Ctrl Pts',(-9.83957192047864,143.824999999435,
7.14886745759505));
#278452=CARTESIAN_POINT('Ctrl Pts',(-7.51676407774755,143.974999999434,
10.3459381770588));
#278453=CARTESIAN_POINT('Ctrl Pts',(-3.75838203887382,144.124999999434,
11.5671105274568));
#278454=CARTESIAN_POINT('Ctrl Pts',(-9.32168723546326E-14,144.274999999433,
12.7882828778549));
#278455=CARTESIAN_POINT('Ctrl Pts',(3.75838203887363,144.424999999432,11.5671105274568));
#278456=CARTESIAN_POINT('Ctrl Pts',(7.51676407774736,144.574999999432,10.3459381770588));
#278457=CARTESIAN_POINT('Ctrl Pts',(9.83957192047845,144.724999999431,7.14886745759505));
#278458=CARTESIAN_POINT('Ctrl Pts',(12.1623797632095,144.874999999431,3.95179673813132));
#278459=CARTESIAN_POINT('Ctrl Pts',(12.1623797632095,145.02499999943,-1.48946194470292E-15));
#278460=CARTESIAN_POINT('Ctrl Pts',(12.1623797632095,145.174999999429,-3.95179673813132));
#278461=CARTESIAN_POINT('Ctrl Pts',(9.83957192047845,145.324999999429,-7.14886745759505));
#278462=CARTESIAN_POINT('Ctrl Pts',(7.51676407774736,145.474999999428,-10.3459381770588));
#278463=CARTESIAN_POINT('Ctrl Pts',(3.75838203887363,145.624999999428,-11.5671105274568));
#278464=CARTESIAN_POINT('Ctrl Pts',(-9.72129529290547E-14,145.774999999427,
-12.7882828778549));
#278465=CARTESIAN_POINT('Ctrl Pts',(-3.75838203887382,145.924999999426,
-11.5671105274568));
#278466=CARTESIAN_POINT('Ctrl Pts',(-7.51676407774755,146.074999999426,
-10.3459381770588));
#278467=CARTESIAN_POINT('Ctrl Pts',(-9.83957192047865,146.224999999425,
-7.14886745759505));
#278468=CARTESIAN_POINT('Ctrl Pts',(-12.1623797632097,146.374999999425,
-3.95179673813132));
#278469=CARTESIAN_POINT('Ctrl Pts',(-12.1623797632097,146.524999999424,
2.97892388940585E-15));
#278470=CARTESIAN_POINT('Ctrl Pts',(-12.1623797632097,146.674999999423,
3.95179673813133));
#278471=CARTESIAN_POINT('Ctrl Pts',(-9.83957192047865,146.824999999423,
7.14886745759505));
#278472=CARTESIAN_POINT('Ctrl Pts',(-7.51676407774755,146.974999999422,
10.3459381770588));
#278473=CARTESIAN_POINT('Ctrl Pts',(-3.75838203887382,147.124999999422,
11.5671105274568));
#278474=CARTESIAN_POINT('Ctrl Pts',(-9.49445816262944E-14,147.274999999421,
12.7882828778549));
#278475=CARTESIAN_POINT('Ctrl Pts',(3.75838203887363,147.42499999942,11.5671105274568));
#278476=CARTESIAN_POINT('Ctrl Pts',(7.51676407774736,147.57499999942,10.3459381770588));
#278477=CARTESIAN_POINT('Ctrl Pts',(9.83957192047845,147.724999999419,7.14886745759505));
#278478=CARTESIAN_POINT('Ctrl Pts',(12.1623797632095,147.874999999419,3.95179673813132));
#278479=CARTESIAN_POINT('Ctrl Pts',(12.1623797632095,148.024999999418,-1.48946194470292E-15));
#278480=CARTESIAN_POINT('Ctrl Pts',(12.1623797632095,148.174999999417,-3.95179673813132));
#278481=CARTESIAN_POINT('Ctrl Pts',(9.83957192047845,148.324999999417,-7.14886745759505));
#278482=CARTESIAN_POINT('Ctrl Pts',(7.51676407774736,148.474999999416,-10.3459381770588));
#278483=CARTESIAN_POINT('Ctrl Pts',(3.75838203887363,148.624999999416,-11.5671105274568));
#278484=CARTESIAN_POINT('Ctrl Pts',(-9.89406622007166E-14,148.774999999415,
-12.7882828778549));
#278485=CARTESIAN_POINT('Ctrl Pts',(-3.75838203887383,148.924999999414,
-11.5671105274568));
#278486=CARTESIAN_POINT('Ctrl Pts',(-7.51676407774756,149.074999999414,
-10.3459381770588));
#278487=CARTESIAN_POINT('Ctrl Pts',(-9.83957192047865,149.224999999413,
-7.14886745759505));
#278488=CARTESIAN_POINT('Ctrl Pts',(-12.1623797632097,149.374999999413,
-3.95179673813132));
#278489=CARTESIAN_POINT('Ctrl Pts',(-12.1623797632097,149.524999999412,
2.97892388940585E-15));
#278490=CARTESIAN_POINT('Ctrl Pts',(-12.1623797632097,149.674999999411,
3.95179673813133));
#278491=CARTESIAN_POINT('Ctrl Pts',(-9.83957192047865,149.824999999411,
7.14886745759505));
#278492=CARTESIAN_POINT('Ctrl Pts',(-7.51676407774755,149.97499999941,10.3459381770588));
#278493=CARTESIAN_POINT('Ctrl Pts',(-3.75838203887382,150.12499999941,11.5671105274568));
#278494=CARTESIAN_POINT('Ctrl Pts',(-9.66722908979563E-14,150.274999999409,
12.7882828778549));
#278495=CARTESIAN_POINT('Ctrl Pts',(3.75838203887363,150.424999999408,11.5671105274568));
#278496=CARTESIAN_POINT('Ctrl Pts',(7.51676407774736,150.574999999408,10.3459381770588));
#278497=CARTESIAN_POINT('Ctrl Pts',(9.83957192047845,150.724999999407,7.14886745759505));
#278498=CARTESIAN_POINT('Ctrl Pts',(12.1623797632095,150.874999999407,3.95179673813132));
#278499=CARTESIAN_POINT('Ctrl Pts',(12.1623797632095,151.024999999406,-1.48946194470292E-15));
#278500=CARTESIAN_POINT('Ctrl Pts',(12.1623797632095,151.174999999405,-3.95179673813132));
#278501=CARTESIAN_POINT('Ctrl Pts',(9.83957192047845,151.324999999405,-7.14886745759505));
#278502=CARTESIAN_POINT('Ctrl Pts',(7.51676407774736,151.474999999404,-10.3459381770588));
#278503=CARTESIAN_POINT('Ctrl Pts',(3.75838203887363,151.624999999404,-11.5671105274568));
#278504=CARTESIAN_POINT('Ctrl Pts',(-1.00668371472378E-13,151.774999999403,
-12.7882828778549));
#278505=CARTESIAN_POINT('Ctrl Pts',(-3.75838203887383,151.924999999402,
-11.5671105274568));
#278506=CARTESIAN_POINT('Ctrl Pts',(-7.51676407774756,152.074999999402,
-10.3459381770588));
#278507=CARTESIAN_POINT('Ctrl Pts',(-9.83957192047865,152.224999999401,
-7.14886745759505));
#278508=CARTESIAN_POINT('Ctrl Pts',(-12.1623797632097,152.374999999401,
-3.95179673813132));
#278509=CARTESIAN_POINT('Ctrl Pts',(-12.1623797632097,152.5249999994,2.97892388940585E-15));
#278510=CARTESIAN_POINT('Ctrl Pts',(-12.1623797632097,152.674999999399,
3.95179673813133));
#278511=CARTESIAN_POINT('Ctrl Pts',(-9.83957192047865,152.824999999399,
7.14886745759505));
#278512=CARTESIAN_POINT('Ctrl Pts',(-7.51676407774756,152.974999999398,
10.3459381770588));
#278513=CARTESIAN_POINT('Ctrl Pts',(-3.75838203887383,153.124999999398,
11.5671105274568));
#278514=CARTESIAN_POINT('Ctrl Pts',(-9.84000001696181E-14,153.274999999397,
12.7882828778549));
#278515=CARTESIAN_POINT('Ctrl Pts',(3.75838203887363,153.424999999396,11.5671105274568));
#278516=CARTESIAN_POINT('Ctrl Pts',(7.51676407774736,153.574999999396,10.3459381770588));
#278517=CARTESIAN_POINT('Ctrl Pts',(9.83957192047845,153.724999999395,7.14886745759505));
#278518=CARTESIAN_POINT('Ctrl Pts',(12.1623797632095,153.874999999395,3.95179673813132));
#278519=CARTESIAN_POINT('Ctrl Pts',(12.1623797632095,154.024999999394,-1.48946194470292E-15));
#278520=CARTESIAN_POINT('Ctrl Pts',(12.1623797632095,154.174999999393,-3.95179673813132));
#278521=CARTESIAN_POINT('Ctrl Pts',(9.83957192047845,154.324999999393,-7.14886745759505));
#278522=CARTESIAN_POINT('Ctrl Pts',(7.51676407774735,154.474999999392,-10.3459381770588));
#278523=CARTESIAN_POINT('Ctrl Pts',(3.75838203887363,154.624999999392,-11.5671105274568));
#278524=CARTESIAN_POINT('Ctrl Pts',(-1.0239608074404E-13,154.774999999391,
-12.7882828778549));
#278525=CARTESIAN_POINT('Ctrl Pts',(-3.75838203887383,154.92499999939,-11.5671105274568));
#278526=CARTESIAN_POINT('Ctrl Pts',(10.0514428414941,95.8062499996273,-1.23094673026484E-15));
#278527=CARTESIAN_POINT('Ctrl Pts',(10.0514428414941,95.9562499996266,-3.26591175476071));
#278528=CARTESIAN_POINT('Ctrl Pts',(8.13178807675712,96.1062499996261,-5.90808986649102));
#278529=CARTESIAN_POINT('Ctrl Pts',(6.21213331202015,96.2562499996255,-8.55026797822134));
#278530=CARTESIAN_POINT('Ctrl Pts',(3.10606665601004,96.4062499996248,-9.5594902125713));
#278531=CARTESIAN_POINT('Ctrl Pts',(-6.87318131996666E-14,96.5562499996243,
-10.5687124469213));
#278532=CARTESIAN_POINT('Ctrl Pts',(-3.10606665601018,96.7062499996236,
-9.5594902125713));
#278533=CARTESIAN_POINT('Ctrl Pts',(-6.21213331202028,96.856249999623,-8.55026797822134));
#278534=CARTESIAN_POINT('Ctrl Pts',(-8.13178807675726,97.0062499996224,
-5.90808986649102));
#278535=CARTESIAN_POINT('Ctrl Pts',(-10.0514428414942,97.1562499996218,
-3.2659117547607));
#278536=CARTESIAN_POINT('Ctrl Pts',(-10.0514428414942,97.3062499996212,
2.46189346052968E-15));
#278537=CARTESIAN_POINT('Ctrl Pts',(-10.0514428414942,97.4562499996206,
3.26591175476071));
#278538=CARTESIAN_POINT('Ctrl Pts',(-8.13178807675726,97.60624999962,5.90808986649102));
#278539=CARTESIAN_POINT('Ctrl Pts',(-6.21213331202028,97.7562499996194,
8.55026797822134));
#278540=CARTESIAN_POINT('Ctrl Pts',(-3.10606665601018,97.9062499996189,
9.5594902125713));
#278541=CARTESIAN_POINT('Ctrl Pts',(-6.70070798616514E-14,98.0562499996182,
10.5687124469213));
#278542=CARTESIAN_POINT('Ctrl Pts',(3.10606665601004,98.2062499996177,9.5594902125713));
#278543=CARTESIAN_POINT('Ctrl Pts',(6.21213331202015,98.3562499996171,8.55026797822134));
#278544=CARTESIAN_POINT('Ctrl Pts',(8.13178807675712,98.5062499996165,5.90808986649102));
#278545=CARTESIAN_POINT('Ctrl Pts',(10.0514428414941,98.6562499996158,3.2659117547607));
#278546=CARTESIAN_POINT('Ctrl Pts',(10.0514428414941,98.8062499996153,-1.23094673026484E-15));
#278547=CARTESIAN_POINT('Ctrl Pts',(-12.1623797632103,-3.28749999997638,
2.97892388940601E-15));
#278548=CARTESIAN_POINT('Ctrl Pts',(-12.1623797632103,-3.13749999997698,
3.95179673813154));
#278549=CARTESIAN_POINT('Ctrl Pts',(-9.83957192047908,-2.98749999997758,
7.14886745759543));
#278550=CARTESIAN_POINT('Ctrl Pts',(-7.51676407774787,-2.83749999997817,
10.3459381770593));
#278551=CARTESIAN_POINT('Ctrl Pts',(-3.75838203887394,-2.68749999997877,
11.5671105274575));
#278552=CARTESIAN_POINT('Ctrl Pts',(-8.66709987268145E-15,-2.53749999997937,
12.7882828778556));
#278553=CARTESIAN_POINT('Ctrl Pts',(3.75838203887392,-2.38749999997997,
11.5671105274575));
#278554=CARTESIAN_POINT('Ctrl Pts',(7.51676407774785,-2.23749999998057,
10.3459381770593));
#278555=CARTESIAN_POINT('Ctrl Pts',(9.83957192047906,-2.08749999998117,
7.14886745759543));
#278556=CARTESIAN_POINT('Ctrl Pts',(12.1623797632103,-1.93749999998176,
3.95179673813153));
#278557=CARTESIAN_POINT('Ctrl Pts',(12.1623797632103,-1.78749999998236,
-1.489461944703E-15));
#278558=CARTESIAN_POINT('Ctrl Pts',(12.1623797632103,-1.63749999998296,
-3.95179673813154));
#278559=CARTESIAN_POINT('Ctrl Pts',(9.83957192047906,-1.48749999998357,
-7.14886745759543));
#278560=CARTESIAN_POINT('Ctrl Pts',(7.51676407774784,-1.33749999998417,
-10.3459381770593));
#278561=CARTESIAN_POINT('Ctrl Pts',(3.75838203887392,-1.18749999998477,
-11.5671105274575));
#278562=CARTESIAN_POINT('Ctrl Pts',(-1.26631804471037E-14,-1.03749999998537,
-12.7882828778556));
#278563=CARTESIAN_POINT('Ctrl Pts',(-3.75838203887394,-0.887499999985973,
-11.5671105274575));
#278564=CARTESIAN_POINT('Ctrl Pts',(-7.51676407774787,-0.737499999986575,
-10.3459381770593));
#278565=CARTESIAN_POINT('Ctrl Pts',(-9.83957192047909,-0.587499999987176,
-7.14886745759543));
#278566=CARTESIAN_POINT('Ctrl Pts',(-12.1623797632103,-0.437499999987778,
-3.95179673813153));
#278567=CARTESIAN_POINT('Ctrl Pts',(-12.1623797632103,-0.287499999988378,
2.97892388940601E-15));
#278568=CARTESIAN_POINT('Ctrl Pts',(-12.1623797632103,-0.137499999988978,
3.95179673813154));
#278569=CARTESIAN_POINT('Ctrl Pts',(-9.83957192047909,0.0125000000104236,
7.14886745759543));
#278570=CARTESIAN_POINT('Ctrl Pts',(-7.51676407774787,0.162500000009825,
10.3459381770593));
#278571=CARTESIAN_POINT('Ctrl Pts',(-3.75838203887394,0.312500000009227,
11.5671105274575));
#278572=CARTESIAN_POINT('Ctrl Pts',(-1.03948091443433E-14,0.462500000008629,
12.7882828778556));
#278573=CARTESIAN_POINT('Ctrl Pts',(3.75838203887392,0.612500000008031,
11.5671105274575));
#278574=CARTESIAN_POINT('Ctrl Pts',(7.51676407774785,0.762500000007433,
10.3459381770593));
#278575=CARTESIAN_POINT('Ctrl Pts',(9.83957192047906,0.912500000006835,
7.14886745759543));
#278576=CARTESIAN_POINT('Ctrl Pts',(12.1623797632103,1.06250000000624,3.95179673813153));
#278577=CARTESIAN_POINT('Ctrl Pts',(12.1623797632103,1.21250000000564,-1.489461944703E-15));
#278578=CARTESIAN_POINT('Ctrl Pts',(12.1623797632103,1.36250000000504,-3.95179673813154));
#278579=CARTESIAN_POINT('Ctrl Pts',(9.83957192047906,1.51250000000444,-7.14886745759543));
#278580=CARTESIAN_POINT('Ctrl Pts',(7.51676407774784,1.66250000000383,-10.3459381770593));
#278581=CARTESIAN_POINT('Ctrl Pts',(3.75838203887391,1.81250000000323,-11.5671105274575));
#278582=CARTESIAN_POINT('Ctrl Pts',(-1.43908897187656E-14,1.96250000000263,
-12.7882828778556));
#278583=CARTESIAN_POINT('Ctrl Pts',(-3.75838203887394,2.11250000000203,
-11.5671105274575));
#278584=CARTESIAN_POINT('Ctrl Pts',(-7.51676407774787,2.26250000000143,
-10.3459381770593));
#278585=CARTESIAN_POINT('Ctrl Pts',(-9.83957192047909,2.41250000000082,
-7.14886745759543));
#278586=CARTESIAN_POINT('Ctrl Pts',(-12.1623797632103,2.56250000000022,
-3.95179673813153));
#278587=CARTESIAN_POINT('Ctrl Pts',(-12.1623797632103,2.71249999999962,
2.97892388940601E-15));
#278588=CARTESIAN_POINT('Ctrl Pts',(-12.1623797632103,2.86249999999902,
3.95179673813154));
#278589=CARTESIAN_POINT('Ctrl Pts',(-9.83957192047909,3.01249999999842,
7.14886745759543));
#278590=CARTESIAN_POINT('Ctrl Pts',(-7.51676407774787,3.16249999999782,
10.3459381770593));
#278591=CARTESIAN_POINT('Ctrl Pts',(-3.75838203887394,3.31249999999723,
11.5671105274575));
#278592=CARTESIAN_POINT('Ctrl Pts',(-1.21225184160051E-14,3.46249999999663,
12.7882828778556));
#278593=CARTESIAN_POINT('Ctrl Pts',(3.75838203887392,3.61249999999603,11.5671105274575));
#278594=CARTESIAN_POINT('Ctrl Pts',(7.51676407774784,3.76249999999543,10.3459381770593));
#278595=CARTESIAN_POINT('Ctrl Pts',(9.83957192047906,3.91249999999483,7.14886745759543));
#278596=CARTESIAN_POINT('Ctrl Pts',(12.1623797632103,4.06249999999424,3.95179673813153));
#278597=CARTESIAN_POINT('Ctrl Pts',(12.1623797632103,4.21249999999364,-1.489461944703E-15));
#278598=CARTESIAN_POINT('Ctrl Pts',(12.1623797632103,4.36249999999303,-3.95179673813154));
#278599=CARTESIAN_POINT('Ctrl Pts',(9.83957192047906,4.51249999999243,-7.14886745759543));
#278600=CARTESIAN_POINT('Ctrl Pts',(7.51676407774784,4.66249999999183,-10.3459381770593));
#278601=CARTESIAN_POINT('Ctrl Pts',(3.75838203887391,4.81249999999123,-11.5671105274575));
#278602=CARTESIAN_POINT('Ctrl Pts',(-1.61185989904274E-14,4.96249999999063,
-12.7882828778556));
#278603=CARTESIAN_POINT('Ctrl Pts',(-3.75838203887394,5.11249999999003,
-11.5671105274575));
#278604=CARTESIAN_POINT('Ctrl Pts',(-7.51676407774788,5.26249999998942,
-10.3459381770593));
#278605=CARTESIAN_POINT('Ctrl Pts',(-9.83957192047909,5.41249999998882,
-7.14886745759543));
#278606=CARTESIAN_POINT('Ctrl Pts',(-12.1623797632103,5.56249999998822,
-3.95179673813153));
#278607=CARTESIAN_POINT('Ctrl Pts',(-12.1623797632103,5.71249999998762,
2.97892388940601E-15));
#278608=CARTESIAN_POINT('Ctrl Pts',(-12.1623797632103,5.86249999998702,
3.95179673813154));
#278609=CARTESIAN_POINT('Ctrl Pts',(-9.83957192047909,6.01249999998642,
7.14886745759543));
#278610=CARTESIAN_POINT('Ctrl Pts',(-7.51676407774787,6.16249999998582,
10.3459381770593));
#278611=CARTESIAN_POINT('Ctrl Pts',(-3.75838203887394,6.31249999998523,
11.5671105274575));
#278612=CARTESIAN_POINT('Ctrl Pts',(-1.3850227687667E-14,6.46249999998463,
12.7882828778556));
#278613=CARTESIAN_POINT('Ctrl Pts',(3.75838203887392,6.61249999998403,11.5671105274575));
#278614=CARTESIAN_POINT('Ctrl Pts',(7.51676407774784,6.76249999998343,10.3459381770593));
#278615=CARTESIAN_POINT('Ctrl Pts',(9.83957192047906,6.91249999998283,7.14886745759543));
#278616=CARTESIAN_POINT('Ctrl Pts',(12.1623797632103,7.06249999998224,3.95179673813153));
#278617=CARTESIAN_POINT('Ctrl Pts',(12.1623797632103,7.21249999998164,-1.489461944703E-15));
#278618=CARTESIAN_POINT('Ctrl Pts',(12.1623797632103,7.36249999998104,-3.95179673813154));
#278619=CARTESIAN_POINT('Ctrl Pts',(9.83957192047906,7.51249999998044,-7.14886745759543));
#278620=CARTESIAN_POINT('Ctrl Pts',(7.51676407774784,7.66249999997983,-10.3459381770593));
#278621=CARTESIAN_POINT('Ctrl Pts',(3.75838203887391,7.81249999997923,-11.5671105274575));
#278622=CARTESIAN_POINT('Ctrl Pts',(-1.78463082620892E-14,7.96249999997863,
-12.7882828778556));
#278623=CARTESIAN_POINT('Ctrl Pts',(-3.75838203887395,8.11249999997803,
-11.5671105274575));
#278624=CARTESIAN_POINT('Ctrl Pts',(-7.51676407774788,8.26249999997743,
-10.3459381770593));
#278625=CARTESIAN_POINT('Ctrl Pts',(-9.83957192047909,8.41249999997682,
-7.14886745759543));
#278626=CARTESIAN_POINT('Ctrl Pts',(-12.1623797632103,8.56249999997622,
-3.95179673813153));
#278627=CARTESIAN_POINT('Ctrl Pts',(-12.1623797632103,8.71249999997562,
2.97892388940601E-15));
#278628=CARTESIAN_POINT('Ctrl Pts',(-12.1623797632103,8.86249999997502,
3.95179673813154));
#278629=CARTESIAN_POINT('Ctrl Pts',(-9.83957192047909,9.01249999997442,
7.14886745759543));
#278630=CARTESIAN_POINT('Ctrl Pts',(-7.51676407774787,9.16249999997382,
10.3459381770593));
#278631=CARTESIAN_POINT('Ctrl Pts',(-3.75838203887394,9.31249999997323,
11.5671105274575));
#278632=CARTESIAN_POINT('Ctrl Pts',(-1.55779369593288E-14,9.46249999997263,
12.7882828778556));
#278633=CARTESIAN_POINT('Ctrl Pts',(3.75838203887391,9.61249999997203,11.5671105274575));
#278634=CARTESIAN_POINT('Ctrl Pts',(7.51676407774784,9.76249999997144,10.3459381770593));
#278635=CARTESIAN_POINT('Ctrl Pts',(9.83957192047906,9.91249999997084,7.14886745759543));
#278636=CARTESIAN_POINT('Ctrl Pts',(12.1623797632103,10.0624999999702,3.95179673813153));
#278637=CARTESIAN_POINT('Ctrl Pts',(12.1623797632103,10.2124999999696,-1.489461944703E-15));
#278638=CARTESIAN_POINT('Ctrl Pts',(12.1623797632103,10.362499999969,-3.95179673813154));
#278639=CARTESIAN_POINT('Ctrl Pts',(9.83957192047905,10.5124999999684,-7.14886745759543));
#278640=CARTESIAN_POINT('Ctrl Pts',(7.51676407774784,10.6624999999678,-10.3459381770593));
#278641=CARTESIAN_POINT('Ctrl Pts',(3.75838203887391,10.8124999999672,-11.5671105274575));
#278642=CARTESIAN_POINT('Ctrl Pts',(-1.95740175337511E-14,10.9624999999666,
-12.7882828778556));
#278643=CARTESIAN_POINT('Ctrl Pts',(-3.75838203887395,11.112499999966,-11.5671105274575));
#278644=CARTESIAN_POINT('Ctrl Pts',(-7.51676407774788,11.2624999999654,
-10.3459381770593));
#278645=CARTESIAN_POINT('Ctrl Pts',(-9.83957192047909,11.4124999999648,
-7.14886745759543));
#278646=CARTESIAN_POINT('Ctrl Pts',(-12.1623797632103,11.5624999999642,
-3.95179673813153));
#278647=CARTESIAN_POINT('Ctrl Pts',(-12.1623797632103,11.7124999999636,
2.97892388940601E-15));
#278648=CARTESIAN_POINT('Ctrl Pts',(-12.1623797632103,11.862499999963,3.95179673813154));
#278649=CARTESIAN_POINT('Ctrl Pts',(-9.83957192047909,12.0124999999624,
7.14886745759543));
#278650=CARTESIAN_POINT('Ctrl Pts',(-7.51676407774788,12.1624999999618,
10.3459381770593));
#278651=CARTESIAN_POINT('Ctrl Pts',(-3.75838203887395,12.3124999999612,
11.5671105274575));
#278652=CARTESIAN_POINT('Ctrl Pts',(-1.73056462309906E-14,12.4624999999606,
12.7882828778556));
#278653=CARTESIAN_POINT('Ctrl Pts',(3.75838203887391,12.61249999996,11.5671105274575));
#278654=CARTESIAN_POINT('Ctrl Pts',(7.51676407774784,12.7624999999594,10.3459381770593));
#278655=CARTESIAN_POINT('Ctrl Pts',(9.83957192047906,12.9124999999588,7.14886745759543));
#278656=CARTESIAN_POINT('Ctrl Pts',(12.1623797632103,13.0624999999582,3.95179673813153));
#278657=CARTESIAN_POINT('Ctrl Pts',(12.1623797632103,13.2124999999576,-1.489461944703E-15));
#278658=CARTESIAN_POINT('Ctrl Pts',(12.1623797632103,13.362499999957,-3.95179673813154));
#278659=CARTESIAN_POINT('Ctrl Pts',(9.83957192047905,13.5124999999564,-7.14886745759543));
#278660=CARTESIAN_POINT('Ctrl Pts',(7.51676407774784,13.6624999999558,-10.3459381770593));
#278661=CARTESIAN_POINT('Ctrl Pts',(3.75838203887391,13.8124999999552,-11.5671105274575));
#278662=CARTESIAN_POINT('Ctrl Pts',(-2.13017268054129E-14,13.9624999999546,
-12.7882828778556));
#278663=CARTESIAN_POINT('Ctrl Pts',(-3.75838203887395,14.112499999954,-11.5671105274575));
#278664=CARTESIAN_POINT('Ctrl Pts',(-7.51676407774788,14.2624999999534,
-10.3459381770593));
#278665=CARTESIAN_POINT('Ctrl Pts',(-9.8395719204791,14.4124999999528,-7.14886745759543));
#278666=CARTESIAN_POINT('Ctrl Pts',(-12.1623797632103,14.5624999999522,
-3.95179673813153));
#278667=CARTESIAN_POINT('Ctrl Pts',(-12.1623797632103,14.7124999999516,
2.97892388940601E-15));
#278668=CARTESIAN_POINT('Ctrl Pts',(-12.1623797632103,14.862499999951,3.95179673813154));
#278669=CARTESIAN_POINT('Ctrl Pts',(-9.83957192047909,15.0124999999504,
7.14886745759543));
#278670=CARTESIAN_POINT('Ctrl Pts',(-7.51676407774788,15.1624999999498,
10.3459381770593));
#278671=CARTESIAN_POINT('Ctrl Pts',(-3.75838203887395,15.3124999999492,
11.5671105274575));
#278672=CARTESIAN_POINT('Ctrl Pts',(-1.90333555026525E-14,15.4624999999486,
12.7882828778556));
#278673=CARTESIAN_POINT('Ctrl Pts',(3.75838203887391,15.612499999948,11.5671105274575));
#278674=CARTESIAN_POINT('Ctrl Pts',(7.51676407774784,15.7624999999474,10.3459381770593));
#278675=CARTESIAN_POINT('Ctrl Pts',(9.83957192047905,15.9124999999468,7.14886745759543));
#278676=CARTESIAN_POINT('Ctrl Pts',(12.1623797632103,16.0624999999462,3.95179673813153));
#278677=CARTESIAN_POINT('Ctrl Pts',(12.1623797632103,16.2124999999456,-1.489461944703E-15));
#278678=CARTESIAN_POINT('Ctrl Pts',(12.1623797632103,16.362499999945,-3.95179673813154));
#278679=CARTESIAN_POINT('Ctrl Pts',(9.83957192047905,16.5124999999444,-7.14886745759543));
#278680=CARTESIAN_POINT('Ctrl Pts',(7.51676407774784,16.6624999999438,-10.3459381770593));
#278681=CARTESIAN_POINT('Ctrl Pts',(3.75838203887391,16.8124999999432,-11.5671105274575));
#278682=CARTESIAN_POINT('Ctrl Pts',(-2.30294360770748E-14,16.9624999999426,
-12.7882828778556));
#278683=CARTESIAN_POINT('Ctrl Pts',(-3.75838203887395,17.112499999942,-11.5671105274575));
#278684=CARTESIAN_POINT('Ctrl Pts',(-7.51676407774788,17.2624999999414,
-10.3459381770593));
#278685=CARTESIAN_POINT('Ctrl Pts',(-9.8395719204791,17.4124999999408,-7.14886745759543));
#278686=CARTESIAN_POINT('Ctrl Pts',(-12.1623797632103,17.5624999999402,
-3.95179673813153));
#278687=CARTESIAN_POINT('Ctrl Pts',(-12.1623797632103,17.7124999999396,
2.97892388940601E-15));
#278688=CARTESIAN_POINT('Ctrl Pts',(-12.1623797632103,17.862499999939,3.95179673813154));
#278689=CARTESIAN_POINT('Ctrl Pts',(-9.8395719204791,18.0124999999384,7.14886745759543));
#278690=CARTESIAN_POINT('Ctrl Pts',(-7.51676407774788,18.1624999999378,
10.3459381770593));
#278691=CARTESIAN_POINT('Ctrl Pts',(-3.75838203887395,18.3124999999372,
11.5671105274575));
#278692=CARTESIAN_POINT('Ctrl Pts',(-2.07610647743143E-14,18.4624999999366,
12.7882828778556));
#278693=CARTESIAN_POINT('Ctrl Pts',(3.75838203887391,18.612499999936,11.5671105274575));
#278694=CARTESIAN_POINT('Ctrl Pts',(7.51676407774784,18.7624999999354,10.3459381770593));
#278695=CARTESIAN_POINT('Ctrl Pts',(9.83957192047905,18.9124999999348,7.14886745759543));
#278696=CARTESIAN_POINT('Ctrl Pts',(12.1623797632103,19.0624999999342,3.95179673813153));
#278697=CARTESIAN_POINT('Ctrl Pts',(12.1623797632103,19.2124999999336,-1.489461944703E-15));
#278698=CARTESIAN_POINT('Ctrl Pts',(12.1623797632103,19.362499999933,-3.95179673813154));
#278699=CARTESIAN_POINT('Ctrl Pts',(9.83957192047905,19.5124999999324,-7.14886745759543));
#278700=CARTESIAN_POINT('Ctrl Pts',(7.51676407774784,19.6624999999318,-10.3459381770593));
#278701=CARTESIAN_POINT('Ctrl Pts',(3.7583820388739,19.8124999999312,-11.5671105274575));
#278702=CARTESIAN_POINT('Ctrl Pts',(-2.47571453487366E-14,19.9624999999306,
-12.7882828778556));
#278703=CARTESIAN_POINT('Ctrl Pts',(-3.75838203887395,20.11249999993,-11.5671105274575));
#278704=CARTESIAN_POINT('Ctrl Pts',(-7.51676407774788,20.2624999999294,
-10.3459381770593));
#278705=CARTESIAN_POINT('Ctrl Pts',(-9.8395719204791,20.4124999999288,-7.14886745759543));
#278706=CARTESIAN_POINT('Ctrl Pts',(-12.1623797632103,20.5624999999282,
-3.95179673813153));
#278707=CARTESIAN_POINT('Ctrl Pts',(-12.1623797632103,20.7124999999276,
2.97892388940601E-15));
#278708=CARTESIAN_POINT('Ctrl Pts',(-12.1623797632103,20.862499999927,3.95179673813154));
#278709=CARTESIAN_POINT('Ctrl Pts',(-9.8395719204791,21.0124999999264,7.14886745759543));
#278710=CARTESIAN_POINT('Ctrl Pts',(-7.51676407774788,21.1624999999258,
10.3459381770593));
#278711=CARTESIAN_POINT('Ctrl Pts',(-3.75838203887395,21.3124999999252,
11.5671105274575));
#278712=CARTESIAN_POINT('Ctrl Pts',(-2.24887740459762E-14,21.4624999999246,
12.7882828778556));
#278713=CARTESIAN_POINT('Ctrl Pts',(3.75838203887391,21.612499999924,11.5671105274575));
#278714=CARTESIAN_POINT('Ctrl Pts',(7.51676407774784,21.7624999999234,10.3459381770593));
#278715=CARTESIAN_POINT('Ctrl Pts',(9.83957192047905,21.9124999999228,7.14886745759543));
#278716=CARTESIAN_POINT('Ctrl Pts',(12.1623797632103,22.0624999999222,3.95179673813153));
#278717=CARTESIAN_POINT('Ctrl Pts',(12.1623797632103,22.2124999999216,-1.489461944703E-15));
#278718=CARTESIAN_POINT('Ctrl Pts',(12.1623797632103,22.362499999921,-3.95179673813154));
#278719=CARTESIAN_POINT('Ctrl Pts',(9.83957192047905,22.5124999999204,-7.14886745759543));
#278720=CARTESIAN_POINT('Ctrl Pts',(7.51676407774783,22.6624999999198,-10.3459381770593));
#278721=CARTESIAN_POINT('Ctrl Pts',(3.7583820388739,22.8124999999192,-11.5671105274575));
#278722=CARTESIAN_POINT('Ctrl Pts',(-2.64848546203984E-14,22.9624999999186,
-12.7882828778556));
#278723=CARTESIAN_POINT('Ctrl Pts',(-3.75838203887396,23.112499999918,-11.5671105274575));
#278724=CARTESIAN_POINT('Ctrl Pts',(-7.51676407774788,23.2624999999174,
-10.3459381770593));
#278725=CARTESIAN_POINT('Ctrl Pts',(-9.8395719204791,23.4124999999168,-7.14886745759543));
#278726=CARTESIAN_POINT('Ctrl Pts',(-12.1623797632103,23.5624999999162,
-3.95179673813153));
#278727=CARTESIAN_POINT('Ctrl Pts',(-12.1623797632103,23.7124999999156,
2.97892388940601E-15));
#278728=CARTESIAN_POINT('Ctrl Pts',(-12.1623797632103,23.862499999915,3.95179673813154));
#278729=CARTESIAN_POINT('Ctrl Pts',(-9.8395719204791,24.0124999999144,7.14886745759543));
#278730=CARTESIAN_POINT('Ctrl Pts',(-7.51676407774788,24.1624999999138,
10.3459381770593));
#278731=CARTESIAN_POINT('Ctrl Pts',(-3.75838203887395,24.3124999999132,
11.5671105274575));
#278732=CARTESIAN_POINT('Ctrl Pts',(-2.4216483317638E-14,24.4624999999126,
12.7882828778556));
#278733=CARTESIAN_POINT('Ctrl Pts',(3.7583820388739,24.612499999912,11.5671105274575));
#278734=CARTESIAN_POINT('Ctrl Pts',(7.51676407774783,24.7624999999114,10.3459381770593));
#278735=CARTESIAN_POINT('Ctrl Pts',(9.83957192047905,24.9124999999108,7.14886745759543));
#278736=CARTESIAN_POINT('Ctrl Pts',(12.1623797632103,25.0624999999102,3.95179673813153));
#278737=CARTESIAN_POINT('Ctrl Pts',(12.1623797632103,25.2124999999096,-1.489461944703E-15));
#278738=CARTESIAN_POINT('Ctrl Pts',(12.1623797632103,25.362499999909,-3.95179673813154));
#278739=CARTESIAN_POINT('Ctrl Pts',(9.83957192047905,25.5124999999084,-7.14886745759543));
#278740=CARTESIAN_POINT('Ctrl Pts',(7.51676407774783,25.6624999999078,-10.3459381770593));
#278741=CARTESIAN_POINT('Ctrl Pts',(3.7583820388739,25.8124999999072,-11.5671105274575));
#278742=CARTESIAN_POINT('Ctrl Pts',(-2.82125638920603E-14,25.9624999999066,
-12.7882828778556));
#278743=CARTESIAN_POINT('Ctrl Pts',(-3.75838203887396,26.112499999906,-11.5671105274575));
#278744=CARTESIAN_POINT('Ctrl Pts',(-7.51676407774788,26.2624999999054,
-10.3459381770593));
#278745=CARTESIAN_POINT('Ctrl Pts',(-9.8395719204791,26.4124999999048,-7.14886745759543));
#278746=CARTESIAN_POINT('Ctrl Pts',(-12.1623797632103,26.5624999999042,
-3.95179673813153));
#278747=CARTESIAN_POINT('Ctrl Pts',(-12.1623797632103,26.7124999999036,
2.97892388940601E-15));
#278748=CARTESIAN_POINT('Ctrl Pts',(-12.1623797632103,26.862499999903,3.95179673813154));
#278749=CARTESIAN_POINT('Ctrl Pts',(-9.8395719204791,27.0124999999024,7.14886745759543));
#278750=CARTESIAN_POINT('Ctrl Pts',(-7.51676407774788,27.1624999999018,
10.3459381770593));
#278751=CARTESIAN_POINT('Ctrl Pts',(-3.75838203887396,27.3124999999012,
11.5671105274575));
#278752=CARTESIAN_POINT('Ctrl Pts',(-2.59441925892998E-14,27.4624999999006,
12.7882828778556));
#278753=CARTESIAN_POINT('Ctrl Pts',(3.7583820388739,27.6124999999,11.5671105274575));
#278754=CARTESIAN_POINT('Ctrl Pts',(7.51676407774783,27.7624999998994,10.3459381770593));
#278755=CARTESIAN_POINT('Ctrl Pts',(9.83957192047905,27.9124999998988,7.14886745759543));
#278756=CARTESIAN_POINT('Ctrl Pts',(12.1623797632103,28.0624999998982,3.95179673813153));
#278757=CARTESIAN_POINT('Ctrl Pts',(12.1623797632103,28.2124999998976,-1.489461944703E-15));
#278758=CARTESIAN_POINT('Ctrl Pts',(12.1623797632103,28.362499999897,-3.95179673813154));
#278759=CARTESIAN_POINT('Ctrl Pts',(9.83957192047905,28.5124999998964,-7.14886745759543));
#278760=CARTESIAN_POINT('Ctrl Pts',(7.51676407774783,28.6624999998958,-10.3459381770593));
#278761=CARTESIAN_POINT('Ctrl Pts',(3.7583820388739,28.8124999998952,-11.5671105274575));
#278762=CARTESIAN_POINT('Ctrl Pts',(-2.99402731637221E-14,28.9624999998946,
-12.7882828778556));
#278763=CARTESIAN_POINT('Ctrl Pts',(-3.75838203887396,29.112499999894,-11.5671105274575));
#278764=CARTESIAN_POINT('Ctrl Pts',(-7.51676407774789,29.2624999998934,
-10.3459381770593));
#278765=CARTESIAN_POINT('Ctrl Pts',(-9.8395719204791,29.4124999998928,-7.14886745759543));
#278766=CARTESIAN_POINT('Ctrl Pts',(-12.1623797632103,29.5624999998922,
-3.95179673813153));
#278767=CARTESIAN_POINT('Ctrl Pts',(-12.1623797632103,29.7124999998916,
2.97892388940601E-15));
#278768=CARTESIAN_POINT('Ctrl Pts',(-12.1623797632103,29.862499999891,3.95179673813154));
#278769=CARTESIAN_POINT('Ctrl Pts',(-9.8395719204791,30.0124999998904,7.14886745759543));
#278770=CARTESIAN_POINT('Ctrl Pts',(-7.51676407774788,30.1624999998898,
10.3459381770593));
#278771=CARTESIAN_POINT('Ctrl Pts',(-3.75838203887396,30.3124999998892,
11.5671105274575));
#278772=CARTESIAN_POINT('Ctrl Pts',(-2.76719018609617E-14,30.4624999998886,
12.7882828778556));
#278773=CARTESIAN_POINT('Ctrl Pts',(3.7583820388739,30.612499999888,11.5671105274575));
#278774=CARTESIAN_POINT('Ctrl Pts',(7.51676407774783,30.7624999998874,10.3459381770593));
#278775=CARTESIAN_POINT('Ctrl Pts',(9.83957192047905,30.9124999998868,7.14886745759543));
#278776=CARTESIAN_POINT('Ctrl Pts',(12.1623797632103,31.0624999998862,3.95179673813153));
#278777=CARTESIAN_POINT('Ctrl Pts',(12.1623797632103,31.2124999998856,-1.489461944703E-15));
#278778=CARTESIAN_POINT('Ctrl Pts',(12.1623797632103,31.362499999885,-3.95179673813154));
#278779=CARTESIAN_POINT('Ctrl Pts',(9.83957192047904,31.5124999998844,-7.14886745759543));
#278780=CARTESIAN_POINT('Ctrl Pts',(7.51676407774783,31.6624999998838,-10.3459381770593));
#278781=CARTESIAN_POINT('Ctrl Pts',(3.7583820388739,31.8124999998832,-11.5671105274575));
#278782=CARTESIAN_POINT('Ctrl Pts',(-3.16679824353839E-14,31.9624999998826,
-12.7882828778556));
#278783=CARTESIAN_POINT('Ctrl Pts',(-3.75838203887396,32.112499999882,-11.5671105274575));
#278784=CARTESIAN_POINT('Ctrl Pts',(-7.51676407774789,32.2624999998814,
-10.3459381770593));
#278785=CARTESIAN_POINT('Ctrl Pts',(-9.83957192047911,32.4124999998808,
-7.14886745759543));
#278786=CARTESIAN_POINT('Ctrl Pts',(-12.1623797632103,32.5624999998802,
-3.95179673813153));
#278787=CARTESIAN_POINT('Ctrl Pts',(-12.1623797632103,32.7124999998796,
2.97892388940601E-15));
#278788=CARTESIAN_POINT('Ctrl Pts',(-12.1623797632103,32.862499999879,3.95179673813154));
#278789=CARTESIAN_POINT('Ctrl Pts',(-9.8395719204791,33.0124999998784,7.14886745759543));
#278790=CARTESIAN_POINT('Ctrl Pts',(-7.51676407774789,33.1624999998778,
10.3459381770593));
#278791=CARTESIAN_POINT('Ctrl Pts',(-3.75838203887396,33.3124999998772,
11.5671105274575));
#278792=CARTESIAN_POINT('Ctrl Pts',(-2.93996111326235E-14,33.4624999998766,
12.7882828778556));
#278793=CARTESIAN_POINT('Ctrl Pts',(3.7583820388739,33.612499999876,11.5671105274575));
#278794=CARTESIAN_POINT('Ctrl Pts',(7.51676407774783,33.7624999998754,10.3459381770593));
#278795=CARTESIAN_POINT('Ctrl Pts',(9.83957192047905,33.9124999998748,7.14886745759543));
#278796=CARTESIAN_POINT('Ctrl Pts',(12.1623797632103,34.0624999998742,3.95179673813153));
#278797=CARTESIAN_POINT('Ctrl Pts',(12.1623797632103,34.2124999998736,-1.489461944703E-15));
#278798=CARTESIAN_POINT('Ctrl Pts',(12.1623797632103,34.362499999873,-3.95179673813154));
#278799=CARTESIAN_POINT('Ctrl Pts',(9.83957192047904,34.5124999998724,-7.14886745759543));
#278800=CARTESIAN_POINT('Ctrl Pts',(7.51676407774783,34.6624999998718,-10.3459381770593));
#278801=CARTESIAN_POINT('Ctrl Pts',(3.7583820388739,34.8124999998712,-11.5671105274575));
#278802=CARTESIAN_POINT('Ctrl Pts',(-3.33956917070458E-14,34.9624999998706,
-12.7882828778556));
#278803=CARTESIAN_POINT('Ctrl Pts',(-3.75838203887396,35.11249999987,-11.5671105274575));
#278804=CARTESIAN_POINT('Ctrl Pts',(-7.51676407774789,35.2624999998694,
-10.3459381770593));
#278805=CARTESIAN_POINT('Ctrl Pts',(-9.83957192047911,35.4124999998688,
-7.14886745759543));
#278806=CARTESIAN_POINT('Ctrl Pts',(-12.1623797632103,35.5624999998682,
-3.95179673813153));
#278807=CARTESIAN_POINT('Ctrl Pts',(-12.1623797632103,35.7124999998676,
2.97892388940601E-15));
#278808=CARTESIAN_POINT('Ctrl Pts',(-12.1623797632103,35.862499999867,3.95179673813154));
#278809=CARTESIAN_POINT('Ctrl Pts',(-9.83957192047911,36.0124999998664,
7.14886745759543));
#278810=CARTESIAN_POINT('Ctrl Pts',(-7.51676407774789,36.1624999998658,
10.3459381770593));
#278811=CARTESIAN_POINT('Ctrl Pts',(-3.75838203887396,36.3124999998652,
11.5671105274575));
#278812=CARTESIAN_POINT('Ctrl Pts',(-3.11273204042854E-14,36.4624999998646,
12.7882828778556));
#278813=CARTESIAN_POINT('Ctrl Pts',(3.7583820388739,36.612499999864,11.5671105274575));
#278814=CARTESIAN_POINT('Ctrl Pts',(7.51676407774783,36.7624999998634,10.3459381770593));
#278815=CARTESIAN_POINT('Ctrl Pts',(9.83957192047904,36.9124999998628,7.14886745759543));
#278816=CARTESIAN_POINT('Ctrl Pts',(12.1623797632103,37.0624999998622,3.95179673813153));
#278817=CARTESIAN_POINT('Ctrl Pts',(12.1623797632103,37.2124999998616,-1.489461944703E-15));
#278818=CARTESIAN_POINT('Ctrl Pts',(12.1623797632103,37.362499999861,-3.95179673813154));
#278819=CARTESIAN_POINT('Ctrl Pts',(9.83957192047904,37.5124999998604,-7.14886745759543));
#278820=CARTESIAN_POINT('Ctrl Pts',(7.51676407774782,37.6624999998598,-10.3459381770593));
#278821=CARTESIAN_POINT('Ctrl Pts',(3.75838203887389,37.8124999998592,-11.5671105274575));
#278822=CARTESIAN_POINT('Ctrl Pts',(-3.51234009787076E-14,37.9624999998586,
-12.7882828778556));
#278823=CARTESIAN_POINT('Ctrl Pts',(-3.75838203887396,38.112499999858,-11.5671105274575));
#278824=CARTESIAN_POINT('Ctrl Pts',(-7.51676407774789,38.2624999998574,
-10.3459381770593));
#278825=CARTESIAN_POINT('Ctrl Pts',(-9.83957192047911,38.4124999998568,
-7.14886745759543));
#278826=CARTESIAN_POINT('Ctrl Pts',(-12.1623797632103,38.5624999998562,
-3.95179673813153));
#278827=CARTESIAN_POINT('Ctrl Pts',(-12.1623797632103,38.7124999998556,
2.97892388940601E-15));
#278828=CARTESIAN_POINT('Ctrl Pts',(-12.1623797632103,38.862499999855,3.95179673813154));
#278829=CARTESIAN_POINT('Ctrl Pts',(-9.83957192047911,39.0124999998544,
7.14886745759543));
#278830=CARTESIAN_POINT('Ctrl Pts',(-7.51676407774789,39.1624999998538,
10.3459381770593));
#278831=CARTESIAN_POINT('Ctrl Pts',(-3.75838203887396,39.3124999998532,
11.5671105274575));
#278832=CARTESIAN_POINT('Ctrl Pts',(-3.28550296759472E-14,39.4624999998526,
12.7882828778556));
#278833=CARTESIAN_POINT('Ctrl Pts',(3.7583820388739,39.612499999852,11.5671105274575));
#278834=CARTESIAN_POINT('Ctrl Pts',(7.51676407774782,39.7624999998514,10.3459381770593));
#278835=CARTESIAN_POINT('Ctrl Pts',(9.83957192047904,39.9124999998508,7.14886745759543));
#278836=CARTESIAN_POINT('Ctrl Pts',(12.1623797632103,40.0624999998502,3.95179673813153));
#278837=CARTESIAN_POINT('Ctrl Pts',(12.1623797632103,40.2124999998496,-1.489461944703E-15));
#278838=CARTESIAN_POINT('Ctrl Pts',(12.1623797632103,40.362499999849,-3.95179673813154));
#278839=CARTESIAN_POINT('Ctrl Pts',(9.83957192047904,40.5124999998484,-7.14886745759543));
#278840=CARTESIAN_POINT('Ctrl Pts',(7.51676407774782,40.6624999998478,-10.3459381770593));
#278841=CARTESIAN_POINT('Ctrl Pts',(3.75838203887389,40.8124999998472,-11.5671105274575));
#278842=CARTESIAN_POINT('Ctrl Pts',(-3.68511102503695E-14,40.9624999998466,
-12.7882828778556));
#278843=CARTESIAN_POINT('Ctrl Pts',(-3.75838203887397,41.112499999846,-11.5671105274575));
#278844=CARTESIAN_POINT('Ctrl Pts',(-7.51676407774789,41.2624999998454,
-10.3459381770593));
#278845=CARTESIAN_POINT('Ctrl Pts',(-9.83957192047911,41.4124999998448,
-7.14886745759543));
#278846=CARTESIAN_POINT('Ctrl Pts',(-12.1623797632103,41.5624999998442,
-3.95179673813153));
#278847=CARTESIAN_POINT('Ctrl Pts',(-12.1623797632103,41.7124999998436,
2.97892388940601E-15));
#278848=CARTESIAN_POINT('Ctrl Pts',(-12.1623797632103,41.862499999843,3.95179673813154));
#278849=CARTESIAN_POINT('Ctrl Pts',(-9.83957192047911,42.0124999998424,
7.14886745759543));
#278850=CARTESIAN_POINT('Ctrl Pts',(-7.51676407774789,42.1624999998418,
10.3459381770593));
#278851=CARTESIAN_POINT('Ctrl Pts',(-3.75838203887396,42.3124999998412,
11.5671105274575));
#278852=CARTESIAN_POINT('Ctrl Pts',(-3.4582738947609E-14,42.4624999998406,
12.7882828778556));
#278853=CARTESIAN_POINT('Ctrl Pts',(3.75838203887389,42.61249999984,11.5671105274575));
#278854=CARTESIAN_POINT('Ctrl Pts',(7.51676407774782,42.7624999998394,10.3459381770593));
#278855=CARTESIAN_POINT('Ctrl Pts',(9.83957192047904,42.9124999998388,7.14886745759543));
#278856=CARTESIAN_POINT('Ctrl Pts',(12.1623797632103,43.0624999998382,3.95179673813153));
#278857=CARTESIAN_POINT('Ctrl Pts',(12.1623797632103,43.2124999998376,-1.489461944703E-15));
#278858=CARTESIAN_POINT('Ctrl Pts',(12.1623797632103,43.362499999837,-3.95179673813154));
#278859=CARTESIAN_POINT('Ctrl Pts',(9.83957192047903,43.5124999998364,-7.14886745759543));
#278860=CARTESIAN_POINT('Ctrl Pts',(7.51676407774782,43.6624999998358,-10.3459381770593));
#278861=CARTESIAN_POINT('Ctrl Pts',(3.75838203887389,43.8124999998352,-11.5671105274575));
#278862=CARTESIAN_POINT('Ctrl Pts',(-3.85788195220313E-14,43.9624999998346,
-12.7882828778556));
#278863=CARTESIAN_POINT('Ctrl Pts',(-3.75838203887397,44.112499999834,-11.5671105274575));
#278864=CARTESIAN_POINT('Ctrl Pts',(-7.5167640777479,44.2624999998334,-10.3459381770593));
#278865=CARTESIAN_POINT('Ctrl Pts',(-9.83957192047911,44.4124999998328,
-7.14886745759543));
#278866=CARTESIAN_POINT('Ctrl Pts',(-12.1623797632103,44.5624999998322,
-3.95179673813153));
#278867=CARTESIAN_POINT('Ctrl Pts',(-12.1623797632103,44.7124999998316,
2.97892388940601E-15));
#278868=CARTESIAN_POINT('Ctrl Pts',(-12.1623797632103,44.862499999831,3.95179673813154));
#278869=CARTESIAN_POINT('Ctrl Pts',(-9.83957192047911,45.0124999998304,
7.14886745759543));
#278870=CARTESIAN_POINT('Ctrl Pts',(-7.51676407774789,45.1624999998298,
10.3459381770593));
#278871=CARTESIAN_POINT('Ctrl Pts',(-3.75838203887397,45.3124999998292,
11.5671105274575));
#278872=CARTESIAN_POINT('Ctrl Pts',(-3.63104482192709E-14,45.4624999998286,
12.7882828778556));
#278873=CARTESIAN_POINT('Ctrl Pts',(3.75838203887389,45.612499999828,11.5671105274575));
#278874=CARTESIAN_POINT('Ctrl Pts',(7.51676407774782,45.7624999998274,10.3459381770593));
#278875=CARTESIAN_POINT('Ctrl Pts',(9.83957192047904,45.9124999998268,7.14886745759543));
#278876=CARTESIAN_POINT('Ctrl Pts',(12.1623797632103,46.0624999998262,3.95179673813153));
#278877=CARTESIAN_POINT('Ctrl Pts',(12.1623797632103,46.2124999998256,-1.489461944703E-15));
#278878=CARTESIAN_POINT('Ctrl Pts',(12.1623797632103,46.362499999825,-3.95179673813154));
#278879=CARTESIAN_POINT('Ctrl Pts',(9.83957192047903,46.5124999998244,-7.14886745759543));
#278880=CARTESIAN_POINT('Ctrl Pts',(7.51676407774782,46.6624999998238,-10.3459381770593));
#278881=CARTESIAN_POINT('Ctrl Pts',(3.75838203887389,46.8124999998232,-11.5671105274575));
#278882=CARTESIAN_POINT('Ctrl Pts',(-4.03065287936931E-14,46.9624999998226,
-12.7882828778556));
#278883=CARTESIAN_POINT('Ctrl Pts',(-3.75838203887397,47.112499999822,-11.5671105274575));
#278884=CARTESIAN_POINT('Ctrl Pts',(-7.5167640777479,47.2624999998214,-10.3459381770593));
#278885=CARTESIAN_POINT('Ctrl Pts',(-9.83957192047912,47.4124999998208,
-7.14886745759543));
#278886=CARTESIAN_POINT('Ctrl Pts',(-12.1623797632103,47.5624999998202,
-3.95179673813153));
#278887=CARTESIAN_POINT('Ctrl Pts',(-12.1623797632103,47.7124999998196,
2.97892388940601E-15));
#278888=CARTESIAN_POINT('Ctrl Pts',(-12.1623797632103,47.862499999819,3.95179673813154));
#278889=CARTESIAN_POINT('Ctrl Pts',(-9.83957192047911,48.0124999998184,
7.14886745759543));
#278890=CARTESIAN_POINT('Ctrl Pts',(-7.51676407774789,48.1624999998178,
10.3459381770593));
#278891=CARTESIAN_POINT('Ctrl Pts',(-3.75838203887397,48.3124999998172,
11.5671105274575));
#278892=CARTESIAN_POINT('Ctrl Pts',(-3.80381574909327E-14,48.4624999998166,
12.7882828778556));
#278893=CARTESIAN_POINT('Ctrl Pts',(3.75838203887389,48.612499999816,11.5671105274575));
#278894=CARTESIAN_POINT('Ctrl Pts',(7.51676407774782,48.7624999998154,10.3459381770593));
#278895=CARTESIAN_POINT('Ctrl Pts',(9.83957192047903,48.9124999998148,7.14886745759543));
#278896=CARTESIAN_POINT('Ctrl Pts',(12.1623797632103,49.0624999998142,3.95179673813153));
#278897=CARTESIAN_POINT('Ctrl Pts',(12.1623797632103,49.2124999998136,-1.489461944703E-15));
#278898=CARTESIAN_POINT('Ctrl Pts',(12.1623797632103,49.362499999813,-3.95179673813154));
#278899=CARTESIAN_POINT('Ctrl Pts',(9.83957192047903,49.5124999998124,-7.14886745759543));
#278900=CARTESIAN_POINT('Ctrl Pts',(7.51676407774782,49.6624999998118,-10.3459381770593));
#278901=CARTESIAN_POINT('Ctrl Pts',(3.75838203887389,49.8124999998112,-11.5671105274575));
#278902=CARTESIAN_POINT('Ctrl Pts',(-4.2034238065355E-14,49.9624999998106,
-12.7882828778556));
#278903=CARTESIAN_POINT('Ctrl Pts',(-3.75838203887397,50.11249999981,-11.5671105274575));
#278904=CARTESIAN_POINT('Ctrl Pts',(-7.5167640777479,50.2624999998094,-10.3459381770593));
#278905=CARTESIAN_POINT('Ctrl Pts',(-9.83957192047912,50.4124999998088,
-7.14886745759543));
#278906=CARTESIAN_POINT('Ctrl Pts',(-12.1623797632103,50.5624999998082,
-3.95179673813153));
#278907=CARTESIAN_POINT('Ctrl Pts',(-12.1623797632103,50.7124999998076,
2.97892388940601E-15));
#278908=CARTESIAN_POINT('Ctrl Pts',(-12.1623797632103,50.862499999807,3.95179673813154));
#278909=CARTESIAN_POINT('Ctrl Pts',(-9.83957192047912,51.0124999998064,
7.14886745759543));
#278910=CARTESIAN_POINT('Ctrl Pts',(-7.5167640777479,51.1624999998058,10.3459381770593));
#278911=CARTESIAN_POINT('Ctrl Pts',(-3.75838203887397,51.3124999998052,
11.5671105274575));
#278912=CARTESIAN_POINT('Ctrl Pts',(-3.97658667625946E-14,51.4624999998046,
12.7882828778556));
#278913=CARTESIAN_POINT('Ctrl Pts',(3.75838203887389,51.612499999804,11.5671105274575));
#278914=CARTESIAN_POINT('Ctrl Pts',(7.51676407774782,51.7624999998034,10.3459381770593));
#278915=CARTESIAN_POINT('Ctrl Pts',(9.83957192047903,51.9124999998028,7.14886745759543));
#278916=CARTESIAN_POINT('Ctrl Pts',(12.1623797632103,52.0624999998022,3.95179673813153));
#278917=CARTESIAN_POINT('Ctrl Pts',(12.1623797632103,52.2124999998016,-1.489461944703E-15));
#278918=CARTESIAN_POINT('Ctrl Pts',(12.1623797632103,52.362499999801,-3.95179673813154));
#278919=CARTESIAN_POINT('Ctrl Pts',(9.83957192047903,52.5124999998004,-7.14886745759543));
#278920=CARTESIAN_POINT('Ctrl Pts',(7.51676407774781,52.6624999997998,-10.3459381770593));
#278921=CARTESIAN_POINT('Ctrl Pts',(3.75838203887388,52.8124999997992,-11.5671105274575));
#278922=CARTESIAN_POINT('Ctrl Pts',(-4.37619473370168E-14,52.9624999997986,
-12.7882828778556));
#278923=CARTESIAN_POINT('Ctrl Pts',(-3.75838203887397,53.112499999798,-11.5671105274575));
#278924=CARTESIAN_POINT('Ctrl Pts',(-7.5167640777479,53.2624999997974,-10.3459381770593));
#278925=CARTESIAN_POINT('Ctrl Pts',(-9.83957192047912,53.4124999997968,
-7.14886745759543));
#278926=CARTESIAN_POINT('Ctrl Pts',(-12.1623797632103,53.5624999997962,
-3.95179673813153));
#278927=CARTESIAN_POINT('Ctrl Pts',(-12.1623797632103,53.7124999997956,
2.97892388940601E-15));
#278928=CARTESIAN_POINT('Ctrl Pts',(-12.1623797632103,53.862499999795,3.95179673813154));
#278929=CARTESIAN_POINT('Ctrl Pts',(-9.83957192047912,54.0124999997944,
7.14886745759543));
#278930=CARTESIAN_POINT('Ctrl Pts',(-7.5167640777479,54.1624999997938,10.3459381770593));
#278931=CARTESIAN_POINT('Ctrl Pts',(-3.75838203887397,54.3124999997932,
11.5671105274575));
#278932=CARTESIAN_POINT('Ctrl Pts',(-4.14935760342564E-14,54.4624999997926,
12.7882828778556));
#278933=CARTESIAN_POINT('Ctrl Pts',(3.75838203887389,54.612499999792,11.5671105274575));
#278934=CARTESIAN_POINT('Ctrl Pts',(7.51676407774782,54.7624999997914,10.3459381770593));
#278935=CARTESIAN_POINT('Ctrl Pts',(9.83957192047903,54.9124999997908,7.14886745759543));
#278936=CARTESIAN_POINT('Ctrl Pts',(12.1623797632103,55.0624999997902,3.95179673813153));
#278937=CARTESIAN_POINT('Ctrl Pts',(12.1623797632103,55.2124999997896,-1.489461944703E-15));
#278938=CARTESIAN_POINT('Ctrl Pts',(12.1623797632103,55.362499999789,-3.95179673813154));
#278939=CARTESIAN_POINT('Ctrl Pts',(9.83957192047903,55.5124999997884,-7.14886745759543));
#278940=CARTESIAN_POINT('Ctrl Pts',(7.51676407774781,55.6624999997878,-10.3459381770593));
#278941=CARTESIAN_POINT('Ctrl Pts',(3.75838203887388,55.8124999997872,-11.5671105274575));
#278942=CARTESIAN_POINT('Ctrl Pts',(-4.54896566086787E-14,55.9624999997866,
-12.7882828778556));
#278943=CARTESIAN_POINT('Ctrl Pts',(-3.75838203887397,56.112499999786,-11.5671105274575));
#278944=CARTESIAN_POINT('Ctrl Pts',(-7.5167640777479,56.2624999997854,-10.3459381770593));
#278945=CARTESIAN_POINT('Ctrl Pts',(-9.83957192047912,56.4124999997848,
-7.14886745759543));
#278946=CARTESIAN_POINT('Ctrl Pts',(-12.1623797632103,56.5624999997842,
-3.95179673813153));
#278947=CARTESIAN_POINT('Ctrl Pts',(-12.1623797632103,56.7124999997836,
2.97892388940601E-15));
#278948=CARTESIAN_POINT('Ctrl Pts',(-12.1623797632103,56.862499999783,3.95179673813154));
#278949=CARTESIAN_POINT('Ctrl Pts',(-9.83957192047912,57.0124999997824,
7.14886745759543));
#278950=CARTESIAN_POINT('Ctrl Pts',(-7.5167640777479,57.1624999997818,10.3459381770593));
#278951=CARTESIAN_POINT('Ctrl Pts',(-3.75838203887397,57.3124999997812,
11.5671105274575));
#278952=CARTESIAN_POINT('Ctrl Pts',(-4.32212853059182E-14,57.4624999997806,
12.7882828778556));
#278953=CARTESIAN_POINT('Ctrl Pts',(3.75838203887389,57.61249999978,11.5671105274575));
#278954=CARTESIAN_POINT('Ctrl Pts',(7.51676407774781,57.7624999997794,10.3459381770593));
#278955=CARTESIAN_POINT('Ctrl Pts',(9.83957192047903,57.9124999997788,7.14886745759543));
#278956=CARTESIAN_POINT('Ctrl Pts',(12.1623797632103,58.0624999997782,3.95179673813153));
#278957=CARTESIAN_POINT('Ctrl Pts',(12.1623797632102,58.2124999997776,-1.489461944703E-15));
#278958=CARTESIAN_POINT('Ctrl Pts',(12.1623797632102,58.362499999777,-3.95179673813154));
#278959=CARTESIAN_POINT('Ctrl Pts',(9.83957192047903,58.5124999997764,-7.14886745759543));
#278960=CARTESIAN_POINT('Ctrl Pts',(7.51676407774781,58.6624999997758,-10.3459381770593));
#278961=CARTESIAN_POINT('Ctrl Pts',(3.75838203887388,58.8124999997752,-11.5671105274575));
#278962=CARTESIAN_POINT('Ctrl Pts',(-4.72173658803405E-14,58.9624999997746,
-12.7882828778556));
#278963=CARTESIAN_POINT('Ctrl Pts',(-3.75838203887398,59.112499999774,-11.5671105274575));
#278964=CARTESIAN_POINT('Ctrl Pts',(-7.51676407774791,59.2624999997734,
-10.3459381770593));
#278965=CARTESIAN_POINT('Ctrl Pts',(-9.83957192047912,59.4124999997728,
-7.14886745759543));
#278966=CARTESIAN_POINT('Ctrl Pts',(-12.1623797632103,59.5624999997722,
-3.95179673813153));
#278967=CARTESIAN_POINT('Ctrl Pts',(-12.1623797632103,59.7124999997716,
2.97892388940601E-15));
#278968=CARTESIAN_POINT('Ctrl Pts',(-12.1623797632103,59.862499999771,3.95179673813154));
#278969=CARTESIAN_POINT('Ctrl Pts',(-9.83957192047912,60.0124999997704,
7.14886745759543));
#278970=CARTESIAN_POINT('Ctrl Pts',(-7.5167640777479,60.1624999997698,10.3459381770593));
#278971=CARTESIAN_POINT('Ctrl Pts',(-3.75838203887397,60.3124999997692,
11.5671105274575));
#278972=CARTESIAN_POINT('Ctrl Pts',(-4.49489945775801E-14,60.4624999997686,
12.7882828778556));
#278973=CARTESIAN_POINT('Ctrl Pts',(3.75838203887388,60.612499999768,11.5671105274575));
#278974=CARTESIAN_POINT('Ctrl Pts',(7.51676407774781,60.7624999997674,10.3459381770593));
#278975=CARTESIAN_POINT('Ctrl Pts',(9.83957192047903,60.9124999997668,7.14886745759543));
#278976=CARTESIAN_POINT('Ctrl Pts',(12.1623797632103,61.0624999997662,3.95179673813153));
#278977=CARTESIAN_POINT('Ctrl Pts',(12.1623797632102,61.2124999997656,-1.489461944703E-15));
#278978=CARTESIAN_POINT('Ctrl Pts',(12.1623797632102,61.362499999765,-3.95179673813154));
#278979=CARTESIAN_POINT('Ctrl Pts',(9.83957192047902,61.5124999997644,-7.14886745759543));
#278980=CARTESIAN_POINT('Ctrl Pts',(7.51676407774781,61.6624999997638,-10.3459381770593));
#278981=CARTESIAN_POINT('Ctrl Pts',(3.75838203887388,61.8124999997632,-11.5671105274575));
#278982=CARTESIAN_POINT('Ctrl Pts',(-4.89450751520023E-14,61.9624999997626,
-12.7882828778556));
#278983=CARTESIAN_POINT('Ctrl Pts',(-3.75838203887398,62.112499999762,-11.5671105274575));
#278984=CARTESIAN_POINT('Ctrl Pts',(-7.51676407774791,62.2624999997614,
-10.3459381770593));
#278985=CARTESIAN_POINT('Ctrl Pts',(-9.83957192047912,62.4124999997608,
-7.14886745759543));
#278986=CARTESIAN_POINT('Ctrl Pts',(-12.1623797632103,62.5624999997602,
-3.95179673813153));
#278987=CARTESIAN_POINT('Ctrl Pts',(-12.1623797632103,62.7124999997596,
2.97892388940601E-15));
#278988=CARTESIAN_POINT('Ctrl Pts',(-12.1623797632103,62.862499999759,3.95179673813154));
#278989=CARTESIAN_POINT('Ctrl Pts',(-9.83957192047912,63.0124999997584,
7.14886745759543));
#278990=CARTESIAN_POINT('Ctrl Pts',(-7.5167640777479,63.1624999997578,10.3459381770593));
#278991=CARTESIAN_POINT('Ctrl Pts',(-3.75838203887398,63.3124999997572,
11.5671105274575));
#278992=CARTESIAN_POINT('Ctrl Pts',(-4.66767038492419E-14,63.4624999997566,
12.7882828778556));
#278993=CARTESIAN_POINT('Ctrl Pts',(3.75838203887388,63.612499999756,11.5671105274575));
#278994=CARTESIAN_POINT('Ctrl Pts',(7.51676407774781,63.7624999997554,10.3459381770593));
#278995=CARTESIAN_POINT('Ctrl Pts',(9.83957192047903,63.9124999997548,7.14886745759543));
#278996=CARTESIAN_POINT('Ctrl Pts',(12.1623797632102,64.0624999997542,3.95179673813153));
#278997=CARTESIAN_POINT('Ctrl Pts',(12.1623797632102,64.2124999997536,-1.489461944703E-15));
#278998=CARTESIAN_POINT('Ctrl Pts',(12.1623797632102,64.362499999753,-3.95179673813154));
#278999=CARTESIAN_POINT('Ctrl Pts',(9.83957192047902,64.5124999997524,-7.14886745759543));
#279000=CARTESIAN_POINT('Ctrl Pts',(7.51676407774781,64.6624999997518,-10.3459381770593));
#279001=CARTESIAN_POINT('Ctrl Pts',(3.75838203887388,64.8124999997512,-11.5671105274575));
#279002=CARTESIAN_POINT('Ctrl Pts',(-5.06727844236642E-14,64.9624999997506,
-12.7882828778556));
#279003=CARTESIAN_POINT('Ctrl Pts',(-3.75838203887398,65.11249999975,-11.5671105274575));
#279004=CARTESIAN_POINT('Ctrl Pts',(-7.51676407774791,65.2624999997494,
-10.3459381770593));
#279005=CARTESIAN_POINT('Ctrl Pts',(-9.83957192047913,65.4124999997488,
-7.14886745759543));
#279006=CARTESIAN_POINT('Ctrl Pts',(-12.1623797632103,65.5624999997482,
-3.95179673813153));
#279007=CARTESIAN_POINT('Ctrl Pts',(-12.1623797632103,65.7124999997476,
2.97892388940601E-15));
#279008=CARTESIAN_POINT('Ctrl Pts',(-12.1623797632103,65.862499999747,3.95179673813154));
#279009=CARTESIAN_POINT('Ctrl Pts',(-9.83957192047912,66.0124999997464,
7.14886745759543));
#279010=CARTESIAN_POINT('Ctrl Pts',(-7.51676407774791,66.1624999997458,
10.3459381770593));
#279011=CARTESIAN_POINT('Ctrl Pts',(-3.75838203887398,66.3124999997452,
11.5671105274575));
#279012=CARTESIAN_POINT('Ctrl Pts',(-4.84044131209037E-14,66.4624999997446,
12.7882828778556));
#279013=CARTESIAN_POINT('Ctrl Pts',(3.75838203887388,66.612499999744,11.5671105274575));
#279014=CARTESIAN_POINT('Ctrl Pts',(7.51676407774781,66.7624999997434,10.3459381770593));
#279015=CARTESIAN_POINT('Ctrl Pts',(9.83957192047902,66.9124999997428,7.14886745759543));
#279016=CARTESIAN_POINT('Ctrl Pts',(12.1623797632102,67.0624999997422,3.95179673813153));
#279017=CARTESIAN_POINT('Ctrl Pts',(12.1623797632102,67.2124999997416,-1.489461944703E-15));
#279018=CARTESIAN_POINT('Ctrl Pts',(12.1623797632102,67.362499999741,-3.95179673813154));
#279019=CARTESIAN_POINT('Ctrl Pts',(9.83957192047902,67.5124999997404,-7.14886745759543));
#279020=CARTESIAN_POINT('Ctrl Pts',(7.51676407774781,67.6624999997398,-10.3459381770593));
#279021=CARTESIAN_POINT('Ctrl Pts',(3.75838203887388,67.8124999997392,-11.5671105274575));
#279022=CARTESIAN_POINT('Ctrl Pts',(-5.2400493695326E-14,67.9624999997386,
-12.7882828778556));
#279023=CARTESIAN_POINT('Ctrl Pts',(-3.75838203887398,68.112499999738,-11.5671105274575));
#279024=CARTESIAN_POINT('Ctrl Pts',(-7.51676407774791,68.2624999997374,
-10.3459381770593));
#279025=CARTESIAN_POINT('Ctrl Pts',(-9.83957192047913,68.4124999997368,
-7.14886745759543));
#279026=CARTESIAN_POINT('Ctrl Pts',(-12.1623797632103,68.5624999997362,
-3.95179673813153));
#279027=CARTESIAN_POINT('Ctrl Pts',(-12.1623797632103,68.7124999997356,
2.97892388940601E-15));
#279028=CARTESIAN_POINT('Ctrl Pts',(-12.1623797632103,68.862499999735,3.95179673813154));
#279029=CARTESIAN_POINT('Ctrl Pts',(-9.83957192047913,69.0124999997344,
7.14886745759543));
#279030=CARTESIAN_POINT('Ctrl Pts',(-7.51676407774791,69.1624999997338,
10.3459381770593));
#279031=CARTESIAN_POINT('Ctrl Pts',(-3.75838203887398,69.3124999997332,
11.5671105274575));
#279032=CARTESIAN_POINT('Ctrl Pts',(-5.01321223925656E-14,69.4624999997326,
12.7882828778556));
#279033=CARTESIAN_POINT('Ctrl Pts',(3.75838203887388,69.612499999732,11.5671105274575));
#279034=CARTESIAN_POINT('Ctrl Pts',(7.51676407774781,69.7624999997314,10.3459381770593));
#279035=CARTESIAN_POINT('Ctrl Pts',(9.83957192047902,69.9124999997308,7.14886745759543));
#279036=CARTESIAN_POINT('Ctrl Pts',(12.1623797632102,70.0624999997302,3.95179673813153));
#279037=CARTESIAN_POINT('Ctrl Pts',(12.1623797632102,70.2124999997296,-1.489461944703E-15));
#279038=CARTESIAN_POINT('Ctrl Pts',(12.1623797632102,70.362499999729,-3.95179673813154));
#279039=CARTESIAN_POINT('Ctrl Pts',(9.83957192047902,70.5124999997284,-7.14886745759543));
#279040=CARTESIAN_POINT('Ctrl Pts',(7.5167640777478,70.6624999997278,-10.3459381770593));
#279041=CARTESIAN_POINT('Ctrl Pts',(3.75838203887388,70.8124999997272,-11.5671105274575));
#279042=CARTESIAN_POINT('Ctrl Pts',(-5.41282029669879E-14,70.9624999997266,
-12.7882828778556));
#279043=CARTESIAN_POINT('Ctrl Pts',(-3.75838203887398,71.112499999726,-11.5671105274575));
#279044=CARTESIAN_POINT('Ctrl Pts',(-7.51676407774791,71.2624999997254,
-10.3459381770593));
#279045=CARTESIAN_POINT('Ctrl Pts',(-9.83957192047913,71.4124999997248,
-7.14886745759543));
#279046=CARTESIAN_POINT('Ctrl Pts',(-12.1623797632103,71.5624999997242,
-3.95179673813153));
#279047=CARTESIAN_POINT('Ctrl Pts',(-12.1623797632103,71.7124999997236,
2.97892388940601E-15));
#279048=CARTESIAN_POINT('Ctrl Pts',(-12.1623797632103,71.862499999723,3.95179673813154));
#279049=CARTESIAN_POINT('Ctrl Pts',(-9.83957192047913,72.0124999997224,
7.14886745759543));
#279050=CARTESIAN_POINT('Ctrl Pts',(-7.51676407774791,72.1624999997218,
10.3459381770593));
#279051=CARTESIAN_POINT('Ctrl Pts',(-3.75838203887398,72.3124999997212,
11.5671105274575));
#279052=CARTESIAN_POINT('Ctrl Pts',(-5.18598316642274E-14,72.4624999997206,
12.7882828778556));
#279053=CARTESIAN_POINT('Ctrl Pts',(3.75838203887388,72.61249999972,11.5671105274575));
#279054=CARTESIAN_POINT('Ctrl Pts',(7.51676407774781,72.7624999997194,10.3459381770593));
#279055=CARTESIAN_POINT('Ctrl Pts',(9.83957192047902,72.9124999997188,7.14886745759543));
#279056=CARTESIAN_POINT('Ctrl Pts',(12.1623797632102,73.0624999997182,3.95179673813153));
#279057=CARTESIAN_POINT('Ctrl Pts',(12.1623797632102,73.2124999997176,-1.489461944703E-15));
#279058=CARTESIAN_POINT('Ctrl Pts',(12.1623797632102,73.362499999717,-3.95179673813154));
#279059=CARTESIAN_POINT('Ctrl Pts',(9.83957192047902,73.5124999997164,-7.14886745759543));
#279060=CARTESIAN_POINT('Ctrl Pts',(7.5167640777478,73.6624999997158,-10.3459381770593));
#279061=CARTESIAN_POINT('Ctrl Pts',(3.75838203887387,73.8124999997152,-11.5671105274575));
#279062=CARTESIAN_POINT('Ctrl Pts',(-5.58559122386497E-14,73.9624999997146,
-12.7882828778556));
#279063=CARTESIAN_POINT('Ctrl Pts',(-3.75838203887398,74.112499999714,-11.5671105274575));
#279064=CARTESIAN_POINT('Ctrl Pts',(-7.51676407774791,74.2624999997134,
-10.3459381770593));
#279065=CARTESIAN_POINT('Ctrl Pts',(-9.83957192047913,74.4124999997128,
-7.14886745759543));
#279066=CARTESIAN_POINT('Ctrl Pts',(-12.1623797632103,74.5624999997122,
-3.95179673813153));
#279067=CARTESIAN_POINT('Ctrl Pts',(-12.1623797632103,74.7124999997116,
2.97892388940601E-15));
#279068=CARTESIAN_POINT('Ctrl Pts',(-12.1623797632103,74.862499999711,3.95179673813154));
#279069=CARTESIAN_POINT('Ctrl Pts',(-9.83957192047913,75.0124999997104,
7.14886745759543));
#279070=CARTESIAN_POINT('Ctrl Pts',(-7.51676407774791,75.1624999997098,
10.3459381770593));
#279071=CARTESIAN_POINT('Ctrl Pts',(-3.75838203887398,75.3124999997092,
11.5671105274575));
#279072=CARTESIAN_POINT('Ctrl Pts',(-5.35875409358893E-14,75.4624999997086,
12.7882828778556));
#279073=CARTESIAN_POINT('Ctrl Pts',(3.75838203887388,75.612499999708,11.5671105274575));
#279074=CARTESIAN_POINT('Ctrl Pts',(7.5167640777478,75.7624999997074,10.3459381770593));
#279075=CARTESIAN_POINT('Ctrl Pts',(9.83957192047902,75.9124999997068,7.14886745759543));
#279076=CARTESIAN_POINT('Ctrl Pts',(12.1623797632102,76.0624999997062,3.95179673813153));
#279077=CARTESIAN_POINT('Ctrl Pts',(12.1623797632102,76.2124999997056,-1.489461944703E-15));
#279078=CARTESIAN_POINT('Ctrl Pts',(12.1623797632102,76.362499999705,-3.95179673813154));
#279079=CARTESIAN_POINT('Ctrl Pts',(9.83957192047902,76.5124999997044,-7.14886745759543));
#279080=CARTESIAN_POINT('Ctrl Pts',(7.5167640777478,76.6624999997038,-10.3459381770593));
#279081=CARTESIAN_POINT('Ctrl Pts',(3.75838203887387,76.8124999997032,-11.5671105274575));
#279082=CARTESIAN_POINT('Ctrl Pts',(-5.75836215103115E-14,76.9624999997026,
-12.7882828778556));
#279083=CARTESIAN_POINT('Ctrl Pts',(-3.75838203887399,77.112499999702,-11.5671105274575));
#279084=CARTESIAN_POINT('Ctrl Pts',(-7.51676407774791,77.2624999997014,
-10.3459381770593));
#279085=CARTESIAN_POINT('Ctrl Pts',(-9.83957192047913,77.4124999997008,
-7.14886745759543));
#279086=CARTESIAN_POINT('Ctrl Pts',(-12.1623797632103,77.5624999997002,
-3.95179673813153));
#279087=CARTESIAN_POINT('Ctrl Pts',(-12.1623797632103,77.7124999996996,
2.97892388940601E-15));
#279088=CARTESIAN_POINT('Ctrl Pts',(-12.1623797632103,77.862499999699,3.95179673813154));
#279089=CARTESIAN_POINT('Ctrl Pts',(-9.83957192047913,78.0124999996984,
7.14886745759543));
#279090=CARTESIAN_POINT('Ctrl Pts',(-7.51676407774791,78.1624999996978,
10.3459381770593));
#279091=CARTESIAN_POINT('Ctrl Pts',(-3.75838203887398,78.3124999996972,
11.5671105274575));
#279092=CARTESIAN_POINT('Ctrl Pts',(-5.53152502075511E-14,78.4624999996966,
12.7882828778556));
#279093=CARTESIAN_POINT('Ctrl Pts',(3.75838203887387,78.612499999696,11.5671105274575));
#279094=CARTESIAN_POINT('Ctrl Pts',(7.5167640777478,78.7624999996954,10.3459381770593));
#279095=CARTESIAN_POINT('Ctrl Pts',(9.83957192047902,78.9124999996948,7.14886745759543));
#279096=CARTESIAN_POINT('Ctrl Pts',(12.1623797632102,79.0624999996942,3.95179673813153));
#279097=CARTESIAN_POINT('Ctrl Pts',(12.1623797632102,79.2124999996936,-1.489461944703E-15));
#279098=CARTESIAN_POINT('Ctrl Pts',(12.1623797632102,79.362499999693,-3.95179673813154));
#279099=CARTESIAN_POINT('Ctrl Pts',(9.83957192047902,79.5124999996924,-7.14886745759543));
#279100=CARTESIAN_POINT('Ctrl Pts',(7.5167640777478,79.6624999996918,-10.3459381770593));
#279101=CARTESIAN_POINT('Ctrl Pts',(3.75838203887387,79.8124999996912,-11.5671105274575));
#279102=CARTESIAN_POINT('Ctrl Pts',(-5.93113307819734E-14,79.9624999996906,
-12.7882828778556));
#279103=CARTESIAN_POINT('Ctrl Pts',(-3.75838203887399,80.11249999969,-11.5671105274575));
#279104=CARTESIAN_POINT('Ctrl Pts',(-7.51676407774791,80.2624999996894,
-10.3459381770593));
#279105=CARTESIAN_POINT('Ctrl Pts',(-9.83957192047913,80.4124999996888,
-7.14886745759543));
#279106=CARTESIAN_POINT('Ctrl Pts',(-12.1623797632104,80.5624999996882,
-3.95179673813153));
#279107=CARTESIAN_POINT('Ctrl Pts',(-12.1623797632104,80.7124999996876,
2.97892388940601E-15));
#279108=CARTESIAN_POINT('Ctrl Pts',(-12.1623797632104,80.862499999687,3.95179673813154));
#279109=CARTESIAN_POINT('Ctrl Pts',(-9.83957192047913,81.0124999996864,
7.14886745759543));
#279110=CARTESIAN_POINT('Ctrl Pts',(-7.51676407774791,81.1624999996858,
10.3459381770593));
#279111=CARTESIAN_POINT('Ctrl Pts',(-3.75838203887399,81.3124999996852,
11.5671105274575));
#279112=CARTESIAN_POINT('Ctrl Pts',(-5.70429594792129E-14,81.4624999996846,
12.7882828778556));
#279113=CARTESIAN_POINT('Ctrl Pts',(3.75838203887387,81.612499999684,11.5671105274575));
#279114=CARTESIAN_POINT('Ctrl Pts',(7.5167640777478,81.7624999996834,10.3459381770593));
#279115=CARTESIAN_POINT('Ctrl Pts',(9.83957192047902,81.9124999996828,7.14886745759543));
#279116=CARTESIAN_POINT('Ctrl Pts',(12.1623797632102,82.0624999996822,3.95179673813153));
#279117=CARTESIAN_POINT('Ctrl Pts',(12.1623797632102,82.2124999996816,-1.489461944703E-15));
#279118=CARTESIAN_POINT('Ctrl Pts',(12.1623797632102,82.362499999681,-3.95179673813154));
#279119=CARTESIAN_POINT('Ctrl Pts',(9.83957192047902,82.5124999996804,-7.14886745759543));
#279120=CARTESIAN_POINT('Ctrl Pts',(7.5167640777478,82.6624999996798,-10.3459381770593));
#279121=CARTESIAN_POINT('Ctrl Pts',(3.75838203887387,82.8124999996792,-11.5671105274575));
#279122=CARTESIAN_POINT('Ctrl Pts',(-6.10390400536352E-14,82.9624999996786,
-12.7882828778556));
#279123=CARTESIAN_POINT('Ctrl Pts',(-3.75838203887399,83.112499999678,-11.5671105274575));
#279124=CARTESIAN_POINT('Ctrl Pts',(-7.51676407774792,83.2624999996774,
-10.3459381770593));
#279125=CARTESIAN_POINT('Ctrl Pts',(-9.83957192047914,83.4124999996768,
-7.14886745759543));
#279126=CARTESIAN_POINT('Ctrl Pts',(-12.1623797632104,83.5624999996762,
-3.95179673813153));
#279127=CARTESIAN_POINT('Ctrl Pts',(-12.1623797632104,83.7124999996756,
2.97892388940601E-15));
#279128=CARTESIAN_POINT('Ctrl Pts',(-12.1623797632104,83.862499999675,3.95179673813154));
#279129=CARTESIAN_POINT('Ctrl Pts',(-9.83957192047913,84.0124999996744,
7.14886745759543));
#279130=CARTESIAN_POINT('Ctrl Pts',(-7.51676407774791,84.1624999996738,
10.3459381770593));
#279131=CARTESIAN_POINT('Ctrl Pts',(-3.75838203887399,84.3124999996732,
11.5671105274575));
#279132=CARTESIAN_POINT('Ctrl Pts',(-5.87706687508748E-14,84.4624999996726,
12.7882828778556));
#279133=CARTESIAN_POINT('Ctrl Pts',(3.75838203887387,84.6124999996721,11.5671105274575));
#279134=CARTESIAN_POINT('Ctrl Pts',(7.5167640777478,84.7624999996714,10.3459381770593));
#279135=CARTESIAN_POINT('Ctrl Pts',(9.83957192047902,84.9124999996708,7.14886745759543));
#279136=CARTESIAN_POINT('Ctrl Pts',(12.1623797632102,85.0624999996702,3.95179673813153));
#279137=CARTESIAN_POINT('Ctrl Pts',(12.1623797632102,85.2124999996696,-1.489461944703E-15));
#279138=CARTESIAN_POINT('Ctrl Pts',(12.1623797632102,85.362499999669,-3.95179673813154));
#279139=CARTESIAN_POINT('Ctrl Pts',(9.83957192047901,85.5124999996684,-7.14886745759543));
#279140=CARTESIAN_POINT('Ctrl Pts',(7.5167640777478,85.6624999996678,-10.3459381770593));
#279141=CARTESIAN_POINT('Ctrl Pts',(3.75838203887387,85.8124999996672,-11.5671105274575));
#279142=CARTESIAN_POINT('Ctrl Pts',(-6.27667493252971E-14,85.9624999996666,
-12.7882828778556));
#279143=CARTESIAN_POINT('Ctrl Pts',(-3.75838203887399,86.112499999666,-11.5671105274575));
#279144=CARTESIAN_POINT('Ctrl Pts',(-7.51676407774792,86.2624999996654,
-10.3459381770593));
#279145=CARTESIAN_POINT('Ctrl Pts',(-9.83957192047914,86.4124999996648,
-7.14886745759543));
#279146=CARTESIAN_POINT('Ctrl Pts',(-12.1623797632104,86.5624999996642,
-3.95179673813153));
#279147=CARTESIAN_POINT('Ctrl Pts',(-12.1623797632104,86.7124999996636,
2.97892388940601E-15));
#279148=CARTESIAN_POINT('Ctrl Pts',(-12.1623797632104,86.862499999663,3.95179673813154));
#279149=CARTESIAN_POINT('Ctrl Pts',(-9.83957192047914,87.0124999996624,
7.14886745759543));
#279150=CARTESIAN_POINT('Ctrl Pts',(-7.51676407774792,87.1624999996618,
10.3459381770593));
#279151=CARTESIAN_POINT('Ctrl Pts',(-3.75838203887399,87.3124999996612,
11.5671105274575));
#279152=CARTESIAN_POINT('Ctrl Pts',(-6.04983780225366E-14,87.4624999996606,
12.7882828778556));
#279153=CARTESIAN_POINT('Ctrl Pts',(3.75838203887387,87.61249999966,11.5671105274575));
#279154=CARTESIAN_POINT('Ctrl Pts',(7.5167640777478,87.7624999996594,10.3459381770593));
#279155=CARTESIAN_POINT('Ctrl Pts',(9.83957192047901,87.9124999996588,7.14886745759543));
#279156=CARTESIAN_POINT('Ctrl Pts',(12.1623797632102,88.0624999996582,3.95179673813153));
#279157=CARTESIAN_POINT('Ctrl Pts',(12.1623797632102,88.2124999996576,-1.489461944703E-15));
#279158=CARTESIAN_POINT('Ctrl Pts',(12.1623797632102,88.362499999657,-3.95179673813154));
#279159=CARTESIAN_POINT('Ctrl Pts',(9.83957192047901,88.5124999996564,-7.14886745759543));
#279160=CARTESIAN_POINT('Ctrl Pts',(7.51676407774779,88.6624999996558,-10.3459381770593));
#279161=CARTESIAN_POINT('Ctrl Pts',(3.75838203887386,88.8124999996552,-11.5671105274575));
#279162=CARTESIAN_POINT('Ctrl Pts',(-6.44944585969589E-14,88.9624999996546,
-12.7882828778556));
#279163=CARTESIAN_POINT('Ctrl Pts',(-3.75838203887399,89.112499999654,-11.5671105274575));
#279164=CARTESIAN_POINT('Ctrl Pts',(-7.51676407774792,89.2624999996534,
-10.3459381770593));
#279165=CARTESIAN_POINT('Ctrl Pts',(-9.83957192047914,89.4124999996528,
-7.14886745759543));
#279166=CARTESIAN_POINT('Ctrl Pts',(-12.1623797632104,89.5624999996522,
-3.95179673813153));
#279167=CARTESIAN_POINT('Ctrl Pts',(-12.1623797632104,89.7124999996516,
2.97892388940601E-15));
#279168=CARTESIAN_POINT('Ctrl Pts',(-12.1623797632104,89.862499999651,3.95179673813154));
#279169=CARTESIAN_POINT('Ctrl Pts',(-9.83957192047914,90.0124999996504,
7.14886745759543));
#279170=CARTESIAN_POINT('Ctrl Pts',(-7.51676407774792,90.1624999996498,
10.3459381770593));
#279171=CARTESIAN_POINT('Ctrl Pts',(-3.75838203887399,90.3124999996492,
11.5671105274575));
#279172=CARTESIAN_POINT('Ctrl Pts',(-6.22260872941985E-14,90.4624999996486,
12.7882828778556));
#279173=CARTESIAN_POINT('Ctrl Pts',(3.75838203887387,90.612499999648,11.5671105274575));
#279174=CARTESIAN_POINT('Ctrl Pts',(7.5167640777478,90.7624999996474,10.3459381770593));
#279175=CARTESIAN_POINT('Ctrl Pts',(9.83957192047901,90.9124999996468,7.14886745759543));
#279176=CARTESIAN_POINT('Ctrl Pts',(12.1623797632102,91.0624999996462,3.95179673813153));
#279177=CARTESIAN_POINT('Ctrl Pts',(12.1623797632102,91.2124999996456,-1.489461944703E-15));
#279178=CARTESIAN_POINT('Ctrl Pts',(12.1623797632102,91.362499999645,-3.95179673813154));
#279179=CARTESIAN_POINT('Ctrl Pts',(9.83957192047901,91.5124999996444,-7.14886745759543));
#279180=CARTESIAN_POINT('Ctrl Pts',(7.51676407774779,91.6624999996438,-10.3459381770593));
#279181=CARTESIAN_POINT('Ctrl Pts',(3.75838203887386,91.8124999996432,-11.5671105274575));
#279182=CARTESIAN_POINT('Ctrl Pts',(-6.62221678686207E-14,91.9624999996426,
-12.7882828778556));
#279183=CARTESIAN_POINT('Ctrl Pts',(-3.75838203887399,92.112499999642,-11.5671105274575));
#279184=CARTESIAN_POINT('Ctrl Pts',(-7.51676407774792,92.2624999996414,
-10.3459381770593));
#279185=CARTESIAN_POINT('Ctrl Pts',(-9.83957192047914,92.4124999996408,
-7.14886745759543));
#279186=CARTESIAN_POINT('Ctrl Pts',(-12.1623797632104,92.5624999996402,
-3.95179673813153));
#279187=CARTESIAN_POINT('Ctrl Pts',(-12.1623797632104,92.7124999996396,
2.97892388940601E-15));
#279188=CARTESIAN_POINT('Ctrl Pts',(-12.1623797632104,92.862499999639,3.95179673813154));
#279189=CARTESIAN_POINT('Ctrl Pts',(-9.83957192047914,93.0124999996384,
7.14886745759543));
#279190=CARTESIAN_POINT('Ctrl Pts',(-7.51676407774792,93.1624999996378,
10.3459381770593));
#279191=CARTESIAN_POINT('Ctrl Pts',(-3.75838203887399,93.3124999996372,
11.5671105274575));
#279192=CARTESIAN_POINT('Ctrl Pts',(-6.39537965658603E-14,93.4624999996366,
12.7882828778556));
#279193=CARTESIAN_POINT('Ctrl Pts',(3.75838203887386,93.612499999636,11.5671105274575));
#279194=CARTESIAN_POINT('Ctrl Pts',(7.51676407774779,93.7624999996354,10.3459381770593));
#279195=CARTESIAN_POINT('Ctrl Pts',(9.83957192047901,93.9124999996348,7.14886745759543));
#279196=CARTESIAN_POINT('Ctrl Pts',(12.1623797632102,94.0624999996342,3.95179673813153));
#279197=CARTESIAN_POINT('Ctrl Pts',(12.1623797632102,94.2124999996336,-1.489461944703E-15));
#279198=CARTESIAN_POINT('Ctrl Pts',(12.1623797632102,94.362499999633,-3.95179673813154));
#279199=CARTESIAN_POINT('Ctrl Pts',(9.83957192047901,94.5124999996324,-7.14886745759543));
#279200=CARTESIAN_POINT('Ctrl Pts',(7.51676407774779,94.6624999996318,-10.3459381770593));
#279201=CARTESIAN_POINT('Ctrl Pts',(3.75838203887386,94.8124999996312,-11.5671105274575));
#279202=CARTESIAN_POINT('Ctrl Pts',(-6.79498771402825E-14,94.9624999996306,
-12.7882828778556));
#279203=CARTESIAN_POINT('Ctrl Pts',(-3.758382038874,95.11249999963,-11.5671105274575));
#279204=CARTESIAN_POINT('Ctrl Pts',(-7.51676407774792,95.2624999996294,
-10.3459381770593));
#279205=CARTESIAN_POINT('Ctrl Pts',(-9.83957192047914,95.4124999996288,
-7.14886745759543));
#279206=CARTESIAN_POINT('Ctrl Pts',(-12.1623797632104,95.5624999996282,
-3.95179673813153));
#279207=CARTESIAN_POINT('Ctrl Pts',(-12.1623797632104,95.7124999996276,
2.97892388940601E-15));
#279208=CARTESIAN_POINT('Ctrl Pts',(-12.1623797632104,95.862499999627,3.95179673813154));
#279209=CARTESIAN_POINT('Ctrl Pts',(-9.83957192047914,96.0124999996264,
7.14886745759543));
#279210=CARTESIAN_POINT('Ctrl Pts',(-7.51676407774792,96.1624999996258,
10.3459381770593));
#279211=CARTESIAN_POINT('Ctrl Pts',(-3.75838203887399,96.3124999996252,
11.5671105274575));
#279212=CARTESIAN_POINT('Ctrl Pts',(-6.56815058375222E-14,96.4624999996246,
12.7882828778556));
#279213=CARTESIAN_POINT('Ctrl Pts',(3.75838203887386,96.612499999624,11.5671105274575));
#279214=CARTESIAN_POINT('Ctrl Pts',(7.51676407774779,96.7624999996234,10.3459381770593));
#279215=CARTESIAN_POINT('Ctrl Pts',(9.83957192047901,96.9124999996228,7.14886745759543));
#279216=CARTESIAN_POINT('Ctrl Pts',(12.1623797632102,97.0624999996222,3.95179673813153));
#279217=CARTESIAN_POINT('Ctrl Pts',(12.1623797632102,97.2124999996216,-1.489461944703E-15));
#279218=CARTESIAN_POINT('Ctrl Pts',(12.1623797632102,97.3624999996211,-3.95179673813154));
#279219=CARTESIAN_POINT('Ctrl Pts',(9.83957192047901,97.5124999996204,-7.14886745759543));
#279220=CARTESIAN_POINT('Ctrl Pts',(7.51676407774779,97.6624999996198,-10.3459381770593));
#279221=CARTESIAN_POINT('Ctrl Pts',(3.75838203887386,97.8124999996192,-11.5671105274575));
#279222=CARTESIAN_POINT('Ctrl Pts',(-6.96775864119444E-14,97.9624999996187,
-12.7882828778556));
#279223=CARTESIAN_POINT('Ctrl Pts',(-3.758382038874,98.112499999618,-11.5671105274575));
#279224=CARTESIAN_POINT('Ctrl Pts',(-7.51676407774793,98.2624999996174,
-10.3459381770593));
#279225=CARTESIAN_POINT('Ctrl Pts',(-9.83957192047914,98.4124999996168,
-7.14886745759543));
#279226=CARTESIAN_POINT('Ctrl Pts',(-12.1623797632104,98.5624999996162,
-3.95179673813153));
#279227=CARTESIAN_POINT('Ctrl Pts',(-12.1623797632104,98.7124999996156,
2.97892388940601E-15));
#279228=CARTESIAN_POINT('Ctrl Pts',(-12.1623797632104,98.862499999615,3.95179673813154));
#279229=CARTESIAN_POINT('Ctrl Pts',(-9.83957192047914,99.0124999996144,
7.14886745759543));
#279230=CARTESIAN_POINT('Ctrl Pts',(-7.51676407774792,99.1624999996138,
10.3459381770593));
#279231=CARTESIAN_POINT('Ctrl Pts',(-3.758382038874,99.3124999996132,11.5671105274575));
#279232=CARTESIAN_POINT('Ctrl Pts',(-6.7409215109184E-14,99.4624999996126,
12.7882828778556));
#279233=CARTESIAN_POINT('Ctrl Pts',(3.75838203887386,99.612499999612,11.5671105274575));
#279234=CARTESIAN_POINT('Ctrl Pts',(7.51676407774779,99.7624999996114,10.3459381770593));
#279235=CARTESIAN_POINT('Ctrl Pts',(9.83957192047901,99.9124999996108,7.14886745759543));
#279236=CARTESIAN_POINT('Ctrl Pts',(12.1623797632102,100.06249999961,3.95179673813153));
#279237=CARTESIAN_POINT('Ctrl Pts',(12.1623797632102,100.21249999961,-1.489461944703E-15));
#279238=CARTESIAN_POINT('Ctrl Pts',(12.1623797632102,100.362499999609,-3.95179673813154));
#279239=CARTESIAN_POINT('Ctrl Pts',(9.839571920479,100.512499999608,-7.14886745759543));
#279240=CARTESIAN_POINT('Ctrl Pts',(7.51676407774779,100.662499999608,-10.3459381770593));
#279241=CARTESIAN_POINT('Ctrl Pts',(3.75838203887386,100.812499999607,-11.5671105274575));
#279242=CARTESIAN_POINT('Ctrl Pts',(-7.14052956836063E-14,100.962499999607,
-12.7882828778556));
#279243=CARTESIAN_POINT('Ctrl Pts',(-3.758382038874,101.112499999606,-11.5671105274575));
#279244=CARTESIAN_POINT('Ctrl Pts',(-7.51676407774793,101.262499999605,
-10.3459381770593));
#279245=CARTESIAN_POINT('Ctrl Pts',(-9.83957192047915,101.412499999605,
-7.14886745759543));
#279246=CARTESIAN_POINT('Ctrl Pts',(-12.1623797632104,101.562499999604,
-3.95179673813153));
#279247=CARTESIAN_POINT('Ctrl Pts',(-12.1623797632104,101.712499999604,
2.97892388940601E-15));
#279248=CARTESIAN_POINT('Ctrl Pts',(-12.1623797632104,101.862499999603,
3.95179673813154));
#279249=CARTESIAN_POINT('Ctrl Pts',(-9.83957192047914,102.012499999602,
7.14886745759543));
#279250=CARTESIAN_POINT('Ctrl Pts',(-7.51676407774793,102.162499999602,
10.3459381770593));
#279251=CARTESIAN_POINT('Ctrl Pts',(-3.758382038874,102.312499999601,11.5671105274575));
#279252=CARTESIAN_POINT('Ctrl Pts',(-6.91369243808458E-14,102.462499999601,
12.7882828778556));
#279253=CARTESIAN_POINT('Ctrl Pts',(3.75838203887386,102.6124999996,11.5671105274575));
#279254=CARTESIAN_POINT('Ctrl Pts',(7.51676407774779,102.762499999599,10.3459381770593));
#279255=CARTESIAN_POINT('Ctrl Pts',(9.839571920479,102.912499999599,7.14886745759543));
#279256=CARTESIAN_POINT('Ctrl Pts',(12.1623797632102,103.062499999598,3.95179673813153));
#279257=CARTESIAN_POINT('Ctrl Pts',(12.1623797632102,103.212499999598,-1.489461944703E-15));
#279258=CARTESIAN_POINT('Ctrl Pts',(12.1623797632102,103.362499999597,-3.95179673813154));
#279259=CARTESIAN_POINT('Ctrl Pts',(9.839571920479,103.512499999596,-7.14886745759543));
#279260=CARTESIAN_POINT('Ctrl Pts',(7.51676407774779,103.662499999596,-10.3459381770593));
#279261=CARTESIAN_POINT('Ctrl Pts',(3.75838203887386,103.812499999595,-11.5671105274575));
#279262=CARTESIAN_POINT('Ctrl Pts',(-7.31330049552681E-14,103.962499999595,
-12.7882828778556));
#279263=CARTESIAN_POINT('Ctrl Pts',(-3.758382038874,104.112499999594,-11.5671105274575));
#279264=CARTESIAN_POINT('Ctrl Pts',(-7.51676407774793,104.262499999593,
-10.3459381770593));
#279265=CARTESIAN_POINT('Ctrl Pts',(-9.83957192047915,104.412499999593,
-7.14886745759543));
#279266=CARTESIAN_POINT('Ctrl Pts',(-12.1623797632104,104.562499999592,
-3.95179673813153));
#279267=CARTESIAN_POINT('Ctrl Pts',(-12.1623797632104,104.712499999592,
2.97892388940601E-15));
#279268=CARTESIAN_POINT('Ctrl Pts',(-12.1623797632104,104.862499999591,
3.95179673813154));
#279269=CARTESIAN_POINT('Ctrl Pts',(-9.83957192047915,105.01249999959,7.14886745759543));
#279270=CARTESIAN_POINT('Ctrl Pts',(-7.51676407774793,105.16249999959,10.3459381770593));
#279271=CARTESIAN_POINT('Ctrl Pts',(-3.758382038874,105.312499999589,11.5671105274575));
#279272=CARTESIAN_POINT('Ctrl Pts',(-7.08646336525076E-14,105.462499999589,
12.7882828778556));
#279273=CARTESIAN_POINT('Ctrl Pts',(3.75838203887386,105.612499999588,11.5671105274575));
#279274=CARTESIAN_POINT('Ctrl Pts',(7.51676407774779,105.762499999587,10.3459381770593));
#279275=CARTESIAN_POINT('Ctrl Pts',(9.839571920479,105.912499999587,7.14886745759543));
#279276=CARTESIAN_POINT('Ctrl Pts',(12.1623797632102,106.062499999586,3.95179673813153));
#279277=CARTESIAN_POINT('Ctrl Pts',(12.1623797632102,106.212499999586,-1.489461944703E-15));
#279278=CARTESIAN_POINT('Ctrl Pts',(12.1623797632102,106.362499999585,-3.95179673813154));
#279279=CARTESIAN_POINT('Ctrl Pts',(9.839571920479,106.512499999584,-7.14886745759543));
#279280=CARTESIAN_POINT('Ctrl Pts',(7.51676407774778,106.662499999584,-10.3459381770593));
#279281=CARTESIAN_POINT('Ctrl Pts',(3.75838203887385,106.812499999583,-11.5671105274575));
#279282=CARTESIAN_POINT('Ctrl Pts',(-7.48607142269299E-14,106.962499999583,
-12.7882828778556));
#279283=CARTESIAN_POINT('Ctrl Pts',(-3.758382038874,107.112499999582,-11.5671105274575));
#279284=CARTESIAN_POINT('Ctrl Pts',(-7.51676407774793,107.262499999581,
-10.3459381770593));
#279285=CARTESIAN_POINT('Ctrl Pts',(-9.83957192047915,107.412499999581,
-7.14886745759543));
#279286=CARTESIAN_POINT('Ctrl Pts',(-12.1623797632104,107.56249999958,-3.95179673813153));
#279287=CARTESIAN_POINT('Ctrl Pts',(-12.1623797632104,107.71249999958,2.97892388940601E-15));
#279288=CARTESIAN_POINT('Ctrl Pts',(-12.1623797632104,107.862499999579,
3.95179673813154));
#279289=CARTESIAN_POINT('Ctrl Pts',(-9.83957192047915,108.012499999578,
7.14886745759543));
#279290=CARTESIAN_POINT('Ctrl Pts',(-7.51676407774793,108.162499999578,
10.3459381770593));
#279291=CARTESIAN_POINT('Ctrl Pts',(-3.758382038874,108.312499999577,11.5671105274575));
#279292=CARTESIAN_POINT('Ctrl Pts',(-7.25923429241695E-14,108.462499999577,
12.7882828778556));
#279293=CARTESIAN_POINT('Ctrl Pts',(3.75838203887386,108.612499999576,11.5671105274575));
#279294=CARTESIAN_POINT('Ctrl Pts',(7.51676407774779,108.762499999575,10.3459381770593));
#279295=CARTESIAN_POINT('Ctrl Pts',(9.839571920479,108.912499999575,7.14886745759543));
#279296=CARTESIAN_POINT('Ctrl Pts',(12.1623797632102,109.062499999574,3.95179673813153));
#279297=CARTESIAN_POINT('Ctrl Pts',(12.1623797632102,109.212499999574,-1.489461944703E-15));
#279298=CARTESIAN_POINT('Ctrl Pts',(12.1623797632102,109.362499999573,-3.95179673813154));
#279299=CARTESIAN_POINT('Ctrl Pts',(9.839571920479,109.512499999572,-7.14886745759543));
#279300=CARTESIAN_POINT('Ctrl Pts',(7.51676407774778,109.662499999572,-10.3459381770593));
#279301=CARTESIAN_POINT('Ctrl Pts',(3.75838203887385,109.812499999571,-11.5671105274575));
#279302=CARTESIAN_POINT('Ctrl Pts',(-7.65884234985918E-14,109.962499999571,
-12.7882828778556));
#279303=CARTESIAN_POINT('Ctrl Pts',(-3.75838203887401,110.11249999957,-11.5671105274575));
#279304=CARTESIAN_POINT('Ctrl Pts',(-7.51676407774793,110.262499999569,
-10.3459381770593));
#279305=CARTESIAN_POINT('Ctrl Pts',(-9.83957192047915,110.412499999569,
-7.14886745759543));
#279306=CARTESIAN_POINT('Ctrl Pts',(-12.1623797632104,110.562499999568,
-3.95179673813153));
#279307=CARTESIAN_POINT('Ctrl Pts',(-12.1623797632104,110.712499999568,
2.97892388940601E-15));
#279308=CARTESIAN_POINT('Ctrl Pts',(-12.1623797632104,110.862499999567,
3.95179673813154));
#279309=CARTESIAN_POINT('Ctrl Pts',(-9.83957192047915,111.012499999566,
7.14886745759543));
#279310=CARTESIAN_POINT('Ctrl Pts',(-7.51676407774793,111.162499999566,
10.3459381770593));
#279311=CARTESIAN_POINT('Ctrl Pts',(-3.758382038874,111.312499999565,11.5671105274575));
#279312=CARTESIAN_POINT('Ctrl Pts',(-7.43200521958313E-14,111.462499999565,
12.7882828778556));
#279313=CARTESIAN_POINT('Ctrl Pts',(3.75838203887385,111.612499999564,11.5671105274575));
#279314=CARTESIAN_POINT('Ctrl Pts',(7.51676407774778,111.762499999563,10.3459381770593));
#279315=CARTESIAN_POINT('Ctrl Pts',(9.839571920479,111.912499999563,7.14886745759543));
#279316=CARTESIAN_POINT('Ctrl Pts',(12.1623797632102,112.062499999562,3.95179673813153));
#279317=CARTESIAN_POINT('Ctrl Pts',(12.1623797632102,112.212499999562,-1.489461944703E-15));
#279318=CARTESIAN_POINT('Ctrl Pts',(12.1623797632102,112.362499999561,-3.95179673813154));
#279319=CARTESIAN_POINT('Ctrl Pts',(9.839571920479,112.51249999956,-7.14886745759543));
#279320=CARTESIAN_POINT('Ctrl Pts',(7.51676407774778,112.66249999956,-10.3459381770593));
#279321=CARTESIAN_POINT('Ctrl Pts',(3.75838203887385,112.812499999559,-11.5671105274575));
#279322=CARTESIAN_POINT('Ctrl Pts',(-7.83161327702536E-14,112.962499999559,
-12.7882828778556));
#279323=CARTESIAN_POINT('Ctrl Pts',(-3.75838203887401,113.112499999558,
-11.5671105274575));
#279324=CARTESIAN_POINT('Ctrl Pts',(-7.51676407774793,113.262499999557,
-10.3459381770593));
#279325=CARTESIAN_POINT('Ctrl Pts',(-9.83957192047915,113.412499999557,
-7.14886745759543));
#279326=CARTESIAN_POINT('Ctrl Pts',(-12.1623797632104,113.562499999556,
-3.95179673813153));
#279327=CARTESIAN_POINT('Ctrl Pts',(-12.1623797632104,113.712499999556,
2.97892388940601E-15));
#279328=CARTESIAN_POINT('Ctrl Pts',(-12.1623797632104,113.862499999555,
3.95179673813154));
#279329=CARTESIAN_POINT('Ctrl Pts',(-9.83957192047915,114.012499999554,
7.14886745759543));
#279330=CARTESIAN_POINT('Ctrl Pts',(-7.51676407774793,114.162499999554,
10.3459381770593));
#279331=CARTESIAN_POINT('Ctrl Pts',(-3.758382038874,114.312499999553,11.5671105274575));
#279332=CARTESIAN_POINT('Ctrl Pts',(-7.60477614674932E-14,114.462499999553,
12.7882828778556));
#279333=CARTESIAN_POINT('Ctrl Pts',(3.75838203887385,114.612499999552,11.5671105274575));
#279334=CARTESIAN_POINT('Ctrl Pts',(7.51676407774778,114.762499999551,10.3459381770593));
#279335=CARTESIAN_POINT('Ctrl Pts',(9.839571920479,114.912499999551,7.14886745759543));
#279336=CARTESIAN_POINT('Ctrl Pts',(12.1623797632102,115.06249999955,3.95179673813153));
#279337=CARTESIAN_POINT('Ctrl Pts',(12.1623797632102,115.21249999955,-1.489461944703E-15));
#279338=CARTESIAN_POINT('Ctrl Pts',(12.1623797632102,115.362499999549,-3.95179673813154));
#279339=CARTESIAN_POINT('Ctrl Pts',(9.839571920479,115.512499999548,-7.14886745759543));
#279340=CARTESIAN_POINT('Ctrl Pts',(7.51676407774778,115.662499999548,-10.3459381770593));
#279341=CARTESIAN_POINT('Ctrl Pts',(3.75838203887385,115.812499999547,-11.5671105274575));
#279342=CARTESIAN_POINT('Ctrl Pts',(-8.00438420419154E-14,115.962499999547,
-12.7882828778556));
#279343=CARTESIAN_POINT('Ctrl Pts',(-3.75838203887401,116.112499999546,
-11.5671105274575));
#279344=CARTESIAN_POINT('Ctrl Pts',(-7.51676407774794,116.262499999545,
-10.3459381770593));
#279345=CARTESIAN_POINT('Ctrl Pts',(-9.83957192047916,116.412499999545,
-7.14886745759543));
#279346=CARTESIAN_POINT('Ctrl Pts',(-12.1623797632104,116.562499999544,
-3.95179673813153));
#279347=CARTESIAN_POINT('Ctrl Pts',(-12.1623797632104,116.712499999544,
2.97892388940601E-15));
#279348=CARTESIAN_POINT('Ctrl Pts',(-12.1623797632104,116.862499999543,
3.95179673813154));
#279349=CARTESIAN_POINT('Ctrl Pts',(-9.83957192047915,117.012499999542,
7.14886745759543));
#279350=CARTESIAN_POINT('Ctrl Pts',(-7.51676407774793,117.162499999542,
10.3459381770593));
#279351=CARTESIAN_POINT('Ctrl Pts',(-3.75838203887401,117.312499999541,
11.5671105274575));
#279352=CARTESIAN_POINT('Ctrl Pts',(-7.7775470739155E-14,117.462499999541,
12.7882828778556));
#279353=CARTESIAN_POINT('Ctrl Pts',(3.75838203887385,117.61249999954,11.5671105274575));
#279354=CARTESIAN_POINT('Ctrl Pts',(7.51676407774778,117.762499999539,10.3459381770593));
#279355=CARTESIAN_POINT('Ctrl Pts',(9.839571920479,117.912499999539,7.14886745759543));
#279356=CARTESIAN_POINT('Ctrl Pts',(12.1623797632102,118.062499999538,3.95179673813153));
#279357=CARTESIAN_POINT('Ctrl Pts',(12.1623797632102,118.212499999538,-1.489461944703E-15));
#279358=CARTESIAN_POINT('Ctrl Pts',(12.1623797632102,118.362499999537,-3.95179673813154));
#279359=CARTESIAN_POINT('Ctrl Pts',(9.83957192047899,118.512499999536,-7.14886745759543));
#279360=CARTESIAN_POINT('Ctrl Pts',(7.51676407774778,118.662499999536,-10.3459381770593));
#279361=CARTESIAN_POINT('Ctrl Pts',(3.75838203887385,118.812499999535,-11.5671105274575));
#279362=CARTESIAN_POINT('Ctrl Pts',(-8.17715513135773E-14,118.962499999535,
-12.7882828778556));
#279363=CARTESIAN_POINT('Ctrl Pts',(-3.75838203887401,119.112499999534,
-11.5671105274575));
#279364=CARTESIAN_POINT('Ctrl Pts',(-7.51676407774794,119.262499999533,
-10.3459381770593));
#279365=CARTESIAN_POINT('Ctrl Pts',(-9.83957192047916,119.412499999533,
-7.14886745759543));
#279366=CARTESIAN_POINT('Ctrl Pts',(-12.1623797632104,119.562499999532,
-3.95179673813153));
#279367=CARTESIAN_POINT('Ctrl Pts',(-12.1623797632104,119.712499999532,
2.97892388940601E-15));
#279368=CARTESIAN_POINT('Ctrl Pts',(-12.1623797632104,119.862499999531,
3.95179673813154));
#279369=CARTESIAN_POINT('Ctrl Pts',(-9.83957192047916,120.01249999953,7.14886745759543));
#279370=CARTESIAN_POINT('Ctrl Pts',(-7.51676407774794,120.16249999953,10.3459381770593));
#279371=CARTESIAN_POINT('Ctrl Pts',(-3.75838203887401,120.312499999529,
11.5671105274575));
#279372=CARTESIAN_POINT('Ctrl Pts',(-7.95031800108169E-14,120.462499999529,
12.7882828778556));
#279373=CARTESIAN_POINT('Ctrl Pts',(3.75838203887385,120.612499999528,11.5671105274575));
#279374=CARTESIAN_POINT('Ctrl Pts',(7.51676407774778,120.762499999527,10.3459381770593));
#279375=CARTESIAN_POINT('Ctrl Pts',(9.83957192047899,120.912499999527,7.14886745759543));
#279376=CARTESIAN_POINT('Ctrl Pts',(12.1623797632102,121.062499999526,3.95179673813153));
#279377=CARTESIAN_POINT('Ctrl Pts',(12.1623797632102,121.212499999526,-1.489461944703E-15));
#279378=CARTESIAN_POINT('Ctrl Pts',(12.1623797632102,121.362499999525,-3.95179673813154));
#279379=CARTESIAN_POINT('Ctrl Pts',(9.83957192047899,121.512499999524,-7.14886745759543));
#279380=CARTESIAN_POINT('Ctrl Pts',(7.51676407774777,121.662499999524,-10.3459381770593));
#279381=CARTESIAN_POINT('Ctrl Pts',(3.75838203887385,121.812499999523,-11.5671105274575));
#279382=CARTESIAN_POINT('Ctrl Pts',(-8.34992605852391E-14,121.962499999523,
-12.7882828778556));
#279383=CARTESIAN_POINT('Ctrl Pts',(-3.75838203887401,122.112499999522,
-11.5671105274575));
#279384=CARTESIAN_POINT('Ctrl Pts',(-7.51676407774794,122.262499999521,
-10.3459381770593));
#279385=CARTESIAN_POINT('Ctrl Pts',(-9.83957192047916,122.412499999521,
-7.14886745759543));
#279386=CARTESIAN_POINT('Ctrl Pts',(-12.1623797632104,122.56249999952,-3.95179673813153));
#279387=CARTESIAN_POINT('Ctrl Pts',(-12.1623797632104,122.71249999952,2.97892388940601E-15));
#279388=CARTESIAN_POINT('Ctrl Pts',(-12.1623797632104,122.862499999519,
3.95179673813154));
#279389=CARTESIAN_POINT('Ctrl Pts',(-9.83957192047916,123.012499999518,
7.14886745759543));
#279390=CARTESIAN_POINT('Ctrl Pts',(-7.51676407774794,123.162499999518,
10.3459381770593));
#279391=CARTESIAN_POINT('Ctrl Pts',(-3.75838203887401,123.312499999517,
11.5671105274575));
#279392=CARTESIAN_POINT('Ctrl Pts',(-8.12308892824787E-14,123.462499999517,
12.7882828778556));
#279393=CARTESIAN_POINT('Ctrl Pts',(3.75838203887385,123.612499999516,11.5671105274575));
#279394=CARTESIAN_POINT('Ctrl Pts',(7.51676407774778,123.762499999515,10.3459381770593));
#279395=CARTESIAN_POINT('Ctrl Pts',(9.83957192047899,123.912499999515,7.14886745759543));
#279396=CARTESIAN_POINT('Ctrl Pts',(12.1623797632102,124.062499999514,3.95179673813153));
#279397=CARTESIAN_POINT('Ctrl Pts',(12.1623797632102,124.212499999514,-1.489461944703E-15));
#279398=CARTESIAN_POINT('Ctrl Pts',(12.1623797632102,124.362499999513,-3.95179673813154));
#279399=CARTESIAN_POINT('Ctrl Pts',(9.83957192047899,124.512499999512,-7.14886745759543));
#279400=CARTESIAN_POINT('Ctrl Pts',(7.51676407774777,124.662499999512,-10.3459381770593));
#279401=CARTESIAN_POINT('Ctrl Pts',(3.75838203887384,124.812499999511,-11.5671105274575));
#279402=CARTESIAN_POINT('Ctrl Pts',(-8.52269698569009E-14,124.962499999511,
-12.7882828778556));
#279403=CARTESIAN_POINT('Ctrl Pts',(-3.75838203887401,125.11249999951,-11.5671105274575));
#279404=CARTESIAN_POINT('Ctrl Pts',(-7.51676407774794,125.262499999509,
-10.3459381770593));
#279405=CARTESIAN_POINT('Ctrl Pts',(-9.83957192047916,125.412499999509,
-7.14886745759543));
#279406=CARTESIAN_POINT('Ctrl Pts',(-12.1623797632104,125.562499999508,
-3.95179673813153));
#279407=CARTESIAN_POINT('Ctrl Pts',(-12.1623797632104,125.712499999508,
2.97892388940601E-15));
#279408=CARTESIAN_POINT('Ctrl Pts',(-12.1623797632104,125.862499999507,
3.95179673813154));
#279409=CARTESIAN_POINT('Ctrl Pts',(-9.83957192047916,126.012499999506,
7.14886745759543));
#279410=CARTESIAN_POINT('Ctrl Pts',(-7.51676407774794,126.162499999506,
10.3459381770593));
#279411=CARTESIAN_POINT('Ctrl Pts',(-3.75838203887401,126.312499999505,
11.5671105274575));
#279412=CARTESIAN_POINT('Ctrl Pts',(-8.29585985541405E-14,126.462499999505,
12.7882828778556));
#279413=CARTESIAN_POINT('Ctrl Pts',(3.75838203887385,126.612499999504,11.5671105274575));
#279414=CARTESIAN_POINT('Ctrl Pts',(7.51676407774777,126.762499999503,10.3459381770593));
#279415=CARTESIAN_POINT('Ctrl Pts',(9.83957192047899,126.912499999503,7.14886745759543));
#279416=CARTESIAN_POINT('Ctrl Pts',(12.1623797632102,127.062499999502,3.95179673813153));
#279417=CARTESIAN_POINT('Ctrl Pts',(12.1623797632102,127.212499999502,-1.489461944703E-15));
#279418=CARTESIAN_POINT('Ctrl Pts',(12.1623797632102,127.362499999501,-3.95179673813154));
#279419=CARTESIAN_POINT('Ctrl Pts',(9.83957192047899,127.5124999995,-7.14886745759543));
#279420=CARTESIAN_POINT('Ctrl Pts',(7.51676407774777,127.6624999995,-10.3459381770593));
#279421=CARTESIAN_POINT('Ctrl Pts',(3.75838203887384,127.812499999499,-11.5671105274575));
#279422=CARTESIAN_POINT('Ctrl Pts',(-8.69546791285628E-14,127.962499999499,
-12.7882828778556));
#279423=CARTESIAN_POINT('Ctrl Pts',(-3.75838203887402,128.112499999498,
-11.5671105274575));
#279424=CARTESIAN_POINT('Ctrl Pts',(-7.51676407774795,128.262499999497,
-10.3459381770593));
#279425=CARTESIAN_POINT('Ctrl Pts',(-9.83957192047916,128.412499999497,
-7.14886745759543));
#279426=CARTESIAN_POINT('Ctrl Pts',(-12.1623797632104,128.562499999496,
-3.95179673813153));
#279427=CARTESIAN_POINT('Ctrl Pts',(-12.1623797632104,128.712499999496,
2.97892388940601E-15));
#279428=CARTESIAN_POINT('Ctrl Pts',(-12.1623797632104,128.862499999495,
3.95179673813154));
#279429=CARTESIAN_POINT('Ctrl Pts',(-9.83957192047916,129.012499999494,
7.14886745759543));
#279430=CARTESIAN_POINT('Ctrl Pts',(-7.51676407774794,129.162499999494,
10.3459381770593));
#279431=CARTESIAN_POINT('Ctrl Pts',(-3.75838203887401,129.312499999493,
11.5671105274575));
#279432=CARTESIAN_POINT('Ctrl Pts',(-8.46863078258024E-14,129.462499999493,
12.7882828778556));
#279433=CARTESIAN_POINT('Ctrl Pts',(3.75838203887384,129.612499999492,11.5671105274575));
#279434=CARTESIAN_POINT('Ctrl Pts',(7.51676407774777,129.762499999491,10.3459381770593));
#279435=CARTESIAN_POINT('Ctrl Pts',(9.83957192047899,129.912499999491,7.14886745759543));
#279436=CARTESIAN_POINT('Ctrl Pts',(12.1623797632102,130.06249999949,3.95179673813153));
#279437=CARTESIAN_POINT('Ctrl Pts',(12.1623797632102,130.21249999949,-1.489461944703E-15));
#279438=CARTESIAN_POINT('Ctrl Pts',(12.1623797632102,130.362499999489,-3.95179673813154));
#279439=CARTESIAN_POINT('Ctrl Pts',(9.83957192047899,130.512499999488,-7.14886745759543));
#279440=CARTESIAN_POINT('Ctrl Pts',(7.51676407774777,130.662499999488,-10.3459381770593));
#279441=CARTESIAN_POINT('Ctrl Pts',(3.75838203887384,130.812499999487,-11.5671105274575));
#279442=CARTESIAN_POINT('Ctrl Pts',(-8.86823884002247E-14,130.962499999487,
-12.7882828778556));
#279443=CARTESIAN_POINT('Ctrl Pts',(-3.75838203887402,131.112499999486,
-11.5671105274575));
#279444=CARTESIAN_POINT('Ctrl Pts',(-7.51676407774795,131.262499999485,
-10.3459381770593));
#279445=CARTESIAN_POINT('Ctrl Pts',(-9.83957192047916,131.412499999485,
-7.14886745759543));
#279446=CARTESIAN_POINT('Ctrl Pts',(-12.1623797632104,131.562499999484,
-3.95179673813153));
#279447=CARTESIAN_POINT('Ctrl Pts',(-12.1623797632104,131.712499999484,
2.97892388940601E-15));
#279448=CARTESIAN_POINT('Ctrl Pts',(-12.1623797632104,131.862499999483,
3.95179673813154));
#279449=CARTESIAN_POINT('Ctrl Pts',(-9.83957192047916,132.012499999482,
7.14886745759543));
#279450=CARTESIAN_POINT('Ctrl Pts',(-7.51676407774795,132.162499999482,
10.3459381770593));
#279451=CARTESIAN_POINT('Ctrl Pts',(-3.75838203887402,132.312499999481,
11.5671105274575));
#279452=CARTESIAN_POINT('Ctrl Pts',(-8.64140170974642E-14,132.462499999481,
12.7882828778556));
#279453=CARTESIAN_POINT('Ctrl Pts',(3.75838203887384,132.61249999948,11.5671105274575));
#279454=CARTESIAN_POINT('Ctrl Pts',(7.51676407774777,132.762499999479,10.3459381770593));
#279455=CARTESIAN_POINT('Ctrl Pts',(9.83957192047899,132.912499999479,7.14886745759543));
#279456=CARTESIAN_POINT('Ctrl Pts',(12.1623797632102,133.062499999478,3.95179673813153));
#279457=CARTESIAN_POINT('Ctrl Pts',(12.1623797632102,133.212499999478,-1.489461944703E-15));
#279458=CARTESIAN_POINT('Ctrl Pts',(12.1623797632102,133.362499999477,-3.95179673813154));
#279459=CARTESIAN_POINT('Ctrl Pts',(9.83957192047898,133.512499999476,-7.14886745759543));
#279460=CARTESIAN_POINT('Ctrl Pts',(7.51676407774777,133.662499999476,-10.3459381770593));
#279461=CARTESIAN_POINT('Ctrl Pts',(3.75838203887384,133.812499999475,-11.5671105274575));
#279462=CARTESIAN_POINT('Ctrl Pts',(-9.04100976718865E-14,133.962499999475,
-12.7882828778556));
#279463=CARTESIAN_POINT('Ctrl Pts',(-3.75838203887402,134.112499999474,
-11.5671105274575));
#279464=CARTESIAN_POINT('Ctrl Pts',(-7.51676407774795,134.262499999473,
-10.3459381770593));
#279465=CARTESIAN_POINT('Ctrl Pts',(-9.83957192047917,134.412499999473,
-7.14886745759543));
#279466=CARTESIAN_POINT('Ctrl Pts',(-12.1623797632104,134.562499999472,
-3.95179673813153));
#279467=CARTESIAN_POINT('Ctrl Pts',(-12.1623797632104,134.712499999472,
2.97892388940601E-15));
#279468=CARTESIAN_POINT('Ctrl Pts',(-12.1623797632104,134.862499999471,
3.95179673813154));
#279469=CARTESIAN_POINT('Ctrl Pts',(-9.83957192047916,135.01249999947,7.14886745759543));
#279470=CARTESIAN_POINT('Ctrl Pts',(-7.51676407774795,135.16249999947,10.3459381770593));
#279471=CARTESIAN_POINT('Ctrl Pts',(-3.75838203887402,135.312499999469,
11.5671105274575));
#279472=CARTESIAN_POINT('Ctrl Pts',(-8.8141726369126E-14,135.462499999469,
12.7882828778556));
#279473=CARTESIAN_POINT('Ctrl Pts',(3.75838203887384,135.612499999468,11.5671105274575));
#279474=CARTESIAN_POINT('Ctrl Pts',(7.51676407774777,135.762499999467,10.3459381770593));
#279475=CARTESIAN_POINT('Ctrl Pts',(9.83957192047898,135.912499999467,7.14886745759543));
#279476=CARTESIAN_POINT('Ctrl Pts',(12.1623797632102,136.062499999466,3.95179673813153));
#279477=CARTESIAN_POINT('Ctrl Pts',(12.1623797632102,136.212499999466,-1.489461944703E-15));
#279478=CARTESIAN_POINT('Ctrl Pts',(12.1623797632102,136.362499999465,-3.95179673813154));
#279479=CARTESIAN_POINT('Ctrl Pts',(9.83957192047898,136.512499999464,-7.14886745759543));
#279480=CARTESIAN_POINT('Ctrl Pts',(7.51676407774776,136.662499999464,-10.3459381770593));
#279481=CARTESIAN_POINT('Ctrl Pts',(3.75838203887384,136.812499999463,-11.5671105274575));
#279482=CARTESIAN_POINT('Ctrl Pts',(-9.21378069435483E-14,136.962499999463,
-12.7882828778556));
#279483=CARTESIAN_POINT('Ctrl Pts',(-3.75838203887402,137.112499999462,
-11.5671105274575));
#279484=CARTESIAN_POINT('Ctrl Pts',(-7.51676407774795,137.262499999461,
-10.3459381770593));
#279485=CARTESIAN_POINT('Ctrl Pts',(-9.83957192047917,137.412499999461,
-7.14886745759543));
#279486=CARTESIAN_POINT('Ctrl Pts',(-12.1623797632104,137.56249999946,-3.95179673813153));
#279487=CARTESIAN_POINT('Ctrl Pts',(-12.1623797632104,137.71249999946,2.97892388940601E-15));
#279488=CARTESIAN_POINT('Ctrl Pts',(-12.1623797632104,137.862499999459,
3.95179673813154));
#279489=CARTESIAN_POINT('Ctrl Pts',(-9.83957192047917,138.012499999458,
7.14886745759543));
#279490=CARTESIAN_POINT('Ctrl Pts',(-7.51676407774795,138.162499999458,
10.3459381770593));
#279491=CARTESIAN_POINT('Ctrl Pts',(-3.75838203887402,138.312499999457,
11.5671105274575));
#279492=CARTESIAN_POINT('Ctrl Pts',(-8.98694356407879E-14,138.462499999457,
12.7882828778556));
#279493=CARTESIAN_POINT('Ctrl Pts',(3.75838203887384,138.612499999456,11.5671105274575));
#279494=CARTESIAN_POINT('Ctrl Pts',(7.51676407774777,138.762499999455,10.3459381770593));
#279495=CARTESIAN_POINT('Ctrl Pts',(9.83957192047898,138.912499999455,7.14886745759543));
#279496=CARTESIAN_POINT('Ctrl Pts',(12.1623797632102,139.062499999454,3.95179673813153));
#279497=CARTESIAN_POINT('Ctrl Pts',(12.1623797632102,139.212499999454,-1.489461944703E-15));
#279498=CARTESIAN_POINT('Ctrl Pts',(12.1623797632102,139.362499999453,-3.95179673813154));
#279499=CARTESIAN_POINT('Ctrl Pts',(9.83957192047898,139.512499999452,-7.14886745759543));
#279500=CARTESIAN_POINT('Ctrl Pts',(7.51676407774776,139.662499999452,-10.3459381770593));
#279501=CARTESIAN_POINT('Ctrl Pts',(3.75838203887384,139.812499999451,-11.5671105274575));
#279502=CARTESIAN_POINT('Ctrl Pts',(-9.38655162152102E-14,139.962499999451,
-12.7882828778556));
#279503=CARTESIAN_POINT('Ctrl Pts',(-3.75838203887402,140.11249999945,-11.5671105274575));
#279504=CARTESIAN_POINT('Ctrl Pts',(-7.51676407774795,140.262499999449,
-10.3459381770593));
#279505=CARTESIAN_POINT('Ctrl Pts',(-9.83957192047917,140.412499999449,
-7.14886745759543));
#279506=CARTESIAN_POINT('Ctrl Pts',(-12.1623797632104,140.562499999448,
-3.95179673813153));
#279507=CARTESIAN_POINT('Ctrl Pts',(-12.1623797632104,140.712499999448,
2.97892388940601E-15));
#279508=CARTESIAN_POINT('Ctrl Pts',(-12.1623797632104,140.862499999447,
3.95179673813154));
#279509=CARTESIAN_POINT('Ctrl Pts',(-9.83957192047917,141.012499999446,
7.14886745759543));
#279510=CARTESIAN_POINT('Ctrl Pts',(-7.51676407774795,141.162499999446,
10.3459381770593));
#279511=CARTESIAN_POINT('Ctrl Pts',(-3.75838203887402,141.312499999445,
11.5671105274575));
#279512=CARTESIAN_POINT('Ctrl Pts',(-9.15971449124498E-14,141.462499999445,
12.7882828778556));
#279513=CARTESIAN_POINT('Ctrl Pts',(3.75838203887384,141.612499999444,11.5671105274575));
#279514=CARTESIAN_POINT('Ctrl Pts',(7.51676407774776,141.762499999443,10.3459381770593));
#279515=CARTESIAN_POINT('Ctrl Pts',(9.83957192047898,141.912499999443,7.14886745759543));
#279516=CARTESIAN_POINT('Ctrl Pts',(12.1623797632102,142.062499999442,3.95179673813153));
#279517=CARTESIAN_POINT('Ctrl Pts',(12.1623797632102,142.212499999442,-1.489461944703E-15));
#279518=CARTESIAN_POINT('Ctrl Pts',(12.1623797632102,142.362499999441,-3.95179673813154));
#279519=CARTESIAN_POINT('Ctrl Pts',(9.83957192047898,142.51249999944,-7.14886745759543));
#279520=CARTESIAN_POINT('Ctrl Pts',(7.51676407774776,142.66249999944,-10.3459381770593));
#279521=CARTESIAN_POINT('Ctrl Pts',(3.75838203887383,142.812499999439,-11.5671105274575));
#279522=CARTESIAN_POINT('Ctrl Pts',(-9.5593225486872E-14,142.962499999439,
-12.7882828778556));
#279523=CARTESIAN_POINT('Ctrl Pts',(-3.75838203887402,143.112499999438,
-11.5671105274575));
#279524=CARTESIAN_POINT('Ctrl Pts',(-7.51676407774795,143.262499999437,
-10.3459381770593));
#279525=CARTESIAN_POINT('Ctrl Pts',(-9.83957192047917,143.412499999437,
-7.14886745759543));
#279526=CARTESIAN_POINT('Ctrl Pts',(-12.1623797632104,143.562499999436,
-3.95179673813153));
#279527=CARTESIAN_POINT('Ctrl Pts',(-12.1623797632104,143.712499999436,
2.97892388940601E-15));
#279528=CARTESIAN_POINT('Ctrl Pts',(-12.1623797632104,143.862499999435,
3.95179673813154));
#279529=CARTESIAN_POINT('Ctrl Pts',(-9.83957192047917,144.012499999434,
7.14886745759543));
#279530=CARTESIAN_POINT('Ctrl Pts',(-7.51676407774795,144.162499999434,
10.3459381770593));
#279531=CARTESIAN_POINT('Ctrl Pts',(-3.75838203887402,144.312499999433,
11.5671105274575));
#279532=CARTESIAN_POINT('Ctrl Pts',(-9.33248541841116E-14,144.462499999433,
12.7882828778556));
#279533=CARTESIAN_POINT('Ctrl Pts',(3.75838203887384,144.612499999432,11.5671105274575));
#279534=CARTESIAN_POINT('Ctrl Pts',(7.51676407774776,144.762499999431,10.3459381770593));
#279535=CARTESIAN_POINT('Ctrl Pts',(9.83957192047898,144.912499999431,7.14886745759543));
#279536=CARTESIAN_POINT('Ctrl Pts',(12.1623797632102,145.06249999943,3.95179673813153));
#279537=CARTESIAN_POINT('Ctrl Pts',(12.1623797632102,145.21249999943,-1.489461944703E-15));
#279538=CARTESIAN_POINT('Ctrl Pts',(12.1623797632102,145.362499999429,-3.95179673813154));
#279539=CARTESIAN_POINT('Ctrl Pts',(9.83957192047898,145.512499999428,-7.14886745759543));
#279540=CARTESIAN_POINT('Ctrl Pts',(7.51676407774776,145.662499999428,-10.3459381770593));
#279541=CARTESIAN_POINT('Ctrl Pts',(3.75838203887383,145.812499999427,-11.5671105274575));
#279542=CARTESIAN_POINT('Ctrl Pts',(-9.73209347585338E-14,145.962499999427,
-12.7882828778556));
#279543=CARTESIAN_POINT('Ctrl Pts',(-3.75838203887403,146.112499999426,
-11.5671105274575));
#279544=CARTESIAN_POINT('Ctrl Pts',(-7.51676407774795,146.262499999425,
-10.3459381770593));
#279545=CARTESIAN_POINT('Ctrl Pts',(-9.83957192047917,146.412499999425,
-7.14886745759543));
#279546=CARTESIAN_POINT('Ctrl Pts',(-12.1623797632104,146.562499999424,
-3.95179673813153));
#279547=CARTESIAN_POINT('Ctrl Pts',(-12.1623797632104,146.712499999424,
2.97892388940601E-15));
#279548=CARTESIAN_POINT('Ctrl Pts',(-12.1623797632104,146.862499999423,
3.95179673813154));
#279549=CARTESIAN_POINT('Ctrl Pts',(-9.83957192047917,147.012499999422,
7.14886745759543));
#279550=CARTESIAN_POINT('Ctrl Pts',(-7.51676407774795,147.162499999422,
10.3459381770593));
#279551=CARTESIAN_POINT('Ctrl Pts',(-3.75838203887402,147.312499999421,
11.5671105274575));
#279552=CARTESIAN_POINT('Ctrl Pts',(-9.50525634557734E-14,147.462499999421,
12.7882828778556));
#279553=CARTESIAN_POINT('Ctrl Pts',(3.75838203887383,147.61249999942,11.5671105274575));
#279554=CARTESIAN_POINT('Ctrl Pts',(7.51676407774776,147.762499999419,10.3459381770593));
#279555=CARTESIAN_POINT('Ctrl Pts',(9.83957192047898,147.912499999419,7.14886745759543));
#279556=CARTESIAN_POINT('Ctrl Pts',(12.1623797632102,148.062499999418,3.95179673813153));
#279557=CARTESIAN_POINT('Ctrl Pts',(12.1623797632102,148.212499999418,-1.489461944703E-15));
#279558=CARTESIAN_POINT('Ctrl Pts',(12.1623797632102,148.362499999417,-3.95179673813154));
#279559=CARTESIAN_POINT('Ctrl Pts',(9.83957192047898,148.512499999416,-7.14886745759543));
#279560=CARTESIAN_POINT('Ctrl Pts',(7.51676407774776,148.662499999416,-10.3459381770593));
#279561=CARTESIAN_POINT('Ctrl Pts',(3.75838203887383,148.812499999415,-11.5671105274575));
#279562=CARTESIAN_POINT('Ctrl Pts',(-9.90486440301957E-14,148.962499999415,
-12.7882828778556));
#279563=CARTESIAN_POINT('Ctrl Pts',(-3.75838203887403,149.112499999414,
-11.5671105274575));
#279564=CARTESIAN_POINT('Ctrl Pts',(-7.51676407774795,149.262499999413,
-10.3459381770593));
#279565=CARTESIAN_POINT('Ctrl Pts',(-9.83957192047917,149.412499999413,
-7.14886745759543));
#279566=CARTESIAN_POINT('Ctrl Pts',(-12.1623797632104,149.562499999412,
-3.95179673813153));
#279567=CARTESIAN_POINT('Ctrl Pts',(-12.1623797632104,149.712499999412,
2.97892388940601E-15));
#279568=CARTESIAN_POINT('Ctrl Pts',(-12.1623797632104,149.862499999411,
3.95179673813154));
#279569=CARTESIAN_POINT('Ctrl Pts',(-9.83957192047917,150.01249999941,7.14886745759543));
#279570=CARTESIAN_POINT('Ctrl Pts',(-7.51676407774795,150.16249999941,10.3459381770593));
#279571=CARTESIAN_POINT('Ctrl Pts',(-3.75838203887403,150.312499999409,
11.5671105274575));
#279572=CARTESIAN_POINT('Ctrl Pts',(-9.67802727274353E-14,150.462499999409,
12.7882828778556));
#279573=CARTESIAN_POINT('Ctrl Pts',(3.75838203887383,150.612499999408,11.5671105274575));
#279574=CARTESIAN_POINT('Ctrl Pts',(7.51676407774776,150.762499999407,10.3459381770593));
#279575=CARTESIAN_POINT('Ctrl Pts',(9.83957192047898,150.912499999407,7.14886745759543));
#279576=CARTESIAN_POINT('Ctrl Pts',(12.1623797632102,151.062499999406,3.95179673813153));
#279577=CARTESIAN_POINT('Ctrl Pts',(12.1623797632102,151.212499999406,-1.489461944703E-15));
#279578=CARTESIAN_POINT('Ctrl Pts',(12.1623797632102,151.362499999405,-3.95179673813154));
#279579=CARTESIAN_POINT('Ctrl Pts',(9.83957192047897,151.512499999404,-7.14886745759543));
#279580=CARTESIAN_POINT('Ctrl Pts',(7.51676407774776,151.662499999404,-10.3459381770593));
#279581=CARTESIAN_POINT('Ctrl Pts',(3.75838203887383,151.812499999403,-11.5671105274575));
#279582=CARTESIAN_POINT('Ctrl Pts',(-1.00776353301858E-13,151.962499999403,
-12.7882828778556));
#279583=CARTESIAN_POINT('Ctrl Pts',(-3.75838203887403,152.112499999402,
-11.5671105274575));
#279584=CARTESIAN_POINT('Ctrl Pts',(-10.0514278971316,-2.0687413718495,
2.46188980021652E-15));
#279585=CARTESIAN_POINT('Ctrl Pts',(-10.0514278971316,-1.9187413718501,
3.26590689904296));
#279586=CARTESIAN_POINT('Ctrl Pts',(-8.13177598651391,-1.7687413718507,
5.9080810824151));
#279587=CARTESIAN_POINT('Ctrl Pts',(-6.21212407589621,-1.61874137185129,
8.55025526578723));
#279588=CARTESIAN_POINT('Ctrl Pts',(-3.10606203794811,-1.46874137185189,
9.55947599963789));
#279589=CARTESIAN_POINT('Ctrl Pts',(-9.77671809333146E-15,-1.31874137185249,
10.5686967334885));
#279590=CARTESIAN_POINT('Ctrl Pts',(3.10606203794809,-1.16874137185309,
9.55947599963789));
#279591=CARTESIAN_POINT('Ctrl Pts',(6.21212407589619,-1.01874137185369,
8.55025526578723));
#279592=CARTESIAN_POINT('Ctrl Pts',(8.13177598651388,-0.868741371854286,
5.90808108241509));
#279593=CARTESIAN_POINT('Ctrl Pts',(10.0514278971316,-0.718741371854885,
3.26590689904295));
#279594=CARTESIAN_POINT('Ctrl Pts',(10.0514278971316,-0.568741371855485,
-1.23094490010826E-15));
#279595=CARTESIAN_POINT('Ctrl Pts',(10.0514278971316,-0.418741371856085,
-3.26590689904296));
#279596=CARTESIAN_POINT('Ctrl Pts',(8.13177598651388,-0.268741371856686,
-5.9080810824151));
#279597=CARTESIAN_POINT('Ctrl Pts',(6.21212407589619,-0.118741371857287,
-8.55025526578723));
#279598=CARTESIAN_POINT('Ctrl Pts',(3.10606203794809,0.0312586281421111,
-9.55947599963789));
#279599=CARTESIAN_POINT('Ctrl Pts',(-1.32291568543275E-14,0.181258628141509,
-10.5686967334885));
#279600=CARTESIAN_POINT('Ctrl Pts',(-3.10606203794812,0.331258628140907,
-9.55947599963789));
#279601=CARTESIAN_POINT('Ctrl Pts',(-6.21212407589621,0.481258628140306,
-8.55025526578723));
#279602=CARTESIAN_POINT('Ctrl Pts',(-8.13177598651391,0.631258628139705,
-5.90808108241509));
#279603=CARTESIAN_POINT('Ctrl Pts',(-10.0514278971316,0.781258628139103,
-3.26590689904296));
#279604=CARTESIAN_POINT('Ctrl Pts',(-10.0514278971316,0.931258628138503,
2.46188980021652E-15));
#279605=CARTESIAN_POINT('Ctrl Pts',(-10.0514278971316,1.0812586281379,3.26590689904296));
#279606=CARTESIAN_POINT('Ctrl Pts',(-8.13177598651391,1.2312586281373,5.9080810824151));
#279607=CARTESIAN_POINT('Ctrl Pts',(-6.21212407589621,1.38125862813671,
8.55025526578723));
#279608=CARTESIAN_POINT('Ctrl Pts',(-3.10606203794811,1.53125862813611,
9.55947599963789));
#279609=CARTESIAN_POINT('Ctrl Pts',(-1.15044273649933E-14,1.68125862813551,
10.5686967334885));
#279610=CARTESIAN_POINT('Ctrl Pts',(3.10606203794809,1.83125862813491,9.55947599963789));
#279611=CARTESIAN_POINT('Ctrl Pts',(6.21212407589619,1.98125862813431,8.55025526578723));
#279612=CARTESIAN_POINT('Ctrl Pts',(8.13177598651388,2.13125862813371,5.90808108241509));
#279613=CARTESIAN_POINT('Ctrl Pts',(10.0514278971316,2.28125862813311,3.26590689904295));
#279614=CARTESIAN_POINT('Ctrl Pts',(10.0514278971316,2.43125862813252,-1.23094490010826E-15));
#279615=CARTESIAN_POINT('Ctrl Pts',(10.0514278971316,2.58125862813192,-3.26590689904296));
#279616=CARTESIAN_POINT('Ctrl Pts',(8.13177598651388,2.73125862813131,-5.9080810824151));
#279617=CARTESIAN_POINT('Ctrl Pts',(6.21212407589619,2.88125862813071,-8.55025526578723));
#279618=CARTESIAN_POINT('Ctrl Pts',(3.10606203794809,3.03125862813011,-9.55947599963789));
#279619=CARTESIAN_POINT('Ctrl Pts',(-1.49568661259894E-14,3.18125862812951,
-10.5686967334885));
#279620=CARTESIAN_POINT('Ctrl Pts',(-3.10606203794812,3.33125862812891,
-9.55947599963789));
#279621=CARTESIAN_POINT('Ctrl Pts',(-6.21212407589622,3.48125862812831,
-8.55025526578723));
#279622=CARTESIAN_POINT('Ctrl Pts',(-8.13177598651391,3.6312586281277,-5.90808108241509));
#279623=CARTESIAN_POINT('Ctrl Pts',(-10.0514278971316,3.7812586281271,-3.26590689904296));
#279624=CARTESIAN_POINT('Ctrl Pts',(-10.0514278971316,3.9312586281265,2.46188980021652E-15));
#279625=CARTESIAN_POINT('Ctrl Pts',(-10.0514278971316,4.0812586281259,3.26590689904296));
#279626=CARTESIAN_POINT('Ctrl Pts',(-8.13177598651391,4.2312586281253,5.9080810824151));
#279627=CARTESIAN_POINT('Ctrl Pts',(-6.21212407589621,4.38125862812471,
8.55025526578723));
#279628=CARTESIAN_POINT('Ctrl Pts',(-3.10606203794812,4.53125862812411,
9.55947599963789));
#279629=CARTESIAN_POINT('Ctrl Pts',(-1.32321366366551E-14,4.68125862812351,
10.5686967334885));
#279630=CARTESIAN_POINT('Ctrl Pts',(3.10606203794809,4.83125862812291,9.55947599963789));
#279631=CARTESIAN_POINT('Ctrl Pts',(6.21212407589619,4.98125862812231,8.55025526578723));
#279632=CARTESIAN_POINT('Ctrl Pts',(8.13177598651388,5.13125862812171,5.90808108241509));
#279633=CARTESIAN_POINT('Ctrl Pts',(10.0514278971316,5.28125862812112,3.26590689904295));
#279634=CARTESIAN_POINT('Ctrl Pts',(10.0514278971316,5.43125862812051,-1.23094490010826E-15));
#279635=CARTESIAN_POINT('Ctrl Pts',(10.0514278971316,5.58125862811991,-3.26590689904296));
#279636=CARTESIAN_POINT('Ctrl Pts',(8.13177598651388,5.73125862811931,-5.9080810824151));
#279637=CARTESIAN_POINT('Ctrl Pts',(6.21212407589619,5.88125862811871,-8.55025526578723));
#279638=CARTESIAN_POINT('Ctrl Pts',(3.10606203794809,6.03125862811811,-9.55947599963789));
#279639=CARTESIAN_POINT('Ctrl Pts',(-1.66845753976512E-14,6.18125862811751,
-10.5686967334885));
#279640=CARTESIAN_POINT('Ctrl Pts',(-3.10606203794812,6.33125862811691,
-9.55947599963789));
#279641=CARTESIAN_POINT('Ctrl Pts',(-6.21212407589622,6.48125862811631,
-8.55025526578723));
#279642=CARTESIAN_POINT('Ctrl Pts',(-8.13177598651391,6.63125862811571,
-5.90808108241509));
#279643=CARTESIAN_POINT('Ctrl Pts',(-10.0514278971316,6.7812586281151,-3.26590689904296));
#279644=CARTESIAN_POINT('Ctrl Pts',(-10.0514278971316,6.9312586281145,2.46188980021652E-15));
#279645=CARTESIAN_POINT('Ctrl Pts',(-10.0514278971316,7.0812586281139,3.26590689904296));
#279646=CARTESIAN_POINT('Ctrl Pts',(-8.13177598651391,7.2312586281133,5.9080810824151));
#279647=CARTESIAN_POINT('Ctrl Pts',(-6.21212407589622,7.38125862811271,
8.55025526578723));
#279648=CARTESIAN_POINT('Ctrl Pts',(-3.10606203794812,7.53125862811211,
9.55947599963789));
#279649=CARTESIAN_POINT('Ctrl Pts',(-1.4959845908317E-14,7.68125862811151,
10.5686967334885));
#279650=CARTESIAN_POINT('Ctrl Pts',(3.10606203794809,7.83125862811091,9.55947599963789));
#279651=CARTESIAN_POINT('Ctrl Pts',(6.21212407589619,7.98125862811031,8.55025526578723));
#279652=CARTESIAN_POINT('Ctrl Pts',(8.13177598651388,8.13125862810971,5.90808108241509));
#279653=CARTESIAN_POINT('Ctrl Pts',(10.0514278971316,8.28125862810912,3.26590689904295));
#279654=CARTESIAN_POINT('Ctrl Pts',(10.0514278971316,8.43125862810852,-1.23094490010826E-15));
#279655=CARTESIAN_POINT('Ctrl Pts',(10.0514278971316,8.58125862810792,-3.26590689904296));
#279656=CARTESIAN_POINT('Ctrl Pts',(8.13177598651388,8.73125862810731,-5.9080810824151));
#279657=CARTESIAN_POINT('Ctrl Pts',(6.21212407589618,8.88125862810671,-8.55025526578723));
#279658=CARTESIAN_POINT('Ctrl Pts',(3.10606203794808,9.03125862810611,-9.55947599963789));
#279659=CARTESIAN_POINT('Ctrl Pts',(-1.84122846693131E-14,9.18125862810551,
-10.5686967334885));
#279660=CARTESIAN_POINT('Ctrl Pts',(-3.10606203794812,9.33125862810491,
-9.55947599963789));
#279661=CARTESIAN_POINT('Ctrl Pts',(-6.21212407589622,9.48125862810431,
-8.55025526578723));
#279662=CARTESIAN_POINT('Ctrl Pts',(-8.13177598651391,9.6312586281037,-5.90808108241509));
#279663=CARTESIAN_POINT('Ctrl Pts',(-10.0514278971316,9.7812586281031,-3.26590689904296));
#279664=CARTESIAN_POINT('Ctrl Pts',(-10.0514278971316,9.9312586281025,2.46188980021652E-15));
#279665=CARTESIAN_POINT('Ctrl Pts',(-10.0514278971316,10.0812586281019,
3.26590689904296));
#279666=CARTESIAN_POINT('Ctrl Pts',(-8.13177598651391,10.2312586281013,
5.9080810824151));
#279667=CARTESIAN_POINT('Ctrl Pts',(-6.21212407589622,10.3812586281007,
8.55025526578723));
#279668=CARTESIAN_POINT('Ctrl Pts',(-3.10606203794812,10.5312586281001,
9.55947599963789));
#279669=CARTESIAN_POINT('Ctrl Pts',(-1.66875551799788E-14,10.6812586280995,
10.5686967334885));
#279670=CARTESIAN_POINT('Ctrl Pts',(3.10606203794808,10.8312586280989,9.55947599963789));
#279671=CARTESIAN_POINT('Ctrl Pts',(6.21212407589618,10.9812586280983,8.55025526578723));
#279672=CARTESIAN_POINT('Ctrl Pts',(8.13177598651388,11.1312586280977,5.90808108241509));
#279673=CARTESIAN_POINT('Ctrl Pts',(10.0514278971316,11.2812586280971,3.26590689904295));
#279674=CARTESIAN_POINT('Ctrl Pts',(10.0514278971316,11.4312586280965,-1.23094490010826E-15));
#279675=CARTESIAN_POINT('Ctrl Pts',(10.0514278971316,11.5812586280959,-3.26590689904296));
#279676=CARTESIAN_POINT('Ctrl Pts',(8.13177598651387,11.7312586280953,-5.9080810824151));
#279677=CARTESIAN_POINT('Ctrl Pts',(6.21212407589618,11.8812586280947,-8.55025526578723));
#279678=CARTESIAN_POINT('Ctrl Pts',(3.10606203794808,12.0312586280941,-9.55947599963789));
#279679=CARTESIAN_POINT('Ctrl Pts',(-2.01399939409749E-14,12.1812586280935,
-10.5686967334885));
#279680=CARTESIAN_POINT('Ctrl Pts',(-3.10606203794812,12.3312586280929,
-9.55947599963789));
#279681=CARTESIAN_POINT('Ctrl Pts',(-6.21212407589622,12.4812586280923,
-8.55025526578723));
#279682=CARTESIAN_POINT('Ctrl Pts',(-8.13177598651392,12.6312586280917,
-5.90808108241509));
#279683=CARTESIAN_POINT('Ctrl Pts',(-10.0514278971316,12.7812586280911,
-3.26590689904296));
#279684=CARTESIAN_POINT('Ctrl Pts',(-10.0514278971316,12.9312586280905,
2.46188980021652E-15));
#279685=CARTESIAN_POINT('Ctrl Pts',(-10.0514278971316,13.0812586280899,
3.26590689904296));
#279686=CARTESIAN_POINT('Ctrl Pts',(-8.13177598651392,13.2312586280893,
5.9080810824151));
#279687=CARTESIAN_POINT('Ctrl Pts',(-6.21212407589622,13.3812586280887,
8.55025526578723));
#279688=CARTESIAN_POINT('Ctrl Pts',(-3.10606203794812,13.5312586280881,
9.55947599963789));
#279689=CARTESIAN_POINT('Ctrl Pts',(-1.84152644516406E-14,13.6812586280875,
10.5686967334885));
#279690=CARTESIAN_POINT('Ctrl Pts',(3.10606203794808,13.8312586280869,9.55947599963789));
#279691=CARTESIAN_POINT('Ctrl Pts',(6.21212407589618,13.9812586280863,8.55025526578723));
#279692=CARTESIAN_POINT('Ctrl Pts',(8.13177598651387,14.1312586280857,5.90808108241509));
#279693=CARTESIAN_POINT('Ctrl Pts',(10.0514278971316,14.2812586280851,3.26590689904295));
#279694=CARTESIAN_POINT('Ctrl Pts',(10.0514278971316,14.4312586280845,-1.23094490010826E-15));
#279695=CARTESIAN_POINT('Ctrl Pts',(10.0514278971316,14.5812586280839,-3.26590689904296));
#279696=CARTESIAN_POINT('Ctrl Pts',(8.13177598651387,14.7312586280833,-5.9080810824151));
#279697=CARTESIAN_POINT('Ctrl Pts',(6.21212407589618,14.8812586280827,-8.55025526578723));
#279698=CARTESIAN_POINT('Ctrl Pts',(3.10606203794808,15.0312586280821,-9.55947599963789));
#279699=CARTESIAN_POINT('Ctrl Pts',(-2.18677032126367E-14,15.1812586280815,
-10.5686967334885));
#279700=CARTESIAN_POINT('Ctrl Pts',(-3.10606203794812,15.3312586280809,
-9.55947599963789));
#279701=CARTESIAN_POINT('Ctrl Pts',(-6.21212407589623,15.4812586280803,
-8.55025526578723));
#279702=CARTESIAN_POINT('Ctrl Pts',(-8.13177598651392,15.6312586280797,
-5.90808108241509));
#279703=CARTESIAN_POINT('Ctrl Pts',(-10.0514278971316,15.7812586280791,
-3.26590689904296));
#279704=CARTESIAN_POINT('Ctrl Pts',(-10.0514278971316,15.9312586280785,
2.46188980021652E-15));
#279705=CARTESIAN_POINT('Ctrl Pts',(-10.0514278971316,16.0812586280779,
3.26590689904296));
#279706=CARTESIAN_POINT('Ctrl Pts',(-8.13177598651392,16.2312586280773,
5.9080810824151));
#279707=CARTESIAN_POINT('Ctrl Pts',(-6.21212407589622,16.3812586280767,
8.55025526578723));
#279708=CARTESIAN_POINT('Ctrl Pts',(-3.10606203794812,16.5312586280761,
9.55947599963789));
#279709=CARTESIAN_POINT('Ctrl Pts',(-2.01429737233025E-14,16.6812586280755,
10.5686967334885));
#279710=CARTESIAN_POINT('Ctrl Pts',(3.10606203794808,16.8312586280749,9.55947599963789));
#279711=CARTESIAN_POINT('Ctrl Pts',(6.21212407589618,16.9812586280743,8.55025526578723));
#279712=CARTESIAN_POINT('Ctrl Pts',(8.13177598651387,17.1312586280737,5.90808108241509));
#279713=CARTESIAN_POINT('Ctrl Pts',(10.0514278971316,17.2812586280731,3.26590689904295));
#279714=CARTESIAN_POINT('Ctrl Pts',(10.0514278971316,17.4312586280725,-1.23094490010826E-15));
#279715=CARTESIAN_POINT('Ctrl Pts',(10.0514278971316,17.5812586280719,-3.26590689904296));
#279716=CARTESIAN_POINT('Ctrl Pts',(8.13177598651387,17.7312586280713,-5.9080810824151));
#279717=CARTESIAN_POINT('Ctrl Pts',(6.21212407589618,17.8812586280707,-8.55025526578723));
#279718=CARTESIAN_POINT('Ctrl Pts',(3.10606203794808,18.0312586280701,-9.55947599963789));
#279719=CARTESIAN_POINT('Ctrl Pts',(-2.35954124842986E-14,18.1812586280695,
-10.5686967334885));
#279720=CARTESIAN_POINT('Ctrl Pts',(-3.10606203794813,18.3312586280689,
-9.55947599963789));
#279721=CARTESIAN_POINT('Ctrl Pts',(-6.21212407589623,18.4812586280683,
-8.55025526578723));
#279722=CARTESIAN_POINT('Ctrl Pts',(-8.13177598651392,18.6312586280677,
-5.90808108241509));
#279723=CARTESIAN_POINT('Ctrl Pts',(-10.0514278971316,18.7812586280671,
-3.26590689904296));
#279724=CARTESIAN_POINT('Ctrl Pts',(-10.0514278971316,18.9312586280665,
2.46188980021652E-15));
#279725=CARTESIAN_POINT('Ctrl Pts',(-10.0514278971316,19.0812586280659,
3.26590689904296));
#279726=CARTESIAN_POINT('Ctrl Pts',(-8.13177598651392,19.2312586280653,
5.9080810824151));
#279727=CARTESIAN_POINT('Ctrl Pts',(-6.21212407589623,19.3812586280647,
8.55025526578723));
#279728=CARTESIAN_POINT('Ctrl Pts',(-3.10606203794812,19.5312586280641,
9.55947599963789));
#279729=CARTESIAN_POINT('Ctrl Pts',(-2.18706829949643E-14,19.6812586280635,
10.5686967334885));
#279730=CARTESIAN_POINT('Ctrl Pts',(3.10606203794808,19.8312586280629,9.55947599963789));
#279731=CARTESIAN_POINT('Ctrl Pts',(6.21212407589618,19.9812586280623,8.55025526578723));
#279732=CARTESIAN_POINT('Ctrl Pts',(8.13177598651387,20.1312586280617,5.90808108241509));
#279733=CARTESIAN_POINT('Ctrl Pts',(10.0514278971316,20.2812586280611,3.26590689904295));
#279734=CARTESIAN_POINT('Ctrl Pts',(10.0514278971316,20.4312586280605,-1.23094490010826E-15));
#279735=CARTESIAN_POINT('Ctrl Pts',(10.0514278971316,20.5812586280599,-3.26590689904296));
#279736=CARTESIAN_POINT('Ctrl Pts',(8.13177598651387,20.7312586280593,-5.9080810824151));
#279737=CARTESIAN_POINT('Ctrl Pts',(6.21212407589618,20.8812586280587,-8.55025526578723));
#279738=CARTESIAN_POINT('Ctrl Pts',(3.10606203794808,21.0312586280581,-9.55947599963789));
#279739=CARTESIAN_POINT('Ctrl Pts',(-2.53231217559604E-14,21.1812586280575,
-10.5686967334885));
#279740=CARTESIAN_POINT('Ctrl Pts',(-3.10606203794813,21.3312586280569,
-9.55947599963789));
#279741=CARTESIAN_POINT('Ctrl Pts',(-6.21212407589623,21.4812586280563,
-8.55025526578723));
#279742=CARTESIAN_POINT('Ctrl Pts',(-8.13177598651392,21.6312586280557,
-5.90808108241509));
#279743=CARTESIAN_POINT('Ctrl Pts',(-10.0514278971316,21.7812586280551,
-3.26590689904296));
#279744=CARTESIAN_POINT('Ctrl Pts',(-10.0514278971316,21.9312586280545,
2.46188980021652E-15));
#279745=CARTESIAN_POINT('Ctrl Pts',(-10.0514278971316,22.0812586280539,
3.26590689904296));
#279746=CARTESIAN_POINT('Ctrl Pts',(-8.13177598651392,22.2312586280533,
5.9080810824151));
#279747=CARTESIAN_POINT('Ctrl Pts',(-6.21212407589623,22.3812586280527,
8.55025526578723));
#279748=CARTESIAN_POINT('Ctrl Pts',(-3.10606203794813,22.5312586280521,
9.55947599963789));
#279749=CARTESIAN_POINT('Ctrl Pts',(-2.35983922666262E-14,22.6812586280515,
10.5686967334885));
#279750=CARTESIAN_POINT('Ctrl Pts',(3.10606203794808,22.8312586280509,9.55947599963789));
#279751=CARTESIAN_POINT('Ctrl Pts',(6.21212407589618,22.9812586280503,8.55025526578723));
#279752=CARTESIAN_POINT('Ctrl Pts',(8.13177598651387,23.1312586280497,5.90808108241509));
#279753=CARTESIAN_POINT('Ctrl Pts',(10.0514278971316,23.2812586280491,3.26590689904295));
#279754=CARTESIAN_POINT('Ctrl Pts',(10.0514278971316,23.4312586280485,-1.23094490010826E-15));
#279755=CARTESIAN_POINT('Ctrl Pts',(10.0514278971316,23.5812586280479,-3.26590689904296));
#279756=CARTESIAN_POINT('Ctrl Pts',(8.13177598651387,23.7312586280473,-5.9080810824151));
#279757=CARTESIAN_POINT('Ctrl Pts',(6.21212407589618,23.8812586280467,-8.55025526578723));
#279758=CARTESIAN_POINT('Ctrl Pts',(3.10606203794807,24.0312586280461,-9.55947599963789));
#279759=CARTESIAN_POINT('Ctrl Pts',(-2.70508310276223E-14,24.1812586280455,
-10.5686967334885));
#279760=CARTESIAN_POINT('Ctrl Pts',(-3.10606203794813,24.3312586280449,
-9.55947599963789));
#279761=CARTESIAN_POINT('Ctrl Pts',(-6.21212407589623,24.4812586280443,
-8.55025526578723));
#279762=CARTESIAN_POINT('Ctrl Pts',(-8.13177598651392,24.6312586280437,
-5.90808108241509));
#279763=CARTESIAN_POINT('Ctrl Pts',(-10.0514278971316,24.7812586280431,
-3.26590689904296));
#279764=CARTESIAN_POINT('Ctrl Pts',(-10.0514278971316,24.9312586280425,
2.46188980021652E-15));
#279765=CARTESIAN_POINT('Ctrl Pts',(-10.0514278971316,25.0812586280419,
3.26590689904296));
#279766=CARTESIAN_POINT('Ctrl Pts',(-8.13177598651392,25.2312586280413,
5.9080810824151));
#279767=CARTESIAN_POINT('Ctrl Pts',(-6.21212407589623,25.3812586280407,
8.55025526578723));
#279768=CARTESIAN_POINT('Ctrl Pts',(-3.10606203794813,25.5312586280401,
9.55947599963789));
#279769=CARTESIAN_POINT('Ctrl Pts',(-2.5326101538288E-14,25.6812586280395,
10.5686967334885));
#279770=CARTESIAN_POINT('Ctrl Pts',(3.10606203794808,25.8312586280389,9.55947599963789));
#279771=CARTESIAN_POINT('Ctrl Pts',(6.21212407589618,25.9812586280383,8.55025526578723));
#279772=CARTESIAN_POINT('Ctrl Pts',(8.13177598651387,26.1312586280377,5.90808108241509));
#279773=CARTESIAN_POINT('Ctrl Pts',(10.0514278971316,26.2812586280371,3.26590689904295));
#279774=CARTESIAN_POINT('Ctrl Pts',(10.0514278971316,26.4312586280365,-1.23094490010826E-15));
#279775=CARTESIAN_POINT('Ctrl Pts',(10.0514278971316,26.5812586280359,-3.26590689904296));
#279776=CARTESIAN_POINT('Ctrl Pts',(8.13177598651387,26.7312586280353,-5.9080810824151));
#279777=CARTESIAN_POINT('Ctrl Pts',(6.21212407589617,26.8812586280347,-8.55025526578723));
#279778=CARTESIAN_POINT('Ctrl Pts',(3.10606203794807,27.0312586280341,-9.55947599963789));
#279779=CARTESIAN_POINT('Ctrl Pts',(-2.87785402992841E-14,27.1812586280335,
-10.5686967334885));
#279780=CARTESIAN_POINT('Ctrl Pts',(-3.10606203794813,27.3312586280329,
-9.55947599963789));
#279781=CARTESIAN_POINT('Ctrl Pts',(-6.21212407589623,27.4812586280323,
-8.55025526578723));
#279782=CARTESIAN_POINT('Ctrl Pts',(-8.13177598651393,27.6312586280317,
-5.90808108241509));
#279783=CARTESIAN_POINT('Ctrl Pts',(-10.0514278971316,27.7812586280311,
-3.26590689904296));
#279784=CARTESIAN_POINT('Ctrl Pts',(-10.0514278971316,27.9312586280305,
2.46188980021652E-15));
#279785=CARTESIAN_POINT('Ctrl Pts',(-10.0514278971316,28.0812586280299,
3.26590689904296));
#279786=CARTESIAN_POINT('Ctrl Pts',(-8.13177598651393,28.2312586280293,
5.9080810824151));
#279787=CARTESIAN_POINT('Ctrl Pts',(-6.21212407589623,28.3812586280287,
8.55025526578723));
#279788=CARTESIAN_POINT('Ctrl Pts',(-3.10606203794813,28.5312586280281,
9.55947599963789));
#279789=CARTESIAN_POINT('Ctrl Pts',(-2.70538108099498E-14,28.6812586280275,
10.5686967334885));
#279790=CARTESIAN_POINT('Ctrl Pts',(3.10606203794807,28.8312586280269,9.55947599963789));
#279791=CARTESIAN_POINT('Ctrl Pts',(6.21212407589618,28.9812586280263,8.55025526578723));
#279792=CARTESIAN_POINT('Ctrl Pts',(8.13177598651387,29.1312586280257,5.90808108241509));
#279793=CARTESIAN_POINT('Ctrl Pts',(10.0514278971316,29.2812586280251,3.26590689904295));
#279794=CARTESIAN_POINT('Ctrl Pts',(10.0514278971316,29.4312586280245,-1.23094490010826E-15));
#279795=CARTESIAN_POINT('Ctrl Pts',(10.0514278971316,29.5812586280239,-3.26590689904296));
#279796=CARTESIAN_POINT('Ctrl Pts',(8.13177598651386,29.7312586280233,-5.9080810824151));
#279797=CARTESIAN_POINT('Ctrl Pts',(6.21212407589617,29.8812586280227,-8.55025526578723));
#279798=CARTESIAN_POINT('Ctrl Pts',(3.10606203794807,30.0312586280221,-9.55947599963789));
#279799=CARTESIAN_POINT('Ctrl Pts',(-3.05062495709459E-14,30.1812586280215,
-10.5686967334885));
#279800=CARTESIAN_POINT('Ctrl Pts',(-3.10606203794813,30.3312586280209,
-9.55947599963789));
#279801=CARTESIAN_POINT('Ctrl Pts',(-6.21212407589623,30.4812586280203,
-8.55025526578723));
#279802=CARTESIAN_POINT('Ctrl Pts',(-8.13177598651393,30.6312586280197,
-5.90808108241509));
#279803=CARTESIAN_POINT('Ctrl Pts',(-10.0514278971316,30.7812586280191,
-3.26590689904296));
#279804=CARTESIAN_POINT('Ctrl Pts',(-10.0514278971316,30.9312586280185,
2.46188980021652E-15));
#279805=CARTESIAN_POINT('Ctrl Pts',(-10.0514278971316,31.0812586280179,
3.26590689904296));
#279806=CARTESIAN_POINT('Ctrl Pts',(-8.13177598651393,31.2312586280173,
5.9080810824151));
#279807=CARTESIAN_POINT('Ctrl Pts',(-6.21212407589623,31.3812586280167,
8.55025526578723));
#279808=CARTESIAN_POINT('Ctrl Pts',(-3.10606203794813,31.5312586280161,
9.55947599963789));
#279809=CARTESIAN_POINT('Ctrl Pts',(-2.87815200816117E-14,31.6812586280155,
10.5686967334885));
#279810=CARTESIAN_POINT('Ctrl Pts',(3.10606203794807,31.8312586280149,9.55947599963789));
#279811=CARTESIAN_POINT('Ctrl Pts',(6.21212407589617,31.9812586280143,8.55025526578723));
#279812=CARTESIAN_POINT('Ctrl Pts',(8.13177598651386,32.1312586280137,5.90808108241509));
#279813=CARTESIAN_POINT('Ctrl Pts',(10.0514278971316,32.2812586280131,3.26590689904295));
#279814=CARTESIAN_POINT('Ctrl Pts',(10.0514278971316,32.4312586280125,-1.23094490010826E-15));
#279815=CARTESIAN_POINT('Ctrl Pts',(10.0514278971316,32.5812586280119,-3.26590689904296));
#279816=CARTESIAN_POINT('Ctrl Pts',(8.13177598651386,32.7312586280113,-5.9080810824151));
#279817=CARTESIAN_POINT('Ctrl Pts',(6.21212407589617,32.8812586280107,-8.55025526578723));
#279818=CARTESIAN_POINT('Ctrl Pts',(3.10606203794807,33.0312586280101,-9.55947599963789));
#279819=CARTESIAN_POINT('Ctrl Pts',(-3.22339588426078E-14,33.1812586280095,
-10.5686967334885));
#279820=CARTESIAN_POINT('Ctrl Pts',(-3.10606203794813,33.3312586280089,
-9.55947599963789));
#279821=CARTESIAN_POINT('Ctrl Pts',(-6.21212407589623,33.4812586280083,
-8.55025526578723));
#279822=CARTESIAN_POINT('Ctrl Pts',(-8.13177598651393,33.6312586280077,
-5.90808108241509));
#279823=CARTESIAN_POINT('Ctrl Pts',(-10.0514278971316,33.7812586280071,
-3.26590689904296));
#279824=CARTESIAN_POINT('Ctrl Pts',(-10.0514278971316,33.9312586280065,
2.46188980021652E-15));
#279825=CARTESIAN_POINT('Ctrl Pts',(-10.0514278971316,34.0812586280059,
3.26590689904296));
#279826=CARTESIAN_POINT('Ctrl Pts',(-8.13177598651393,34.2312586280053,
5.9080810824151));
#279827=CARTESIAN_POINT('Ctrl Pts',(-6.21212407589623,34.3812586280047,
8.55025526578723));
#279828=CARTESIAN_POINT('Ctrl Pts',(-3.10606203794813,34.5312586280041,
9.55947599963789));
#279829=CARTESIAN_POINT('Ctrl Pts',(-3.05092293532735E-14,34.6812586280035,
10.5686967334885));
#279830=CARTESIAN_POINT('Ctrl Pts',(3.10606203794807,34.8312586280029,9.55947599963789));
#279831=CARTESIAN_POINT('Ctrl Pts',(6.21212407589617,34.9812586280023,8.55025526578723));
#279832=CARTESIAN_POINT('Ctrl Pts',(8.13177598651386,35.1312586280017,5.90808108241509));
#279833=CARTESIAN_POINT('Ctrl Pts',(10.0514278971316,35.2812586280011,3.26590689904295));
#279834=CARTESIAN_POINT('Ctrl Pts',(10.0514278971316,35.4312586280005,-1.23094490010826E-15));
#279835=CARTESIAN_POINT('Ctrl Pts',(10.0514278971315,35.5812586279999,-3.26590689904296));
#279836=CARTESIAN_POINT('Ctrl Pts',(8.13177598651386,35.7312586279993,-5.9080810824151));
#279837=CARTESIAN_POINT('Ctrl Pts',(6.21212407589617,35.8812586279987,-8.55025526578723));
#279838=CARTESIAN_POINT('Ctrl Pts',(3.10606203794807,36.0312586279981,-9.55947599963789));
#279839=CARTESIAN_POINT('Ctrl Pts',(-3.39616681142696E-14,36.1812586279975,
-10.5686967334885));
#279840=CARTESIAN_POINT('Ctrl Pts',(-3.10606203794814,36.3312586279969,
-9.55947599963789));
#279841=CARTESIAN_POINT('Ctrl Pts',(-6.21212407589624,36.4812586279963,
-8.55025526578723));
#279842=CARTESIAN_POINT('Ctrl Pts',(-8.13177598651393,36.6312586279957,
-5.90808108241509));
#279843=CARTESIAN_POINT('Ctrl Pts',(-10.0514278971316,36.7812586279951,
-3.26590689904296));
#279844=CARTESIAN_POINT('Ctrl Pts',(-10.0514278971316,36.9312586279945,
2.46188980021652E-15));
#279845=CARTESIAN_POINT('Ctrl Pts',(-10.0514278971316,37.0812586279939,
3.26590689904296));
#279846=CARTESIAN_POINT('Ctrl Pts',(-8.13177598651393,37.2312586279933,
5.9080810824151));
#279847=CARTESIAN_POINT('Ctrl Pts',(-6.21212407589623,37.3812586279927,
8.55025526578723));
#279848=CARTESIAN_POINT('Ctrl Pts',(-3.10606203794813,37.5312586279921,
9.55947599963789));
#279849=CARTESIAN_POINT('Ctrl Pts',(-3.22369386249354E-14,37.6812586279915,
10.5686967334885));
#279850=CARTESIAN_POINT('Ctrl Pts',(3.10606203794807,37.8312586279909,9.55947599963789));
#279851=CARTESIAN_POINT('Ctrl Pts',(6.21212407589617,37.9812586279903,8.55025526578723));
#279852=CARTESIAN_POINT('Ctrl Pts',(8.13177598651386,38.1312586279897,5.90808108241509));
#279853=CARTESIAN_POINT('Ctrl Pts',(10.0514278971316,38.2812586279891,3.26590689904295));
#279854=CARTESIAN_POINT('Ctrl Pts',(10.0514278971316,38.4312586279885,-1.23094490010826E-15));
#279855=CARTESIAN_POINT('Ctrl Pts',(10.0514278971315,38.5812586279879,-3.26590689904296));
#279856=CARTESIAN_POINT('Ctrl Pts',(8.13177598651386,38.7312586279873,-5.9080810824151));
#279857=CARTESIAN_POINT('Ctrl Pts',(6.21212407589617,38.8812586279867,-8.55025526578723));
#279858=CARTESIAN_POINT('Ctrl Pts',(3.10606203794807,39.0312586279861,-9.55947599963789));
#279859=CARTESIAN_POINT('Ctrl Pts',(-3.56893773859315E-14,39.1812586279855,
-10.5686967334885));
#279860=CARTESIAN_POINT('Ctrl Pts',(-3.10606203794814,39.3312586279849,
-9.55947599963789));
#279861=CARTESIAN_POINT('Ctrl Pts',(-6.21212407589624,39.4812586279843,
-8.55025526578723));
#279862=CARTESIAN_POINT('Ctrl Pts',(-8.13177598651393,39.6312586279837,
-5.90808108241509));
#279863=CARTESIAN_POINT('Ctrl Pts',(-10.0514278971316,39.7812586279831,
-3.26590689904296));
#279864=CARTESIAN_POINT('Ctrl Pts',(-10.0514278971316,39.9312586279825,
2.46188980021652E-15));
#279865=CARTESIAN_POINT('Ctrl Pts',(-10.0514278971316,40.0812586279819,
3.26590689904296));
#279866=CARTESIAN_POINT('Ctrl Pts',(-8.13177598651393,40.2312586279813,
5.9080810824151));
#279867=CARTESIAN_POINT('Ctrl Pts',(-6.21212407589624,40.3812586279807,
8.55025526578723));
#279868=CARTESIAN_POINT('Ctrl Pts',(-3.10606203794814,40.5312586279801,
9.55947599963789));
#279869=CARTESIAN_POINT('Ctrl Pts',(-3.39646478965972E-14,40.6812586279795,
10.5686967334885));
#279870=CARTESIAN_POINT('Ctrl Pts',(3.10606203794807,40.8312586279789,9.55947599963789));
#279871=CARTESIAN_POINT('Ctrl Pts',(6.21212407589617,40.9812586279783,8.55025526578723));
#279872=CARTESIAN_POINT('Ctrl Pts',(8.13177598651386,41.1312586279777,5.90808108241509));
#279873=CARTESIAN_POINT('Ctrl Pts',(10.0514278971315,41.2812586279771,3.26590689904295));
#279874=CARTESIAN_POINT('Ctrl Pts',(10.0514278971315,41.4312586279765,-1.23094490010826E-15));
#279875=CARTESIAN_POINT('Ctrl Pts',(10.0514278971315,41.5812586279759,-3.26590689904296));
#279876=CARTESIAN_POINT('Ctrl Pts',(8.13177598651386,41.7312586279753,-5.9080810824151));
#279877=CARTESIAN_POINT('Ctrl Pts',(6.21212407589617,41.8812586279747,-8.55025526578723));
#279878=CARTESIAN_POINT('Ctrl Pts',(3.10606203794806,42.0312586279741,-9.55947599963789));
#279879=CARTESIAN_POINT('Ctrl Pts',(-3.74170866575933E-14,42.1812586279735,
-10.5686967334885));
#279880=CARTESIAN_POINT('Ctrl Pts',(-3.10606203794814,42.3312586279729,
-9.55947599963789));
#279881=CARTESIAN_POINT('Ctrl Pts',(-6.21212407589624,42.4812586279723,
-8.55025526578723));
#279882=CARTESIAN_POINT('Ctrl Pts',(-8.13177598651393,42.6312586279717,
-5.90808108241509));
#279883=CARTESIAN_POINT('Ctrl Pts',(-10.0514278971316,42.7812586279711,
-3.26590689904296));
#279884=CARTESIAN_POINT('Ctrl Pts',(-10.0514278971316,42.9312586279705,
2.46188980021652E-15));
#279885=CARTESIAN_POINT('Ctrl Pts',(-10.0514278971316,43.0812586279699,
3.26590689904296));
#279886=CARTESIAN_POINT('Ctrl Pts',(-8.13177598651393,43.2312586279693,
5.9080810824151));
#279887=CARTESIAN_POINT('Ctrl Pts',(-6.21212407589624,43.3812586279687,
8.55025526578723));
#279888=CARTESIAN_POINT('Ctrl Pts',(-3.10606203794814,43.5312586279681,
9.55947599963789));
#279889=CARTESIAN_POINT('Ctrl Pts',(-3.5692357168259E-14,43.6812586279675,
10.5686967334885));
#279890=CARTESIAN_POINT('Ctrl Pts',(3.10606203794807,43.8312586279669,9.55947599963789));
#279891=CARTESIAN_POINT('Ctrl Pts',(6.21212407589617,43.9812586279663,8.55025526578723));
#279892=CARTESIAN_POINT('Ctrl Pts',(8.13177598651386,44.1312586279657,5.90808108241509));
#279893=CARTESIAN_POINT('Ctrl Pts',(10.0514278971315,44.2812586279651,3.26590689904295));
#279894=CARTESIAN_POINT('Ctrl Pts',(10.0514278971315,44.4312586279645,-1.23094490010826E-15));
#279895=CARTESIAN_POINT('Ctrl Pts',(10.0514278971315,44.5812586279639,-3.26590689904296));
#279896=CARTESIAN_POINT('Ctrl Pts',(8.13177598651385,44.7312586279633,-5.9080810824151));
#279897=CARTESIAN_POINT('Ctrl Pts',(6.21212407589616,44.8812586279627,-8.55025526578723));
#279898=CARTESIAN_POINT('Ctrl Pts',(3.10606203794806,45.0312586279621,-9.55947599963789));
#279899=CARTESIAN_POINT('Ctrl Pts',(-3.91447959292551E-14,45.1812586279615,
-10.5686967334885));
#279900=CARTESIAN_POINT('Ctrl Pts',(-3.10606203794814,45.3312586279609,
-9.55947599963789));
#279901=CARTESIAN_POINT('Ctrl Pts',(-6.21212407589624,45.4812586279603,
-8.55025526578723));
#279902=CARTESIAN_POINT('Ctrl Pts',(-8.13177598651393,45.6312586279597,
-5.90808108241509));
#279903=CARTESIAN_POINT('Ctrl Pts',(-10.0514278971316,45.7812586279591,
-3.26590689904296));
#279904=CARTESIAN_POINT('Ctrl Pts',(-10.0514278971316,45.9312586279585,
2.46188980021652E-15));
#279905=CARTESIAN_POINT('Ctrl Pts',(-10.0514278971316,46.0812586279579,
3.26590689904296));
#279906=CARTESIAN_POINT('Ctrl Pts',(-8.13177598651393,46.2312586279573,
5.9080810824151));
#279907=CARTESIAN_POINT('Ctrl Pts',(-6.21212407589624,46.3812586279567,
8.55025526578723));
#279908=CARTESIAN_POINT('Ctrl Pts',(-3.10606203794814,46.5312586279561,
9.55947599963789));
#279909=CARTESIAN_POINT('Ctrl Pts',(-3.74200664399209E-14,46.6812586279555,
10.5686967334885));
#279910=CARTESIAN_POINT('Ctrl Pts',(3.10606203794806,46.8312586279549,9.55947599963789));
#279911=CARTESIAN_POINT('Ctrl Pts',(6.21212407589617,46.9812586279543,8.55025526578723));
#279912=CARTESIAN_POINT('Ctrl Pts',(8.13177598651385,47.1312586279537,5.90808108241509));
#279913=CARTESIAN_POINT('Ctrl Pts',(10.0514278971315,47.2812586279531,3.26590689904295));
#279914=CARTESIAN_POINT('Ctrl Pts',(10.0514278971315,47.4312586279525,-1.23094490010826E-15));
#279915=CARTESIAN_POINT('Ctrl Pts',(10.0514278971315,47.5812586279519,-3.26590689904296));
#279916=CARTESIAN_POINT('Ctrl Pts',(8.13177598651385,47.7312586279513,-5.9080810824151));
#279917=CARTESIAN_POINT('Ctrl Pts',(6.21212407589616,47.8812586279507,-8.55025526578723));
#279918=CARTESIAN_POINT('Ctrl Pts',(3.10606203794806,48.0312586279501,-9.55947599963789));
#279919=CARTESIAN_POINT('Ctrl Pts',(-4.0872505200917E-14,48.1812586279495,
-10.5686967334885));
#279920=CARTESIAN_POINT('Ctrl Pts',(-3.10606203794814,48.3312586279489,
-9.55947599963789));
#279921=CARTESIAN_POINT('Ctrl Pts',(-6.21212407589625,48.4812586279483,
-8.55025526578723));
#279922=CARTESIAN_POINT('Ctrl Pts',(-8.13177598651394,48.6312586279477,
-5.90808108241509));
#279923=CARTESIAN_POINT('Ctrl Pts',(-10.0514278971316,48.7812586279471,
-3.26590689904296));
#279924=CARTESIAN_POINT('Ctrl Pts',(-10.0514278971316,48.9312586279465,
2.46188980021652E-15));
#279925=CARTESIAN_POINT('Ctrl Pts',(-10.0514278971316,49.0812586279459,
3.26590689904296));
#279926=CARTESIAN_POINT('Ctrl Pts',(-8.13177598651394,49.2312586279453,
5.9080810824151));
#279927=CARTESIAN_POINT('Ctrl Pts',(-6.21212407589624,49.3812586279447,
8.55025526578723));
#279928=CARTESIAN_POINT('Ctrl Pts',(-3.10606203794814,49.5312586279441,
9.55947599963789));
#279929=CARTESIAN_POINT('Ctrl Pts',(-3.91477757115827E-14,49.6812586279435,
10.5686967334885));
#279930=CARTESIAN_POINT('Ctrl Pts',(3.10606203794806,49.8312586279429,9.55947599963789));
#279931=CARTESIAN_POINT('Ctrl Pts',(6.21212407589616,49.9812586279423,8.55025526578723));
#279932=CARTESIAN_POINT('Ctrl Pts',(8.13177598651385,50.1312586279417,5.90808108241509));
#279933=CARTESIAN_POINT('Ctrl Pts',(10.0514278971315,50.2812586279411,3.26590689904295));
#279934=CARTESIAN_POINT('Ctrl Pts',(10.0514278971315,50.4312586279405,-1.23094490010826E-15));
#279935=CARTESIAN_POINT('Ctrl Pts',(10.0514278971315,50.5812586279399,-3.26590689904296));
#279936=CARTESIAN_POINT('Ctrl Pts',(8.13177598651385,50.7312586279393,-5.9080810824151));
#279937=CARTESIAN_POINT('Ctrl Pts',(6.21212407589616,50.8812586279387,-8.55025526578723));
#279938=CARTESIAN_POINT('Ctrl Pts',(3.10606203794806,51.0312586279381,-9.55947599963789));
#279939=CARTESIAN_POINT('Ctrl Pts',(-4.26002144725788E-14,51.1812586279375,
-10.5686967334885));
#279940=CARTESIAN_POINT('Ctrl Pts',(-3.10606203794814,51.3312586279369,
-9.55947599963789));
#279941=CARTESIAN_POINT('Ctrl Pts',(-6.21212407589625,51.4812586279363,
-8.55025526578723));
#279942=CARTESIAN_POINT('Ctrl Pts',(-8.13177598651394,51.6312586279357,
-5.90808108241509));
#279943=CARTESIAN_POINT('Ctrl Pts',(-10.0514278971316,51.7812586279351,
-3.26590689904296));
#279944=CARTESIAN_POINT('Ctrl Pts',(-10.0514278971316,51.9312586279345,
2.46188980021652E-15));
#279945=CARTESIAN_POINT('Ctrl Pts',(-10.0514278971316,52.0812586279339,
3.26590689904296));
#279946=CARTESIAN_POINT('Ctrl Pts',(-8.13177598651394,52.2312586279333,
5.9080810824151));
#279947=CARTESIAN_POINT('Ctrl Pts',(-6.21212407589625,52.3812586279327,
8.55025526578723));
#279948=CARTESIAN_POINT('Ctrl Pts',(-3.10606203794814,52.5312586279321,
9.55947599963789));
#279949=CARTESIAN_POINT('Ctrl Pts',(-4.08754849832446E-14,52.6812586279315,
10.5686967334885));
#279950=CARTESIAN_POINT('Ctrl Pts',(3.10606203794806,52.8312586279309,9.55947599963789));
#279951=CARTESIAN_POINT('Ctrl Pts',(6.21212407589616,52.9812586279303,8.55025526578723));
#279952=CARTESIAN_POINT('Ctrl Pts',(8.13177598651385,53.1312586279297,5.90808108241509));
#279953=CARTESIAN_POINT('Ctrl Pts',(10.0514278971315,53.2812586279291,3.26590689904295));
#279954=CARTESIAN_POINT('Ctrl Pts',(10.0514278971315,53.4312586279285,-1.23094490010826E-15));
#279955=CARTESIAN_POINT('Ctrl Pts',(10.0514278971315,53.5812586279279,-3.26590689904296));
#279956=CARTESIAN_POINT('Ctrl Pts',(8.13177598651385,53.7312586279273,-5.9080810824151));
#279957=CARTESIAN_POINT('Ctrl Pts',(6.21212407589616,53.8812586279267,-8.55025526578723));
#279958=CARTESIAN_POINT('Ctrl Pts',(3.10606203794806,54.0312586279261,-9.55947599963789));
#279959=CARTESIAN_POINT('Ctrl Pts',(-4.43279237442407E-14,54.1812586279255,
-10.5686967334885));
#279960=CARTESIAN_POINT('Ctrl Pts',(-3.10606203794815,54.3312586279249,
-9.55947599963789));
#279961=CARTESIAN_POINT('Ctrl Pts',(-6.21212407589625,54.4812586279243,
-8.55025526578723));
#279962=CARTESIAN_POINT('Ctrl Pts',(-8.13177598651394,54.6312586279237,
-5.90808108241509));
#279963=CARTESIAN_POINT('Ctrl Pts',(-10.0514278971316,54.7812586279231,
-3.26590689904296));
#279964=CARTESIAN_POINT('Ctrl Pts',(-10.0514278971316,54.9312586279225,
2.46188980021652E-15));
#279965=CARTESIAN_POINT('Ctrl Pts',(-10.0514278971316,55.0812586279219,
3.26590689904296));
#279966=CARTESIAN_POINT('Ctrl Pts',(-8.13177598651394,55.2312586279213,
5.9080810824151));
#279967=CARTESIAN_POINT('Ctrl Pts',(-6.21212407589625,55.3812586279207,
8.55025526578723));
#279968=CARTESIAN_POINT('Ctrl Pts',(-3.10606203794814,55.5312586279201,
9.55947599963789));
#279969=CARTESIAN_POINT('Ctrl Pts',(-4.26031942549064E-14,55.6812586279195,
10.5686967334885));
#279970=CARTESIAN_POINT('Ctrl Pts',(3.10606203794806,55.8312586279189,9.55947599963789));
#279971=CARTESIAN_POINT('Ctrl Pts',(6.21212407589616,55.9812586279183,8.55025526578723));
#279972=CARTESIAN_POINT('Ctrl Pts',(8.13177598651385,56.1312586279177,5.90808108241509));
#279973=CARTESIAN_POINT('Ctrl Pts',(10.0514278971315,56.2812586279171,3.26590689904295));
#279974=CARTESIAN_POINT('Ctrl Pts',(10.0514278971315,56.4312586279165,-1.23094490010826E-15));
#279975=CARTESIAN_POINT('Ctrl Pts',(10.0514278971315,56.5812586279159,-3.26590689904296));
#279976=CARTESIAN_POINT('Ctrl Pts',(8.13177598651385,56.7312586279153,-5.9080810824151));
#279977=CARTESIAN_POINT('Ctrl Pts',(6.21212407589616,56.8812586279147,-8.55025526578723));
#279978=CARTESIAN_POINT('Ctrl Pts',(3.10606203794806,57.0312586279141,-9.55947599963789));
#279979=CARTESIAN_POINT('Ctrl Pts',(-4.60556330159025E-14,57.1812586279135,
-10.5686967334885));
#279980=CARTESIAN_POINT('Ctrl Pts',(-3.10606203794815,57.3312586279129,
-9.55947599963789));
#279981=CARTESIAN_POINT('Ctrl Pts',(-6.21212407589625,57.4812586279123,
-8.55025526578723));
#279982=CARTESIAN_POINT('Ctrl Pts',(-8.13177598651394,57.6312586279117,
-5.90808108241509));
#279983=CARTESIAN_POINT('Ctrl Pts',(-10.0514278971316,57.7812586279111,
-3.26590689904296));
#279984=CARTESIAN_POINT('Ctrl Pts',(-10.0514278971316,57.9312586279105,
2.46188980021652E-15));
#279985=CARTESIAN_POINT('Ctrl Pts',(-10.0514278971316,58.0812586279099,
3.26590689904296));
#279986=CARTESIAN_POINT('Ctrl Pts',(-8.13177598651394,58.2312586279093,
5.9080810824151));
#279987=CARTESIAN_POINT('Ctrl Pts',(-6.21212407589625,58.3812586279087,
8.55025526578723));
#279988=CARTESIAN_POINT('Ctrl Pts',(-3.10606203794815,58.5312586279081,
9.55947599963789));
#279989=CARTESIAN_POINT('Ctrl Pts',(-4.43309035265682E-14,58.6812586279075,
10.5686967334885));
#279990=CARTESIAN_POINT('Ctrl Pts',(3.10606203794806,58.8312586279069,9.55947599963789));
#279991=CARTESIAN_POINT('Ctrl Pts',(6.21212407589616,58.9812586279063,8.55025526578723));
#279992=CARTESIAN_POINT('Ctrl Pts',(8.13177598651385,59.1312586279057,5.90808108241509));
#279993=CARTESIAN_POINT('Ctrl Pts',(10.0514278971315,59.2812586279051,3.26590689904295));
#279994=CARTESIAN_POINT('Ctrl Pts',(10.0514278971315,59.4312586279045,-1.23094490010826E-15));
#279995=CARTESIAN_POINT('Ctrl Pts',(10.0514278971315,59.5812586279039,-3.26590689904296));
#279996=CARTESIAN_POINT('Ctrl Pts',(8.13177598651385,59.7312586279033,-5.9080810824151));
#279997=CARTESIAN_POINT('Ctrl Pts',(6.21212407589616,59.8812586279027,-8.55025526578723));
#279998=CARTESIAN_POINT('Ctrl Pts',(3.10606203794805,60.0312586279021,-9.55947599963789));
#279999=CARTESIAN_POINT('Ctrl Pts',(-4.77833422875643E-14,60.1812586279015,
-10.5686967334885));
#280000=CARTESIAN_POINT('Ctrl Pts',(-3.10606203794815,60.3312586279009,
-9.55947599963789));
#280001=CARTESIAN_POINT('Ctrl Pts',(-6.21212407589625,60.4812586279003,
-8.55025526578723));
#280002=CARTESIAN_POINT('Ctrl Pts',(-8.13177598651394,60.6312586278997,
-5.90808108241509));
#280003=CARTESIAN_POINT('Ctrl Pts',(-10.0514278971316,60.7812586278991,
-3.26590689904296));
#280004=CARTESIAN_POINT('Ctrl Pts',(-10.0514278971316,60.9312586278985,
2.46188980021652E-15));
#280005=CARTESIAN_POINT('Ctrl Pts',(-10.0514278971316,61.0812586278979,
3.26590689904296));
#280006=CARTESIAN_POINT('Ctrl Pts',(-8.13177598651394,61.2312586278973,
5.9080810824151));
#280007=CARTESIAN_POINT('Ctrl Pts',(-6.21212407589625,61.3812586278967,
8.55025526578723));
#280008=CARTESIAN_POINT('Ctrl Pts',(-3.10606203794815,61.5312586278961,
9.55947599963789));
#280009=CARTESIAN_POINT('Ctrl Pts',(-4.60586127982301E-14,61.6812586278955,
10.5686967334885));
#280010=CARTESIAN_POINT('Ctrl Pts',(3.10606203794806,61.8312586278949,9.55947599963789));
#280011=CARTESIAN_POINT('Ctrl Pts',(6.21212407589616,61.9812586278943,8.55025526578723));
#280012=CARTESIAN_POINT('Ctrl Pts',(8.13177598651385,62.1312586278937,5.90808108241509));
#280013=CARTESIAN_POINT('Ctrl Pts',(10.0514278971315,62.2812586278931,3.26590689904295));
#280014=CARTESIAN_POINT('Ctrl Pts',(10.0514278971315,62.4312586278925,-1.23094490010826E-15));
#280015=CARTESIAN_POINT('Ctrl Pts',(10.0514278971315,62.5812586278919,-3.26590689904296));
#280016=CARTESIAN_POINT('Ctrl Pts',(8.13177598651384,62.7312586278913,-5.9080810824151));
#280017=CARTESIAN_POINT('Ctrl Pts',(6.21212407589615,62.8812586278907,-8.55025526578723));
#280018=CARTESIAN_POINT('Ctrl Pts',(3.10606203794805,63.0312586278901,-9.55947599963789));
#280019=CARTESIAN_POINT('Ctrl Pts',(-4.95110515592262E-14,63.1812586278895,
-10.5686967334885));
#280020=CARTESIAN_POINT('Ctrl Pts',(-3.10606203794815,63.3312586278889,
-9.55947599963789));
#280021=CARTESIAN_POINT('Ctrl Pts',(-6.21212407589625,63.4812586278883,
-8.55025526578723));
#280022=CARTESIAN_POINT('Ctrl Pts',(-8.13177598651395,63.6312586278877,
-5.90808108241509));
#280023=CARTESIAN_POINT('Ctrl Pts',(-10.0514278971316,63.7812586278871,
-3.26590689904296));
#280024=CARTESIAN_POINT('Ctrl Pts',(-10.0514278971316,63.9312586278865,
2.46188980021652E-15));
#280025=CARTESIAN_POINT('Ctrl Pts',(-10.0514278971316,64.0812586278859,
3.26590689904296));
#280026=CARTESIAN_POINT('Ctrl Pts',(-8.13177598651395,64.2312586278853,
5.9080810824151));
#280027=CARTESIAN_POINT('Ctrl Pts',(-6.21212407589625,64.3812586278847,
8.55025526578723));
#280028=CARTESIAN_POINT('Ctrl Pts',(-3.10606203794815,64.5312586278841,
9.55947599963789));
#280029=CARTESIAN_POINT('Ctrl Pts',(-4.77863220698919E-14,64.6812586278835,
10.5686967334885));
#280030=CARTESIAN_POINT('Ctrl Pts',(3.10606203794805,64.8312586278829,9.55947599963789));
#280031=CARTESIAN_POINT('Ctrl Pts',(6.21212407589616,64.9812586278823,8.55025526578723));
#280032=CARTESIAN_POINT('Ctrl Pts',(8.13177598651384,65.1312586278817,5.90808108241509));
#280033=CARTESIAN_POINT('Ctrl Pts',(10.0514278971315,65.2812586278811,3.26590689904295));
#280034=CARTESIAN_POINT('Ctrl Pts',(10.0514278971315,65.4312586278805,-1.23094490010826E-15));
#280035=CARTESIAN_POINT('Ctrl Pts',(10.0514278971315,65.5812586278799,-3.26590689904296));
#280036=CARTESIAN_POINT('Ctrl Pts',(8.13177598651384,65.7312586278793,-5.9080810824151));
#280037=CARTESIAN_POINT('Ctrl Pts',(6.21212407589615,65.8812586278787,-8.55025526578723));
#280038=CARTESIAN_POINT('Ctrl Pts',(3.10606203794805,66.0312586278781,-9.55947599963789));
#280039=CARTESIAN_POINT('Ctrl Pts',(-5.1238760830888E-14,66.1812586278775,
-10.5686967334885));
#280040=CARTESIAN_POINT('Ctrl Pts',(-3.10606203794815,66.3312586278769,
-9.55947599963789));
#280041=CARTESIAN_POINT('Ctrl Pts',(-6.21212407589625,66.4812586278763,
-8.55025526578723));
#280042=CARTESIAN_POINT('Ctrl Pts',(-8.13177598651395,66.6312586278757,
-5.90808108241509));
#280043=CARTESIAN_POINT('Ctrl Pts',(-10.0514278971316,66.7812586278751,
-3.26590689904296));
#280044=CARTESIAN_POINT('Ctrl Pts',(-10.0514278971316,66.9312586278745,
2.46188980021652E-15));
#280045=CARTESIAN_POINT('Ctrl Pts',(-10.0514278971316,67.0812586278739,
3.26590689904296));
#280046=CARTESIAN_POINT('Ctrl Pts',(-8.13177598651395,67.2312586278733,
5.9080810824151));
#280047=CARTESIAN_POINT('Ctrl Pts',(-6.21212407589625,67.3812586278727,
8.55025526578723));
#280048=CARTESIAN_POINT('Ctrl Pts',(-3.10606203794815,67.5312586278721,
9.55947599963789));
#280049=CARTESIAN_POINT('Ctrl Pts',(-4.95140313415538E-14,67.6812586278715,
10.5686967334885));
#280050=CARTESIAN_POINT('Ctrl Pts',(3.10606203794805,67.8312586278709,9.55947599963789));
#280051=CARTESIAN_POINT('Ctrl Pts',(6.21212407589615,67.9812586278703,8.55025526578723));
#280052=CARTESIAN_POINT('Ctrl Pts',(8.13177598651384,68.1312586278697,5.90808108241509));
#280053=CARTESIAN_POINT('Ctrl Pts',(10.0514278971315,68.2812586278691,3.26590689904295));
#280054=CARTESIAN_POINT('Ctrl Pts',(10.0514278971315,68.4312586278685,-1.23094490010826E-15));
#280055=CARTESIAN_POINT('Ctrl Pts',(10.0514278971315,68.5812586278679,-3.26590689904296));
#280056=CARTESIAN_POINT('Ctrl Pts',(8.13177598651384,68.7312586278673,-5.9080810824151));
#280057=CARTESIAN_POINT('Ctrl Pts',(6.21212407589615,68.8812586278667,-8.55025526578723));
#280058=CARTESIAN_POINT('Ctrl Pts',(3.10606203794805,69.0312586278661,-9.55947599963789));
#280059=CARTESIAN_POINT('Ctrl Pts',(-5.29664701025498E-14,69.1812586278655,
-10.5686967334885));
#280060=CARTESIAN_POINT('Ctrl Pts',(-3.10606203794816,69.3312586278649,
-9.55947599963789));
#280061=CARTESIAN_POINT('Ctrl Pts',(-6.21212407589626,69.4812586278643,
-8.55025526578723));
#280062=CARTESIAN_POINT('Ctrl Pts',(-8.13177598651395,69.6312586278637,
-5.90808108241509));
#280063=CARTESIAN_POINT('Ctrl Pts',(-10.0514278971316,69.7812586278631,
-3.26590689904296));
#280064=CARTESIAN_POINT('Ctrl Pts',(-10.0514278971316,69.9312586278625,
2.46188980021652E-15));
#280065=CARTESIAN_POINT('Ctrl Pts',(-10.0514278971316,70.0812586278619,
3.26590689904296));
#280066=CARTESIAN_POINT('Ctrl Pts',(-8.13177598651395,70.2312586278613,
5.9080810824151));
#280067=CARTESIAN_POINT('Ctrl Pts',(-6.21212407589625,70.3812586278607,
8.55025526578723));
#280068=CARTESIAN_POINT('Ctrl Pts',(-3.10606203794815,70.5312586278601,
9.55947599963789));
#280069=CARTESIAN_POINT('Ctrl Pts',(-5.12417406132156E-14,70.6812586278595,
10.5686967334885));
#280070=CARTESIAN_POINT('Ctrl Pts',(3.10606203794805,70.8312586278589,9.55947599963789));
#280071=CARTESIAN_POINT('Ctrl Pts',(6.21212407589615,70.9812586278583,8.55025526578723));
#280072=CARTESIAN_POINT('Ctrl Pts',(8.13177598651384,71.1312586278577,5.90808108241509));
#280073=CARTESIAN_POINT('Ctrl Pts',(10.0514278971315,71.2812586278571,3.26590689904295));
#280074=CARTESIAN_POINT('Ctrl Pts',(10.0514278971315,71.4312586278565,-1.23094490010826E-15));
#280075=CARTESIAN_POINT('Ctrl Pts',(10.0514278971315,71.5812586278559,-3.26590689904296));
#280076=CARTESIAN_POINT('Ctrl Pts',(8.13177598651384,71.7312586278553,-5.9080810824151));
#280077=CARTESIAN_POINT('Ctrl Pts',(6.21212407589615,71.8812586278547,-8.55025526578723));
#280078=CARTESIAN_POINT('Ctrl Pts',(3.10606203794805,72.0312586278541,-9.55947599963789));
#280079=CARTESIAN_POINT('Ctrl Pts',(-5.46941793742117E-14,72.1812586278535,
-10.5686967334885));
#280080=CARTESIAN_POINT('Ctrl Pts',(-3.10606203794816,72.3312586278529,
-9.55947599963789));
#280081=CARTESIAN_POINT('Ctrl Pts',(-6.21212407589626,72.4812586278523,
-8.55025526578723));
#280082=CARTESIAN_POINT('Ctrl Pts',(-8.13177598651395,72.6312586278517,
-5.90808108241509));
#280083=CARTESIAN_POINT('Ctrl Pts',(-10.0514278971316,72.7812586278511,
-3.26590689904296));
#280084=CARTESIAN_POINT('Ctrl Pts',(-10.0514278971316,72.9312586278505,
2.46188980021652E-15));
#280085=CARTESIAN_POINT('Ctrl Pts',(-10.0514278971316,73.0812586278499,
3.26590689904296));
#280086=CARTESIAN_POINT('Ctrl Pts',(-8.13177598651395,73.2312586278493,
5.9080810824151));
#280087=CARTESIAN_POINT('Ctrl Pts',(-6.21212407589625,73.3812586278487,
8.55025526578723));
#280088=CARTESIAN_POINT('Ctrl Pts',(-3.10606203794815,73.5312586278481,
9.55947599963789));
#280089=CARTESIAN_POINT('Ctrl Pts',(-5.29694498848774E-14,73.6812586278475,
10.5686967334885));
#280090=CARTESIAN_POINT('Ctrl Pts',(3.10606203794805,73.8312586278469,9.55947599963789));
#280091=CARTESIAN_POINT('Ctrl Pts',(6.21212407589615,73.9812586278463,8.55025526578723));
#280092=CARTESIAN_POINT('Ctrl Pts',(8.13177598651384,74.1312586278457,5.90808108241509));
#280093=CARTESIAN_POINT('Ctrl Pts',(10.0514278971315,74.2812586278451,3.26590689904295));
#280094=CARTESIAN_POINT('Ctrl Pts',(10.0514278971315,74.4312586278445,-1.23094490010826E-15));
#280095=CARTESIAN_POINT('Ctrl Pts',(10.0514278971315,74.5812586278439,-3.26590689904296));
#280096=CARTESIAN_POINT('Ctrl Pts',(8.13177598651384,74.7312586278433,-5.9080810824151));
#280097=CARTESIAN_POINT('Ctrl Pts',(6.21212407589614,74.8812586278427,-8.55025526578723));
#280098=CARTESIAN_POINT('Ctrl Pts',(3.10606203794805,75.0312586278421,-9.55947599963789));
#280099=CARTESIAN_POINT('Ctrl Pts',(-5.64218886458735E-14,75.1812586278415,
-10.5686967334885));
#280100=CARTESIAN_POINT('Ctrl Pts',(-3.10606203794816,75.3312586278409,
-9.55947599963789));
#280101=CARTESIAN_POINT('Ctrl Pts',(-6.21212407589626,75.4812586278403,
-8.55025526578723));
#280102=CARTESIAN_POINT('Ctrl Pts',(-8.13177598651395,75.6312586278397,
-5.90808108241509));
#280103=CARTESIAN_POINT('Ctrl Pts',(-10.0514278971316,75.7812586278391,
-3.26590689904296));
#280104=CARTESIAN_POINT('Ctrl Pts',(-10.0514278971316,75.9312586278385,
2.46188980021652E-15));
#280105=CARTESIAN_POINT('Ctrl Pts',(-10.0514278971316,76.0812586278379,
3.26590689904296));
#280106=CARTESIAN_POINT('Ctrl Pts',(-8.13177598651395,76.2312586278373,
5.9080810824151));
#280107=CARTESIAN_POINT('Ctrl Pts',(-6.21212407589626,76.3812586278367,
8.55025526578723));
#280108=CARTESIAN_POINT('Ctrl Pts',(-3.10606203794816,76.5312586278361,
9.55947599963789));
#280109=CARTESIAN_POINT('Ctrl Pts',(-5.46971591565393E-14,76.6812586278355,
10.5686967334885));
#280110=CARTESIAN_POINT('Ctrl Pts',(3.10606203794805,76.8312586278349,9.55947599963789));
#280111=CARTESIAN_POINT('Ctrl Pts',(6.21212407589615,76.9812586278343,8.55025526578723));
#280112=CARTESIAN_POINT('Ctrl Pts',(8.13177598651384,77.1312586278337,5.90808108241509));
#280113=CARTESIAN_POINT('Ctrl Pts',(10.0514278971315,77.2812586278331,3.26590689904295));
#280114=CARTESIAN_POINT('Ctrl Pts',(10.0514278971315,77.4312586278325,-1.23094490010826E-15));
#280115=CARTESIAN_POINT('Ctrl Pts',(10.0514278971315,77.5812586278319,-3.26590689904296));
#280116=CARTESIAN_POINT('Ctrl Pts',(8.13177598651384,77.7312586278313,-5.9080810824151));
#280117=CARTESIAN_POINT('Ctrl Pts',(6.21212407589614,77.8812586278307,-8.55025526578723));
#280118=CARTESIAN_POINT('Ctrl Pts',(3.10606203794804,78.0312586278301,-9.55947599963789));
#280119=CARTESIAN_POINT('Ctrl Pts',(-5.81495979175354E-14,78.1812586278295,
-10.5686967334885));
#280120=CARTESIAN_POINT('Ctrl Pts',(-3.10606203794816,78.3312586278289,
-9.55947599963789));
#280121=CARTESIAN_POINT('Ctrl Pts',(-6.21212407589626,78.4812586278283,
-8.55025526578723));
#280122=CARTESIAN_POINT('Ctrl Pts',(-8.13177598651395,78.6312586278277,
-5.90808108241509));
#280123=CARTESIAN_POINT('Ctrl Pts',(-10.0514278971316,78.7812586278271,
-3.26590689904296));
#280124=CARTESIAN_POINT('Ctrl Pts',(-10.0514278971316,78.9312586278265,
2.46188980021652E-15));
#280125=CARTESIAN_POINT('Ctrl Pts',(-10.0514278971316,79.0812586278259,
3.26590689904296));
#280126=CARTESIAN_POINT('Ctrl Pts',(-8.13177598651395,79.2312586278253,
5.9080810824151));
#280127=CARTESIAN_POINT('Ctrl Pts',(-6.21212407589626,79.3812586278247,
8.55025526578723));
#280128=CARTESIAN_POINT('Ctrl Pts',(-3.10606203794816,79.5312586278241,
9.55947599963789));
#280129=CARTESIAN_POINT('Ctrl Pts',(-5.64248684282011E-14,79.6812586278235,
10.5686967334885));
#280130=CARTESIAN_POINT('Ctrl Pts',(3.10606203794805,79.8312586278229,9.55947599963789));
#280131=CARTESIAN_POINT('Ctrl Pts',(6.21212407589614,79.9812586278223,8.55025526578723));
#280132=CARTESIAN_POINT('Ctrl Pts',(8.13177598651384,80.1312586278217,5.90808108241509));
#280133=CARTESIAN_POINT('Ctrl Pts',(10.0514278971315,80.2812586278211,3.26590689904295));
#280134=CARTESIAN_POINT('Ctrl Pts',(10.0514278971315,80.4312586278205,-1.23094490010826E-15));
#280135=CARTESIAN_POINT('Ctrl Pts',(10.0514278971315,80.5812586278199,-3.26590689904296));
#280136=CARTESIAN_POINT('Ctrl Pts',(8.13177598651384,80.7312586278193,-5.9080810824151));
#280137=CARTESIAN_POINT('Ctrl Pts',(6.21212407589614,80.8812586278187,-8.55025526578723));
#280138=CARTESIAN_POINT('Ctrl Pts',(3.10606203794804,81.0312586278181,-9.55947599963789));
#280139=CARTESIAN_POINT('Ctrl Pts',(-5.98773071891972E-14,81.1812586278175,
-10.5686967334885));
#280140=CARTESIAN_POINT('Ctrl Pts',(-3.10606203794816,81.3312586278169,
-9.55947599963789));
#280141=CARTESIAN_POINT('Ctrl Pts',(-6.21212407589626,81.4812586278163,
-8.55025526578723));
#280142=CARTESIAN_POINT('Ctrl Pts',(-8.13177598651396,81.6312586278157,
-5.90808108241509));
#280143=CARTESIAN_POINT('Ctrl Pts',(-10.0514278971316,81.7812586278151,
-3.26590689904296));
#280144=CARTESIAN_POINT('Ctrl Pts',(-10.0514278971316,81.9312586278145,
2.46188980021652E-15));
#280145=CARTESIAN_POINT('Ctrl Pts',(-10.0514278971316,82.0812586278139,
3.26590689904296));
#280146=CARTESIAN_POINT('Ctrl Pts',(-8.13177598651396,82.2312586278133,
5.9080810824151));
#280147=CARTESIAN_POINT('Ctrl Pts',(-6.21212407589626,82.3812586278127,
8.55025526578723));
#280148=CARTESIAN_POINT('Ctrl Pts',(-3.10606203794816,82.5312586278121,
9.55947599963789));
#280149=CARTESIAN_POINT('Ctrl Pts',(-5.8152577699863E-14,82.6812586278115,
10.5686967334885));
#280150=CARTESIAN_POINT('Ctrl Pts',(3.10606203794804,82.8312586278109,9.55947599963789));
#280151=CARTESIAN_POINT('Ctrl Pts',(6.21212407589614,82.9812586278103,8.55025526578723));
#280152=CARTESIAN_POINT('Ctrl Pts',(8.13177598651383,83.1312586278097,5.90808108241509));
#280153=CARTESIAN_POINT('Ctrl Pts',(10.0514278971315,83.2812586278091,3.26590689904295));
#280154=CARTESIAN_POINT('Ctrl Pts',(10.0514278971315,83.4312586278085,-1.23094490010826E-15));
#280155=CARTESIAN_POINT('Ctrl Pts',(10.0514278971315,83.5812586278079,-3.26590689904296));
#280156=CARTESIAN_POINT('Ctrl Pts',(8.13177598651383,83.7312586278073,-5.9080810824151));
#280157=CARTESIAN_POINT('Ctrl Pts',(6.21212407589614,83.8812586278067,-8.55025526578723));
#280158=CARTESIAN_POINT('Ctrl Pts',(3.10606203794804,84.0312586278061,-9.55947599963789));
#280159=CARTESIAN_POINT('Ctrl Pts',(-6.1605016460859E-14,84.1812586278055,
-10.5686967334885));
#280160=CARTESIAN_POINT('Ctrl Pts',(-3.10606203794816,84.3312586278049,
-9.55947599963789));
#280161=CARTESIAN_POINT('Ctrl Pts',(-6.21212407589626,84.4812586278043,
-8.55025526578723));
#280162=CARTESIAN_POINT('Ctrl Pts',(-8.13177598651396,84.6312586278037,
-5.90808108241509));
#280163=CARTESIAN_POINT('Ctrl Pts',(-10.0514278971316,84.7812586278031,
-3.26590689904296));
#280164=CARTESIAN_POINT('Ctrl Pts',(-10.0514278971316,84.9312586278025,
2.46188980021652E-15));
#280165=CARTESIAN_POINT('Ctrl Pts',(-10.0514278971316,85.0812586278019,
3.26590689904296));
#280166=CARTESIAN_POINT('Ctrl Pts',(-8.13177598651396,85.2312586278013,
5.9080810824151));
#280167=CARTESIAN_POINT('Ctrl Pts',(-6.21212407589626,85.3812586278007,
8.55025526578723));
#280168=CARTESIAN_POINT('Ctrl Pts',(-3.10606203794816,85.5312586278001,
9.55947599963789));
#280169=CARTESIAN_POINT('Ctrl Pts',(-5.98802869715248E-14,85.6812586277995,
10.5686967334885));
#280170=CARTESIAN_POINT('Ctrl Pts',(3.10606203794804,85.8312586277989,9.55947599963789));
#280171=CARTESIAN_POINT('Ctrl Pts',(6.21212407589614,85.9812586277983,8.55025526578723));
#280172=CARTESIAN_POINT('Ctrl Pts',(8.13177598651383,86.1312586277977,5.90808108241509));
#280173=CARTESIAN_POINT('Ctrl Pts',(10.0514278971315,86.2812586277971,3.26590689904295));
#280174=CARTESIAN_POINT('Ctrl Pts',(10.0514278971315,86.4312586277965,-1.23094490010826E-15));
#280175=CARTESIAN_POINT('Ctrl Pts',(10.0514278971315,86.5812586277959,-3.26590689904296));
#280176=CARTESIAN_POINT('Ctrl Pts',(8.13177598651383,86.7312586277953,-5.9080810824151));
#280177=CARTESIAN_POINT('Ctrl Pts',(6.21212407589614,86.8812586277947,-8.55025526578723));
#280178=CARTESIAN_POINT('Ctrl Pts',(3.10606203794804,87.0312586277941,-9.55947599963789));
#280179=CARTESIAN_POINT('Ctrl Pts',(-6.33327257325209E-14,87.1812586277935,
-10.5686967334885));
#280180=CARTESIAN_POINT('Ctrl Pts',(-3.10606203794817,87.3312586277929,
-9.55947599963789));
#280181=CARTESIAN_POINT('Ctrl Pts',(-6.21212407589627,87.4812586277923,
-8.55025526578723));
#280182=CARTESIAN_POINT('Ctrl Pts',(-8.13177598651396,87.6312586277917,
-5.90808108241509));
#280183=CARTESIAN_POINT('Ctrl Pts',(-10.0514278971317,87.7812586277911,
-3.26590689904296));
#280184=CARTESIAN_POINT('Ctrl Pts',(-10.0514278971317,87.9312586277905,
2.46188980021652E-15));
#280185=CARTESIAN_POINT('Ctrl Pts',(-10.0514278971317,88.0812586277899,
3.26590689904296));
#280186=CARTESIAN_POINT('Ctrl Pts',(-8.13177598651396,88.2312586277893,
5.9080810824151));
#280187=CARTESIAN_POINT('Ctrl Pts',(-6.21212407589626,88.3812586277887,
8.55025526578723));
#280188=CARTESIAN_POINT('Ctrl Pts',(-3.10606203794816,88.5312586277881,
9.55947599963789));
#280189=CARTESIAN_POINT('Ctrl Pts',(-6.16079962431866E-14,88.6812586277875,
10.5686967334885));
#280190=CARTESIAN_POINT('Ctrl Pts',(3.10606203794804,88.8312586277869,9.55947599963789));
#280191=CARTESIAN_POINT('Ctrl Pts',(6.21212407589614,88.9812586277863,8.55025526578723));
#280192=CARTESIAN_POINT('Ctrl Pts',(8.13177598651383,89.1312586277857,5.90808108241509));
#280193=CARTESIAN_POINT('Ctrl Pts',(10.0514278971315,89.2812586277851,3.26590689904295));
#280194=CARTESIAN_POINT('Ctrl Pts',(10.0514278971315,89.4312586277845,-1.23094490010826E-15));
#280195=CARTESIAN_POINT('Ctrl Pts',(10.0514278971315,89.5812586277839,-3.26590689904296));
#280196=CARTESIAN_POINT('Ctrl Pts',(8.13177598651383,89.7312586277833,-5.9080810824151));
#280197=CARTESIAN_POINT('Ctrl Pts',(6.21212407589614,89.8812586277827,-8.55025526578723));
#280198=CARTESIAN_POINT('Ctrl Pts',(3.10606203794804,90.0312586277821,-9.55947599963789));
#280199=CARTESIAN_POINT('Ctrl Pts',(-6.50604350041827E-14,90.1812586277815,
-10.5686967334885));
#280200=CARTESIAN_POINT('Ctrl Pts',(-3.10606203794817,90.3312586277809,
-9.55947599963789));
#280201=CARTESIAN_POINT('Ctrl Pts',(-6.21212407589627,90.4812586277803,
-8.55025526578723));
#280202=CARTESIAN_POINT('Ctrl Pts',(-8.13177598651396,90.6312586277797,
-5.90808108241509));
#280203=CARTESIAN_POINT('Ctrl Pts',(-10.0514278971317,90.7812586277791,
-3.26590689904296));
#280204=CARTESIAN_POINT('Ctrl Pts',(-10.0514278971317,90.9312586277785,
2.46188980021652E-15));
#280205=CARTESIAN_POINT('Ctrl Pts',(-10.0514278971317,91.0812586277779,
3.26590689904296));
#280206=CARTESIAN_POINT('Ctrl Pts',(-8.13177598651396,91.2312586277773,
5.9080810824151));
#280207=CARTESIAN_POINT('Ctrl Pts',(-6.21212407589627,91.3812586277767,
8.55025526578723));
#280208=CARTESIAN_POINT('Ctrl Pts',(-3.10606203794817,91.5312586277761,
9.55947599963789));
#280209=CARTESIAN_POINT('Ctrl Pts',(-6.33357055148485E-14,91.6812586277755,
10.5686967334885));
#280210=CARTESIAN_POINT('Ctrl Pts',(3.10606203794804,91.8312586277749,9.55947599963789));
#280211=CARTESIAN_POINT('Ctrl Pts',(6.21212407589614,91.9812586277743,8.55025526578723));
#280212=CARTESIAN_POINT('Ctrl Pts',(8.13177598651383,92.1312586277737,5.90808108241509));
#280213=CARTESIAN_POINT('Ctrl Pts',(10.0514278971315,92.2812586277731,3.26590689904295));
#280214=CARTESIAN_POINT('Ctrl Pts',(10.0514278971315,92.4312586277725,-1.23094490010826E-15));
#280215=CARTESIAN_POINT('Ctrl Pts',(10.0514278971315,92.5812586277719,-3.26590689904296));
#280216=CARTESIAN_POINT('Ctrl Pts',(8.13177598651383,92.7312586277713,-5.9080810824151));
#280217=CARTESIAN_POINT('Ctrl Pts',(6.21212407589614,92.8812586277707,-8.55025526578723));
#280218=CARTESIAN_POINT('Ctrl Pts',(3.10606203794804,93.0312586277701,-9.55947599963789));
#280219=CARTESIAN_POINT('Ctrl Pts',(-6.67881442758446E-14,93.1812586277695,
-10.5686967334885));
#280220=CARTESIAN_POINT('Ctrl Pts',(-3.10606203794817,93.3312586277689,
-9.55947599963789));
#280221=CARTESIAN_POINT('Ctrl Pts',(-6.21212407589627,93.4812586277683,
-8.55025526578723));
#280222=CARTESIAN_POINT('Ctrl Pts',(-8.13177598651396,93.6312586277677,
-5.90808108241509));
#280223=CARTESIAN_POINT('Ctrl Pts',(-10.0514278971317,93.7812586277671,
-3.26590689904296));
#280224=CARTESIAN_POINT('Ctrl Pts',(-10.0514278971317,93.9312586277665,
2.46188980021652E-15));
#280225=CARTESIAN_POINT('Ctrl Pts',(-10.0514278971317,94.0812586277659,
3.26590689904296));
#280226=CARTESIAN_POINT('Ctrl Pts',(-8.13177598651396,94.2312586277653,
5.9080810824151));
#280227=CARTESIAN_POINT('Ctrl Pts',(-6.21212407589627,94.3812586277647,
8.55025526578723));
#280228=CARTESIAN_POINT('Ctrl Pts',(-3.10606203794817,94.5312586277641,
9.55947599963789));
#280229=CARTESIAN_POINT('Ctrl Pts',(-6.50634147865103E-14,94.6812586277635,
10.5686967334885));
#280230=CARTESIAN_POINT('Ctrl Pts',(3.10606203794804,94.8312586277629,9.55947599963789));
#280231=CARTESIAN_POINT('Ctrl Pts',(6.21212407589614,94.9812586277623,8.55025526578723));
#280232=CARTESIAN_POINT('Ctrl Pts',(8.13177598651383,95.1312586277617,5.90808108241509));
#280233=CARTESIAN_POINT('Ctrl Pts',(10.0514278971315,95.2812586277611,3.26590689904295));
#280234=CARTESIAN_POINT('Ctrl Pts',(10.0514278971315,95.4312586277605,-1.23094490010826E-15));
#280235=CARTESIAN_POINT('Ctrl Pts',(10.0514278971315,95.5812586277599,-3.26590689904296));
#280236=CARTESIAN_POINT('Ctrl Pts',(8.13177598651383,95.7312586277593,-5.9080810824151));
#280237=CARTESIAN_POINT('Ctrl Pts',(6.21212407589613,95.8812586277587,-8.55025526578723));
#280238=CARTESIAN_POINT('Ctrl Pts',(3.10606203794803,96.0312586277581,-9.55947599963789));
#280239=CARTESIAN_POINT('Ctrl Pts',(-6.85158535475064E-14,96.1812586277575,
-10.5686967334885));
#280240=CARTESIAN_POINT('Ctrl Pts',(-3.10606203794817,96.3312586277569,
-9.55947599963789));
#280241=CARTESIAN_POINT('Ctrl Pts',(-6.21212407589627,96.4812586277563,
-8.55025526578723));
#280242=CARTESIAN_POINT('Ctrl Pts',(-8.13177598651396,96.6312586277557,
-5.90808108241509));
#280243=CARTESIAN_POINT('Ctrl Pts',(-10.0514278971317,96.7812586277551,
-3.26590689904296));
#280244=CARTESIAN_POINT('Ctrl Pts',(-10.0514278971317,96.9312586277545,
2.46188980021652E-15));
#280245=CARTESIAN_POINT('Ctrl Pts',(-10.0514278971317,97.0812586277539,
3.26590689904296));
#280246=CARTESIAN_POINT('Ctrl Pts',(-8.13177598651396,97.2312586277533,
5.9080810824151));
#280247=CARTESIAN_POINT('Ctrl Pts',(-6.21212407589627,97.3812586277527,
8.55025526578723));
#280248=CARTESIAN_POINT('Ctrl Pts',(-3.10606203794817,97.5312586277521,
9.55947599963789));
#280249=CARTESIAN_POINT('Ctrl Pts',(-6.67911240581722E-14,97.6812586277515,
10.5686967334885));
#280250=CARTESIAN_POINT('Ctrl Pts',(3.10606203794803,97.8312586277509,9.55947599963789));
#280251=CARTESIAN_POINT('Ctrl Pts',(6.21212407589614,97.9812586277503,8.55025526578723));
#280252=CARTESIAN_POINT('Ctrl Pts',(8.13177598651382,98.1312586277497,5.90808108241509));
#280253=CARTESIAN_POINT('Ctrl Pts',(10.0514278971315,98.2812586277491,3.26590689904295));
#280254=CARTESIAN_POINT('Ctrl Pts',(10.0514278971315,98.4312586277485,-1.23094490010826E-15));
#280255=CARTESIAN_POINT('Ctrl Pts',(10.0514278971315,98.581258627748,-3.26590689904296));
#280256=CARTESIAN_POINT('Ctrl Pts',(8.13177598651382,98.7312586277473,-5.9080810824151));
#280257=CARTESIAN_POINT('Ctrl Pts',(6.21212407589613,98.8812586277467,-8.55025526578723));
#280258=CARTESIAN_POINT('Ctrl Pts',(3.10606203794803,99.0312586277461,-9.55947599963789));
#280259=CARTESIAN_POINT('Ctrl Pts',(-7.02435628191682E-14,99.1812586277455,
-10.5686967334885));
#280260=CARTESIAN_POINT('Ctrl Pts',(-3.10606203794817,99.3312586277449,
-9.55947599963789));
#280261=CARTESIAN_POINT('Ctrl Pts',(-6.21212407589627,99.4812586277443,
-8.55025526578723));
#280262=CARTESIAN_POINT('Ctrl Pts',(-8.13177598651396,99.6312586277437,
-5.90808108241509));
#280263=CARTESIAN_POINT('Ctrl Pts',(-10.0514278971317,99.7812586277431,
-3.26590689904296));
#280264=CARTESIAN_POINT('Ctrl Pts',(-10.0514278971317,99.9312586277425,
2.46188980021652E-15));
#280265=CARTESIAN_POINT('Ctrl Pts',(-10.0514278971317,100.081258627742,
3.26590689904296));
#280266=CARTESIAN_POINT('Ctrl Pts',(-8.13177598651396,100.231258627741,
5.9080810824151));
#280267=CARTESIAN_POINT('Ctrl Pts',(-6.21212407589627,100.381258627741,
8.55025526578723));
#280268=CARTESIAN_POINT('Ctrl Pts',(-3.10606203794817,100.53125862774,9.55947599963789));
#280269=CARTESIAN_POINT('Ctrl Pts',(-6.8518833329834E-14,100.681258627739,
10.5686967334885));
#280270=CARTESIAN_POINT('Ctrl Pts',(3.10606203794803,100.831258627739,9.55947599963789));
#280271=CARTESIAN_POINT('Ctrl Pts',(6.21212407589613,100.981258627738,8.55025526578723));
#280272=CARTESIAN_POINT('Ctrl Pts',(8.13177598651382,101.131258627738,5.90808108241509));
#280273=CARTESIAN_POINT('Ctrl Pts',(10.0514278971315,101.281258627737,3.26590689904295));
#280274=CARTESIAN_POINT('Ctrl Pts',(10.0514278971315,101.431258627737,-1.23094490010826E-15));
#280275=CARTESIAN_POINT('Ctrl Pts',(10.0514278971315,101.581258627736,-3.26590689904296));
#280276=CARTESIAN_POINT('Ctrl Pts',(8.13177598651382,101.731258627735,-5.9080810824151));
#280277=CARTESIAN_POINT('Ctrl Pts',(6.21212407589613,101.881258627735,-8.55025526578723));
#280278=CARTESIAN_POINT('Ctrl Pts',(3.10606203794803,102.031258627734,-9.55947599963789));
#280279=CARTESIAN_POINT('Ctrl Pts',(-7.19712720908301E-14,102.181258627733,
-10.5686967334885));
#280280=CARTESIAN_POINT('Ctrl Pts',(-3.10606203794817,102.331258627733,
-9.55947599963789));
#280281=CARTESIAN_POINT('Ctrl Pts',(-6.21212407589628,102.481258627732,
-8.55025526578723));
#280282=CARTESIAN_POINT('Ctrl Pts',(-8.13177598651397,102.631258627732,
-5.90808108241509));
#280283=CARTESIAN_POINT('Ctrl Pts',(-10.0514278971317,102.781258627731,
-3.26590689904296));
#280284=CARTESIAN_POINT('Ctrl Pts',(-10.0514278971317,102.931258627731,
2.46188980021652E-15));
#280285=CARTESIAN_POINT('Ctrl Pts',(-10.0514278971317,103.08125862773,3.26590689904296));
#280286=CARTESIAN_POINT('Ctrl Pts',(-8.13177598651397,103.231258627729,
5.9080810824151));
#280287=CARTESIAN_POINT('Ctrl Pts',(-6.21212407589627,103.381258627729,
8.55025526578723));
#280288=CARTESIAN_POINT('Ctrl Pts',(-3.10606203794817,103.531258627728,
9.55947599963789));
#280289=CARTESIAN_POINT('Ctrl Pts',(-7.02465426014958E-14,103.681258627728,
10.5686967334885));
#280290=CARTESIAN_POINT('Ctrl Pts',(3.10606203794803,103.831258627727,9.55947599963789));
#280291=CARTESIAN_POINT('Ctrl Pts',(6.21212407589613,103.981258627726,8.55025526578723));
#280292=CARTESIAN_POINT('Ctrl Pts',(8.13177598651382,104.131258627726,5.90808108241509));
#280293=CARTESIAN_POINT('Ctrl Pts',(10.0514278971315,104.281258627725,3.26590689904295));
#280294=CARTESIAN_POINT('Ctrl Pts',(10.0514278971315,104.431258627725,-1.23094490010826E-15));
#280295=CARTESIAN_POINT('Ctrl Pts',(10.0514278971315,104.581258627724,-3.26590689904296));
#280296=CARTESIAN_POINT('Ctrl Pts',(8.13177598651382,104.731258627723,-5.9080810824151));
#280297=CARTESIAN_POINT('Ctrl Pts',(6.21212407589613,104.881258627723,-8.55025526578723));
#280298=CARTESIAN_POINT('Ctrl Pts',(3.10606203794803,105.031258627722,-9.55947599963789));
#280299=CARTESIAN_POINT('Ctrl Pts',(-7.36989813624919E-14,105.181258627722,
-10.5686967334885));
#280300=CARTESIAN_POINT('Ctrl Pts',(-3.10606203794818,105.331258627721,
-9.55947599963789));
#280301=CARTESIAN_POINT('Ctrl Pts',(-6.21212407589628,105.48125862772,-8.55025526578723));
#280302=CARTESIAN_POINT('Ctrl Pts',(-8.13177598651397,105.63125862772,-5.90808108241509));
#280303=CARTESIAN_POINT('Ctrl Pts',(-10.0514278971317,105.781258627719,
-3.26590689904296));
#280304=CARTESIAN_POINT('Ctrl Pts',(-10.0514278971317,105.931258627719,
2.46188980021652E-15));
#280305=CARTESIAN_POINT('Ctrl Pts',(-10.0514278971317,106.081258627718,
3.26590689904296));
#280306=CARTESIAN_POINT('Ctrl Pts',(-8.13177598651397,106.231258627717,
5.9080810824151));
#280307=CARTESIAN_POINT('Ctrl Pts',(-6.21212407589628,106.381258627717,
8.55025526578723));
#280308=CARTESIAN_POINT('Ctrl Pts',(-3.10606203794817,106.531258627716,
9.55947599963789));
#280309=CARTESIAN_POINT('Ctrl Pts',(-7.19742518731577E-14,106.681258627715,
10.5686967334885));
#280310=CARTESIAN_POINT('Ctrl Pts',(3.10606203794803,106.831258627715,9.55947599963789));
#280311=CARTESIAN_POINT('Ctrl Pts',(6.21212407589613,106.981258627714,8.55025526578723));
#280312=CARTESIAN_POINT('Ctrl Pts',(8.13177598651382,107.131258627714,5.90808108241509));
#280313=CARTESIAN_POINT('Ctrl Pts',(10.0514278971315,107.281258627713,3.26590689904295));
#280314=CARTESIAN_POINT('Ctrl Pts',(10.0514278971315,107.431258627713,-1.23094490010826E-15));
#280315=CARTESIAN_POINT('Ctrl Pts',(10.0514278971315,107.581258627712,-3.26590689904296));
#280316=CARTESIAN_POINT('Ctrl Pts',(8.13177598651382,107.731258627711,-5.9080810824151));
#280317=CARTESIAN_POINT('Ctrl Pts',(6.21212407589613,107.881258627711,-8.55025526578723));
#280318=CARTESIAN_POINT('Ctrl Pts',(3.10606203794803,108.03125862771,-9.55947599963789));
#280319=CARTESIAN_POINT('Ctrl Pts',(-7.54266906341537E-14,108.18125862771,
-10.5686967334885));
#280320=CARTESIAN_POINT('Ctrl Pts',(-3.10606203794818,108.331258627709,
-9.55947599963789));
#280321=CARTESIAN_POINT('Ctrl Pts',(-6.21212407589628,108.481258627708,
-8.55025526578723));
#280322=CARTESIAN_POINT('Ctrl Pts',(-8.13177598651397,108.631258627708,
-5.90808108241509));
#280323=CARTESIAN_POINT('Ctrl Pts',(-10.0514278971317,108.781258627707,
-3.26590689904296));
#280324=CARTESIAN_POINT('Ctrl Pts',(-10.0514278971317,108.931258627707,
2.46188980021652E-15));
#280325=CARTESIAN_POINT('Ctrl Pts',(-10.0514278971317,109.081258627706,
3.26590689904296));
#280326=CARTESIAN_POINT('Ctrl Pts',(-8.13177598651397,109.231258627705,
5.9080810824151));
#280327=CARTESIAN_POINT('Ctrl Pts',(-6.21212407589628,109.381258627705,
8.55025526578723));
#280328=CARTESIAN_POINT('Ctrl Pts',(-3.10606203794818,109.531258627704,
9.55947599963789));
#280329=CARTESIAN_POINT('Ctrl Pts',(-7.37019611448195E-14,109.681258627703,
10.5686967334885));
#280330=CARTESIAN_POINT('Ctrl Pts',(3.10606203794803,109.831258627703,9.55947599963789));
#280331=CARTESIAN_POINT('Ctrl Pts',(6.21212407589613,109.981258627702,8.55025526578723));
#280332=CARTESIAN_POINT('Ctrl Pts',(8.13177598651382,110.131258627702,5.90808108241509));
#280333=CARTESIAN_POINT('Ctrl Pts',(10.0514278971315,110.281258627701,3.26590689904295));
#280334=CARTESIAN_POINT('Ctrl Pts',(10.0514278971315,110.431258627701,-1.23094490010826E-15));
#280335=CARTESIAN_POINT('Ctrl Pts',(10.0514278971315,110.5812586277,-3.26590689904296));
#280336=CARTESIAN_POINT('Ctrl Pts',(8.13177598651382,110.731258627699,-5.9080810824151));
#280337=CARTESIAN_POINT('Ctrl Pts',(6.21212407589613,110.881258627699,-8.55025526578723));
#280338=CARTESIAN_POINT('Ctrl Pts',(3.10606203794803,111.031258627698,-9.55947599963789));
#280339=CARTESIAN_POINT('Ctrl Pts',(-7.71543999058156E-14,111.181258627698,
-10.5686967334885));
#280340=CARTESIAN_POINT('Ctrl Pts',(-3.10606203794818,111.331258627697,
-9.55947599963789));
#280341=CARTESIAN_POINT('Ctrl Pts',(-6.21212407589628,111.481258627696,
-8.55025526578723));
#280342=CARTESIAN_POINT('Ctrl Pts',(-8.13177598651397,111.631258627696,
-5.90808108241509));
#280343=CARTESIAN_POINT('Ctrl Pts',(-10.0514278971317,111.781258627695,
-3.26590689904296));
#280344=CARTESIAN_POINT('Ctrl Pts',(-10.0514278971317,111.931258627695,
2.46188980021652E-15));
#280345=CARTESIAN_POINT('Ctrl Pts',(-10.0514278971317,112.081258627694,
3.26590689904296));
#280346=CARTESIAN_POINT('Ctrl Pts',(-8.13177598651397,112.231258627693,
5.9080810824151));
#280347=CARTESIAN_POINT('Ctrl Pts',(-6.21212407589628,112.381258627693,
8.55025526578723));
#280348=CARTESIAN_POINT('Ctrl Pts',(-3.10606203794818,112.531258627692,
9.55947599963789));
#280349=CARTESIAN_POINT('Ctrl Pts',(-7.54296704164813E-14,112.681258627692,
10.5686967334885));
#280350=CARTESIAN_POINT('Ctrl Pts',(3.10606203794803,112.831258627691,9.55947599963789));
#280351=CARTESIAN_POINT('Ctrl Pts',(6.21212407589613,112.98125862769,8.55025526578723));
#280352=CARTESIAN_POINT('Ctrl Pts',(8.13177598651382,113.13125862769,5.90808108241509));
#280353=CARTESIAN_POINT('Ctrl Pts',(10.0514278971315,113.281258627689,3.26590689904295));
#280354=CARTESIAN_POINT('Ctrl Pts',(10.0514278971315,113.431258627689,-1.23094490010826E-15));
#280355=CARTESIAN_POINT('Ctrl Pts',(10.0514278971315,113.581258627688,-3.26590689904296));
#280356=CARTESIAN_POINT('Ctrl Pts',(8.13177598651382,113.731258627687,-5.9080810824151));
#280357=CARTESIAN_POINT('Ctrl Pts',(6.21212407589613,113.881258627687,-8.55025526578723));
#280358=CARTESIAN_POINT('Ctrl Pts',(3.10606203794802,114.031258627686,-9.55947599963789));
#280359=CARTESIAN_POINT('Ctrl Pts',(-7.88821091774774E-14,114.181258627685,
-10.5686967334885));
#280360=CARTESIAN_POINT('Ctrl Pts',(-3.10606203794818,114.331258627685,
-9.55947599963789));
#280361=CARTESIAN_POINT('Ctrl Pts',(-6.21212407589628,114.481258627684,
-8.55025526578723));
#280362=CARTESIAN_POINT('Ctrl Pts',(-8.13177598651397,114.631258627684,
-5.90808108241509));
#280363=CARTESIAN_POINT('Ctrl Pts',(-10.0514278971317,114.781258627683,
-3.26590689904296));
#280364=CARTESIAN_POINT('Ctrl Pts',(-10.0514278971317,114.931258627683,
2.46188980021652E-15));
#280365=CARTESIAN_POINT('Ctrl Pts',(-10.0514278971317,115.081258627682,
3.26590689904296));
#280366=CARTESIAN_POINT('Ctrl Pts',(-8.13177598651397,115.231258627681,
5.9080810824151));
#280367=CARTESIAN_POINT('Ctrl Pts',(-6.21212407589628,115.381258627681,
8.55025526578723));
#280368=CARTESIAN_POINT('Ctrl Pts',(-3.10606203794818,115.53125862768,9.55947599963789));
#280369=CARTESIAN_POINT('Ctrl Pts',(-7.71573796881432E-14,115.681258627679,
10.5686967334885));
#280370=CARTESIAN_POINT('Ctrl Pts',(3.10606203794802,115.831258627679,9.55947599963789));
#280371=CARTESIAN_POINT('Ctrl Pts',(6.21212407589613,115.981258627678,8.55025526578723));
#280372=CARTESIAN_POINT('Ctrl Pts',(8.13177598651382,116.131258627678,5.90808108241509));
#280373=CARTESIAN_POINT('Ctrl Pts',(10.0514278971315,116.281258627677,3.26590689904295));
#280374=CARTESIAN_POINT('Ctrl Pts',(10.0514278971315,116.431258627676,-1.23094490010826E-15));
#280375=CARTESIAN_POINT('Ctrl Pts',(10.0514278971315,116.581258627676,-3.26590689904296));
#280376=CARTESIAN_POINT('Ctrl Pts',(8.13177598651382,116.731258627675,-5.9080810824151));
#280377=CARTESIAN_POINT('Ctrl Pts',(6.21212407589612,116.881258627675,-8.55025526578723));
#280378=CARTESIAN_POINT('Ctrl Pts',(3.10606203794802,117.031258627674,-9.55947599963789));
#280379=CARTESIAN_POINT('Ctrl Pts',(-8.06098184491393E-14,117.181258627674,
-10.5686967334885));
#280380=CARTESIAN_POINT('Ctrl Pts',(-3.10606203794818,117.331258627673,
-9.55947599963789));
#280381=CARTESIAN_POINT('Ctrl Pts',(-6.21212407589629,117.481258627672,
-8.55025526578723));
#280382=CARTESIAN_POINT('Ctrl Pts',(-8.13177598651398,117.631258627672,
-5.90808108241509));
#280383=CARTESIAN_POINT('Ctrl Pts',(-10.0514278971317,117.781258627671,
-3.26590689904296));
#280384=CARTESIAN_POINT('Ctrl Pts',(-10.0514278971317,117.931258627671,
2.46188980021652E-15));
#280385=CARTESIAN_POINT('Ctrl Pts',(-10.0514278971317,118.08125862767,3.26590689904296));
#280386=CARTESIAN_POINT('Ctrl Pts',(-8.13177598651398,118.231258627669,
5.9080810824151));
#280387=CARTESIAN_POINT('Ctrl Pts',(-6.21212407589628,118.381258627669,
8.55025526578723));
#280388=CARTESIAN_POINT('Ctrl Pts',(-3.10606203794818,118.531258627668,
9.55947599963789));
#280389=CARTESIAN_POINT('Ctrl Pts',(-7.8885088959805E-14,118.681258627667,
10.5686967334885));
#280390=CARTESIAN_POINT('Ctrl Pts',(3.10606203794802,118.831258627667,9.55947599963789));
#280391=CARTESIAN_POINT('Ctrl Pts',(6.21212407589613,118.981258627666,8.55025526578723));
#280392=CARTESIAN_POINT('Ctrl Pts',(8.13177598651381,119.131258627666,5.90808108241509));
#280393=CARTESIAN_POINT('Ctrl Pts',(10.0514278971315,119.281258627665,3.26590689904295));
#280394=CARTESIAN_POINT('Ctrl Pts',(10.0514278971315,119.431258627665,-1.23094490010826E-15));
#280395=CARTESIAN_POINT('Ctrl Pts',(10.0514278971315,119.581258627664,-3.26590689904296));
#280396=CARTESIAN_POINT('Ctrl Pts',(8.13177598651381,119.731258627663,-5.9080810824151));
#280397=CARTESIAN_POINT('Ctrl Pts',(6.21212407589612,119.881258627663,-8.55025526578723));
#280398=CARTESIAN_POINT('Ctrl Pts',(3.10606203794802,120.031258627662,-9.55947599963789));
#280399=CARTESIAN_POINT('Ctrl Pts',(-8.23375277208011E-14,120.181258627662,
-10.5686967334885));
#280400=CARTESIAN_POINT('Ctrl Pts',(-3.10606203794818,120.331258627661,
-9.55947599963789));
#280401=CARTESIAN_POINT('Ctrl Pts',(-6.21212407589629,120.48125862766,-8.55025526578723));
#280402=CARTESIAN_POINT('Ctrl Pts',(-8.13177598651398,120.63125862766,-5.90808108241509));
#280403=CARTESIAN_POINT('Ctrl Pts',(-10.0514278971317,120.781258627659,
-3.26590689904296));
#280404=CARTESIAN_POINT('Ctrl Pts',(-10.0514278971317,120.931258627659,
2.46188980021652E-15));
#280405=CARTESIAN_POINT('Ctrl Pts',(-10.0514278971317,121.081258627658,
3.26590689904296));
#280406=CARTESIAN_POINT('Ctrl Pts',(-8.13177598651398,121.231258627657,
5.9080810824151));
#280407=CARTESIAN_POINT('Ctrl Pts',(-6.21212407589629,121.381258627657,
8.55025526578723));
#280408=CARTESIAN_POINT('Ctrl Pts',(-3.10606203794818,121.531258627656,
9.55947599963789));
#280409=CARTESIAN_POINT('Ctrl Pts',(-8.06127982314669E-14,121.681258627655,
10.5686967334885));
#280410=CARTESIAN_POINT('Ctrl Pts',(3.10606203794802,121.831258627655,9.55947599963789));
#280411=CARTESIAN_POINT('Ctrl Pts',(6.21212407589612,121.981258627654,8.55025526578723));
#280412=CARTESIAN_POINT('Ctrl Pts',(8.13177598651381,122.131258627654,5.90808108241509));
#280413=CARTESIAN_POINT('Ctrl Pts',(10.0514278971315,122.281258627653,3.26590689904295));
#280414=CARTESIAN_POINT('Ctrl Pts',(10.0514278971315,122.431258627653,-1.23094490010826E-15));
#280415=CARTESIAN_POINT('Ctrl Pts',(10.0514278971315,122.581258627652,-3.26590689904296));
#280416=CARTESIAN_POINT('Ctrl Pts',(8.13177598651381,122.731258627651,-5.9080810824151));
#280417=CARTESIAN_POINT('Ctrl Pts',(6.21212407589612,122.881258627651,-8.55025526578723));
#280418=CARTESIAN_POINT('Ctrl Pts',(3.10606203794802,123.03125862765,-9.55947599963789));
#280419=CARTESIAN_POINT('Ctrl Pts',(-8.40652369924629E-14,123.181258627649,
-10.5686967334885));
#280420=CARTESIAN_POINT('Ctrl Pts',(-3.10606203794819,123.331258627649,
-9.55947599963789));
#280421=CARTESIAN_POINT('Ctrl Pts',(-6.21212407589629,123.481258627648,
-8.55025526578723));
#280422=CARTESIAN_POINT('Ctrl Pts',(-8.13177598651398,123.631258627648,
-5.90808108241509));
#280423=CARTESIAN_POINT('Ctrl Pts',(-10.0514278971317,123.781258627647,
-3.26590689904296));
#280424=CARTESIAN_POINT('Ctrl Pts',(-10.0514278971317,123.931258627646,
2.46188980021652E-15));
#280425=CARTESIAN_POINT('Ctrl Pts',(-10.0514278971317,124.081258627646,
3.26590689904296));
#280426=CARTESIAN_POINT('Ctrl Pts',(-8.13177598651398,124.231258627645,
5.9080810824151));
#280427=CARTESIAN_POINT('Ctrl Pts',(-6.21212407589629,124.381258627645,
8.55025526578723));
#280428=CARTESIAN_POINT('Ctrl Pts',(-3.10606203794818,124.531258627644,
9.55947599963789));
#280429=CARTESIAN_POINT('Ctrl Pts',(-8.23405075031287E-14,124.681258627644,
10.5686967334885));
#280430=CARTESIAN_POINT('Ctrl Pts',(3.10606203794802,124.831258627643,9.55947599963789));
#280431=CARTESIAN_POINT('Ctrl Pts',(6.21212407589612,124.981258627642,8.55025526578723));
#280432=CARTESIAN_POINT('Ctrl Pts',(8.13177598651381,125.131258627642,5.90808108241509));
#280433=CARTESIAN_POINT('Ctrl Pts',(10.0514278971315,125.281258627641,3.26590689904295));
#280434=CARTESIAN_POINT('Ctrl Pts',(10.0514278971315,125.431258627641,-1.23094490010826E-15));
#280435=CARTESIAN_POINT('Ctrl Pts',(10.0514278971315,125.58125862764,-3.26590689904296));
#280436=CARTESIAN_POINT('Ctrl Pts',(8.13177598651381,125.731258627639,-5.9080810824151));
#280437=CARTESIAN_POINT('Ctrl Pts',(6.21212407589612,125.881258627639,-8.55025526578723));
#280438=CARTESIAN_POINT('Ctrl Pts',(3.10606203794802,126.031258627638,-9.55947599963789));
#280439=CARTESIAN_POINT('Ctrl Pts',(-8.57929462641248E-14,126.181258627637,
-10.5686967334885));
#280440=CARTESIAN_POINT('Ctrl Pts',(-3.10606203794819,126.331258627637,
-9.55947599963789));
#280441=CARTESIAN_POINT('Ctrl Pts',(-6.21212407589629,126.481258627636,
-8.55025526578723));
#280442=CARTESIAN_POINT('Ctrl Pts',(-8.13177598651398,126.631258627636,
-5.90808108241509));
#280443=CARTESIAN_POINT('Ctrl Pts',(-10.0514278971317,126.781258627635,
-3.26590689904296));
#280444=CARTESIAN_POINT('Ctrl Pts',(-10.0514278971317,126.931258627634,
2.46188980021652E-15));
#280445=CARTESIAN_POINT('Ctrl Pts',(-10.0514278971317,127.081258627634,
3.26590689904296));
#280446=CARTESIAN_POINT('Ctrl Pts',(-8.13177598651398,127.231258627633,
5.9080810824151));
#280447=CARTESIAN_POINT('Ctrl Pts',(-6.21212407589629,127.381258627633,
8.55025526578723));
#280448=CARTESIAN_POINT('Ctrl Pts',(-3.10606203794819,127.531258627632,
9.55947599963789));
#280449=CARTESIAN_POINT('Ctrl Pts',(-8.40682167747905E-14,127.681258627631,
10.5686967334885));
#280450=CARTESIAN_POINT('Ctrl Pts',(3.10606203794802,127.831258627631,9.55947599963789));
#280451=CARTESIAN_POINT('Ctrl Pts',(6.21212407589612,127.98125862763,8.55025526578723));
#280452=CARTESIAN_POINT('Ctrl Pts',(8.13177598651381,128.13125862763,5.90808108241509));
#280453=CARTESIAN_POINT('Ctrl Pts',(10.0514278971315,128.281258627629,3.26590689904295));
#280454=CARTESIAN_POINT('Ctrl Pts',(10.0514278971315,128.431258627629,-1.23094490010826E-15));
#280455=CARTESIAN_POINT('Ctrl Pts',(10.0514278971315,128.581258627628,-3.26590689904296));
#280456=CARTESIAN_POINT('Ctrl Pts',(8.13177598651381,128.731258627627,-5.9080810824151));
#280457=CARTESIAN_POINT('Ctrl Pts',(6.21212407589612,128.881258627627,-8.55025526578723));
#280458=CARTESIAN_POINT('Ctrl Pts',(3.10606203794801,129.031258627626,-9.55947599963789));
#280459=CARTESIAN_POINT('Ctrl Pts',(-8.75206555357867E-14,129.181258627626,
-10.5686967334885));
#280460=CARTESIAN_POINT('Ctrl Pts',(-3.10606203794819,129.331258627625,
-9.55947599963789));
#280461=CARTESIAN_POINT('Ctrl Pts',(-6.21212407589629,129.481258627624,
-8.55025526578723));
#280462=CARTESIAN_POINT('Ctrl Pts',(-8.13177598651398,129.631258627624,
-5.90808108241509));
#280463=CARTESIAN_POINT('Ctrl Pts',(-10.0514278971317,129.781258627623,
-3.26590689904296));
#280464=CARTESIAN_POINT('Ctrl Pts',(-10.0514278971317,129.931258627622,
2.46188980021652E-15));
#280465=CARTESIAN_POINT('Ctrl Pts',(-10.0514278971317,130.081258627622,
3.26590689904296));
#280466=CARTESIAN_POINT('Ctrl Pts',(-8.13177598651398,130.231258627621,
5.9080810824151));
#280467=CARTESIAN_POINT('Ctrl Pts',(-6.21212407589629,130.381258627621,
8.55025526578723));
#280468=CARTESIAN_POINT('Ctrl Pts',(-3.10606203794819,130.53125862762,9.55947599963789));
#280469=CARTESIAN_POINT('Ctrl Pts',(-8.57959260464524E-14,130.681258627619,
10.5686967334885));
#280470=CARTESIAN_POINT('Ctrl Pts',(3.10606203794802,130.831258627619,9.55947599963789));
#280471=CARTESIAN_POINT('Ctrl Pts',(6.21212407589612,130.981258627618,8.55025526578723));
#280472=CARTESIAN_POINT('Ctrl Pts',(8.13177598651381,131.131258627618,5.90808108241509));
#280473=CARTESIAN_POINT('Ctrl Pts',(10.0514278971315,131.281258627617,3.26590689904295));
#280474=CARTESIAN_POINT('Ctrl Pts',(10.0514278971315,131.431258627617,-1.23094490010826E-15));
#280475=CARTESIAN_POINT('Ctrl Pts',(10.0514278971315,131.581258627616,-3.26590689904296));
#280476=CARTESIAN_POINT('Ctrl Pts',(8.13177598651381,131.731258627615,-5.9080810824151));
#280477=CARTESIAN_POINT('Ctrl Pts',(6.21212407589611,131.881258627615,-8.55025526578723));
#280478=CARTESIAN_POINT('Ctrl Pts',(3.10606203794801,132.031258627614,-9.55947599963789));
#280479=CARTESIAN_POINT('Ctrl Pts',(-8.92483648074485E-14,132.181258627614,
-10.5686967334885));
#280480=CARTESIAN_POINT('Ctrl Pts',(-3.10606203794819,132.331258627613,
-9.55947599963789));
#280481=CARTESIAN_POINT('Ctrl Pts',(-6.21212407589629,132.481258627612,
-8.55025526578723));
#280482=CARTESIAN_POINT('Ctrl Pts',(-8.13177598651398,132.631258627612,
-5.90808108241509));
#280483=CARTESIAN_POINT('Ctrl Pts',(-10.0514278971317,132.781258627611,
-3.26590689904296));
#280484=CARTESIAN_POINT('Ctrl Pts',(-10.0514278971317,132.93125862761,2.46188980021652E-15));
#280485=CARTESIAN_POINT('Ctrl Pts',(-10.0514278971317,133.08125862761,3.26590689904296));
#280486=CARTESIAN_POINT('Ctrl Pts',(-8.13177598651398,133.231258627609,
5.9080810824151));
#280487=CARTESIAN_POINT('Ctrl Pts',(-6.21212407589629,133.381258627609,
8.55025526578723));
#280488=CARTESIAN_POINT('Ctrl Pts',(-3.10606203794819,133.531258627608,
9.55947599963789));
#280489=CARTESIAN_POINT('Ctrl Pts',(-8.75236353181142E-14,133.681258627607,
10.5686967334885));
#280490=CARTESIAN_POINT('Ctrl Pts',(3.10606203794801,133.831258627607,9.55947599963789));
#280491=CARTESIAN_POINT('Ctrl Pts',(6.21212407589612,133.981258627606,8.55025526578723));
#280492=CARTESIAN_POINT('Ctrl Pts',(8.13177598651381,134.131258627606,5.90808108241509));
#280493=CARTESIAN_POINT('Ctrl Pts',(10.0514278971315,134.281258627605,3.26590689904295));
#280494=CARTESIAN_POINT('Ctrl Pts',(10.0514278971315,134.431258627605,-1.23094490010826E-15));
#280495=CARTESIAN_POINT('Ctrl Pts',(10.0514278971315,134.581258627604,-3.26590689904296));
#280496=CARTESIAN_POINT('Ctrl Pts',(8.13177598651381,134.731258627603,-5.9080810824151));
#280497=CARTESIAN_POINT('Ctrl Pts',(6.21212407589611,134.881258627603,-8.55025526578723));
#280498=CARTESIAN_POINT('Ctrl Pts',(3.10606203794801,135.031258627602,-9.55947599963789));
#280499=CARTESIAN_POINT('Ctrl Pts',(-9.09760740791103E-14,135.181258627601,
-10.5686967334885));
#280500=CARTESIAN_POINT('Ctrl Pts',(-3.10606203794819,135.331258627601,
-9.55947599963789));
#280501=CARTESIAN_POINT('Ctrl Pts',(-6.21212407589629,135.4812586276,-8.55025526578723));
#280502=CARTESIAN_POINT('Ctrl Pts',(-8.13177598651399,135.6312586276,-5.90808108241509));
#280503=CARTESIAN_POINT('Ctrl Pts',(-10.0514278971317,135.781258627599,
-3.26590689904296));
#280504=CARTESIAN_POINT('Ctrl Pts',(-10.0514278971317,135.931258627599,
2.46188980021652E-15));
#280505=CARTESIAN_POINT('Ctrl Pts',(-10.0514278971317,136.081258627598,
3.26590689904296));
#280506=CARTESIAN_POINT('Ctrl Pts',(-8.13177598651399,136.231258627597,
5.9080810824151));
#280507=CARTESIAN_POINT('Ctrl Pts',(-6.21212407589629,136.381258627597,
8.55025526578723));
#280508=CARTESIAN_POINT('Ctrl Pts',(-3.10606203794819,136.531258627596,
9.55947599963789));
#280509=CARTESIAN_POINT('Ctrl Pts',(-8.9251344589776E-14,136.681258627595,
10.5686967334885));
#280510=CARTESIAN_POINT('Ctrl Pts',(3.10606203794801,136.831258627595,9.55947599963789));
#280511=CARTESIAN_POINT('Ctrl Pts',(6.21212407589611,136.981258627594,8.55025526578723));
#280512=CARTESIAN_POINT('Ctrl Pts',(8.1317759865138,137.131258627594,5.90808108241509));
#280513=CARTESIAN_POINT('Ctrl Pts',(10.0514278971315,137.281258627593,3.26590689904295));
#280514=CARTESIAN_POINT('Ctrl Pts',(10.0514278971315,137.431258627593,-1.23094490010826E-15));
#280515=CARTESIAN_POINT('Ctrl Pts',(10.0514278971315,137.581258627592,-3.26590689904296));
#280516=CARTESIAN_POINT('Ctrl Pts',(8.1317759865138,137.731258627591,-5.9080810824151));
#280517=CARTESIAN_POINT('Ctrl Pts',(6.21212407589611,137.881258627591,-8.55025526578723));
#280518=CARTESIAN_POINT('Ctrl Pts',(3.10606203794801,138.03125862759,-9.55947599963789));
#280519=CARTESIAN_POINT('Ctrl Pts',(-9.27037833507721E-14,138.18125862759,
-10.5686967334885));
#280520=CARTESIAN_POINT('Ctrl Pts',(-3.10606203794819,138.331258627589,
-9.55947599963789));
#280521=CARTESIAN_POINT('Ctrl Pts',(-6.2121240758963,138.481258627588,-8.55025526578723));
#280522=CARTESIAN_POINT('Ctrl Pts',(-8.13177598651399,138.631258627588,
-5.90808108241509));
#280523=CARTESIAN_POINT('Ctrl Pts',(-10.0514278971317,138.781258627587,
-3.26590689904296));
#280524=CARTESIAN_POINT('Ctrl Pts',(-10.0514278971317,138.931258627586,
2.46188980021652E-15));
#280525=CARTESIAN_POINT('Ctrl Pts',(-10.0514278971317,139.081258627586,
3.26590689904296));
#280526=CARTESIAN_POINT('Ctrl Pts',(-8.13177598651399,139.231258627585,
5.9080810824151));
#280527=CARTESIAN_POINT('Ctrl Pts',(-6.21212407589629,139.381258627585,
8.55025526578723));
#280528=CARTESIAN_POINT('Ctrl Pts',(-3.10606203794819,139.531258627584,
9.55947599963789));
#280529=CARTESIAN_POINT('Ctrl Pts',(-9.09790538614379E-14,139.681258627583,
10.5686967334885));
#280530=CARTESIAN_POINT('Ctrl Pts',(3.10606203794801,139.831258627583,9.55947599963789));
#280531=CARTESIAN_POINT('Ctrl Pts',(6.21212407589611,139.981258627582,8.55025526578723));
#280532=CARTESIAN_POINT('Ctrl Pts',(8.1317759865138,140.131258627582,5.90808108241509));
#280533=CARTESIAN_POINT('Ctrl Pts',(10.0514278971315,140.281258627581,3.26590689904295));
#280534=CARTESIAN_POINT('Ctrl Pts',(10.0514278971315,140.431258627581,-1.23094490010826E-15));
#280535=CARTESIAN_POINT('Ctrl Pts',(10.0514278971315,140.58125862758,-3.26590689904296));
#280536=CARTESIAN_POINT('Ctrl Pts',(8.1317759865138,140.731258627579,-5.9080810824151));
#280537=CARTESIAN_POINT('Ctrl Pts',(6.21212407589611,140.881258627579,-8.55025526578723));
#280538=CARTESIAN_POINT('Ctrl Pts',(3.10606203794801,141.031258627578,-9.55947599963789));
#280539=CARTESIAN_POINT('Ctrl Pts',(-9.4431492622434E-14,141.181258627577,
-10.5686967334885));
#280540=CARTESIAN_POINT('Ctrl Pts',(-3.1060620379482,141.331258627577,-9.55947599963789));
#280541=CARTESIAN_POINT('Ctrl Pts',(-6.2121240758963,141.481258627576,-8.55025526578723));
#280542=CARTESIAN_POINT('Ctrl Pts',(-8.13177598651399,141.631258627576,
-5.90808108241509));
#280543=CARTESIAN_POINT('Ctrl Pts',(-10.0514278971317,141.781258627575,
-3.26590689904296));
#280544=CARTESIAN_POINT('Ctrl Pts',(-10.0514278971317,141.931258627574,
2.46188980021652E-15));
#280545=CARTESIAN_POINT('Ctrl Pts',(-10.0514278971317,142.081258627574,
3.26590689904296));
#280546=CARTESIAN_POINT('Ctrl Pts',(-8.13177598651399,142.231258627573,
5.9080810824151));
#280547=CARTESIAN_POINT('Ctrl Pts',(-6.2121240758963,142.381258627573,8.55025526578723));
#280548=CARTESIAN_POINT('Ctrl Pts',(-3.10606203794819,142.531258627572,
9.55947599963789));
#280549=CARTESIAN_POINT('Ctrl Pts',(-9.27067631330997E-14,142.681258627572,
10.5686967334885));
#280550=CARTESIAN_POINT('Ctrl Pts',(3.10606203794801,142.831258627571,9.55947599963789));
#280551=CARTESIAN_POINT('Ctrl Pts',(6.21212407589611,142.98125862757,8.55025526578723));
#280552=CARTESIAN_POINT('Ctrl Pts',(8.1317759865138,143.13125862757,5.90808108241509));
#280553=CARTESIAN_POINT('Ctrl Pts',(10.0514278971315,143.281258627569,3.26590689904295));
#280554=CARTESIAN_POINT('Ctrl Pts',(10.0514278971315,143.431258627569,-1.23094490010826E-15));
#280555=CARTESIAN_POINT('Ctrl Pts',(10.0514278971315,143.581258627568,-3.26590689904296));
#280556=CARTESIAN_POINT('Ctrl Pts',(8.1317759865138,143.731258627567,-5.9080810824151));
#280557=CARTESIAN_POINT('Ctrl Pts',(6.21212407589611,143.881258627567,-8.55025526578723));
#280558=CARTESIAN_POINT('Ctrl Pts',(3.10606203794801,144.031258627566,-9.55947599963789));
#280559=CARTESIAN_POINT('Ctrl Pts',(-9.61592018940958E-14,144.181258627565,
-10.5686967334885));
#280560=CARTESIAN_POINT('Ctrl Pts',(-3.1060620379482,144.331258627565,-9.55947599963789));
#280561=CARTESIAN_POINT('Ctrl Pts',(-6.2121240758963,144.481258627564,-8.55025526578723));
#280562=CARTESIAN_POINT('Ctrl Pts',(-8.13177598651399,144.631258627564,
-5.90808108241509));
#280563=CARTESIAN_POINT('Ctrl Pts',(-10.0514278971317,144.781258627563,
-3.26590689904296));
#280564=CARTESIAN_POINT('Ctrl Pts',(-10.0514278971317,144.931258627562,
2.46188980021652E-15));
#280565=CARTESIAN_POINT('Ctrl Pts',(-10.0514278971317,145.081258627562,
3.26590689904296));
#280566=CARTESIAN_POINT('Ctrl Pts',(-8.13177598651399,145.231258627561,
5.9080810824151));
#280567=CARTESIAN_POINT('Ctrl Pts',(-6.2121240758963,145.381258627561,8.55025526578723));
#280568=CARTESIAN_POINT('Ctrl Pts',(-3.1060620379482,145.53125862756,9.55947599963789));
#280569=CARTESIAN_POINT('Ctrl Pts',(-9.44344724047616E-14,145.681258627559,
10.5686967334885));
#280570=CARTESIAN_POINT('Ctrl Pts',(3.10606203794801,145.831258627559,9.55947599963789));
#280571=CARTESIAN_POINT('Ctrl Pts',(6.21212407589611,145.981258627558,8.55025526578723));
#280572=CARTESIAN_POINT('Ctrl Pts',(8.1317759865138,146.131258627558,5.90808108241509));
#280573=CARTESIAN_POINT('Ctrl Pts',(10.0514278971315,146.281258627557,3.26590689904295));
#280574=CARTESIAN_POINT('Ctrl Pts',(10.0514278971315,146.431258627557,-1.23094490010826E-15));
#280575=CARTESIAN_POINT('Ctrl Pts',(10.0514278971315,146.581258627556,-3.26590689904296));
#280576=CARTESIAN_POINT('Ctrl Pts',(8.1317759865138,146.731258627555,-5.9080810824151));
#280577=CARTESIAN_POINT('Ctrl Pts',(6.2121240758961,146.881258627555,-8.55025526578723));
#280578=CARTESIAN_POINT('Ctrl Pts',(3.106062037948,147.031258627554,-9.55947599963789));
#280579=CARTESIAN_POINT('Ctrl Pts',(-9.78869111657577E-14,147.181258627553,
-10.5686967334885));
#280580=CARTESIAN_POINT('Ctrl Pts',(-3.1060620379482,147.331258627553,-9.55947599963789));
#280581=CARTESIAN_POINT('Ctrl Pts',(-6.2121240758963,147.481258627552,-8.55025526578723));
#280582=CARTESIAN_POINT('Ctrl Pts',(-8.13177598651399,147.631258627552,
-5.90808108241509));
#280583=CARTESIAN_POINT('Ctrl Pts',(-10.0514278971317,147.781258627551,
-3.26590689904296));
#280584=CARTESIAN_POINT('Ctrl Pts',(-10.0514278971317,147.931258627551,
2.46188980021652E-15));
#280585=CARTESIAN_POINT('Ctrl Pts',(-10.0514278971317,148.08125862755,3.26590689904296));
#280586=CARTESIAN_POINT('Ctrl Pts',(-8.13177598651399,148.231258627549,
5.9080810824151));
#280587=CARTESIAN_POINT('Ctrl Pts',(-6.2121240758963,148.381258627549,8.55025526578723));
#280588=CARTESIAN_POINT('Ctrl Pts',(-3.1060620379482,148.531258627548,9.55947599963789));
#280589=CARTESIAN_POINT('Ctrl Pts',(-9.61621816764234E-14,148.681258627547,
10.5686967334885));
#280590=CARTESIAN_POINT('Ctrl Pts',(3.10606203794801,148.831258627547,9.55947599963789));
#280591=CARTESIAN_POINT('Ctrl Pts',(6.21212407589611,148.981258627546,8.55025526578723));
#280592=CARTESIAN_POINT('Ctrl Pts',(8.1317759865138,149.131258627546,5.90808108241509));
#280593=CARTESIAN_POINT('Ctrl Pts',(10.0514278971315,149.281258627545,3.26590689904295));
#280594=CARTESIAN_POINT('Ctrl Pts',(10.0514278971315,149.431258627545,-1.23094490010826E-15));
#280595=CARTESIAN_POINT('Ctrl Pts',(10.0514278971315,149.581258627544,-3.26590689904296));
#280596=CARTESIAN_POINT('Ctrl Pts',(8.1317759865138,149.731258627543,-5.9080810824151));
#280597=CARTESIAN_POINT('Ctrl Pts',(6.2121240758961,149.881258627543,-8.55025526578723));
#280598=CARTESIAN_POINT('Ctrl Pts',(3.106062037948,150.031258627542,-9.55947599963789));
#280599=CARTESIAN_POINT('Ctrl Pts',(-9.96146204374195E-14,150.181258627541,
-10.5686967334885));
#280600=CARTESIAN_POINT('Ctrl Pts',(-3.1060620379482,150.331258627541,-9.55947599963789));
#280601=CARTESIAN_POINT('Ctrl Pts',(-6.2121240758963,150.48125862754,-8.55025526578723));
#280602=CARTESIAN_POINT('Ctrl Pts',(-8.131775986514,150.63125862754,-5.90808108241509));
#280603=CARTESIAN_POINT('Ctrl Pts',(-10.0514278971317,150.781258627539,
-3.26590689904296));
#280604=CARTESIAN_POINT('Ctrl Pts',(-10.0514278971317,150.931258627538,
2.46188980021652E-15));
#280605=CARTESIAN_POINT('Ctrl Pts',(-10.0514278971317,151.081258627538,
3.26590689904296));
#280606=CARTESIAN_POINT('Ctrl Pts',(-8.131775986514,151.231258627537,5.9080810824151));
#280607=CARTESIAN_POINT('Ctrl Pts',(-6.2121240758963,151.381258627537,8.55025526578723));
#280608=CARTESIAN_POINT('Ctrl Pts',(-3.1060620379482,151.531258627536,9.55947599963789));
#280609=CARTESIAN_POINT('Ctrl Pts',(-9.78898909480853E-14,151.681258627535,
10.5686967334885));
#280610=CARTESIAN_POINT('Ctrl Pts',(3.106062037948,151.831258627535,9.55947599963789));
#280611=CARTESIAN_POINT('Ctrl Pts',(6.2121240758961,151.981258627534,8.55025526578723));
#280612=CARTESIAN_POINT('Ctrl Pts',(8.13177598651379,152.131258627534,5.90808108241509));
#280613=CARTESIAN_POINT('Ctrl Pts',(10.0514278971315,152.281258627533,3.26590689904295));
#280614=CARTESIAN_POINT('Ctrl Pts',(10.0514278971315,152.431258627532,-1.23094490010826E-15));
#280615=CARTESIAN_POINT('Ctrl Pts',(10.0514278971315,152.581258627532,-3.26590689904296));
#280616=CARTESIAN_POINT('Ctrl Pts',(8.13177598651379,152.731258627531,-5.9080810824151));
#280617=CARTESIAN_POINT('Ctrl Pts',(6.2121240758961,152.881258627531,-8.55025526578723));
#280618=CARTESIAN_POINT('Ctrl Pts',(3.106062037948,153.03125862753,-9.55947599963789));
#280619=CARTESIAN_POINT('Ctrl Pts',(-1.01342329709081E-13,153.181258627529,
-10.5686967334885));
#280620=CARTESIAN_POINT('Ctrl Pts',(-3.1060620379482,153.331258627529,-9.55947599963789));
#280621=CARTESIAN_POINT('Ctrl Pts',(10.0514428414941,95.4312499996288,-1.23094673026484E-15));
#280622=CARTESIAN_POINT('Ctrl Pts',(10.0514428414941,95.5812499996282,-3.26591175476071));
#280623=CARTESIAN_POINT('Ctrl Pts',(8.13178807675712,95.7312499996276,-5.90808986649102));
#280624=CARTESIAN_POINT('Ctrl Pts',(6.21213331202015,95.8812499996269,-8.55026797822134));
#280625=CARTESIAN_POINT('Ctrl Pts',(3.10606665601004,96.0312499996264,-9.5594902125713));
#280626=CARTESIAN_POINT('Ctrl Pts',(-6.85158495407089E-14,96.1812499996257,
-10.5687124469213));
#280627=CARTESIAN_POINT('Ctrl Pts',(-3.10606665601018,96.3312499996252,
-9.5594902125713));
#280628=CARTESIAN_POINT('Ctrl Pts',(-6.21213331202028,96.4812499996245,
-8.55026797822134));
#280629=CARTESIAN_POINT('Ctrl Pts',(-8.13178807675726,96.6312499996239,
-5.90808986649102));
#280630=CARTESIAN_POINT('Ctrl Pts',(-10.0514428414942,96.7812499996234,
-3.2659117547607));
#280631=CARTESIAN_POINT('Ctrl Pts',(-10.0514428414942,96.9312499996227,
2.46189346052968E-15));
#280632=CARTESIAN_POINT('Ctrl Pts',(-10.0514428414942,97.0812499996221,
3.26591175476071));
#280633=CARTESIAN_POINT('Ctrl Pts',(-8.13178807675726,97.2312499996215,
5.90808986649102));
#280634=CARTESIAN_POINT('Ctrl Pts',(-6.21213331202028,97.381249999621,8.55026797822134));
#280635=CARTESIAN_POINT('Ctrl Pts',(-3.10606665601017,97.5312499996203,
9.5594902125713));
#280636=CARTESIAN_POINT('Ctrl Pts',(-6.67911162026936E-14,97.6812499996198,
10.5687124469213));
#280637=CARTESIAN_POINT('Ctrl Pts',(3.10606665601004,97.8312499996191,9.5594902125713));
#280638=CARTESIAN_POINT('Ctrl Pts',(6.21213331202015,97.9812499996186,8.55026797822134));
#280639=CARTESIAN_POINT('Ctrl Pts',(8.13178807675712,98.1312499996179,5.90808986649102));
#280640=CARTESIAN_POINT('Ctrl Pts',(10.0514428414941,98.2812499996173,3.2659117547607));
#280641=CARTESIAN_POINT('Ctrl Pts',(10.0514428414941,98.4312499996168,-1.23094673026484E-15));
#280642=CARTESIAN_POINT('Origin',(-3.77475828372553E-14,-1.881249999982,
2.68644078414671E-15));
#280643=CARTESIAN_POINT('Origin',(-3.77475828372553E-14,-1.881249999982,
2.68644078414671E-15));
#280644=CARTESIAN_POINT('',(10.0514428414941,17.4312499999408,1.37532313762869E-15));
#280645=CARTESIAN_POINT('',(10.0514428414941,17.8062499999393,1.37376642080824E-15));
#280646=CARTESIAN_POINT('',(10.0514428414941,-1.881249999982,4.14193483802857E-15));
#280647=CARTESIAN_POINT('',(-7.47704554734297,18.9576928414942,-6.71753623576259));
#280648=CARTESIAN_POINT('Ctrl Pts',(10.0514428414941,17.8062499999393,-1.23094673026484E-15));
#280649=CARTESIAN_POINT('Ctrl Pts',(10.0514428414941,17.9562499999387,-3.26591175476071));
#280650=CARTESIAN_POINT('Ctrl Pts',(8.13178807675717,18.1062499999381,-5.90808986649102));
#280651=CARTESIAN_POINT('Ctrl Pts',(6.21213331202019,18.2562499999375,-8.55026797822134));
#280652=CARTESIAN_POINT('Ctrl Pts',(3.10606665601008,18.4062499999369,-9.5594902125713));
#280653=CARTESIAN_POINT('Ctrl Pts',(-2.38113721364588E-14,18.5562499999362,
-10.5687124469213));
#280654=CARTESIAN_POINT('Ctrl Pts',(-3.10606665601013,18.7062499999357,
-9.5594902125713));
#280655=CARTESIAN_POINT('Ctrl Pts',(-5.67314056620243,18.8302206448612,
-8.72539733746421));
#280656=CARTESIAN_POINT('Ctrl Pts',(-7.47704554734297,18.9576928414942,
-6.71753623576259));
#280657=CARTESIAN_POINT('',(-10.0352413152989,18.9576928414942,0.570469052221818));
#280658=CARTESIAN_POINT('Origin',(-3.33066907387547E-14,18.9576928414942,
-4.01761957036229E-14));
#280659=CARTESIAN_POINT('Ctrl Pts',(10.0514428414941,17.4312499999408,-1.23094673026484E-15));
#280660=CARTESIAN_POINT('Ctrl Pts',(10.0514428414941,17.5812499999402,-3.26591175476071));
#280661=CARTESIAN_POINT('Ctrl Pts',(8.13178807675717,17.7312499999396,-5.90808986649102));
#280662=CARTESIAN_POINT('Ctrl Pts',(6.21213331202019,17.881249999939,-8.55026797822134));
#280663=CARTESIAN_POINT('Ctrl Pts',(3.10606665601008,18.0312499999384,-9.5594902125713));
#280664=CARTESIAN_POINT('Ctrl Pts',(-2.35954084775011E-14,18.1812499999378,
-10.5687124469213));
#280665=CARTESIAN_POINT('Ctrl Pts',(-3.10606665601013,18.3312499999371,
-9.5594902125713));
#280666=CARTESIAN_POINT('Ctrl Pts',(-6.21213331202024,18.4812499999365,
-8.55026797822134));
#280667=CARTESIAN_POINT('Ctrl Pts',(-8.13178807675721,18.6312499999359,
-5.90808986649102));
#280668=CARTESIAN_POINT('Ctrl Pts',(-10.0514428414942,18.7812499999353,
-3.2659117547607));
#280669=CARTESIAN_POINT('Ctrl Pts',(-10.0514428414942,18.9312499999347,
2.46189346052968E-15));
#280670=CARTESIAN_POINT('Ctrl Pts',(-10.0514428414942,18.9443610977903,
0.285464590696237));
#280671=CARTESIAN_POINT('Ctrl Pts',(-10.0352413152989,18.9576928414942,
0.570469052221818));
#280672=CARTESIAN_POINT('Origin',(-3.77475828372553E-14,-1.881249999982,
2.68644078414671E-15));
#280673=CARTESIAN_POINT('',(10.0514428414941,14.4312499999528,1.38777687219229E-15));
#280674=CARTESIAN_POINT('',(10.0514428414941,14.8062499999513,1.38622015537184E-15));
#280675=CARTESIAN_POINT('',(10.0514428414941,-1.881249999982,4.14193483802857E-15));
#280676=CARTESIAN_POINT('Ctrl Pts',(10.0514428414941,14.8062499999513,-1.23094673026484E-15));
#280677=CARTESIAN_POINT('Ctrl Pts',(10.0514428414941,14.9562499999507,-3.26591175476071));
#280678=CARTESIAN_POINT('Ctrl Pts',(8.13178807675717,15.1062499999501,-5.90808986649102));
#280679=CARTESIAN_POINT('Ctrl Pts',(6.21213331202019,15.2562499999495,-8.55026797822134));
#280680=CARTESIAN_POINT('Ctrl Pts',(3.10606665601009,15.4062499999489,-9.5594902125713));
#280681=CARTESIAN_POINT('Ctrl Pts',(-2.2083662864797E-14,15.5562499999482,
-10.5687124469213));
#280682=CARTESIAN_POINT('Ctrl Pts',(-3.10606665601013,15.7062499999477,
-9.5594902125713));
#280683=CARTESIAN_POINT('Ctrl Pts',(-6.21213331202024,15.856249999947,-8.55026797822134));
#280684=CARTESIAN_POINT('Ctrl Pts',(-8.13178807675721,16.0062499999464,
-5.90808986649102));
#280685=CARTESIAN_POINT('Ctrl Pts',(-10.0514428414942,16.1562499999458,
-3.2659117547607));
#280686=CARTESIAN_POINT('Ctrl Pts',(-10.0514428414942,16.3062499999452,
2.46189346052968E-15));
#280687=CARTESIAN_POINT('Ctrl Pts',(-10.0514428414942,16.4562499999446,
3.26591175476071));
#280688=CARTESIAN_POINT('Ctrl Pts',(-8.13178807675721,16.606249999944,5.90808986649102));
#280689=CARTESIAN_POINT('Ctrl Pts',(-6.21213331202024,16.7562499999434,
8.55026797822134));
#280690=CARTESIAN_POINT('Ctrl Pts',(-3.10606665601013,16.9062499999428,
9.5594902125713));
#280691=CARTESIAN_POINT('Ctrl Pts',(-2.03589295267817E-14,17.0562499999422,
10.5687124469213));
#280692=CARTESIAN_POINT('Ctrl Pts',(3.10606665601009,17.2062499999417,9.5594902125713));
#280693=CARTESIAN_POINT('Ctrl Pts',(6.2121333120202,17.3562499999411,8.55026797822134));
#280694=CARTESIAN_POINT('Ctrl Pts',(8.13178807675717,17.5062499999405,5.90808986649102));
#280695=CARTESIAN_POINT('Ctrl Pts',(10.0514428414941,17.6562499999399,3.2659117547607));
#280696=CARTESIAN_POINT('Ctrl Pts',(10.0514428414941,17.8062499999393,-1.23094673026484E-15));
#280697=CARTESIAN_POINT('Ctrl Pts',(10.0514428414941,14.4312499999528,-1.23094673026484E-15));
#280698=CARTESIAN_POINT('Ctrl Pts',(10.0514428414941,14.5812499999522,-3.26591175476071));
#280699=CARTESIAN_POINT('Ctrl Pts',(8.13178807675717,14.7312499999516,-5.90808986649102));
#280700=CARTESIAN_POINT('Ctrl Pts',(6.21213331202019,14.881249999951,-8.55026797822134));
#280701=CARTESIAN_POINT('Ctrl Pts',(3.10606665601009,15.0312499999504,-9.5594902125713));
#280702=CARTESIAN_POINT('Ctrl Pts',(-2.18676992058392E-14,15.1812499999498,
-10.5687124469213));
#280703=CARTESIAN_POINT('Ctrl Pts',(-3.10606665601013,15.3312499999492,
-9.5594902125713));
#280704=CARTESIAN_POINT('Ctrl Pts',(-6.21213331202024,15.4812499999485,
-8.55026797822134));
#280705=CARTESIAN_POINT('Ctrl Pts',(-8.13178807675721,15.6312499999479,
-5.90808986649102));
#280706=CARTESIAN_POINT('Ctrl Pts',(-10.0514428414942,15.7812499999473,
-3.2659117547607));
#280707=CARTESIAN_POINT('Ctrl Pts',(-10.0514428414942,15.9312499999467,
2.46189346052968E-15));
#280708=CARTESIAN_POINT('Ctrl Pts',(-10.0514428414942,16.0812499999461,
3.26591175476071));
#280709=CARTESIAN_POINT('Ctrl Pts',(-8.13178807675721,16.2312499999455,
5.90808986649102));
#280710=CARTESIAN_POINT('Ctrl Pts',(-6.21213331202024,16.3812499999449,
8.55026797822134));
#280711=CARTESIAN_POINT('Ctrl Pts',(-3.10606665601013,16.5312499999444,
9.5594902125713));
#280712=CARTESIAN_POINT('Ctrl Pts',(-2.0142965867824E-14,16.6812499999438,
10.5687124469213));
#280713=CARTESIAN_POINT('Ctrl Pts',(3.10606665601009,16.8312499999432,9.5594902125713));
#280714=CARTESIAN_POINT('Ctrl Pts',(6.2121333120202,16.9812499999426,8.55026797822134));
#280715=CARTESIAN_POINT('Ctrl Pts',(8.13178807675717,17.131249999942,5.90808986649102));
#280716=CARTESIAN_POINT('Ctrl Pts',(10.0514428414941,17.2812499999414,3.2659117547607));
#280717=CARTESIAN_POINT('Ctrl Pts',(10.0514428414941,17.4312499999408,-1.23094673026484E-15));
#280718=CARTESIAN_POINT('Origin',(-3.77475828372553E-14,-1.881249999982,
2.68644078414671E-15));
#280719=CARTESIAN_POINT('',(10.0514428414941,11.4312499999648,1.40023060675589E-15));
#280720=CARTESIAN_POINT('',(10.0514428414941,11.8062499999633,1.39867388993544E-15));
#280721=CARTESIAN_POINT('',(10.0514428414941,-1.881249999982,4.14193483802857E-15));
#280722=CARTESIAN_POINT('Ctrl Pts',(10.0514428414941,11.8062499999633,-1.23094673026484E-15));
#280723=CARTESIAN_POINT('Ctrl Pts',(10.0514428414941,11.9562499999627,-3.26591175476071));
#280724=CARTESIAN_POINT('Ctrl Pts',(8.13178807675717,12.1062499999621,-5.90808986649102));
#280725=CARTESIAN_POINT('Ctrl Pts',(6.2121333120202,12.2562499999615,-8.55026797822134));
#280726=CARTESIAN_POINT('Ctrl Pts',(3.10606665601009,12.4062499999609,-9.5594902125713));
#280727=CARTESIAN_POINT('Ctrl Pts',(-2.03559535931351E-14,12.5562499999603,
-10.5687124469213));
#280728=CARTESIAN_POINT('Ctrl Pts',(-3.10606665601013,12.7062499999597,
-9.5594902125713));
#280729=CARTESIAN_POINT('Ctrl Pts',(-6.21213331202024,12.856249999959,-8.55026797822134));
#280730=CARTESIAN_POINT('Ctrl Pts',(-8.13178807675721,13.0062499999584,
-5.90808986649102));
#280731=CARTESIAN_POINT('Ctrl Pts',(-10.0514428414942,13.1562499999578,
-3.2659117547607));
#280732=CARTESIAN_POINT('Ctrl Pts',(-10.0514428414942,13.3062499999572,
2.46189346052968E-15));
#280733=CARTESIAN_POINT('Ctrl Pts',(-10.0514428414942,13.4562499999566,
3.26591175476071));
#280734=CARTESIAN_POINT('Ctrl Pts',(-8.13178807675721,13.606249999956,5.90808986649102));
#280735=CARTESIAN_POINT('Ctrl Pts',(-6.21213331202023,13.7562499999554,
8.55026797822134));
#280736=CARTESIAN_POINT('Ctrl Pts',(-3.10606665601013,13.9062499999549,
9.5594902125713));
#280737=CARTESIAN_POINT('Ctrl Pts',(-1.86312202551199E-14,14.0562499999543,
10.5687124469213));
#280738=CARTESIAN_POINT('Ctrl Pts',(3.10606665601009,14.2062499999537,9.5594902125713));
#280739=CARTESIAN_POINT('Ctrl Pts',(6.2121333120202,14.3562499999531,8.55026797822134));
#280740=CARTESIAN_POINT('Ctrl Pts',(8.13178807675717,14.5062499999525,5.90808986649102));
#280741=CARTESIAN_POINT('Ctrl Pts',(10.0514428414941,14.6562499999519,3.2659117547607));
#280742=CARTESIAN_POINT('Ctrl Pts',(10.0514428414941,14.8062499999513,-1.23094673026484E-15));
#280743=CARTESIAN_POINT('Ctrl Pts',(10.0514428414941,11.4312499999648,-1.23094673026484E-15));
#280744=CARTESIAN_POINT('Ctrl Pts',(10.0514428414941,11.5812499999642,-3.26591175476071));
#280745=CARTESIAN_POINT('Ctrl Pts',(8.13178807675717,11.7312499999636,-5.90808986649102));
#280746=CARTESIAN_POINT('Ctrl Pts',(6.2121333120202,11.881249999963,-8.55026797822134));
#280747=CARTESIAN_POINT('Ctrl Pts',(3.10606665601009,12.0312499999624,-9.5594902125713));
#280748=CARTESIAN_POINT('Ctrl Pts',(-2.01399899341774E-14,12.1812499999618,
-10.5687124469213));
#280749=CARTESIAN_POINT('Ctrl Pts',(-3.10606665601013,12.3312499999612,
-9.5594902125713));
#280750=CARTESIAN_POINT('Ctrl Pts',(-6.21213331202024,12.4812499999605,
-8.55026797822134));
#280751=CARTESIAN_POINT('Ctrl Pts',(-8.13178807675721,12.6312499999599,
-5.90808986649102));
#280752=CARTESIAN_POINT('Ctrl Pts',(-10.0514428414942,12.7812499999593,
-3.2659117547607));
#280753=CARTESIAN_POINT('Ctrl Pts',(-10.0514428414942,12.9312499999587,
2.46189346052968E-15));
#280754=CARTESIAN_POINT('Ctrl Pts',(-10.0514428414942,13.0812499999581,
3.26591175476071));
#280755=CARTESIAN_POINT('Ctrl Pts',(-8.13178807675721,13.2312499999575,
5.90808986649102));
#280756=CARTESIAN_POINT('Ctrl Pts',(-6.21213331202023,13.3812499999569,
8.55026797822134));
#280757=CARTESIAN_POINT('Ctrl Pts',(-3.10606665601013,13.5312499999564,
9.5594902125713));
#280758=CARTESIAN_POINT('Ctrl Pts',(-1.84152565961621E-14,13.6812499999558,
10.5687124469213));
#280759=CARTESIAN_POINT('Ctrl Pts',(3.10606665601009,13.8312499999552,9.5594902125713));
#280760=CARTESIAN_POINT('Ctrl Pts',(6.2121333120202,13.9812499999546,8.55026797822134));
#280761=CARTESIAN_POINT('Ctrl Pts',(8.13178807675717,14.131249999954,5.90808986649102));
#280762=CARTESIAN_POINT('Ctrl Pts',(10.0514428414941,14.2812499999534,3.2659117547607));
#280763=CARTESIAN_POINT('Ctrl Pts',(10.0514428414941,14.4312499999528,-1.23094673026484E-15));
#280764=CARTESIAN_POINT('Origin',(-3.77475828372553E-14,-1.881249999982,
2.68644078414671E-15));
#280765=CARTESIAN_POINT('',(10.0514428414941,8.43124999997676,1.41268434131949E-15));
#280766=CARTESIAN_POINT('',(10.0514428414941,8.80624999997526,1.41112762449904E-15));
#280767=CARTESIAN_POINT('',(10.0514428414941,-1.881249999982,4.14193483802857E-15));
#280768=CARTESIAN_POINT('Ctrl Pts',(10.0514428414941,8.80624999997526,-1.23094673026484E-15));
#280769=CARTESIAN_POINT('Ctrl Pts',(10.0514428414941,8.95624999997466,-3.26591175476071));
#280770=CARTESIAN_POINT('Ctrl Pts',(8.13178807675717,9.10624999997406,-5.90808986649102));
#280771=CARTESIAN_POINT('Ctrl Pts',(6.2121333120202,9.25624999997346,-8.55026797822134));
#280772=CARTESIAN_POINT('Ctrl Pts',(3.10606665601009,9.40624999997286,-9.5594902125713));
#280773=CARTESIAN_POINT('Ctrl Pts',(-1.86282443214733E-14,9.55624999997225,
-10.5687124469213));
#280774=CARTESIAN_POINT('Ctrl Pts',(-3.10606665601013,9.70624999997165,
-9.5594902125713));
#280775=CARTESIAN_POINT('Ctrl Pts',(-6.21213331202024,9.85624999997105,
-8.55026797822134));
#280776=CARTESIAN_POINT('Ctrl Pts',(-8.13178807675721,10.0062499999704,
-5.90808986649102));
#280777=CARTESIAN_POINT('Ctrl Pts',(-10.0514428414942,10.1562499999698,
-3.2659117547607));
#280778=CARTESIAN_POINT('Ctrl Pts',(-10.0514428414942,10.3062499999692,
2.46189346052968E-15));
#280779=CARTESIAN_POINT('Ctrl Pts',(-10.0514428414942,10.4562499999686,
3.26591175476071));
#280780=CARTESIAN_POINT('Ctrl Pts',(-8.13178807675721,10.606249999968,5.90808986649102));
#280781=CARTESIAN_POINT('Ctrl Pts',(-6.21213331202023,10.7562499999674,
8.55026797822134));
#280782=CARTESIAN_POINT('Ctrl Pts',(-3.10606665601013,10.9062499999668,
9.5594902125713));
#280783=CARTESIAN_POINT('Ctrl Pts',(-1.6903510983458E-14,11.0562499999663,
10.5687124469213));
#280784=CARTESIAN_POINT('Ctrl Pts',(3.10606665601009,11.2062499999657,9.5594902125713));
#280785=CARTESIAN_POINT('Ctrl Pts',(6.2121333120202,11.3562499999651,8.55026797822134));
#280786=CARTESIAN_POINT('Ctrl Pts',(8.13178807675717,11.5062499999645,5.90808986649102));
#280787=CARTESIAN_POINT('Ctrl Pts',(10.0514428414941,11.6562499999639,3.2659117547607));
#280788=CARTESIAN_POINT('Ctrl Pts',(10.0514428414941,11.8062499999633,-1.23094673026484E-15));
#280789=CARTESIAN_POINT('Ctrl Pts',(10.0514428414941,8.43124999997676,-1.23094673026484E-15));
#280790=CARTESIAN_POINT('Ctrl Pts',(10.0514428414941,8.58124999997616,-3.26591175476071));
#280791=CARTESIAN_POINT('Ctrl Pts',(8.13178807675717,8.73124999997556,-5.90808986649102));
#280792=CARTESIAN_POINT('Ctrl Pts',(6.2121333120202,8.88124999997496,-8.55026797822134));
#280793=CARTESIAN_POINT('Ctrl Pts',(3.10606665601009,9.03124999997436,-9.5594902125713));
#280794=CARTESIAN_POINT('Ctrl Pts',(-1.84122806625156E-14,9.18124999997375,
-10.5687124469213));
#280795=CARTESIAN_POINT('Ctrl Pts',(-3.10606665601013,9.33124999997315,
-9.5594902125713));
#280796=CARTESIAN_POINT('Ctrl Pts',(-6.21213331202024,9.48124999997255,
-8.55026797822134));
#280797=CARTESIAN_POINT('Ctrl Pts',(-8.13178807675721,9.63124999997195,
-5.90808986649102));
#280798=CARTESIAN_POINT('Ctrl Pts',(-10.0514428414942,9.78124999997135,
-3.2659117547607));
#280799=CARTESIAN_POINT('Ctrl Pts',(-10.0514428414942,9.93124999997075,
2.46189346052968E-15));
#280800=CARTESIAN_POINT('Ctrl Pts',(-10.0514428414942,10.0812499999701,
3.26591175476071));
#280801=CARTESIAN_POINT('Ctrl Pts',(-8.13178807675721,10.2312499999695,
5.90808986649102));
#280802=CARTESIAN_POINT('Ctrl Pts',(-6.21213331202023,10.3812499999689,
8.55026797822134));
#280803=CARTESIAN_POINT('Ctrl Pts',(-3.10606665601012,10.5312499999684,
9.5594902125713));
#280804=CARTESIAN_POINT('Ctrl Pts',(-1.66875473245003E-14,10.6812499999678,
10.5687124469213));
#280805=CARTESIAN_POINT('Ctrl Pts',(3.10606665601009,10.8312499999672,9.5594902125713));
#280806=CARTESIAN_POINT('Ctrl Pts',(6.2121333120202,10.9812499999666,8.55026797822134));
#280807=CARTESIAN_POINT('Ctrl Pts',(8.13178807675717,11.131249999966,5.90808986649102));
#280808=CARTESIAN_POINT('Ctrl Pts',(10.0514428414941,11.2812499999654,3.2659117547607));
#280809=CARTESIAN_POINT('Ctrl Pts',(10.0514428414941,11.4312499999648,-1.23094673026484E-15));
#280810=CARTESIAN_POINT('Origin',(-3.77475828372553E-14,-1.881249999982,
2.68644078414671E-15));
#280811=CARTESIAN_POINT('',(10.0514428414941,5.43124999998876,1.42513807588309E-15));
#280812=CARTESIAN_POINT('',(10.0514428414941,5.80624999998726,1.42358135906264E-15));
#280813=CARTESIAN_POINT('',(10.0514428414941,-1.881249999982,4.14193483802857E-15));
#280814=CARTESIAN_POINT('Ctrl Pts',(10.0514428414941,5.80624999998726,-1.23094673026484E-15));
#280815=CARTESIAN_POINT('Ctrl Pts',(10.0514428414941,5.95624999998666,-3.26591175476071));
#280816=CARTESIAN_POINT('Ctrl Pts',(8.13178807675717,6.10624999998606,-5.90808986649102));
#280817=CARTESIAN_POINT('Ctrl Pts',(6.2121333120202,6.25624999998545,-8.55026797822134));
#280818=CARTESIAN_POINT('Ctrl Pts',(3.10606665601009,6.40624999998485,-9.5594902125713));
#280819=CARTESIAN_POINT('Ctrl Pts',(-1.69005350498115E-14,6.55624999998425,
-10.5687124469213));
#280820=CARTESIAN_POINT('Ctrl Pts',(-3.10606665601013,6.70624999998365,
-9.5594902125713));
#280821=CARTESIAN_POINT('Ctrl Pts',(-6.21213331202023,6.85624999998305,
-8.55026797822134));
#280822=CARTESIAN_POINT('Ctrl Pts',(-8.13178807675721,7.00624999998245,
-5.90808986649102));
#280823=CARTESIAN_POINT('Ctrl Pts',(-10.0514428414942,7.15624999998185,
-3.2659117547607));
#280824=CARTESIAN_POINT('Ctrl Pts',(-10.0514428414942,7.30624999998125,
2.46189346052968E-15));
#280825=CARTESIAN_POINT('Ctrl Pts',(-10.0514428414942,7.45624999998065,
3.26591175476071));
#280826=CARTESIAN_POINT('Ctrl Pts',(-8.13178807675721,7.60624999998005,
5.90808986649102));
#280827=CARTESIAN_POINT('Ctrl Pts',(-6.21213331202023,7.75624999997945,
8.55026797822134));
#280828=CARTESIAN_POINT('Ctrl Pts',(-3.10606665601012,7.90624999997885,
9.5594902125713));
#280829=CARTESIAN_POINT('Ctrl Pts',(-1.51758017117962E-14,8.05624999997825,
10.5687124469213));
#280830=CARTESIAN_POINT('Ctrl Pts',(3.10606665601009,8.20624999997765,9.5594902125713));
#280831=CARTESIAN_POINT('Ctrl Pts',(6.2121333120202,8.35624999997706,8.55026797822134));
#280832=CARTESIAN_POINT('Ctrl Pts',(8.13178807675717,8.50624999997646,5.90808986649102));
#280833=CARTESIAN_POINT('Ctrl Pts',(10.0514428414941,8.65624999997586,3.2659117547607));
#280834=CARTESIAN_POINT('Ctrl Pts',(10.0514428414941,8.80624999997526,-1.23094673026484E-15));
#280835=CARTESIAN_POINT('Ctrl Pts',(10.0514428414941,5.43124999998876,-1.23094673026484E-15));
#280836=CARTESIAN_POINT('Ctrl Pts',(10.0514428414941,5.58124999998816,-3.26591175476071));
#280837=CARTESIAN_POINT('Ctrl Pts',(8.13178807675717,5.73124999998756,-5.90808986649102));
#280838=CARTESIAN_POINT('Ctrl Pts',(6.2121333120202,5.88124999998695,-8.55026797822134));
#280839=CARTESIAN_POINT('Ctrl Pts',(3.10606665601009,6.03124999998635,-9.5594902125713));
#280840=CARTESIAN_POINT('Ctrl Pts',(-1.66845713908537E-14,6.18124999998575,
-10.5687124469213));
#280841=CARTESIAN_POINT('Ctrl Pts',(-3.10606665601012,6.33124999998515,
-9.5594902125713));
#280842=CARTESIAN_POINT('Ctrl Pts',(-6.21213331202023,6.48124999998455,
-8.55026797822134));
#280843=CARTESIAN_POINT('Ctrl Pts',(-8.13178807675721,6.63124999998395,
-5.90808986649102));
#280844=CARTESIAN_POINT('Ctrl Pts',(-10.0514428414942,6.78124999998335,
-3.2659117547607));
#280845=CARTESIAN_POINT('Ctrl Pts',(-10.0514428414942,6.93124999998275,
2.46189346052968E-15));
#280846=CARTESIAN_POINT('Ctrl Pts',(-10.0514428414942,7.08124999998215,
3.26591175476071));
#280847=CARTESIAN_POINT('Ctrl Pts',(-8.13178807675721,7.23124999998155,
5.90808986649102));
#280848=CARTESIAN_POINT('Ctrl Pts',(-6.21213331202023,7.38124999998095,
8.55026797822134));
#280849=CARTESIAN_POINT('Ctrl Pts',(-3.10606665601012,7.53124999998035,
9.5594902125713));
#280850=CARTESIAN_POINT('Ctrl Pts',(-1.49598380528385E-14,7.68124999997975,
10.5687124469213));
#280851=CARTESIAN_POINT('Ctrl Pts',(3.10606665601009,7.83124999997915,9.5594902125713));
#280852=CARTESIAN_POINT('Ctrl Pts',(6.2121333120202,7.98124999997856,8.55026797822134));
#280853=CARTESIAN_POINT('Ctrl Pts',(8.13178807675717,8.13124999997796,5.90808986649102));
#280854=CARTESIAN_POINT('Ctrl Pts',(10.0514428414941,8.28124999997736,3.2659117547607));
#280855=CARTESIAN_POINT('Ctrl Pts',(10.0514428414941,8.43124999997676,-1.23094673026484E-15));
#280856=CARTESIAN_POINT('Origin',(-3.77475828372553E-14,-1.881249999982,
2.68644078414671E-15));
#280857=CARTESIAN_POINT('',(10.0514428414942,2.43125000000076,-1.23094673026484E-15));
#280858=CARTESIAN_POINT('',(10.0514428414942,2.80624999999926,1.43603509362624E-15));
#280859=CARTESIAN_POINT('',(10.0514428414941,-1.881249999982,4.14193483802857E-15));
#280860=CARTESIAN_POINT('',(7.09357268597966,2.43124999999995,7.12128708482866));
#280861=CARTESIAN_POINT('Origin',(-3.77475828372553E-14,2.43125000000001,
2.65063629727636E-15));
#280862=CARTESIAN_POINT('Ctrl Pts',(7.09357268597966,2.43124999999995,7.12128708482865));
#280863=CARTESIAN_POINT('Ctrl Pts',(7.66101577103565,2.46946429917804,6.55605235674466));
#280864=CARTESIAN_POINT('Ctrl Pts',(8.13178807675718,2.50625000000046,5.90808986649102));
#280865=CARTESIAN_POINT('Ctrl Pts',(10.0514428414941,2.65624999999986,3.2659117547607));
#280866=CARTESIAN_POINT('Ctrl Pts',(10.0514428414942,2.80624999999926,-1.23094673026484E-15));
#280867=CARTESIAN_POINT('Origin',(-8.79029313101884E-14,130.96875,0.));
#280868=CARTESIAN_POINT('',(-12.,2.80625000000003,-1.96085794981161E-14));
#280869=CARTESIAN_POINT('',(-12.,2.43125,1.10010189965134E-12));
#280870=CARTESIAN_POINT('',(-12.0000000000001,130.96875,-1.46957615897682E-15));
#280871=CARTESIAN_POINT('',(-8.46872171229246,2.43125,-8.50180878165034));
#280872=CARTESIAN_POINT('Origin',(-1.38777878078145E-14,2.43125000000001,
0.));
#280873=CARTESIAN_POINT('Ctrl Pts',(-8.46872171229245,2.43125000000001,
-8.50180878165033));
#280874=CARTESIAN_POINT('Ctrl Pts',(-9.32728045918118,2.47968070262409,
-7.64659134642077));
#280875=CARTESIAN_POINT('Ctrl Pts',(-10.0513334781109,2.52543312431401,
-6.66627458127563));
#280876=CARTESIAN_POINT('Ctrl Pts',(-11.1884451683539,2.62266495898495,
-4.50834151140613));
#280877=CARTESIAN_POINT('Ctrl Pts',(-11.5906585726304,2.67259700712619,
-3.34111609539217));
#280878=CARTESIAN_POINT('Ctrl Pts',(-11.9363235172771,2.75052914174481,
-1.42769460363205));
#280879=CARTESIAN_POINT('Ctrl Pts',(-12.,2.77879127135541,-0.713750541615098));
#280880=CARTESIAN_POINT('Ctrl Pts',(-12.,2.80625000000003,-5.06539254985228E-14));
#280881=CARTESIAN_POINT('Origin',(-8.79029313101884E-14,130.96875,0.));
#280882=CARTESIAN_POINT('',(-12.,5.80624999998803,-4.62056866567646E-15));
#280883=CARTESIAN_POINT('',(-12.,5.43124999998796,-4.13484609240295E-15));
#280884=CARTESIAN_POINT('',(-12.0000000000001,130.96875,-1.46957615897682E-15));
#280885=CARTESIAN_POINT('Ctrl Pts',(-12.,5.43124999998796,4.9960036108132E-15));
#280886=CARTESIAN_POINT('Ctrl Pts',(-12.,5.40428200239846,-0.700994686785967));
#280887=CARTESIAN_POINT('Ctrl Pts',(-11.9385791761269,5.37653721513424,
-1.40222407934875));
#280888=CARTESIAN_POINT('Ctrl Pts',(-11.5422824562796,5.28562275763319,
-3.63665130268098));
#280889=CARTESIAN_POINT('Ctrl Pts',(-10.9700963138265,5.22180961683611,
-5.10946846096972));
#280890=CARTESIAN_POINT('Ctrl Pts',(-9.28827941189608,5.09885547079727,
-7.75903092660924));
#280891=CARTESIAN_POINT('Ctrl Pts',(-8.1922204615954,5.03753038515127,-8.90855617332867));
#280892=CARTESIAN_POINT('Ctrl Pts',(-5.64057798654912,4.91133636385716,
-10.7040514558091));
#280893=CARTESIAN_POINT('Ctrl Pts',(-4.21524104342245,4.85176008196607,
-11.3412762233036));
#280894=CARTESIAN_POINT('Ctrl Pts',(-1.17023092617838,4.72858683532187,
-12.0467059546444));
#280895=CARTESIAN_POINT('Ctrl Pts',(0.423111701583647,4.66413477213606,
-12.0960096253919));
#280896=CARTESIAN_POINT('Ctrl Pts',(3.51417952374597,4.53909845219181,-11.5788354443557));
#280897=CARTESIAN_POINT('Ctrl Pts',(4.98367674661455,4.48032563488727,-11.0264140689132));
#280898=CARTESIAN_POINT('Ctrl Pts',(7.63013890652938,4.35484690042301,-9.39151076963458));
#280899=CARTESIAN_POINT('Ctrl Pts',(8.78201790847445,4.29177961540221,-8.32442149108578));
#280900=CARTESIAN_POINT('Ctrl Pts',(10.635591354955,4.17064285077446,-5.78081719216585));
#280901=CARTESIAN_POINT('Ctrl Pts',(11.30784934581,4.10611725611296,-4.32053187885184));
#280902=CARTESIAN_POINT('Ctrl Pts',(12.0328413602885,3.97956051015913,-1.26643370783079));
#280903=CARTESIAN_POINT('Ctrl Pts',(12.0957398630745,3.92114872416738,0.293676045080488));
#280904=CARTESIAN_POINT('Ctrl Pts',(11.622503343012,3.79676377226967,3.37312184167239));
#280905=CARTESIAN_POINT('Ctrl Pts',(11.082537936312,3.73273968963923,4.86189128414743));
#280906=CARTESIAN_POINT('Ctrl Pts',(9.46095966411316,3.6091956348989,7.5463603035485));
#280907=CARTESIAN_POINT('Ctrl Pts',(8.39532255435243,3.54874538525415,8.71641626394015));
#280908=CARTESIAN_POINT('Ctrl Pts',(5.89011077929842,3.42271378370603,10.5689867933497));
#280909=CARTESIAN_POINT('Ctrl Pts',(4.47886390989561,3.36242385092618,11.2399520266556));
#280910=CARTESIAN_POINT('Ctrl Pts',(1.44631951535773,3.23975485335779,12.0171624969201));
#280911=CARTESIAN_POINT('Ctrl Pts',(-0.149203109815072,3.17521460742432,
12.1029588003197));
#280912=CARTESIAN_POINT('Ctrl Pts',(-3.25156538805228,3.04972141713474,
11.6548964093293));
#280913=CARTESIAN_POINT('Ctrl Pts',(-4.73023611067824,2.99125037257615,
11.1370609190304));
#280914=CARTESIAN_POINT('Ctrl Pts',(-7.41410523834579,2.86600701276808,
9.5635433962468));
#280915=CARTESIAN_POINT('Ctrl Pts',(-8.59255202546376,2.80264162533294,
8.52048379977188));
#280916=CARTESIAN_POINT('Ctrl Pts',(-10.3307866758556,2.69161560353399,
6.24337183292708));
#280917=CARTESIAN_POINT('Ctrl Pts',(-10.9484046682807,2.63994593786912,
5.08306962327767));
#280918=CARTESIAN_POINT('Ctrl Pts',(-11.7861867448544,2.53421964839238,
2.6070772122473));
#280919=CARTESIAN_POINT('Ctrl Pts',(-11.9999999999999,2.48156496040248,
1.30786573200167));
#280920=CARTESIAN_POINT('Ctrl Pts',(-12.,2.43125,1.11216591491825E-12));
#280921=CARTESIAN_POINT('Ctrl Pts',(-12.,2.80625000000003,-5.07927033766009E-14));
#280922=CARTESIAN_POINT('Ctrl Pts',(-12.,2.83809260234642,0.827703094535515));
#280923=CARTESIAN_POINT('Ctrl Pts',(-11.9143678834799,2.87099240591271,
1.65506306772216));
#280924=CARTESIAN_POINT('Ctrl Pts',(-11.4165365148981,2.96831655978162,
4.02311061157436));
#280925=CARTESIAN_POINT('Ctrl Pts',(-10.7843954258263,3.03293020718696,
5.49725525593906));
#280926=CARTESIAN_POINT('Ctrl Pts',(-9.00354985319716,3.1546886535461,8.08356084583945));
#280927=CARTESIAN_POINT('Ctrl Pts',(-7.88386994414273,3.21648924583216,
9.17893881394363));
#280928=CARTESIAN_POINT('Ctrl Pts',(-5.28285605104015,3.34221742565012,
10.8868875806367));
#280929=CARTESIAN_POINT('Ctrl Pts',(-3.82455859425111,3.40154335506105,
11.4806656367835));
#280930=CARTESIAN_POINT('Ctrl Pts',(-0.748047614205083,3.52599083837247,
12.0797140102831));
#280931=CARTESIAN_POINT('Ctrl Pts',(0.841658075829231,3.59029578433683,
12.073553287322));
#280932=CARTESIAN_POINT('Ctrl Pts',(3.90017388939111,3.71401534787315,11.4533638074065));
#280933=CARTESIAN_POINT('Ctrl Pts',(5.34198612921755,3.7729505871848,10.8560605625585));
#280934=CARTESIAN_POINT('Ctrl Pts',(7.94805013422061,3.89931422881742,9.12833611485889));
#280935=CARTESIAN_POINT('Ctrl Pts',(9.07989705968758,3.96185263740782,8.00331995449505));
#280936=CARTESIAN_POINT('Ctrl Pts',(10.831649647348,4.08407179296626,5.39558600130891));
#280937=CARTESIAN_POINT('Ctrl Pts',(11.4409454271204,4.14759848299899,3.94227237473268));
#280938=CARTESIAN_POINT('Ctrl Pts',(12.0666889074908,4.27268371788102,0.894176234594086));
#280939=CARTESIAN_POINT('Ctrl Pts',(12.0811599033549,4.33104609521448,-0.670909629289751));
#280940=CARTESIAN_POINT('Ctrl Pts',(11.507580289608,4.45679362326614,-3.7531702047656));
#280941=CARTESIAN_POINT('Ctrl Pts',(10.9119981262781,4.52137070290346,-5.23824303713071));
#280942=CARTESIAN_POINT('Ctrl Pts',(9.19762581866298,4.64372126988644,-7.86153843236569));
#280943=CARTESIAN_POINT('Ctrl Pts',(8.10690675886904,4.7045105285579,-8.98211590523337));
#280944=CARTESIAN_POINT('Ctrl Pts',(5.54721341149906,4.83043732643139,-10.755291099315));
#280945=CARTESIAN_POINT('Ctrl Pts',(4.09918917558897,4.89043431468123,-11.3861544471344));
#280946=CARTESIAN_POINT('Ctrl Pts',(1.03667757003992,5.01431551139872,-12.0578834091891));
#280947=CARTESIAN_POINT('Ctrl Pts',(-0.548840370340826,5.07845105933118,
-12.0899118051045));
#280948=CARTESIAN_POINT('Ctrl Pts',(-3.61818808824507,5.20260878260221,
-11.545579735994));
#280949=CARTESIAN_POINT('Ctrl Pts',(-5.07444191571541,5.26116025665351,
-10.9837010305141));
#280950=CARTESIAN_POINT('Ctrl Pts',(-7.72830761428462,5.38765321684513,
-9.31633102641958));
#280951=CARTESIAN_POINT('Ctrl Pts',(-8.89170266286211,5.45142329932537,
-8.21326767702354));
#280952=CARTESIAN_POINT('Ctrl Pts',(-10.7042785399836,5.57295823669527,
-5.64308168585122));
#280953=CARTESIAN_POINT('Ctrl Pts',(-11.3455634256844,5.63619905011406,
-4.20759290526078));
#280954=CARTESIAN_POINT('Ctrl Pts',(-11.8980293264065,5.73551328842991,
-1.8055677862771));
#280955=CARTESIAN_POINT('Ctrl Pts',(-12.,5.77150225280953,-0.903218196644935));
#280956=CARTESIAN_POINT('Ctrl Pts',(-12.,5.80624999998803,1.11022302462516E-15));
#280957=CARTESIAN_POINT('Origin',(-8.79029313101884E-14,130.96875,0.));
#280958=CARTESIAN_POINT('',(-12.,8.80624999997604,1.03764954113354E-13));
#280959=CARTESIAN_POINT('',(-12.,8.43124999997596,1.29348329112088E-14));
#280960=CARTESIAN_POINT('',(-12.0000000000001,130.96875,-1.46957615897682E-15));
#280961=CARTESIAN_POINT('Ctrl Pts',(-12.,8.43124999997596,3.08086889333481E-14));
#280962=CARTESIAN_POINT('Ctrl Pts',(-12.,8.39699003864453,-0.890538898304326));
#280963=CARTESIAN_POINT('Ctrl Pts',(-11.9008722571372,8.36152053074314,
-1.78030968083635));
#280964=CARTESIAN_POINT('Ctrl Pts',(-11.3587162131204,8.26272762338974,
-4.17213341949261));
#280965=CARTESIAN_POINT('Ctrl Pts',(-10.7216942676366,8.19944657225689,
-5.61005323538964));
#280966=CARTESIAN_POINT('Ctrl Pts',(-8.91725471621577,8.07781763716965,
-8.1853262158182));
#280967=CARTESIAN_POINT('Ctrl Pts',(-7.75810310432052,8.01422195318962,
-9.29136231946705));
#280968=CARTESIAN_POINT('Ctrl Pts',(-5.11065784145148,7.88774524607848,
-10.9668857151748));
#280969=CARTESIAN_POINT('Ctrl Pts',(-3.65634228967265,7.82915215245821,
-11.5335430014374));
#280970=CARTESIAN_POINT('Ctrl Pts',(-0.58839170333626,7.70505094434627,
-12.0881175813519));
#280971=CARTESIAN_POINT('Ctrl Pts',(0.997743713920646,7.64089041894949,
-12.0612333077265));
#280972=CARTESIAN_POINT('Ctrl Pts',(4.06220307058269,7.51693043404444,-11.3993078828774));
#280973=CARTESIAN_POINT('Ctrl Pts',(5.5116322884457,7.45703391637837,-10.7734680460166));
#280974=CARTESIAN_POINT('Ctrl Pts',(8.07694712039672,7.33113298492367,-9.00911806416827));
#280975=CARTESIAN_POINT('Ctrl Pts',(9.17159631988134,7.27021652447071,-7.89194794906784));
#280976=CARTESIAN_POINT('Ctrl Pts',(10.8950207952372,7.14794385508041,-5.27361861839748));
#280977=CARTESIAN_POINT('Ctrl Pts',(11.4955806208667,7.08335971465281,-3.78997959136802));
#280978=CARTESIAN_POINT('Ctrl Pts',(12.0789205324003,6.95755349607306,-0.709364752199233));
#280979=CARTESIAN_POINT('Ctrl Pts',(12.0694559833347,6.89920928618014,0.85542033665581));
#280980=CARTESIAN_POINT('Ctrl Pts',(11.4535541993981,6.77416367663518,3.90568423361148));
#280981=CARTESIAN_POINT('Ctrl Pts',(10.8486864033288,6.71060029576505,5.3613903253671));
#280982=CARTESIAN_POINT('Ctrl Pts',(9.10531241508707,6.5882901969422,7.97421059115888));
#280983=CARTESIAN_POINT('Ctrl Pts',(7.97778018551415,6.52590850488026,9.10220317724238));
#280984=CARTESIAN_POINT('Ctrl Pts',(5.37826623328161,6.39956404637928,10.8381361856232));
#280985=CARTESIAN_POINT('Ctrl Pts',(3.93843489438883,6.34056303802432,11.4402666679756));
#280986=CARTESIAN_POINT('Ctrl Pts',(0.88147954041008,6.2169065964041,12.0707786364784));
#280987=CARTESIAN_POINT('Ctrl Pts',(-0.708726898238164,6.15258139473282,
12.0821516304807));
#280988=CARTESIAN_POINT('Ctrl Pts',(-3.78706681449179,6.02805992939772,
11.4930066802789));
#280989=CARTESIAN_POINT('Ctrl Pts',(-5.24673927658173,5.9688122780238,10.9042541867205));
#280990=CARTESIAN_POINT('Ctrl Pts',(-7.85332120820976,5.84311236691359,
9.20515810671939));
#280991=CARTESIAN_POINT('Ctrl Pts',(-8.97691642983155,5.7811619479029,8.11320331071348));
#280992=CARTESIAN_POINT('Ctrl Pts',(-10.7667067410733,5.65948674729555,
5.53196789731668));
#280993=CARTESIAN_POINT('Ctrl Pts',(-11.403767689396,5.59487089658239,4.05936454027656));
#280994=CARTESIAN_POINT('Ctrl Pts',(-11.9117524522773,5.49698725924637,
1.68007305836135));
#280995=CARTESIAN_POINT('Ctrl Pts',(-12.,5.46357521179585,0.840247840106129));
#280996=CARTESIAN_POINT('Ctrl Pts',(-12.,5.43124999998796,3.88578058618805E-15));
#280997=CARTESIAN_POINT('Ctrl Pts',(-12.,5.80624999998803,1.2490009027033E-15));
#280998=CARTESIAN_POINT('Ctrl Pts',(-12.,5.83099605561787,0.643238470259273));
#280999=CARTESIAN_POINT('Ctrl Pts',(-11.9482833205872,5.85640359247076,
1.28686743499849));
#281000=CARTESIAN_POINT('Ctrl Pts',(-11.5911093748506,5.94543216321653,
3.48498547807791));
#281001=CARTESIAN_POINT('Ctrl Pts',(-11.0317226380331,6.00993836902569,
4.979976653213));
#281002=CARTESIAN_POINT('Ctrl Pts',(-9.38320563809063,6.13282993643762,
7.63873227061522));
#281003=CARTESIAN_POINT('Ctrl Pts',(-8.32095697051646,6.19279229952065,
8.78387974016299));
#281004=CARTESIAN_POINT('Ctrl Pts',(-5.80212077898664,6.31889617628815,
10.6207376555748));
#281005=CARTESIAN_POINT('Ctrl Pts',(-4.36438080392958,6.3797070879706,11.2879037183857));
#281006=CARTESIAN_POINT('Ctrl Pts',(-1.31641508298864,6.50299989129578,
12.0300843124326));
#281007=CARTESIAN_POINT('Ctrl Pts',(0.264183353965178,6.56693644113444,
12.0990064476353));
#281008=CARTESIAN_POINT('Ctrl Pts',(3.34298067884587,6.69147640903717,11.6283775643194));
#281009=CARTESIAN_POINT('Ctrl Pts',(4.81307779653889,6.74982155769761,11.100852726935));
#281010=CARTESIAN_POINT('Ctrl Pts',(7.50916246978427,6.8762478441472,9.49439635312942));
#281011=CARTESIAN_POINT('Ctrl Pts',(8.70042697128974,6.94086592426288,8.41629246571222));
#281012=CARTESIAN_POINT('Ctrl Pts',(10.570950077193,7.06219113327966,5.88809168532244));
#281013=CARTESIAN_POINT('Ctrl Pts',(11.2438606194546,7.12478980996596,4.47111460765387));
#281014=CARTESIAN_POINT('Ctrl Pts',(12.0125816948162,7.25037003020925,1.45660826479009));
#281015=CARTESIAN_POINT('Ctrl Pts',(12.1000503244365,7.30932769547842,-0.112508631886311));
#281016=CARTESIAN_POINT('Ctrl Pts',(11.667942147848,7.43414656844159,-3.21659699740878));
#281017=CARTESIAN_POINT('Ctrl Pts',(11.1446562181789,7.49854822981862,-4.72060055222581));
#281018=CARTESIAN_POINT('Ctrl Pts',(9.56191000353393,7.62193542442171,-7.41360951611981));
#281019=CARTESIAN_POINT('Ctrl Pts',(8.52789698680623,7.6812422582497,-8.58293095406429));
#281020=CARTESIAN_POINT('Ctrl Pts',(6.04981872839943,7.80750361436516,-10.4825106951619));
#281021=CARTESIAN_POINT('Ctrl Pts',(4.6224710867094,7.86926711672205,-11.1855208199272));
#281022=CARTESIAN_POINT('Ctrl Pts',(1.58966308417278,7.99194677745798,-11.9965743786724));
#281023=CARTESIAN_POINT('Ctrl Pts',(0.0146910303873457,8.05565573531663,
-12.1014221066078));
#281024=CARTESIAN_POINT('Ctrl Pts',(-3.07233371964743,8.18052850955784,
-11.703010875323));
#281025=CARTESIAN_POINT('Ctrl Pts',(-4.55582240231689,8.23882877065419,
-11.2091110657436));
#281026=CARTESIAN_POINT('Ctrl Pts',(-7.28617656375516,8.36487141394359,
-9.66595804753169));
#281027=CARTESIAN_POINT('Ctrl Pts',(-8.49939669834883,8.42947786260113,
-8.61856269810358));
#281028=CARTESIAN_POINT('Ctrl Pts',(-10.4255624419782,8.55141795323951,
-6.14108644638707));
#281029=CARTESIAN_POINT('Ctrl Pts',(-11.1312039295987,8.61289784773076,
-4.74362485061815));
#281030=CARTESIAN_POINT('Ctrl Pts',(-11.8496202008874,8.72009371706788,
-2.1906485030476));
#281031=CARTESIAN_POINT('Ctrl Pts',(-12.,8.76405334452794,-1.09684195762376));
#281032=CARTESIAN_POINT('Ctrl Pts',(-12.,8.80624999997604,2.16215934045749E-13));
#281033=CARTESIAN_POINT('Origin',(-8.79029313101884E-14,130.96875,0.));
#281034=CARTESIAN_POINT('',(-12.,11.806249999964,7.52114056987762E-14));
#281035=CARTESIAN_POINT('',(-12.,11.431249999964,9.0858611452087E-14));
#281036=CARTESIAN_POINT('',(-12.0000000000001,130.96875,-1.46957615897682E-15));
#281037=CARTESIAN_POINT('Ctrl Pts',(-12.,11.431249999964,1.57374113740616E-13));
#281038=CARTESIAN_POINT('Ctrl Pts',(-12.,11.389588144316,-1.08294059853536));
#281039=CARTESIAN_POINT('Ctrl Pts',(-11.8534082069267,11.3462030315979,
-2.16304424929612));
#281040=CARTESIAN_POINT('Ctrl Pts',(-11.1474361064258,11.2395681924447,
-4.70548077250192));
#281041=CARTESIAN_POINT('Ctrl Pts',(-10.4463866902839,11.1779409983725,
-6.10569158782984));
#281042=CARTESIAN_POINT('Ctrl Pts',(-8.52800813932628,11.0560849524982,
-8.59035119496663));
#281043=CARTESIAN_POINT('Ctrl Pts',(-7.31783574715978,10.9914747568544,
-9.64209899454808));
#281044=CARTESIAN_POINT('Ctrl Pts',(-4.59225812837821,10.8653757798519,
-11.1941956705663));
#281045=CARTESIAN_POINT('Ctrl Pts',(-3.11065270066361,10.8070785448882,
-11.6928484439898));
#281046=CARTESIAN_POINT('Ctrl Pts',(-0.024729051402356,10.6822503111089,
-12.1014704681028));
#281047=CARTESIAN_POINT('Ctrl Pts',(1.55108665626511,10.6185072267339,-12.0016879126557));
#281048=CARTESIAN_POINT('Ctrl Pts',(4.58609229101319,10.4957386699076,-11.2003626816289));
#281049=CARTESIAN_POINT('Ctrl Pts',(6.01492924344135,10.4341191736442,-10.5024374214762));
#281050=CARTESIAN_POINT('Ctrl Pts',(8.49881554186177,10.3078790847169,-8.61174622744464));
#281051=CARTESIAN_POINT('Ctrl Pts',(9.53684202246883,10.2484890722127,-7.44584929710471));
#281052=CARTESIAN_POINT('Ctrl Pts',(11.1289632812859,10.1251698186584,-4.75765250051073));
#281053=CARTESIAN_POINT('Ctrl Pts',(11.6573912043948,10.0607512188981,-3.25487939149134));
#281054=CARTESIAN_POINT('Ctrl Pts',(12.0995477628908,9.93586159518112,-0.152216878092207));
#281055=CARTESIAN_POINT('Ctrl Pts',(12.0172926245384,9.87696672724328,1.41663507310838));
#281056=CARTESIAN_POINT('Ctrl Pts',(11.2587456915536,9.75141649237194,4.43366776818686));
#281057=CARTESIAN_POINT('Ctrl Pts',(10.5903204860711,9.68865215211609,5.85330452076973));
#281058=CARTESIAN_POINT('Ctrl Pts',(8.7274459043467,9.56741403338887,8.38836970557499));
#281059=CARTESIAN_POINT('Ctrl Pts',(7.53923094341759,9.50279706761554,9.47062405795193));
#281060=CARTESIAN_POINT('Ctrl Pts',(4.84788179509845,9.37632143015218,11.0856739517181));
#281061=CARTESIAN_POINT('Ctrl Pts',(3.3796138240055,9.31795825087466,11.6177611184392));
#281062=CARTESIAN_POINT('Ctrl Pts',(0.302011016147692,9.19346660220051,
12.0981839171448));
#281063=CARTESIAN_POINT('Ctrl Pts',(-1.27928918066634,9.12950166557921,
12.0341515012749));
#281064=CARTESIAN_POINT('Ctrl Pts',(-4.32924149411119,9.0061285028992,11.3013233400185));
#281065=CARTESIAN_POINT('Ctrl Pts',(-5.76836621779356,8.94543495540061,
10.6389972126522));
#281066=CARTESIAN_POINT('Ctrl Pts',(-8.2926736112961,8.81935367750649,8.81062023518514));
#281067=CARTESIAN_POINT('Ctrl Pts',(-9.35872514961793,8.7592904954788,7.66874323005069));
#281068=CARTESIAN_POINT('Ctrl Pts',(-11.0160663846226,8.63646880844639,
5.01467122135901));
#281069=CARTESIAN_POINT('Ctrl Pts',(-11.580300837083,8.57195112870678,3.52095691603815));
#281070=CARTESIAN_POINT('Ctrl Pts',(-11.9462969687398,8.48236891808552,
1.31131429491467));
#281071=CARTESIAN_POINT('Ctrl Pts',(-12.,8.45646681014301,0.655475063957913));
#281072=CARTESIAN_POINT('Ctrl Pts',(-12.,8.43124999997596,2.81719092498633E-14));
#281073=CARTESIAN_POINT('Ctrl Pts',(-12.,8.80624999997604,2.17326157070374E-13));
#281074=CARTESIAN_POINT('Ctrl Pts',(-12.,8.82387914688782,0.458244564755818));
#281075=CARTESIAN_POINT('Ctrl Pts',(-11.9737525692637,8.84185579477114,
0.916993615098396));
#281076=CARTESIAN_POINT('Ctrl Pts',(-11.7409281292704,8.92247877912802,
2.93702401571875));
#281077=CARTESIAN_POINT('Ctrl Pts',(-11.2551207775011,8.9867366023522,4.44946623076792));
#281078=CARTESIAN_POINT('Ctrl Pts',(-9.74079553096694,9.11059263174499,
7.17689320743257));
#281079=CARTESIAN_POINT('Ctrl Pts',(-8.73596928917568,9.16939412094754,
8.37100315741494));
#281080=CARTESIAN_POINT('Ctrl Pts',(-6.30027620028189,9.29579879828115,
10.3349489533987));
#281081=CARTESIAN_POINT('Ctrl Pts',(-4.88388425520457,9.35869273192279,
11.0748315659316));
#281082=CARTESIAN_POINT('Ctrl Pts',(-1.86747266436311,9.48070914387332,
11.9560104548374));
#281083=CARTESIAN_POINT('Ctrl Pts',(-0.299057170406009,9.54415288331568,
12.0972702243737));
#281084=CARTESIAN_POINT('Ctrl Pts',(2.79530693938728,9.66932254089551,11.7725603037712));
#281085=CARTESIAN_POINT('Ctrl Pts',(4.29228928804916,9.72773524947492,11.3129655897213));
#281086=CARTESIAN_POINT('Ctrl Pts',(7.05646075467183,9.85335126957896,9.83430122549981));
#281087=CARTESIAN_POINT('Ctrl Pts',(8.29113131987403,9.9179105211198,8.81841490035983));
#281088=CARTESIAN_POINT('Ctrl Pts',(10.272736135536,10.0404294741798,6.3928979063031));
#281089=CARTESIAN_POINT('Ctrl Pts',(11.011191455937,10.1009504193315,5.01518681941377));
#281090=CARTESIAN_POINT('Ctrl Pts',(11.9231536974671,10.2261545125477,2.05699923912446));
#281091=CARTESIAN_POINT('Ctrl Pts',(12.088766400008,10.2857313049205,0.504512301282102));
#281092=CARTESIAN_POINT('Ctrl Pts',(11.8187680163681,10.4089041617859,-2.60946288488135));
#281093=CARTESIAN_POINT('Ctrl Pts',(11.3733158940114,10.4733563091391,-4.14006848777134));
#281094=CARTESIAN_POINT('Ctrl Pts',(9.92631147992378,10.5983930113062,-6.92005923599754));
#281095=CARTESIAN_POINT('Ctrl Pts',(8.94685217287931,10.6571655254461,-8.14694229711963));
#281096=CARTESIAN_POINT('Ctrl Pts',(6.57420247458641,10.7826440862918,-10.1587088160428));
#281097=CARTESIAN_POINT('Ctrl Pts',(5.20340159946979,10.8457116247515,-10.9244886456193));
#281098=CARTESIAN_POINT('Ctrl Pts',(2.21152525060571,10.966848963036,-11.9013775368152));
#281099=CARTESIAN_POINT('Ctrl Pts',(0.61498212470326,11.031373450461,-12.0895090711595));
#281100=CARTESIAN_POINT('Ctrl Pts',(-2.5136705660668,11.157930110277,-11.8353108616964));
#281101=CARTESIAN_POINT('Ctrl Pts',(-4.01686727189288,11.2163420561628,
-11.4130602011789));
#281102=CARTESIAN_POINT('Ctrl Pts',(-6.79938572972625,11.3407266944546,
-10.0114383623218));
#281103=CARTESIAN_POINT('Ctrl Pts',(-8.04845240744468,11.4047509440899,
-9.0378679579154));
#281104=CARTESIAN_POINT('Ctrl Pts',(-10.1004829868513,11.5282954884597,
-6.66614889102401));
#281105=CARTESIAN_POINT('Ctrl Pts',(-10.8839969360667,11.5887450536416,
-5.29111991055287));
#281106=CARTESIAN_POINT('Ctrl Pts',(-11.791482446841,11.7045287953537,-2.57634637217284));
#281107=CARTESIAN_POINT('Ctrl Pts',(-12.,11.7565624003826,-1.29155838100936));
#281108=CARTESIAN_POINT('Ctrl Pts',(-12.,11.806249999964,1.5931700403371E-13));
#281109=CARTESIAN_POINT('Origin',(-8.79029313101884E-14,130.96875,0.));
#281110=CARTESIAN_POINT('',(-12.,14.806249999952,7.34788079488412E-16));
#281111=CARTESIAN_POINT('',(-12.,14.431249999952,8.88810266894734E-14));
#281112=CARTESIAN_POINT('',(-12.0000000000001,130.96875,-1.46957615897682E-15));
#281113=CARTESIAN_POINT('Ctrl Pts',(-12.,14.431249999952,1.65145674912992E-13));
#281114=CARTESIAN_POINT('Ctrl Pts',(-12.,14.3823065495871,-1.27221528201616));
#281115=CARTESIAN_POINT('Ctrl Pts',(-11.7976819562748,14.3310777566137,
-2.53809767281549));
#281116=CARTESIAN_POINT('Ctrl Pts',(-10.9088722919085,14.2160239603072,
-5.23996547038095));
#281117=CARTESIAN_POINT('Ctrl Pts',(-10.1312207970015,14.1554082812044,
-6.61959498633458));
#281118=CARTESIAN_POINT('Ctrl Pts',(-8.08969908479941,14.0319810826221,
-9.00084288154191));
#281119=CARTESIAN_POINT('Ctrl Pts',(-6.84571246974124,13.9679972617242,
-9.97970502074197));
#281120=CARTESIAN_POINT('Ctrl Pts',(-4.07025897930456,13.8435387628565,
-11.3941574172112));
#281121=CARTESIAN_POINT('Ctrl Pts',(-2.56883963781858,13.7851617460955,
-11.823487409551));
#281122=CARTESIAN_POINT('Ctrl Pts',(0.558627108948717,13.6586530587222,
-12.0922194803715));
#281123=CARTESIAN_POINT('Ctrl Pts',(2.15601857273127,13.5940372166789,-11.9115809969756));
#281124=CARTESIAN_POINT('Ctrl Pts',(5.15171928337348,13.4728585774309,-10.9488291593168));
#281125=CARTESIAN_POINT('Ctrl Pts',(6.52552543835335,13.4099801485513,-10.1899618727092));
#281126=CARTESIAN_POINT('Ctrl Pts',(8.907990416113,13.2844504371692,-8.18955361272096));
#281127=CARTESIAN_POINT('Ctrl Pts',(9.89371655991383,13.2255964066297,-6.96674262794056));
#281128=CARTESIAN_POINT('Ctrl Pts',(11.3536103486055,13.100659174132,-4.19352546377302));
#281129=CARTESIAN_POINT('Ctrl Pts',(11.8060909206473,13.0362294645118,-2.6657867795321));
#281130=CARTESIAN_POINT('Ctrl Pts',(12.0910466477122,12.9129568227145,0.44592223833023));
#281131=CARTESIAN_POINT('Ctrl Pts',(11.9329895718556,12.8535084379708,1.99900816849489));
#281132=CARTESIAN_POINT('Ctrl Pts',(11.0280644293945,12.7272830031674,4.98603056075995));
#281133=CARTESIAN_POINT('Ctrl Pts',(10.2794942003153,12.6657596882479,6.38831127923374));
#281134=CARTESIAN_POINT('Ctrl Pts',(8.29003956409569,12.5429310906611,8.8160471031109));
#281135=CARTESIAN_POINT('Ctrl Pts',(7.07134536980327,12.4791651632238,9.82055700326823));
#281136=CARTESIAN_POINT('Ctrl Pts',(4.32900779517834,12.3542709355575,11.2989156424085));
#281137=CARTESIAN_POINT('Ctrl Pts',(2.8338924598131,12.2958833579715,11.7632835526384));
#281138=CARTESIAN_POINT('Ctrl Pts',(-0.259514673870521,12.1707524108885,
12.0982475553265));
#281139=CARTESIAN_POINT('Ctrl Pts',(-1.82889134293284,12.1072697910964,
11.9620377569558));
#281140=CARTESIAN_POINT('Ctrl Pts',(-4.84764043700566,11.9851588251539,
11.0906055638688));
#281141=CARTESIAN_POINT('Ctrl Pts',(-6.26557890992037,11.9224317368724,
10.3558711604917));
#281142=CARTESIAN_POINT('Ctrl Pts',(-8.70721886267572,11.7960459036551,
8.40090307546756));
#281143=CARTESIAN_POINT('Ctrl Pts',(-9.71612932779523,11.7371842182329,
7.21024969635897));
#281144=CARTESIAN_POINT('Ctrl Pts',(-11.2400537405356,11.6133911122404,
4.48757728203246));
#281145=CARTESIAN_POINT('Ctrl Pts',(-11.7311135069529,11.5491109773968,
2.97626172118548));
#281146=CARTESIAN_POINT('Ctrl Pts',(-11.9722226129965,11.4678882290064,
0.943333159935274));
#281147=CARTESIAN_POINT('Ctrl Pts',(-12.,11.4493856810174,0.471411198311356));
#281148=CARTESIAN_POINT('Ctrl Pts',(-12.,11.431249999964,1.62925228863742E-13));
#281149=CARTESIAN_POINT('Ctrl Pts',(-12.,11.806249999964,1.59178226155632E-13));
#281150=CARTESIAN_POINT('Ctrl Pts',(-12.,11.8159717771291,0.252703750665779));
#281151=CARTESIAN_POINT('Ctrl Pts',(-11.9920177414135,11.8258030097974,
0.505659048206776));
#281152=CARTESIAN_POINT('Ctrl Pts',(-11.8759839799423,11.8977356686935,
2.33774440790498));
#281153=CARTESIAN_POINT('Ctrl Pts',(-11.4645665854366,11.9622759756235,
3.88170014686002));
#281154=CARTESIAN_POINT('Ctrl Pts',(-10.0798043248063,12.0877695389606,
6.69379005208959));
#281155=CARTESIAN_POINT('Ctrl Pts',(-9.13040461137842,12.1462403905476,
7.9400858895626));
#281156=CARTESIAN_POINT('Ctrl Pts',(-6.80457932068993,12.2714835337107,
10.0063993645393));
#281157=CARTESIAN_POINT('Ctrl Pts',(-5.44842333302093,12.3348491603387,
10.8048732903662));
#281158=CARTESIAN_POINT('Ctrl Pts',(-2.48267155529713,12.4566779662627,
11.8468016530471));
#281159=CARTESIAN_POINT('Ctrl Pts',(-0.89842029146626,12.5199081357668,
12.0707791359501));
#281160=CARTESIAN_POINT('Ctrl Pts',(2.22736272105365,12.6463487146592,11.8924296877473));
#281161=CARTESIAN_POINT('Ctrl Pts',(3.73965462415031,12.7050417605495,11.5067830828562));
#281162=CARTESIAN_POINT('Ctrl Pts',(6.55807938154271,12.8290189984987,10.1717166683596));
#281163=CARTESIAN_POINT('Ctrl Pts',(7.83300587353999,12.8932308706615,9.22584812478829));
#281164=CARTESIAN_POINT('Ctrl Pts',(9.93882760285228,13.0173573477921,6.90369101150418));
#281165=CARTESIAN_POINT('Ctrl Pts',(10.7523241784602,13.0770488173305,5.55236384193603));
#281166=CARTESIAN_POINT('Ctrl Pts',(11.811475439129,13.2028932743447,2.62535552815208));
#281167=CARTESIAN_POINT('Ctrl Pts',(12.0515012216521,13.264092407653,1.07909280556291));
#281168=CARTESIAN_POINT('Ctrl Pts',(11.9286798792065,13.3861958640999,-2.05490555938842));
#281169=CARTESIAN_POINT('Ctrl Pts',(11.552914872369,13.4507928927077,-3.61191986054169));
#281170=CARTESIAN_POINT('Ctrl Pts',(10.2330810216963,13.576722174506,-6.45643216581518));
#281171=CARTESIAN_POINT('Ctrl Pts',(9.31469434867856,13.6350374464028,-7.72256004961813));
#281172=CARTESIAN_POINT('Ctrl Pts',(7.03784286455176,13.7599958252643,-9.8443034302874));
#281173=CARTESIAN_POINT('Ctrl Pts',(5.6975456848272,13.8236354433468,-10.6761287992143));
#281174=CARTESIAN_POINT('Ctrl Pts',(2.75948640105646,13.9461372360307,-11.7844774161238));
#281175=CARTESIAN_POINT('Ctrl Pts',(1.18799885877861,14.0081944366527,-12.0448164734704));
#281176=CARTESIAN_POINT('Ctrl Pts',(-1.93436825361326,14.1344968394823,
-11.9435955330094));
#281177=CARTESIAN_POINT('Ctrl Pts',(-3.45575955286439,14.1936485964835,
-11.5952143043706));
#281178=CARTESIAN_POINT('Ctrl Pts',(-6.30965930479221,14.3171679826371,
-10.3282315856791));
#281179=CARTESIAN_POINT('Ctrl Pts',(-7.61018914604508,14.3815340387382,
-9.41111828566092));
#281180=CARTESIAN_POINT('Ctrl Pts',(-9.76981475623303,14.5062104246925,
-7.13988752706686));
#281181=CARTESIAN_POINT('Ctrl Pts',(-10.613280708508,14.5653019323891,-5.81252942271048));
#281182=CARTESIAN_POINT('Ctrl Pts',(-11.7219456143113,14.6884953720743,
-2.97051848708096));
#281183=CARTESIAN_POINT('Ctrl Pts',(-12.,14.74887273433,-1.49144029733251));
#281184=CARTESIAN_POINT('Ctrl Pts',(-12.,14.806249999952,-2.77555756156289E-16));
#281185=CARTESIAN_POINT('Origin',(-8.79029313101884E-14,130.96875,0.));
#281186=CARTESIAN_POINT('',(-12.,17.80624999994,-1.4751353765381E-14));
#281187=CARTESIAN_POINT('',(-12.,17.43124999994,-5.45323593414533E-15));
#281188=CARTESIAN_POINT('',(-12.0000000000001,130.96875,-1.46957615897682E-15));
#281189=CARTESIAN_POINT('Ctrl Pts',(-12.,17.43124999994,8.32667268468867E-16));
#281190=CARTESIAN_POINT('Ctrl Pts',(-12.,17.3746355953144,-1.47161081227273));
#281191=CARTESIAN_POINT('Ctrl Pts',(-11.7292898349336,17.3150879968699,
-2.93150675551766));
#281192=CARTESIAN_POINT('Ctrl Pts',(-10.6412379837764,17.1926179533313,
-5.76141162610182));
#281193=CARTESIAN_POINT('Ctrl Pts',(-9.80367175971446,17.1334211137684,
-7.09350945191991));
#281194=CARTESIAN_POINT('Ctrl Pts',(-7.65463816373364,17.0088503852345,
-9.3748750759184));
#281195=CARTESIAN_POINT('Ctrl Pts',(-6.35912640911618,16.9445119589857,
-10.2977331098152));
#281196=CARTESIAN_POINT('Ctrl Pts',(-3.5121749371591,16.820898371858,-11.578241266071));
#281197=CARTESIAN_POINT('Ctrl Pts',(-1.99257551141557,16.7618513725082,
-11.9340128619219));
#281198=CARTESIAN_POINT('Ctrl Pts',(1.1305076194917,16.6355200061212,-12.0505218705341));
#281199=CARTESIAN_POINT('Ctrl Pts',(2.70454543356806,16.5732420527098,-11.79738307137));
#281200=CARTESIAN_POINT('Ctrl Pts',(5.64818469253235,16.450871183792,-10.7022210872036));
#281201=CARTESIAN_POINT('Ctrl Pts',(6.99170350750002,16.3872834703396,-9.87701294909237));
#281202=CARTESIAN_POINT('Ctrl Pts',(9.27837150810931,16.2622649633922,-7.76625194779492));
#281203=CARTESIAN_POINT('Ctrl Pts',(10.2029416438783,16.2039313203782,-6.50406288910224));
#281204=CARTESIAN_POINT('Ctrl Pts',(11.5357778969021,16.0780859920241,-3.66595757065916));
#281205=CARTESIAN_POINT('Ctrl Pts',(11.9186935182967,16.0134974683325,-2.11148771819885));
#281206=CARTESIAN_POINT('Ctrl Pts',(12.0565303645475,15.891277695036,1.02065530465216));
#281207=CARTESIAN_POINT('Ctrl Pts',(11.8241053985494,15.8302737912193,2.56758110483523));
#281208=CARTESIAN_POINT('Ctrl Pts',(10.7792241968896,15.7043904723188,5.50023620124078));
#281209=CARTESIAN_POINT('Ctrl Pts',(9.97171740280202,15.644559966527,6.8563211212477));
#281210=CARTESIAN_POINT('Ctrl Pts',(7.87664645564514,15.5205472616759,9.18849032656098));
#281211=CARTESIAN_POINT('Ctrl Pts',(6.60686838021293,15.4563702630232,10.1399783304692));
#281212=CARTESIAN_POINT('Ctrl Pts',(3.79558520126637,15.332307632391,11.4884657716385));
#281213=CARTESIAN_POINT('Ctrl Pts',(2.28511098038302,15.2736846808067,11.8814786023088));
#281214=CARTESIAN_POINT('Ctrl Pts',(-0.841288922901996,15.1472191481587,
12.0750852080575));
#281215=CARTESIAN_POINT('Ctrl Pts',(-2.42803402963569,15.0837396595986,
11.8583112574829));
#281216=CARTESIAN_POINT('Ctrl Pts',(-5.39912874869519,14.9620476191367,
10.8294889713357));
#281217=CARTESIAN_POINT('Ctrl Pts',(-6.75830585804143,14.8987397183168,
10.0376011230291));
#281218=CARTESIAN_POINT('Ctrl Pts',(-9.09365631450678,14.7734456974542,
7.98225807485496));
#281219=CARTESIAN_POINT('Ctrl Pts',(-10.0491372958055,14.7149257751828,
6.73987402012214));
#281220=CARTESIAN_POINT('Ctrl Pts',(-11.4465469019859,14.5895219160253,
3.93422521894999));
#281221=CARTESIAN_POINT('Ctrl Pts',(-11.8648920847047,14.5249968281946,
2.39291605364606));
#281222=CARTESIAN_POINT('Ctrl Pts',(-11.9907858489882,14.4522660510314,
0.543288455475417));
#281223=CARTESIAN_POINT('Ctrl Pts',(-12.,14.4416950587665,0.271504426974703));
#281224=CARTESIAN_POINT('Ctrl Pts',(-12.,14.431249999952,1.61329283265843E-13));
#281225=CARTESIAN_POINT('Ctrl Pts',(-12.,14.806249999952,2.93915231795365E-15));
#281226=CARTESIAN_POINT('Ctrl Pts',(-12.,14.8085776919202,0.0605050373769862));
#281227=CARTESIAN_POINT('Ctrl Pts',(-11.9995423931535,14.8109118698816,
0.121029983434178));
#281228=CARTESIAN_POINT('Ctrl Pts',(-11.9745681208275,14.8747154420508,
1.77139833348643));
#281229=CARTESIAN_POINT('Ctrl Pts',(-11.6347695110624,14.9393338131942,
3.34065359426618));
#281230=CARTESIAN_POINT('Ctrl Pts',(-10.3802032414723,15.0656598712332,
6.21668625540801));
#281231=CARTESIAN_POINT('Ctrl Pts',(-9.49265983287779,15.1239776301458,
7.50234936474159));
#281232=CARTESIAN_POINT('Ctrl Pts',(-7.2651417573986,15.2486115875892,9.67834968251244));
#281233=CARTESIAN_POINT('Ctrl Pts',(-5.94134751640508,15.3124898214874,
10.5429252185951));
#281234=CARTESIAN_POINT('Ctrl Pts',(-3.03154430393017,15.4356205591155,
11.716617455179));
#281235=CARTESIAN_POINT('Ctrl Pts',(-1.47280762426799,15.4966736800754,
12.0125075855231));
#281236=CARTESIAN_POINT('Ctrl Pts',(1.64574301659647,15.6228217033888,11.9868816261993));
#281237=CARTESIAN_POINT('Ctrl Pts',(3.17590997098518,15.6825916397591,11.6750732916029));
#281238=CARTESIAN_POINT('Ctrl Pts',(6.06355811562229,15.8056205377235,10.4751704425746));
#281239=CARTESIAN_POINT('Ctrl Pts',(7.38847734367979,15.870101979139,9.58677332163239));
#281240=CARTESIAN_POINT('Ctrl Pts',(9.59993987846,15.9952765907215,7.36593535177551));
#281241=CARTESIAN_POINT('Ctrl Pts',(10.4722897871741,16.0539449796668,6.06192650551696));
#281242=CARTESIAN_POINT('Ctrl Pts',(11.6719830965627,16.1793584728463,3.19178536257051));
#281243=CARTESIAN_POINT('Ctrl Pts',(11.9871728371349,16.2425170317467,1.65247993553365));
#281244=CARTESIAN_POINT('Ctrl Pts',(12.0123233958607,16.3638618392866,-1.49353359300221));
#281245=CARTESIAN_POINT('Ctrl Pts',(11.7090926266369,16.4279893770273,-3.06992017829334));
#281246=CARTESIAN_POINT('Ctrl Pts',(10.5221068179719,16.5545138035291,-5.97306736792306));
#281247=CARTESIAN_POINT('Ctrl Pts',(9.66546397675279,16.6129913136869,-7.27812599480033));
#281248=CARTESIAN_POINT('Ctrl Pts',(7.48795963920015,16.7372599557761,-9.50759970543453));
#281249=CARTESIAN_POINT('Ctrl Pts',(6.18140413449528,16.8013434032466,-10.4045332992438));
#281250=CARTESIAN_POINT('Ctrl Pts',(3.30059548053173,16.9250642929444,-11.6429540262693));
#281251=CARTESIAN_POINT('Ctrl Pts',(1.75466748516089,16.9852722091947,-11.9738660457127));
#281252=CARTESIAN_POINT('Ctrl Pts',(-1.35967481828507,17.1112500016836,
-12.0228895360496));
#281253=CARTESIAN_POINT('Ctrl Pts',(-2.89836992220341,17.1717929521038,
-11.7472486716372));
#281254=CARTESIAN_POINT('Ctrl Pts',(-5.81834650237366,17.2942978705331,
-10.6138798842907));
#281255=CARTESIAN_POINT('Ctrl Pts',(-7.16664128401645,17.358858746241,-9.75431556637224));
#281256=CARTESIAN_POINT('Ctrl Pts',(-9.42839959622457,17.4844859773994,
-7.58366729980175));
#281257=CARTESIAN_POINT('Ctrl Pts',(-10.3288130493131,17.5428938940208,
-6.30256531857088));
#281258=CARTESIAN_POINT('Ctrl Pts',(-11.5955599081519,17.6680565822307,
-3.46073051250532));
#281259=CARTESIAN_POINT('Ctrl Pts',(-11.9468073098174,17.7315074318097,
-1.92554324987653));
#281260=CARTESIAN_POINT('Ctrl Pts',(-11.9981396947232,17.7968373715993,
-0.244063417473451));
#281261=CARTESIAN_POINT('Ctrl Pts',(-12.,17.8015567661665,-0.121993927365321));
#281262=CARTESIAN_POINT('Ctrl Pts',(-12.,17.80624999994,8.91647866652079E-15));
#281263=CARTESIAN_POINT('Origin',(-8.79029313101884E-14,130.96875,0.));
#281264=CARTESIAN_POINT('',(-12.,20.806249999928,-1.97473573761942E-14));
#281265=CARTESIAN_POINT('',(-12.,20.431249999928,-4.05190619052819E-16));
#281266=CARTESIAN_POINT('',(-12.0000000000001,130.96875,-1.46957615897682E-15));
#281267=CARTESIAN_POINT('',(-11.7339375393676,20.90625,2.51290863785771));
#281268=CARTESIAN_POINT('Ctrl Pts',(-12.,20.806249999928,1.08246744900953E-14));
#281269=CARTESIAN_POINT('Ctrl Pts',(-12.,20.8386924218465,0.843294549988032));
#281270=CARTESIAN_POINT('Ctrl Pts',(-11.9111127257393,20.8722077061892,
1.685595404463));
#281271=CARTESIAN_POINT('Ctrl Pts',(-11.7339375393676,20.90625,2.51290863785771));
#281272=CARTESIAN_POINT('',(-6.54406206475579,20.90625,10.0585909397204));
#281273=CARTESIAN_POINT('Origin',(-1.38777878078145E-14,20.90625,0.));
#281274=CARTESIAN_POINT('Ctrl Pts',(-6.54406206475577,20.90625,10.0585909397204));
#281275=CARTESIAN_POINT('Ctrl Pts',(-7.59789374773782,20.8554613999318,
9.37297403964269));
#281276=CARTESIAN_POINT('Ctrl Pts',(-8.53748121101216,20.8045743444593,
8.52597257550313));
#281277=CARTESIAN_POINT('Ctrl Pts',(-10.1137548522019,20.7066754868414,
6.57804909368321));
#281278=CARTESIAN_POINT('Ctrl Pts',(-10.7428818779751,20.6582025322463,
5.4908453904987));
#281279=CARTESIAN_POINT('Ctrl Pts',(-11.7267322019416,20.5479783769447,
2.94539781423955));
#281280=CARTESIAN_POINT('Ctrl Pts',(-12.,20.4881310653806,1.47854228066918));
#281281=CARTESIAN_POINT('Ctrl Pts',(-12.,20.431249999928,1.30451205393456E-14));
#281282=CARTESIAN_POINT('Origin',(-8.79029313101884E-14,130.96875,0.));
#281283=CARTESIAN_POINT('Ctrl Pts',(-12.,20.431249999928,-5.18682319317065E-15));
#281284=CARTESIAN_POINT('Ctrl Pts',(-12.,20.4272741804144,-0.1033457654905));
#281285=CARTESIAN_POINT('Ctrl Pts',(-11.9986649616217,20.4232795252713,
-0.206747356078088));
#281286=CARTESIAN_POINT('Ctrl Pts',(-11.9556833500695,20.3587923509042,
-1.86903403241728));
#281287=CARTESIAN_POINT('Ctrl Pts',(-11.6119070931413,20.295399444133,-3.40514267636605));
#281288=CARTESIAN_POINT('Ctrl Pts',(-10.35902432988,20.1701813383277,-6.2529227016142));
#281289=CARTESIAN_POINT('Ctrl Pts',(-9.46441833361632,20.1117319099718,
-7.53878230791702));
#281290=CARTESIAN_POINT('Ctrl Pts',(-7.21306010861394,19.9861957242991,
-9.71991583093426));
#281291=CARTESIAN_POINT('Ctrl Pts',(-5.86957419396658,19.9216485775948,
-10.585521565293));
#281292=CARTESIAN_POINT('Ctrl Pts',(-2.95624811735045,19.7990313393556,
-11.7327679869781));
#281293=CARTESIAN_POINT('Ctrl Pts',(-1.41931771994306,19.7386626077233,
-12.0159453206607));
#281294=CARTESIAN_POINT('Ctrl Pts',(1.69593633306617,19.6126479341898,-11.9824678079457));
#281295=CARTESIAN_POINT('Ctrl Pts',(3.24454879133492,19.5522762116259,-11.6588423345282));
#281296=CARTESIAN_POINT('Ctrl Pts',(6.13148551909505,19.4286756336056,-10.4339163048501));
#281297=CARTESIAN_POINT('Ctrl Pts',(7.44170862444592,19.3646323669676,-9.54372067535896));
#281298=CARTESIAN_POINT('Ctrl Pts',(9.62973473413392,19.2402839235789,-7.3253726195877));
#281299=CARTESIAN_POINT('Ctrl Pts',(10.4928495817328,19.1818528803588,-6.02436208656314));
#281300=CARTESIAN_POINT('Ctrl Pts',(11.6946057288648,19.055306199693,-3.1254356055251));
#281301=CARTESIAN_POINT('Ctrl Pts',(12.0055053537683,18.9909082436387,-1.54894227591795));
#281302=CARTESIAN_POINT('Ctrl Pts',(11.9944702690204,18.8697051689437,1.59797350470092));
#281303=CARTESIAN_POINT('Ctrl Pts',(11.6864647086555,18.8066086521192,3.13800051799432));
#281304=CARTESIAN_POINT('Ctrl Pts',(10.5001757326045,18.681150214187,6.01366526768752));
#281305=CARTESIAN_POINT('Ctrl Pts',(9.63342952707142,18.6224118895613,7.32222245543705));
#281306=CARTESIAN_POINT('Ctrl Pts',(7.43201979404881,18.497331420033,9.55293744733466));
#281307=CARTESIAN_POINT('Ctrl Pts',(6.11180773001238,18.4328697420344,10.4469822042804));
#281308=CARTESIAN_POINT('Ctrl Pts',(3.23067082932968,18.3097418498919,11.6600105573142));
#281309=CARTESIAN_POINT('Ctrl Pts',(1.70220670810676,18.2501057076766,11.9789655069456));
#281310=CARTESIAN_POINT('Ctrl Pts',(-1.41712493239928,18.123926092264,12.0193549813857));
#281311=CARTESIAN_POINT('Ctrl Pts',(-2.97836974245961,18.0626884446831,
11.730401092986));
#281312=CARTESIAN_POINT('Ctrl Pts',(-5.89377845052369,17.9396780981733,
10.5694876277066));
#281313=CARTESIAN_POINT('Ctrl Pts',(-7.220870844797,17.8758440713655,9.71131089359237));
#281314=CARTESIAN_POINT('Ctrl Pts',(-9.45812750288978,17.7511431824503,
7.54589954829269));
#281315=CARTESIAN_POINT('Ctrl Pts',(-10.3517296478602,17.6928382996723,
6.26405976887067));
#281316=CARTESIAN_POINT('Ctrl Pts',(-11.6191706884262,17.5665872700776,
3.3941606319504));
#281317=CARTESIAN_POINT('Ctrl Pts',(-11.9660729768364,17.5019703064257,
1.82725008201508));
#281318=CARTESIAN_POINT('Ctrl Pts',(-11.9992118536821,17.4373707362562,
0.158843738507581));
#281319=CARTESIAN_POINT('Ctrl Pts',(-12.,17.4343048005603,0.0794051911696823));
#281320=CARTESIAN_POINT('Ctrl Pts',(-12.,17.43124999994,2.93915231795365E-15));
#281321=CARTESIAN_POINT('Ctrl Pts',(-12.,17.80624999994,1.41553435639707E-14));
#281322=CARTESIAN_POINT('Ctrl Pts',(-12.,17.8623465268447,1.45814931853264));
#281323=CARTESIAN_POINT('Ctrl Pts',(-11.734218240322,17.9213402806445,2.90525019506248));
#281324=CARTESIAN_POINT('Ctrl Pts',(-10.6644227558352,18.0428057517025,
5.71497448793998));
#281325=CARTESIAN_POINT('Ctrl Pts',(-9.84009188195503,18.101617930102,7.04013335853222));
#281326=CARTESIAN_POINT('Ctrl Pts',(-7.71546696621803,18.2254625856327,
9.32455711532062));
#281327=CARTESIAN_POINT('Ctrl Pts',(-6.42766033170131,18.2897245176208,
10.254803104201));
#281328=CARTESIAN_POINT('Ctrl Pts',(-3.57786992657996,18.4140201366153,
11.5600890339221));
#281329=CARTESIAN_POINT('Ctrl Pts',(-2.04534881871437,18.4735139022491,
11.9269998087708));
#281330=CARTESIAN_POINT('Ctrl Pts',(1.06421374343355,18.5992983501411,12.0529391494687));
#281331=CARTESIAN_POINT('Ctrl Pts',(2.61155160394646,18.6608047950825,11.8146224045516));
#281332=CARTESIAN_POINT('Ctrl Pts',(5.56379596545282,18.7827296562989,10.7500627379407));
#281333=CARTESIAN_POINT('Ctrl Pts',(6.93541654357681,18.8473368381549,9.92065605796218));
#281334=CARTESIAN_POINT('Ctrl Pts',(9.24804821503675,18.9733897874021,7.80212390376018));
#281335=CARTESIAN_POINT('Ctrl Pts',(10.1769150740052,19.0316892688132,6.54445894792941));
#281336=CARTESIAN_POINT('Ctrl Pts',(11.5114761381718,19.1565539965407,3.73240337121364));
#281337=CARTESIAN_POINT('Ctrl Pts',(11.8993775818987,19.2202692144908,2.20225384953143));
#281338=CARTESIAN_POINT('Ctrl Pts',(12.0670171356895,19.3429651122583,-0.932581864117961));
#281339=CARTESIAN_POINT('Ctrl Pts',(11.8404541475837,19.4047021708096,-2.50728436645661));
#281340=CARTESIAN_POINT('Ctrl Pts',(10.8014812183748,19.5309596803679,-5.45158573014176));
#281341=CARTESIAN_POINT('Ctrl Pts',(10.0097370355131,19.590281420537,-6.79683341854125));
#281342=CARTESIAN_POINT('Ctrl Pts',(7.93898916468252,19.7136563001511,-9.13565450066491));
#281343=CARTESIAN_POINT('Ctrl Pts',(6.67080256472679,19.7780610985413,-10.0989138953897));
#281344=CARTESIAN_POINT('Ctrl Pts',(3.85297940085754,19.9028929174297,-11.4707507153434));
#281345=CARTESIAN_POINT('Ctrl Pts',(2.33397058749204,19.9618389064488,-11.8733358465505));
#281346=CARTESIAN_POINT('Ctrl Pts',(-0.770408670177771,20.0874136852702,
-12.0756783444384));
#281347=CARTESIAN_POINT('Ctrl Pts',(-2.32618338058681,20.1500423328747,
-11.8744996390425));
#281348=CARTESIAN_POINT('Ctrl Pts',(-5.30942924959274,20.2713517207859,
-10.8784957640785));
#281349=CARTESIAN_POINT('Ctrl Pts',(-6.70343678962387,20.3359696460101,
-10.079450243893));
#281350=CARTESIAN_POINT('Ctrl Pts',(-9.06562792711455,20.4624049835879,
-8.01304816733746));
#281351=CARTESIAN_POINT('Ctrl Pts',(-10.0223073212644,20.5207532078552,
-6.77849117207222));
#281352=CARTESIAN_POINT('Ctrl Pts',(-11.332244142844,20.6372210020077,-4.17670102245711));
#281353=CARTESIAN_POINT('Ctrl Pts',(-11.7336475631444,20.6928494368794,
-2.86114296700866));
#281354=CARTESIAN_POINT('Ctrl Pts',(-11.9683983166688,20.7671550289339,
-1.0059500786248));
#281355=CARTESIAN_POINT('Ctrl Pts',(-12.,20.7869061651797,-0.502815432834886));
#281356=CARTESIAN_POINT('Ctrl Pts',(-12.,20.806249999928,1.63757896132211E-14));
#281357=CARTESIAN_POINT('Origin',(-3.46944695195361E-15,49.3876222290585,
0.));
#281358=CARTESIAN_POINT('',(44.1739130434783,2.43125000000001,5.40974412145092E-15));
#281359=CARTESIAN_POINT('Origin',(7.22658086056641E-16,2.43125000000001,
0.));
#281360=CARTESIAN_POINT('Origin',(0.,-9.56874999999999,0.));
#281361=CARTESIAN_POINT('',(-22.0315642065426,2.43125000000001,0.));
#281362=CARTESIAN_POINT('Origin',(4.95183270959582E-16,2.43125000000001,
0.));
#281363=CARTESIAN_POINT('',(-8.01975608296216,9.72176245732409,-13.890625));
#281364=CARTESIAN_POINT('',(-16.0395121659243,9.72176245732407,1.30104260698261E-14));
#281365=CARTESIAN_POINT('Origin',(-12.0296341244432,-9.56874999999999,-6.94531250000001));
#281366=CARTESIAN_POINT('',(8.01975608296213,9.7217624573241,-13.890625));
#281367=CARTESIAN_POINT('Origin',(6.00925839494864E-15,-9.56874999999999,
-13.890625));
#281368=CARTESIAN_POINT('',(16.0395121659243,9.7217624573241,-3.46944695195361E-15));
#281369=CARTESIAN_POINT('Origin',(12.0296341244432,-9.56874999999999,-6.94531249999999));
#281370=CARTESIAN_POINT('',(8.01975608296214,9.7217624573241,13.890625));
#281371=CARTESIAN_POINT('Origin',(12.0296341244432,-9.56874999999999,6.94531249999999));
#281372=CARTESIAN_POINT('',(-8.01975608296215,9.72176245732409,13.890625));
#281373=CARTESIAN_POINT('Origin',(0.,-9.56874999999999,13.890625));
#281374=CARTESIAN_POINT('Origin',(-12.0296341244432,-9.56874999999999,6.94531250000002));
#281375=CARTESIAN_POINT('Origin',(0.,21.43125,0.));
#281376=CARTESIAN_POINT('',(-8.01975608296215,17.0122749146482,13.890625));
#281377=CARTESIAN_POINT('',(8.01975608296214,17.0122749146482,13.890625));
#281378=CARTESIAN_POINT('Ctrl Pts',(8.01975608295684,17.012274914652,13.890625));
#281379=CARTESIAN_POINT('Ctrl Pts',(-1.37667655053519E-14,22.7389742468655,
13.890625));
#281380=CARTESIAN_POINT('Ctrl Pts',(-8.01975608295687,17.0122749146519,
13.890625));
#281381=CARTESIAN_POINT('',(16.0395121659243,17.0122749146482,-6.01981791101278E-16));
#281382=CARTESIAN_POINT('Ctrl Pts',(8.01975608296478,17.0122749146519,13.8906249999954));
#281383=CARTESIAN_POINT('Ctrl Pts',(12.0296341244432,22.7389742468655,6.9453125));
#281384=CARTESIAN_POINT('Ctrl Pts',(16.0395121659216,17.012274914652,4.58946936354325E-12));
#281385=CARTESIAN_POINT('',(8.01975608296213,17.0122749146482,-13.890625));
#281386=CARTESIAN_POINT('Ctrl Pts',(16.0395121659216,17.0122749146519,-4.58054260572454E-12));
#281387=CARTESIAN_POINT('Ctrl Pts',(12.0296341244432,22.7389742468655,-6.9453125));
#281388=CARTESIAN_POINT('Ctrl Pts',(8.01975608296477,17.0122749146519,-13.8906249999954));
#281389=CARTESIAN_POINT('',(4.73454552372624E-15,20.0812038373766,-13.890625));
#281390=CARTESIAN_POINT('Ctrl Pts',(8.01975608295685,17.0122749146519,-13.890625));
#281391=CARTESIAN_POINT('Ctrl Pts',(3.72198175111144,20.0812038373766,-13.890625));
#281392=CARTESIAN_POINT('Ctrl Pts',(7.76798010301187E-15,20.0812038373766,
-13.890625));
#281393=CARTESIAN_POINT('',(1.58534355170872E-15,21.43125,-12.9453125));
#281394=CARTESIAN_POINT('',(1.58534355170872E-15,21.43125,-12.9453125));
#281395=CARTESIAN_POINT('Origin',(0.,21.43125,0.));
#281396=CARTESIAN_POINT('',(-8.01975608296216,17.0122749146481,-13.890625));
#281397=CARTESIAN_POINT('Ctrl Pts',(7.76798010301187E-15,20.0812038373766,
-13.890625));
#281398=CARTESIAN_POINT('Ctrl Pts',(-3.72198175111144,20.0812038373766,
-13.890625));
#281399=CARTESIAN_POINT('Ctrl Pts',(-8.01975608295688,17.0122749146519,
-13.890625));
#281400=CARTESIAN_POINT('',(-16.0395121659243,17.0122749146481,1.30536815232815E-14));
#281401=CARTESIAN_POINT('Ctrl Pts',(-8.01975608296479,17.0122749146519,
-13.8906249999954));
#281402=CARTESIAN_POINT('Ctrl Pts',(-12.0296341244432,22.7389742468655,
-6.9453125));
#281403=CARTESIAN_POINT('Ctrl Pts',(-16.0395121659217,17.0122749146519,
-4.55934155590512E-12));
#281404=CARTESIAN_POINT('Ctrl Pts',(-16.0395121659217,17.0122749146519,
4.55859765942022E-12));
#281405=CARTESIAN_POINT('Ctrl Pts',(-12.0296341244432,22.7389742468655,
6.9453125));
#281406=CARTESIAN_POINT('Ctrl Pts',(-8.01975608296479,17.0122749146519,
13.8906249999954));
#281407=CARTESIAN_POINT('Origin',(-1.38777878078145E-14,20.90625,0.));
#281408=CARTESIAN_POINT('',(-1.95755827123136E-14,20.3673715931731,-11.461121593173));
#281409=CARTESIAN_POINT('Ctrl Pts',(-11.7339375393676,20.90625,2.51290863785773));
#281410=CARTESIAN_POINT('Ctrl Pts',(-11.9751037228422,20.8729010024019,
1.2275388253564));
#281411=CARTESIAN_POINT('Ctrl Pts',(-12.0064975767267,20.8411511224719,
-0.0964311651186414));
#281412=CARTESIAN_POINT('Ctrl Pts',(-11.6381351713344,20.7755984205093,
-2.65589242107953));
#281413=CARTESIAN_POINT('Ctrl Pts',(-11.254907610849,20.7423798220322,-3.8780745371738));
#281414=CARTESIAN_POINT('Ctrl Pts',(-10.0336965717947,20.6719176402762,
-6.31370393917634));
#281415=CARTESIAN_POINT('Ctrl Pts',(-9.10186287045269,20.6340528713554,
-7.57878102606151));
#281416=CARTESIAN_POINT('Ctrl Pts',(-6.72218311670212,20.5519138071734,
-9.62438013593598));
#281417=CARTESIAN_POINT('Ctrl Pts',(-5.42418150086199,20.5124695780735,
-10.3671437985956));
#281418=CARTESIAN_POINT('Ctrl Pts',(-2.63477883810742,20.4369825184929,
-11.3209167902397));
#281419=CARTESIAN_POINT('Ctrl Pts',(-1.26957078800877,20.4014603019892,
-11.4952103019892));
#281420=CARTESIAN_POINT('Ctrl Pts',(-3.4555691641458E-14,20.3673715931731,
-11.461121593173));
#281421=CARTESIAN_POINT('',(-1.54116579237465E-14,21.43125,-12.525));
#281422=CARTESIAN_POINT('',(-1.53473639667913E-14,20.90625,-12.));
#281423=CARTESIAN_POINT('Origin',(-1.38777878078145E-14,21.43125,0.));
#281424=CARTESIAN_POINT('Ctrl Pts',(-3.34454686168328E-14,20.3673715931731,
-11.461121593173));
#281425=CARTESIAN_POINT('Ctrl Pts',(0.158753063369545,20.3631089817441,
-11.456858981744));
#281426=CARTESIAN_POINT('Ctrl Pts',(0.316010936333406,20.3588817583139,
-11.4493328807581));
#281427=CARTESIAN_POINT('Ctrl Pts',(1.94465535673269,20.3150547579429,-11.3383180821017));
#281428=CARTESIAN_POINT('Ctrl Pts',(3.39261700236661,20.277278273539,-10.9535572953072));
#281429=CARTESIAN_POINT('Ctrl Pts',(6.03062359817187,20.1990638465944,-9.65839939732408));
#281430=CARTESIAN_POINT('Ctrl Pts',(7.20257467898127,20.15889608411,-8.76757326626974));
#281431=CARTESIAN_POINT('Ctrl Pts',(9.15722478991995,20.0796650678951,-6.57145272022985));
#281432=CARTESIAN_POINT('Ctrl Pts',(9.91561896638193,20.0412329954549,-5.27980368737507));
#281433=CARTESIAN_POINT('Ctrl Pts',(10.8951016967142,19.9572267702433,-2.41007461461997));
#281434=CARTESIAN_POINT('Ctrl Pts',(11.055757000172,19.9173988404041,-0.940533523605604));
#281435=CARTESIAN_POINT('Ctrl Pts',(10.8761591813622,19.8435344687281,1.79187774688301));
#281436=CARTESIAN_POINT('Ctrl Pts',(10.5287658487941,19.8047358903491,3.13038442126089));
#281437=CARTESIAN_POINT('Ctrl Pts',(9.36849149367791,19.7283234991857,5.58068678118078));
#281438=CARTESIAN_POINT('Ctrl Pts',(8.5319769564679,19.6901718697845,6.77150405317055));
#281439=CARTESIAN_POINT('Ctrl Pts',(6.35602709403731,19.6072340141407,8.71949207523714));
#281440=CARTESIAN_POINT('Ctrl Pts',(5.15415641864755,19.5670375971829,9.43423088151185));
#281441=CARTESIAN_POINT('Ctrl Pts',(3.19699827938916,19.5088390625049,10.1327998304645));
#281442=CARTESIAN_POINT('Ctrl Pts',(2.52327522205536,19.4898163385168,10.3018141492848));
#281443=CARTESIAN_POINT('Ctrl Pts',(0.50150453708759,19.4312152241487,10.5990933398486));
#281444=CARTESIAN_POINT('Ctrl Pts',(-0.858157973261501,19.3913667357374,
10.5365366445161));
#281445=CARTESIAN_POINT('Ctrl Pts',(-3.49187560718385,19.3133023101555,
9.89775066976008));
#281446=CARTESIAN_POINT('Ctrl Pts',(-4.7388067620056,19.2752321029848,9.3230150982916));
#281447=CARTESIAN_POINT('Ctrl Pts',(-6.38216076388607,19.214649651135,8.12285448752604));
#281448=CARTESIAN_POINT('Ctrl Pts',(-6.88402838863904,19.1946133285548,
7.67529956416046));
#281449=CARTESIAN_POINT('Ctrl Pts',(-8.17460081443321,19.1383957584764,
6.27619662308116));
#281450=CARTESIAN_POINT('Ctrl Pts',(-8.84515327331929,19.103594295001,5.22343353132837));
#281451=CARTESIAN_POINT('Ctrl Pts',(-9.75620235107338,19.0300319619295,
2.95820155339676));
#281452=CARTESIAN_POINT('Ctrl Pts',(-10.0025670660582,18.9932662710101,
1.7720386495763));
#281453=CARTESIAN_POINT('Ctrl Pts',(-10.0352413152989,18.9576928414942,
0.570469052221604));
#281454=CARTESIAN_POINT('Ctrl Pts',(-7.47704554734297,18.9576928414942,
-6.71753623576258));
#281455=CARTESIAN_POINT('Ctrl Pts',(-8.22914229169097,19.0695296791179,
-6.04774602181526));
#281456=CARTESIAN_POINT('Ctrl Pts',(-8.78589634872411,19.1631164093256,
-5.34312658694975));
#281457=CARTESIAN_POINT('Ctrl Pts',(-9.6773533567784,19.3393049469732,-3.99501404107446));
#281458=CARTESIAN_POINT('Ctrl Pts',(-10.0676634679168,19.4352867858775,
-3.2040722529385));
#281459=CARTESIAN_POINT('Ctrl Pts',(-10.9065983101053,19.7103902849491,
-0.775444565914872));
#281460=CARTESIAN_POINT('Ctrl Pts',(-10.9837592295337,19.8520315258032,
0.697500172039842));
#281461=CARTESIAN_POINT('Ctrl Pts',(-10.8105004116642,20.1219190682211,
3.33356522839727));
#281462=CARTESIAN_POINT('Ctrl Pts',(-10.4176784074616,20.2734600759145,
4.78318445517766));
#281463=CARTESIAN_POINT('Ctrl Pts',(-9.36828133989022,20.4995570830846,
6.8826953758291));
#281464=CARTESIAN_POINT('Ctrl Pts',(-8.89210207419248,20.5800256968209,
7.61064915299536));
#281465=CARTESIAN_POINT('Ctrl Pts',(-7.81751963755748,20.7432184861572,
8.92850556434733));
#281466=CARTESIAN_POINT('Ctrl Pts',(-7.21026201465552,20.8252469301455,
9.52852756505014));
#281467=CARTESIAN_POINT('Ctrl Pts',(-6.5440620647558,20.90625,10.0585909397204));
#281468=CARTESIAN_POINT('Origin',(0.,21.43125,0.));
#281469=CARTESIAN_POINT('Origin',(-8.01975608296216,21.43125,-13.890625));
#281470=CARTESIAN_POINT('',(-8.01975608296216,21.43125,-13.890625));
#281471=CARTESIAN_POINT('',(-16.0395121659243,21.43125,1.21746868952018E-14));
#281472=CARTESIAN_POINT('Origin',(-16.0395121659243,21.43125,1.21746868952018E-14));
#281473=CARTESIAN_POINT('',(-8.01975608296215,21.43125,13.890625));
#281474=CARTESIAN_POINT('Origin',(-8.01975608296215,21.43125,13.890625));
#281475=CARTESIAN_POINT('',(8.01975608296214,21.43125,13.890625));
#281476=CARTESIAN_POINT('Origin',(8.01975608296214,21.43125,13.890625));
#281477=CARTESIAN_POINT('',(16.0395121659243,21.43125,-2.37169225231204E-15));
#281478=CARTESIAN_POINT('Origin',(16.0395121659243,21.43125,-2.37169225231204E-15));
#281479=CARTESIAN_POINT('',(8.01975608296213,21.43125,-13.890625));
#281480=CARTESIAN_POINT('Origin',(8.01975608296213,21.43125,-13.890625));
#281481=CARTESIAN_POINT('Origin',(-44.1739130434783,2.43125000000001,0.));
#281482=CARTESIAN_POINT('Origin',(-1.38777878078145E-14,2.43125000000001,
0.));
#281483=CARTESIAN_POINT('Ctrl Pts',(10.0514428414954,2.43125000000002,1.00752739484733E-13));
#281484=CARTESIAN_POINT('Ctrl Pts',(10.1143780835885,2.43125000000002,-0.791127473640706));
#281485=CARTESIAN_POINT('Ctrl Pts',(10.0855072982437,2.43125000000002,-1.58682843497015));
#281486=CARTESIAN_POINT('Ctrl Pts',(9.84523379682252,2.43125000000002,-3.15557179232318));
#281487=CARTESIAN_POINT('Ctrl Pts',(9.63470068842676,2.43125000000002,-3.92325055631404));
#281488=CARTESIAN_POINT('Ctrl Pts',(8.67230516055593,2.43125000000002,-6.30994543448733));
#281489=CARTESIAN_POINT('Ctrl Pts',(7.71286120753459,2.43125000000002,-7.46066276667367));
#281490=CARTESIAN_POINT('Ctrl Pts',(6.06627958599162,2.43125000000002,-9.1152206243862));
#281491=CARTESIAN_POINT('Ctrl Pts',(4.9464571378071,2.43125000000001,-9.88345895797583));
#281492=CARTESIAN_POINT('Ctrl Pts',(2.75597210659317,2.43125000000001,-10.8484833593829));
#281493=CARTESIAN_POINT('Ctrl Pts',(1.37406648240357,2.43125000000002,-11.29221051564));
#281494=CARTESIAN_POINT('Ctrl Pts',(-1.98461349922251,2.43125000000001,
-11.4457083135333));
#281495=CARTESIAN_POINT('Ctrl Pts',(-3.50022085878334,2.43125000000001,
-11.1473855441023));
#281496=CARTESIAN_POINT('Ctrl Pts',(-6.14735486447011,2.43125000000001,
-10.1719281614562));
#281497=CARTESIAN_POINT('Ctrl Pts',(-7.38835529811323,2.43125000000001,
-9.4385927042382));
#281498=CARTESIAN_POINT('Ctrl Pts',(-8.46872171229246,2.43125000000001,
-8.50180878165033));
#281499=CARTESIAN_POINT('Ctrl Pts',(-12.,2.43125000000001,1.10592091040473E-12));
#281500=CARTESIAN_POINT('Ctrl Pts',(-11.8804643241478,2.43125000000001,
1.79391945396996));
#281501=CARTESIAN_POINT('Ctrl Pts',(-11.3990610613138,2.43125000000001,
3.13396898737023));
#281502=CARTESIAN_POINT('Ctrl Pts',(-10.4104157884427,2.43125000000001,
5.318570795906));
#281503=CARTESIAN_POINT('Ctrl Pts',(-9.57359601299618,2.43125000000001,
6.56829747585552));
#281504=CARTESIAN_POINT('Ctrl Pts',(-7.38873844522587,2.43125000000001,
8.65742934749614));
#281505=CARTESIAN_POINT('Ctrl Pts',(-6.14298665404833,2.43125,9.45156675706131));
#281506=CARTESIAN_POINT('Ctrl Pts',(-3.8073824930157,2.43125,10.362657594245));
#281507=CARTESIAN_POINT('Ctrl Pts',(-2.35484140538957,2.43125000000001,
10.778449175978));
#281508=CARTESIAN_POINT('Ctrl Pts',(1.15015301169903,2.43125000000001,10.6841950237441));
#281509=CARTESIAN_POINT('Ctrl Pts',(2.53388342843634,2.43125000000001,10.2413561793839));
#281510=CARTESIAN_POINT('Ctrl Pts',(4.18319669729398,2.43125000000002,9.5097960999229));
#281511=CARTESIAN_POINT('Ctrl Pts',(4.85072362354194,2.43125000000002,9.11749903031561));
#281512=CARTESIAN_POINT('Ctrl Pts',(6.06416700972034,2.43125000000002,8.20405583130882));
#281513=CARTESIAN_POINT('Ctrl Pts',(6.60953367471901,2.43125000000002,7.69028293020246));
#281514=CARTESIAN_POINT('Ctrl Pts',(7.09357268597975,2.43125000000002,7.12128708482873));
#281515=CARTESIAN_POINT('Ctrl Pts',(-10.0514365206283,-1.69375364933639,
2.46189191236404E-15));
#281516=CARTESIAN_POINT('Ctrl Pts',(-10.0514365206283,-1.54375364933699,
3.26590970098687));
#281517=CARTESIAN_POINT('Ctrl Pts',(-8.13178296306926,-1.39375364933759,
5.90808615117926));
#281518=CARTESIAN_POINT('Ctrl Pts',(-6.21212940551025,-1.24375364933819,
8.55026260137164));
#281519=CARTESIAN_POINT('Ctrl Pts',(-3.10606470275513,-1.09375364933879,
9.55948420107058));
#281520=CARTESIAN_POINT('Ctrl Pts',(-9.99267301601491E-15,-0.943753649339386,
10.5687058007695));
#281521=CARTESIAN_POINT('Ctrl Pts',(3.10606470275511,-0.793753649339984,
9.55948420107058));
#281522=CARTESIAN_POINT('Ctrl Pts',(6.21212940551023,-0.643753649340582,
8.55026260137164));
#281523=CARTESIAN_POINT('Ctrl Pts',(8.13178296306923,-0.493753649341181,
5.90808615117925));
#281524=CARTESIAN_POINT('Ctrl Pts',(10.0514365206282,-0.34375364934178,
3.26590970098687));
#281525=CARTESIAN_POINT('Ctrl Pts',(10.0514365206282,-0.19375364934238,
-1.23094595618202E-15));
#281526=CARTESIAN_POINT('Ctrl Pts',(10.0514365206282,-0.0437536493429801,
-3.26590970098687));
#281527=CARTESIAN_POINT('Ctrl Pts',(8.13178296306923,0.106246350656419,
-5.90808615117926));
#281528=CARTESIAN_POINT('Ctrl Pts',(6.21212940551023,0.256246350655818,
-8.55026260137164));
#281529=CARTESIAN_POINT('Ctrl Pts',(3.10606470275511,0.406246350655216,
-9.55948420107058));
#281530=CARTESIAN_POINT('Ctrl Pts',(-1.34451139978543E-14,0.556246350654614,
-10.5687058007695));
#281531=CARTESIAN_POINT('Ctrl Pts',(-3.10606470275513,0.706246350654012,
-9.55948420107058));
#281532=CARTESIAN_POINT('Ctrl Pts',(-6.21212940551025,0.85624635065341,
-8.55026260137164));
#281533=CARTESIAN_POINT('Ctrl Pts',(-8.13178296306926,1.00624635065281,
-5.90808615117925));
#281534=CARTESIAN_POINT('Ctrl Pts',(-10.0514365206283,1.15624635065221,
-3.26590970098687));
#281535=CARTESIAN_POINT('Ctrl Pts',(-10.0514365206283,1.30624635065161,
2.46189191236404E-15));
#281536=CARTESIAN_POINT('Ctrl Pts',(-10.0514365206283,1.45624635065101,
3.26590970098687));
#281537=CARTESIAN_POINT('Ctrl Pts',(-8.13178296306926,1.60624635065041,
5.90808615117926));
#281538=CARTESIAN_POINT('Ctrl Pts',(-6.21212940551025,1.75624635064981,
8.55026260137164));
#281539=CARTESIAN_POINT('Ctrl Pts',(-3.10606470275513,1.90624635064921,
9.55948420107058));
#281540=CARTESIAN_POINT('Ctrl Pts',(-1.17203822876767E-14,2.05624635064861,
10.5687058007695));
#281541=CARTESIAN_POINT('Ctrl Pts',(3.10606470275511,2.20624635064802,9.55948420107058));
#281542=CARTESIAN_POINT('Ctrl Pts',(6.21212940551023,2.35624635064742,8.55026260137164));
#281543=CARTESIAN_POINT('Ctrl Pts',(8.13178296306923,2.50624635064682,5.90808615117925));
#281544=CARTESIAN_POINT('Ctrl Pts',(10.0514365206282,2.65624635064622,3.26590970098687));
#281545=CARTESIAN_POINT('Ctrl Pts',(10.0514365206282,2.80624635064562,-1.23094595618202E-15));
#281546=CARTESIAN_POINT('Ctrl Pts',(10.0514365206282,2.95624635064502,-3.26590970098687));
#281547=CARTESIAN_POINT('Ctrl Pts',(8.13178296306923,3.10624635064442,-5.90808615117926));
#281548=CARTESIAN_POINT('Ctrl Pts',(6.21212940551023,3.25624635064382,-8.55026260137164));
#281549=CARTESIAN_POINT('Ctrl Pts',(3.10606470275511,3.40624635064322,-9.55948420107058));
#281550=CARTESIAN_POINT('Ctrl Pts',(-1.51728232695162E-14,3.55624635064261,
-10.5687058007695));
#281551=CARTESIAN_POINT('Ctrl Pts',(-3.10606470275514,3.70624635064201,
-9.55948420107058));
#281552=CARTESIAN_POINT('Ctrl Pts',(-6.21212940551026,3.85624635064141,
-8.55026260137164));
#281553=CARTESIAN_POINT('Ctrl Pts',(-8.13178296306926,4.00624635064081,
-5.90808615117925));
#281554=CARTESIAN_POINT('Ctrl Pts',(-10.0514365206283,4.15624635064021,
-3.26590970098687));
#281555=CARTESIAN_POINT('Ctrl Pts',(-10.0514365206283,4.30624635063961,
2.46189191236404E-15));
#281556=CARTESIAN_POINT('Ctrl Pts',(-10.0514365206283,4.45624635063901,
3.26590970098687));
#281557=CARTESIAN_POINT('Ctrl Pts',(-8.13178296306926,4.60624635063841,
5.90808615117926));
#281558=CARTESIAN_POINT('Ctrl Pts',(-6.21212940551025,4.75624635063781,
8.55026260137164));
#281559=CARTESIAN_POINT('Ctrl Pts',(-3.10606470275513,4.90624635063721,
9.55948420107058));
#281560=CARTESIAN_POINT('Ctrl Pts',(-1.34480915593386E-14,5.05624635063661,
10.5687058007695));
#281561=CARTESIAN_POINT('Ctrl Pts',(3.10606470275511,5.20624635063602,9.55948420107058));
#281562=CARTESIAN_POINT('Ctrl Pts',(6.21212940551023,5.35624635063542,8.55026260137164));
#281563=CARTESIAN_POINT('Ctrl Pts',(8.13178296306923,5.50624635063482,5.90808615117925));
#281564=CARTESIAN_POINT('Ctrl Pts',(10.0514365206282,5.65624635063422,3.26590970098687));
#281565=CARTESIAN_POINT('Ctrl Pts',(10.0514365206282,5.80624635063362,-1.23094595618202E-15));
#281566=CARTESIAN_POINT('Ctrl Pts',(10.0514365206282,5.95624635063302,-3.26590970098687));
#281567=CARTESIAN_POINT('Ctrl Pts',(8.13178296306923,6.10624635063242,-5.90808615117926));
#281568=CARTESIAN_POINT('Ctrl Pts',(6.21212940551023,6.25624635063182,-8.55026260137164));
#281569=CARTESIAN_POINT('Ctrl Pts',(3.1060647027551,6.40624635063122,-9.55948420107058));
#281570=CARTESIAN_POINT('Ctrl Pts',(-1.6900532541178E-14,6.55624635063061,
-10.5687058007695));
#281571=CARTESIAN_POINT('Ctrl Pts',(-3.10606470275514,6.70624635063001,
-9.55948420107058));
#281572=CARTESIAN_POINT('Ctrl Pts',(-6.21212940551026,6.85624635062941,
-8.55026260137164));
#281573=CARTESIAN_POINT('Ctrl Pts',(-8.13178296306926,7.00624635062881,
-5.90808615117925));
#281574=CARTESIAN_POINT('Ctrl Pts',(-10.0514365206283,7.15624635062821,
-3.26590970098687));
#281575=CARTESIAN_POINT('Ctrl Pts',(-10.0514365206283,7.30624635062761,
2.46189191236404E-15));
#281576=CARTESIAN_POINT('Ctrl Pts',(-10.0514365206283,7.45624635062701,
3.26590970098687));
#281577=CARTESIAN_POINT('Ctrl Pts',(-8.13178296306926,7.60624635062641,
5.90808615117926));
#281578=CARTESIAN_POINT('Ctrl Pts',(-6.21212940551025,7.75624635062581,
8.55026260137164));
#281579=CARTESIAN_POINT('Ctrl Pts',(-3.10606470275514,7.90624635062521,
9.55948420107058));
#281580=CARTESIAN_POINT('Ctrl Pts',(-1.51758008310004E-14,8.05624635062462,
10.5687058007695));
#281581=CARTESIAN_POINT('Ctrl Pts',(3.1060647027551,8.20624635062402,9.55948420107058));
#281582=CARTESIAN_POINT('Ctrl Pts',(6.21212940551023,8.35624635062342,8.55026260137164));
#281583=CARTESIAN_POINT('Ctrl Pts',(8.13178296306923,8.50624635062282,5.90808615117925));
#281584=CARTESIAN_POINT('Ctrl Pts',(10.0514365206282,8.65624635062222,3.26590970098687));
#281585=CARTESIAN_POINT('Ctrl Pts',(10.0514365206282,8.80624635062162,-1.23094595618202E-15));
#281586=CARTESIAN_POINT('Ctrl Pts',(10.0514365206282,8.95624635062102,-3.26590970098687));
#281587=CARTESIAN_POINT('Ctrl Pts',(8.13178296306923,9.10624635062042,-5.90808615117926));
#281588=CARTESIAN_POINT('Ctrl Pts',(6.21212940551022,9.25624635061982,-8.55026260137164));
#281589=CARTESIAN_POINT('Ctrl Pts',(3.1060647027551,9.40624635061922,-9.55948420107058));
#281590=CARTESIAN_POINT('Ctrl Pts',(-1.86282418128398E-14,9.55624635061861,
-10.5687058007695));
#281591=CARTESIAN_POINT('Ctrl Pts',(-3.10606470275514,9.70624635061801,
-9.55948420107058));
#281592=CARTESIAN_POINT('Ctrl Pts',(-6.21212940551026,9.85624635061741,
-8.55026260137164));
#281593=CARTESIAN_POINT('Ctrl Pts',(-8.13178296306926,10.0062463506168,
-5.90808615117925));
#281594=CARTESIAN_POINT('Ctrl Pts',(-10.0514365206283,10.1562463506162,
-3.26590970098687));
#281595=CARTESIAN_POINT('Ctrl Pts',(-10.0514365206283,10.3062463506156,
2.46189191236404E-15));
#281596=CARTESIAN_POINT('Ctrl Pts',(-10.0514365206283,10.456246350615,3.26590970098687));
#281597=CARTESIAN_POINT('Ctrl Pts',(-8.13178296306926,10.6062463506144,
5.90808615117926));
#281598=CARTESIAN_POINT('Ctrl Pts',(-6.21212940551026,10.7562463506138,
8.55026260137164));
#281599=CARTESIAN_POINT('Ctrl Pts',(-3.10606470275514,10.9062463506132,
9.55948420107058));
#281600=CARTESIAN_POINT('Ctrl Pts',(-1.69035101026623E-14,11.0562463506126,
10.5687058007695));
#281601=CARTESIAN_POINT('Ctrl Pts',(3.1060647027551,11.206246350612,9.55948420107058));
#281602=CARTESIAN_POINT('Ctrl Pts',(6.21212940551022,11.3562463506114,8.55026260137164));
#281603=CARTESIAN_POINT('Ctrl Pts',(8.13178296306923,11.5062463506108,5.90808615117925));
#281604=CARTESIAN_POINT('Ctrl Pts',(10.0514365206282,11.6562463506102,3.26590970098687));
#281605=CARTESIAN_POINT('Ctrl Pts',(10.0514365206282,11.8062463506096,-1.23094595618202E-15));
#281606=CARTESIAN_POINT('Ctrl Pts',(10.0514365206282,11.956246350609,-3.26590970098687));
#281607=CARTESIAN_POINT('Ctrl Pts',(8.13178296306923,12.1062463506084,-5.90808615117926));
#281608=CARTESIAN_POINT('Ctrl Pts',(6.21212940551022,12.2562463506078,-8.55026260137164));
#281609=CARTESIAN_POINT('Ctrl Pts',(3.1060647027551,12.4062463506072,-9.55948420107058));
#281610=CARTESIAN_POINT('Ctrl Pts',(-2.03559510845017E-14,12.5562463506066,
-10.5687058007695));
#281611=CARTESIAN_POINT('Ctrl Pts',(-3.10606470275514,12.706246350606,-9.55948420107058));
#281612=CARTESIAN_POINT('Ctrl Pts',(-6.21212940551026,12.8562463506054,
-8.55026260137164));
#281613=CARTESIAN_POINT('Ctrl Pts',(-8.13178296306927,13.0062463506048,
-5.90808615117925));
#281614=CARTESIAN_POINT('Ctrl Pts',(-10.0514365206283,13.1562463506042,
-3.26590970098687));
#281615=CARTESIAN_POINT('Ctrl Pts',(-10.0514365206283,13.3062463506036,
2.46189191236404E-15));
#281616=CARTESIAN_POINT('Ctrl Pts',(-10.0514365206283,13.456246350603,3.26590970098687));
#281617=CARTESIAN_POINT('Ctrl Pts',(-8.13178296306927,13.6062463506024,
5.90808615117926));
#281618=CARTESIAN_POINT('Ctrl Pts',(-6.21212940551026,13.7562463506018,
8.55026260137164));
#281619=CARTESIAN_POINT('Ctrl Pts',(-3.10606470275514,13.9062463506012,
9.55948420107058));
#281620=CARTESIAN_POINT('Ctrl Pts',(-1.86312193743241E-14,14.0562463506006,
10.5687058007695));
#281621=CARTESIAN_POINT('Ctrl Pts',(3.1060647027551,14.2062463506,9.55948420107058));
#281622=CARTESIAN_POINT('Ctrl Pts',(6.21212940551022,14.3562463505994,8.55026260137164));
#281623=CARTESIAN_POINT('Ctrl Pts',(8.13178296306923,14.5062463505988,5.90808615117925));
#281624=CARTESIAN_POINT('Ctrl Pts',(10.0514365206282,14.6562463505982,3.26590970098687));
#281625=CARTESIAN_POINT('Ctrl Pts',(10.0514365206282,14.8062463505976,-1.23094595618202E-15));
#281626=CARTESIAN_POINT('Ctrl Pts',(10.0514365206282,14.956246350597,-3.26590970098687));
#281627=CARTESIAN_POINT('Ctrl Pts',(8.13178296306922,15.1062463505964,-5.90808615117926));
#281628=CARTESIAN_POINT('Ctrl Pts',(6.21212940551022,15.2562463505958,-8.55026260137164));
#281629=CARTESIAN_POINT('Ctrl Pts',(3.1060647027551,15.4062463505952,-9.55948420107058));
#281630=CARTESIAN_POINT('Ctrl Pts',(-2.20836603561635E-14,15.5562463505946,
-10.5687058007695));
#281631=CARTESIAN_POINT('Ctrl Pts',(-3.10606470275514,15.706246350594,-9.55948420107058));
#281632=CARTESIAN_POINT('Ctrl Pts',(-6.21212940551026,15.8562463505934,
-8.55026260137164));
#281633=CARTESIAN_POINT('Ctrl Pts',(-8.13178296306927,16.0062463505928,
-5.90808615117925));
#281634=CARTESIAN_POINT('Ctrl Pts',(-10.0514365206283,16.1562463505922,
-3.26590970098687));
#281635=CARTESIAN_POINT('Ctrl Pts',(-10.0514365206283,16.3062463505916,
2.46189191236404E-15));
#281636=CARTESIAN_POINT('Ctrl Pts',(-10.0514365206283,16.456246350591,3.26590970098687));
#281637=CARTESIAN_POINT('Ctrl Pts',(-8.13178296306927,16.6062463505904,
5.90808615117926));
#281638=CARTESIAN_POINT('Ctrl Pts',(-6.21212940551026,16.7562463505898,
8.55026260137164));
#281639=CARTESIAN_POINT('Ctrl Pts',(-3.10606470275514,16.9062463505892,
9.55948420107058));
#281640=CARTESIAN_POINT('Ctrl Pts',(-2.03589286459859E-14,17.0562463505886,
10.5687058007695));
#281641=CARTESIAN_POINT('Ctrl Pts',(3.1060647027551,17.206246350588,9.55948420107058));
#281642=CARTESIAN_POINT('Ctrl Pts',(6.21212940551022,17.3562463505874,8.55026260137164));
#281643=CARTESIAN_POINT('Ctrl Pts',(8.13178296306922,17.5062463505868,5.90808615117925));
#281644=CARTESIAN_POINT('Ctrl Pts',(10.0514365206282,17.6562463505862,3.26590970098687));
#281645=CARTESIAN_POINT('Ctrl Pts',(10.0514365206282,17.8062463505856,-1.23094595618202E-15));
#281646=CARTESIAN_POINT('Ctrl Pts',(10.0514365206282,17.956246350585,-3.26590970098687));
#281647=CARTESIAN_POINT('Ctrl Pts',(8.13178296306922,18.1062463505844,-5.90808615117926));
#281648=CARTESIAN_POINT('Ctrl Pts',(6.21212940551022,18.2562463505838,-8.55026260137164));
#281649=CARTESIAN_POINT('Ctrl Pts',(3.1060647027551,18.4062463505832,-9.55948420107058));
#281650=CARTESIAN_POINT('Ctrl Pts',(-2.38113696278254E-14,18.5562463505826,
-10.5687058007695));
#281651=CARTESIAN_POINT('Ctrl Pts',(-3.10606470275514,18.706246350582,-9.55948420107058));
#281652=CARTESIAN_POINT('Ctrl Pts',(-6.21212940551027,18.8562463505814,
-8.55026260137164));
#281653=CARTESIAN_POINT('Ctrl Pts',(-8.13178296306927,19.0062463505808,
-5.90808615117925));
#281654=CARTESIAN_POINT('Ctrl Pts',(-10.0514365206283,19.1562463505802,
-3.26590970098687));
#281655=CARTESIAN_POINT('Ctrl Pts',(-10.0514365206283,19.3062463505796,
2.46189191236404E-15));
#281656=CARTESIAN_POINT('Ctrl Pts',(-10.0514365206283,19.456246350579,3.26590970098687));
#281657=CARTESIAN_POINT('Ctrl Pts',(-8.13178296306927,19.6062463505784,
5.90808615117926));
#281658=CARTESIAN_POINT('Ctrl Pts',(-6.21212940551026,19.7562463505778,
8.55026260137164));
#281659=CARTESIAN_POINT('Ctrl Pts',(-3.10606470275514,19.9062463505772,
9.55948420107058));
#281660=CARTESIAN_POINT('Ctrl Pts',(-2.20866379176478E-14,20.0562463505766,
10.5687058007695));
#281661=CARTESIAN_POINT('Ctrl Pts',(3.1060647027551,20.206246350576,9.55948420107058));
#281662=CARTESIAN_POINT('Ctrl Pts',(6.21212940551022,20.3562463505754,8.55026260137164));
#281663=CARTESIAN_POINT('Ctrl Pts',(8.13178296306922,20.5062463505748,5.90808615117925));
#281664=CARTESIAN_POINT('Ctrl Pts',(10.0514365206282,20.6562463505742,3.26590970098687));
#281665=CARTESIAN_POINT('Ctrl Pts',(10.0514365206282,20.8062463505736,-1.23094595618202E-15));
#281666=CARTESIAN_POINT('Ctrl Pts',(10.0514365206282,20.956246350573,-3.26590970098687));
#281667=CARTESIAN_POINT('Ctrl Pts',(8.13178296306922,21.1062463505724,-5.90808615117926));
#281668=CARTESIAN_POINT('Ctrl Pts',(6.21212940551022,21.2562463505718,-8.55026260137164));
#281669=CARTESIAN_POINT('Ctrl Pts',(3.1060647027551,21.4062463505712,-9.55948420107058));
#281670=CARTESIAN_POINT('Ctrl Pts',(-2.55390788994872E-14,21.5562463505706,
-10.5687058007695));
#281671=CARTESIAN_POINT('Ctrl Pts',(-3.10606470275515,21.70624635057,-9.55948420107058));
#281672=CARTESIAN_POINT('Ctrl Pts',(-6.21212940551027,21.8562463505694,
-8.55026260137164));
#281673=CARTESIAN_POINT('Ctrl Pts',(-8.13178296306927,22.0062463505688,
-5.90808615117925));
#281674=CARTESIAN_POINT('Ctrl Pts',(-10.0514365206283,22.1562463505682,
-3.26590970098687));
#281675=CARTESIAN_POINT('Ctrl Pts',(-10.0514365206283,22.3062463505676,
2.46189191236404E-15));
#281676=CARTESIAN_POINT('Ctrl Pts',(-10.0514365206283,22.456246350567,3.26590970098687));
#281677=CARTESIAN_POINT('Ctrl Pts',(-8.13178296306927,22.6062463505664,
5.90808615117926));
#281678=CARTESIAN_POINT('Ctrl Pts',(-6.21212940551027,22.7562463505658,
8.55026260137164));
#281679=CARTESIAN_POINT('Ctrl Pts',(-3.10606470275514,22.9062463505652,
9.55948420107058));
#281680=CARTESIAN_POINT('Ctrl Pts',(-2.38143471893096E-14,23.0562463505646,
10.5687058007695));
#281681=CARTESIAN_POINT('Ctrl Pts',(3.1060647027551,23.206246350564,9.55948420107058));
#281682=CARTESIAN_POINT('Ctrl Pts',(6.21212940551022,23.3562463505634,8.55026260137164));
#281683=CARTESIAN_POINT('Ctrl Pts',(8.13178296306922,23.5062463505628,5.90808615117925));
#281684=CARTESIAN_POINT('Ctrl Pts',(10.0514365206282,23.6562463505622,3.26590970098687));
#281685=CARTESIAN_POINT('Ctrl Pts',(10.0514365206282,23.8062463505616,-1.23094595618202E-15));
#281686=CARTESIAN_POINT('Ctrl Pts',(10.0514365206282,23.956246350561,-3.26590970098687));
#281687=CARTESIAN_POINT('Ctrl Pts',(8.13178296306922,24.1062463505604,-5.90808615117926));
#281688=CARTESIAN_POINT('Ctrl Pts',(6.21212940551021,24.2562463505598,-8.55026260137164));
#281689=CARTESIAN_POINT('Ctrl Pts',(3.10606470275509,24.4062463505592,-9.55948420107058));
#281690=CARTESIAN_POINT('Ctrl Pts',(-2.7266788171149E-14,24.5562463505586,
-10.5687058007695));
#281691=CARTESIAN_POINT('Ctrl Pts',(-3.10606470275515,24.706246350558,-9.55948420107058));
#281692=CARTESIAN_POINT('Ctrl Pts',(-6.21212940551027,24.8562463505574,
-8.55026260137164));
#281693=CARTESIAN_POINT('Ctrl Pts',(-8.13178296306927,25.0062463505568,
-5.90808615117925));
#281694=CARTESIAN_POINT('Ctrl Pts',(-10.0514365206283,25.1562463505562,
-3.26590970098687));
#281695=CARTESIAN_POINT('Ctrl Pts',(-10.0514365206283,25.3062463505556,
2.46189191236404E-15));
#281696=CARTESIAN_POINT('Ctrl Pts',(-10.0514365206283,25.456246350555,3.26590970098687));
#281697=CARTESIAN_POINT('Ctrl Pts',(-8.13178296306927,25.6062463505544,
5.90808615117926));
#281698=CARTESIAN_POINT('Ctrl Pts',(-6.21212940551027,25.7562463505538,
8.55026260137164));
#281699=CARTESIAN_POINT('Ctrl Pts',(-3.10606470275515,25.9062463505532,
9.55948420107058));
#281700=CARTESIAN_POINT('Ctrl Pts',(-2.55420564609715E-14,26.0562463505526,
10.5687058007695));
#281701=CARTESIAN_POINT('Ctrl Pts',(3.10606470275509,26.206246350552,9.55948420107058));
#281702=CARTESIAN_POINT('Ctrl Pts',(6.21212940551022,26.3562463505514,8.55026260137164));
#281703=CARTESIAN_POINT('Ctrl Pts',(8.13178296306922,26.5062463505508,5.90808615117925));
#281704=CARTESIAN_POINT('Ctrl Pts',(10.0514365206282,26.6562463505502,3.26590970098687));
#281705=CARTESIAN_POINT('Ctrl Pts',(10.0514365206282,26.8062463505496,-1.23094595618202E-15));
#281706=CARTESIAN_POINT('Ctrl Pts',(10.0514365206282,26.956246350549,-3.26590970098687));
#281707=CARTESIAN_POINT('Ctrl Pts',(8.13178296306922,27.1062463505484,-5.90808615117926));
#281708=CARTESIAN_POINT('Ctrl Pts',(6.21212940551021,27.2562463505478,-8.55026260137164));
#281709=CARTESIAN_POINT('Ctrl Pts',(3.10606470275509,27.4062463505472,-9.55948420107058));
#281710=CARTESIAN_POINT('Ctrl Pts',(-2.89944974428109E-14,27.5562463505466,
-10.5687058007695));
#281711=CARTESIAN_POINT('Ctrl Pts',(-3.10606470275515,27.706246350546,-9.55948420107058));
#281712=CARTESIAN_POINT('Ctrl Pts',(-6.21212940551027,27.8562463505454,
-8.55026260137164));
#281713=CARTESIAN_POINT('Ctrl Pts',(-8.13178296306928,28.0062463505448,
-5.90808615117925));
#281714=CARTESIAN_POINT('Ctrl Pts',(-10.0514365206283,28.1562463505442,
-3.26590970098687));
#281715=CARTESIAN_POINT('Ctrl Pts',(-10.0514365206283,28.3062463505436,
2.46189191236404E-15));
#281716=CARTESIAN_POINT('Ctrl Pts',(-10.0514365206283,28.456246350543,3.26590970098687));
#281717=CARTESIAN_POINT('Ctrl Pts',(-8.13178296306928,28.6062463505424,
5.90808615117926));
#281718=CARTESIAN_POINT('Ctrl Pts',(-6.21212940551027,28.7562463505418,
8.55026260137164));
#281719=CARTESIAN_POINT('Ctrl Pts',(-3.10606470275515,28.9062463505412,
9.55948420107058));
#281720=CARTESIAN_POINT('Ctrl Pts',(-2.72697657326333E-14,29.0562463505406,
10.5687058007695));
#281721=CARTESIAN_POINT('Ctrl Pts',(3.10606470275509,29.20624635054,9.55948420107058));
#281722=CARTESIAN_POINT('Ctrl Pts',(6.21212940551021,29.3562463505394,8.55026260137164));
#281723=CARTESIAN_POINT('Ctrl Pts',(8.13178296306922,29.5062463505388,5.90808615117925));
#281724=CARTESIAN_POINT('Ctrl Pts',(10.0514365206282,29.6562463505382,3.26590970098687));
#281725=CARTESIAN_POINT('Ctrl Pts',(10.0514365206282,29.8062463505376,-1.23094595618202E-15));
#281726=CARTESIAN_POINT('Ctrl Pts',(10.0514365206282,29.956246350537,-3.26590970098687));
#281727=CARTESIAN_POINT('Ctrl Pts',(8.13178296306921,30.1062463505364,-5.90808615117926));
#281728=CARTESIAN_POINT('Ctrl Pts',(6.21212940551021,30.2562463505358,-8.55026260137164));
#281729=CARTESIAN_POINT('Ctrl Pts',(3.10606470275509,30.4062463505352,-9.55948420107058));
#281730=CARTESIAN_POINT('Ctrl Pts',(-3.07222067144727E-14,30.5562463505346,
-10.5687058007695));
#281731=CARTESIAN_POINT('Ctrl Pts',(-3.10606470275515,30.706246350534,-9.55948420107058));
#281732=CARTESIAN_POINT('Ctrl Pts',(-6.21212940551027,30.8562463505334,
-8.55026260137164));
#281733=CARTESIAN_POINT('Ctrl Pts',(-8.13178296306928,31.0062463505328,
-5.90808615117925));
#281734=CARTESIAN_POINT('Ctrl Pts',(-10.0514365206283,31.1562463505322,
-3.26590970098687));
#281735=CARTESIAN_POINT('Ctrl Pts',(-10.0514365206283,31.3062463505316,
2.46189191236404E-15));
#281736=CARTESIAN_POINT('Ctrl Pts',(-10.0514365206283,31.456246350531,3.26590970098687));
#281737=CARTESIAN_POINT('Ctrl Pts',(-8.13178296306928,31.6062463505304,
5.90808615117926));
#281738=CARTESIAN_POINT('Ctrl Pts',(-6.21212940551027,31.7562463505298,
8.55026260137164));
#281739=CARTESIAN_POINT('Ctrl Pts',(-3.10606470275515,31.9062463505292,
9.55948420107058));
#281740=CARTESIAN_POINT('Ctrl Pts',(-2.89974750042951E-14,32.0562463505286,
10.5687058007695));
#281741=CARTESIAN_POINT('Ctrl Pts',(3.10606470275509,32.206246350528,9.55948420107058));
#281742=CARTESIAN_POINT('Ctrl Pts',(6.21212940551021,32.3562463505274,8.55026260137164));
#281743=CARTESIAN_POINT('Ctrl Pts',(8.13178296306921,32.5062463505268,5.90808615117925));
#281744=CARTESIAN_POINT('Ctrl Pts',(10.0514365206282,32.6562463505262,3.26590970098687));
#281745=CARTESIAN_POINT('Ctrl Pts',(10.0514365206282,32.8062463505256,-1.23094595618202E-15));
#281746=CARTESIAN_POINT('Ctrl Pts',(10.0514365206282,32.956246350525,-3.26590970098687));
#281747=CARTESIAN_POINT('Ctrl Pts',(8.13178296306921,33.1062463505244,-5.90808615117926));
#281748=CARTESIAN_POINT('Ctrl Pts',(6.21212940551021,33.2562463505238,-8.55026260137164));
#281749=CARTESIAN_POINT('Ctrl Pts',(3.10606470275509,33.4062463505232,-9.55948420107058));
#281750=CARTESIAN_POINT('Ctrl Pts',(-3.24499159861345E-14,33.5562463505226,
-10.5687058007695));
#281751=CARTESIAN_POINT('Ctrl Pts',(-3.10606470275515,33.706246350522,-9.55948420107058));
#281752=CARTESIAN_POINT('Ctrl Pts',(-6.21212940551027,33.8562463505214,
-8.55026260137164));
#281753=CARTESIAN_POINT('Ctrl Pts',(-8.13178296306928,34.0062463505208,
-5.90808615117925));
#281754=CARTESIAN_POINT('Ctrl Pts',(-10.0514365206283,34.1562463505202,
-3.26590970098687));
#281755=CARTESIAN_POINT('Ctrl Pts',(-10.0514365206283,34.3062463505196,
2.46189191236404E-15));
#281756=CARTESIAN_POINT('Ctrl Pts',(-10.0514365206283,34.456246350519,3.26590970098687));
#281757=CARTESIAN_POINT('Ctrl Pts',(-8.13178296306928,34.6062463505184,
5.90808615117926));
#281758=CARTESIAN_POINT('Ctrl Pts',(-6.21212940551027,34.7562463505178,
8.55026260137164));
#281759=CARTESIAN_POINT('Ctrl Pts',(-3.10606470275515,34.9062463505172,
9.55948420107058));
#281760=CARTESIAN_POINT('Ctrl Pts',(-3.0725184275957E-14,35.0562463505166,
10.5687058007695));
#281761=CARTESIAN_POINT('Ctrl Pts',(3.10606470275509,35.206246350516,9.55948420107058));
#281762=CARTESIAN_POINT('Ctrl Pts',(6.21212940551021,35.3562463505154,8.55026260137164));
#281763=CARTESIAN_POINT('Ctrl Pts',(8.13178296306921,35.5062463505148,5.90808615117925));
#281764=CARTESIAN_POINT('Ctrl Pts',(10.0514365206282,35.6562463505142,3.26590970098687));
#281765=CARTESIAN_POINT('Ctrl Pts',(10.0514365206282,35.8062463505136,-1.23094595618202E-15));
#281766=CARTESIAN_POINT('Ctrl Pts',(10.0514365206282,35.956246350513,-3.26590970098687));
#281767=CARTESIAN_POINT('Ctrl Pts',(8.13178296306921,36.1062463505124,-5.90808615117926));
#281768=CARTESIAN_POINT('Ctrl Pts',(6.21212940551021,36.2562463505118,-8.55026260137164));
#281769=CARTESIAN_POINT('Ctrl Pts',(3.10606470275509,36.4062463505112,-9.55948420107058));
#281770=CARTESIAN_POINT('Ctrl Pts',(-3.41776252577964E-14,36.5562463505106,
-10.5687058007695));
#281771=CARTESIAN_POINT('Ctrl Pts',(-3.10606470275516,36.70624635051,-9.55948420107058));
#281772=CARTESIAN_POINT('Ctrl Pts',(-6.21212940551028,36.8562463505094,
-8.55026260137164));
#281773=CARTESIAN_POINT('Ctrl Pts',(-8.13178296306928,37.0062463505088,
-5.90808615117925));
#281774=CARTESIAN_POINT('Ctrl Pts',(-10.0514365206283,37.1562463505082,
-3.26590970098687));
#281775=CARTESIAN_POINT('Ctrl Pts',(-10.0514365206283,37.3062463505076,
2.46189191236404E-15));
#281776=CARTESIAN_POINT('Ctrl Pts',(-10.0514365206283,37.456246350507,3.26590970098687));
#281777=CARTESIAN_POINT('Ctrl Pts',(-8.13178296306928,37.6062463505064,
5.90808615117926));
#281778=CARTESIAN_POINT('Ctrl Pts',(-6.21212940551027,37.7562463505058,
8.55026260137164));
#281779=CARTESIAN_POINT('Ctrl Pts',(-3.10606470275515,37.9062463505052,
9.55948420107058));
#281780=CARTESIAN_POINT('Ctrl Pts',(-3.24528935476188E-14,38.0562463505046,
10.5687058007695));
#281781=CARTESIAN_POINT('Ctrl Pts',(3.10606470275509,38.206246350504,9.55948420107058));
#281782=CARTESIAN_POINT('Ctrl Pts',(6.21212940551021,38.3562463505034,8.55026260137164));
#281783=CARTESIAN_POINT('Ctrl Pts',(8.13178296306921,38.5062463505028,5.90808615117925));
#281784=CARTESIAN_POINT('Ctrl Pts',(10.0514365206282,38.6562463505022,3.26590970098687));
#281785=CARTESIAN_POINT('Ctrl Pts',(10.0514365206282,38.8062463505016,-1.23094595618202E-15));
#281786=CARTESIAN_POINT('Ctrl Pts',(10.0514365206282,38.956246350501,-3.26590970098687));
#281787=CARTESIAN_POINT('Ctrl Pts',(8.13178296306921,39.1062463505004,-5.90808615117926));
#281788=CARTESIAN_POINT('Ctrl Pts',(6.2121294055102,39.2562463504998,-8.55026260137164));
#281789=CARTESIAN_POINT('Ctrl Pts',(3.10606470275508,39.4062463504992,-9.55948420107058));
#281790=CARTESIAN_POINT('Ctrl Pts',(-3.59053345294582E-14,39.5562463504986,
-10.5687058007695));
#281791=CARTESIAN_POINT('Ctrl Pts',(-3.10606470275516,39.706246350498,-9.55948420107058));
#281792=CARTESIAN_POINT('Ctrl Pts',(-6.21212940551028,39.8562463504974,
-8.55026260137164));
#281793=CARTESIAN_POINT('Ctrl Pts',(-8.13178296306928,40.0062463504968,
-5.90808615117925));
#281794=CARTESIAN_POINT('Ctrl Pts',(-10.0514365206283,40.1562463504962,
-3.26590970098687));
#281795=CARTESIAN_POINT('Ctrl Pts',(-10.0514365206283,40.3062463504956,
2.46189191236404E-15));
#281796=CARTESIAN_POINT('Ctrl Pts',(-10.0514365206283,40.456246350495,3.26590970098687));
#281797=CARTESIAN_POINT('Ctrl Pts',(-8.13178296306928,40.6062463504944,
5.90808615117926));
#281798=CARTESIAN_POINT('Ctrl Pts',(-6.21212940551028,40.7562463504938,
8.55026260137164));
#281799=CARTESIAN_POINT('Ctrl Pts',(-3.10606470275516,40.9062463504932,
9.55948420107058));
#281800=CARTESIAN_POINT('Ctrl Pts',(-3.41806028192807E-14,41.0562463504926,
10.5687058007695));
#281801=CARTESIAN_POINT('Ctrl Pts',(3.10606470275509,41.206246350492,9.55948420107058));
#281802=CARTESIAN_POINT('Ctrl Pts',(6.21212940551021,41.3562463504914,8.55026260137164));
#281803=CARTESIAN_POINT('Ctrl Pts',(8.13178296306921,41.5062463504908,5.90808615117925));
#281804=CARTESIAN_POINT('Ctrl Pts',(10.0514365206282,41.6562463504902,3.26590970098687));
#281805=CARTESIAN_POINT('Ctrl Pts',(10.0514365206282,41.8062463504896,-1.23094595618202E-15));
#281806=CARTESIAN_POINT('Ctrl Pts',(10.0514365206282,41.956246350489,-3.26590970098687));
#281807=CARTESIAN_POINT('Ctrl Pts',(8.13178296306921,42.1062463504884,-5.90808615117926));
#281808=CARTESIAN_POINT('Ctrl Pts',(6.2121294055102,42.2562463504878,-8.55026260137164));
#281809=CARTESIAN_POINT('Ctrl Pts',(3.10606470275508,42.4062463504872,-9.55948420107058));
#281810=CARTESIAN_POINT('Ctrl Pts',(-3.76330438011201E-14,42.5562463504866,
-10.5687058007695));
#281811=CARTESIAN_POINT('Ctrl Pts',(-3.10606470275516,42.706246350486,-9.55948420107058));
#281812=CARTESIAN_POINT('Ctrl Pts',(-6.21212940551028,42.8562463504854,
-8.55026260137164));
#281813=CARTESIAN_POINT('Ctrl Pts',(-8.13178296306928,43.0062463504848,
-5.90808615117925));
#281814=CARTESIAN_POINT('Ctrl Pts',(-10.0514365206283,43.1562463504842,
-3.26590970098687));
#281815=CARTESIAN_POINT('Ctrl Pts',(-10.0514365206283,43.3062463504836,
2.46189191236404E-15));
#281816=CARTESIAN_POINT('Ctrl Pts',(-10.0514365206283,43.456246350483,3.26590970098687));
#281817=CARTESIAN_POINT('Ctrl Pts',(-8.13178296306928,43.6062463504824,
5.90808615117926));
#281818=CARTESIAN_POINT('Ctrl Pts',(-6.21212940551028,43.7562463504818,
8.55026260137164));
#281819=CARTESIAN_POINT('Ctrl Pts',(-3.10606470275516,43.9062463504812,
9.55948420107058));
#281820=CARTESIAN_POINT('Ctrl Pts',(-3.59083120909425E-14,44.0562463504806,
10.5687058007695));
#281821=CARTESIAN_POINT('Ctrl Pts',(3.10606470275508,44.20624635048,9.55948420107058));
#281822=CARTESIAN_POINT('Ctrl Pts',(6.2121294055102,44.3562463504794,8.55026260137164));
#281823=CARTESIAN_POINT('Ctrl Pts',(8.13178296306921,44.5062463504788,5.90808615117925));
#281824=CARTESIAN_POINT('Ctrl Pts',(10.0514365206282,44.6562463504782,3.26590970098687));
#281825=CARTESIAN_POINT('Ctrl Pts',(10.0514365206282,44.8062463504776,-1.23094595618202E-15));
#281826=CARTESIAN_POINT('Ctrl Pts',(10.0514365206282,44.956246350477,-3.26590970098687));
#281827=CARTESIAN_POINT('Ctrl Pts',(8.13178296306921,45.1062463504764,-5.90808615117926));
#281828=CARTESIAN_POINT('Ctrl Pts',(6.2121294055102,45.2562463504758,-8.55026260137164));
#281829=CARTESIAN_POINT('Ctrl Pts',(3.10606470275508,45.4062463504752,-9.55948420107058));
#281830=CARTESIAN_POINT('Ctrl Pts',(-3.93607530727819E-14,45.5562463504746,
-10.5687058007695));
#281831=CARTESIAN_POINT('Ctrl Pts',(-3.10606470275516,45.706246350474,-9.55948420107058));
#281832=CARTESIAN_POINT('Ctrl Pts',(-6.21212940551028,45.8562463504734,
-8.55026260137164));
#281833=CARTESIAN_POINT('Ctrl Pts',(-8.13178296306928,46.0062463504728,
-5.90808615117925));
#281834=CARTESIAN_POINT('Ctrl Pts',(-10.0514365206283,46.1562463504722,
-3.26590970098687));
#281835=CARTESIAN_POINT('Ctrl Pts',(-10.0514365206283,46.3062463504716,
2.46189191236404E-15));
#281836=CARTESIAN_POINT('Ctrl Pts',(-10.0514365206283,46.456246350471,3.26590970098687));
#281837=CARTESIAN_POINT('Ctrl Pts',(-8.13178296306928,46.6062463504704,
5.90808615117926));
#281838=CARTESIAN_POINT('Ctrl Pts',(-6.21212940551028,46.7562463504698,
8.55026260137164));
#281839=CARTESIAN_POINT('Ctrl Pts',(-3.10606470275516,46.9062463504692,
9.55948420107058));
#281840=CARTESIAN_POINT('Ctrl Pts',(-3.76360213626043E-14,47.0562463504686,
10.5687058007695));
#281841=CARTESIAN_POINT('Ctrl Pts',(3.10606470275508,47.206246350468,9.55948420107058));
#281842=CARTESIAN_POINT('Ctrl Pts',(6.2121294055102,47.3562463504674,8.55026260137164));
#281843=CARTESIAN_POINT('Ctrl Pts',(8.13178296306921,47.5062463504668,5.90808615117925));
#281844=CARTESIAN_POINT('Ctrl Pts',(10.0514365206282,47.6562463504662,3.26590970098687));
#281845=CARTESIAN_POINT('Ctrl Pts',(10.0514365206282,47.8062463504656,-1.23094595618202E-15));
#281846=CARTESIAN_POINT('Ctrl Pts',(10.0514365206282,47.956246350465,-3.26590970098687));
#281847=CARTESIAN_POINT('Ctrl Pts',(8.1317829630692,48.1062463504644,-5.90808615117926));
#281848=CARTESIAN_POINT('Ctrl Pts',(6.2121294055102,48.2562463504638,-8.55026260137164));
#281849=CARTESIAN_POINT('Ctrl Pts',(3.10606470275508,48.4062463504632,-9.55948420107058));
#281850=CARTESIAN_POINT('Ctrl Pts',(-4.10884623444438E-14,48.5562463504626,
-10.5687058007695));
#281851=CARTESIAN_POINT('Ctrl Pts',(-3.10606470275516,48.706246350462,-9.55948420107058));
#281852=CARTESIAN_POINT('Ctrl Pts',(-6.21212940551028,48.8562463504614,
-8.55026260137164));
#281853=CARTESIAN_POINT('Ctrl Pts',(-8.13178296306929,49.0062463504608,
-5.90808615117925));
#281854=CARTESIAN_POINT('Ctrl Pts',(-10.0514365206283,49.1562463504602,
-3.26590970098687));
#281855=CARTESIAN_POINT('Ctrl Pts',(-10.0514365206283,49.3062463504596,
2.46189191236404E-15));
#281856=CARTESIAN_POINT('Ctrl Pts',(-10.0514365206283,49.456246350459,3.26590970098687));
#281857=CARTESIAN_POINT('Ctrl Pts',(-8.13178296306929,49.6062463504584,
5.90808615117926));
#281858=CARTESIAN_POINT('Ctrl Pts',(-6.21212940551028,49.7562463504578,
8.55026260137164));
#281859=CARTESIAN_POINT('Ctrl Pts',(-3.10606470275516,49.9062463504572,
9.55948420107058));
#281860=CARTESIAN_POINT('Ctrl Pts',(-3.93637306342662E-14,50.0562463504566,
10.5687058007695));
#281861=CARTESIAN_POINT('Ctrl Pts',(3.10606470275508,50.206246350456,9.55948420107058));
#281862=CARTESIAN_POINT('Ctrl Pts',(6.2121294055102,50.3562463504554,8.55026260137164));
#281863=CARTESIAN_POINT('Ctrl Pts',(8.1317829630692,50.5062463504548,5.90808615117925));
#281864=CARTESIAN_POINT('Ctrl Pts',(10.0514365206282,50.6562463504542,3.26590970098687));
#281865=CARTESIAN_POINT('Ctrl Pts',(10.0514365206282,50.8062463504536,-1.23094595618202E-15));
#281866=CARTESIAN_POINT('Ctrl Pts',(10.0514365206282,50.956246350453,-3.26590970098687));
#281867=CARTESIAN_POINT('Ctrl Pts',(8.1317829630692,51.1062463504524,-5.90808615117926));
#281868=CARTESIAN_POINT('Ctrl Pts',(6.2121294055102,51.2562463504518,-8.55026260137164));
#281869=CARTESIAN_POINT('Ctrl Pts',(3.10606470275508,51.4062463504512,-9.55948420107058));
#281870=CARTESIAN_POINT('Ctrl Pts',(-4.28161716161056E-14,51.5562463504506,
-10.5687058007695));
#281871=CARTESIAN_POINT('Ctrl Pts',(-3.10606470275516,51.70624635045,-9.55948420107058));
#281872=CARTESIAN_POINT('Ctrl Pts',(-6.21212940551029,51.8562463504494,
-8.55026260137164));
#281873=CARTESIAN_POINT('Ctrl Pts',(-8.13178296306929,52.0062463504488,
-5.90808615117925));
#281874=CARTESIAN_POINT('Ctrl Pts',(-10.0514365206283,52.1562463504482,
-3.26590970098687));
#281875=CARTESIAN_POINT('Ctrl Pts',(-10.0514365206283,52.3062463504476,
2.46189191236404E-15));
#281876=CARTESIAN_POINT('Ctrl Pts',(-10.0514365206283,52.456246350447,3.26590970098687));
#281877=CARTESIAN_POINT('Ctrl Pts',(-8.13178296306929,52.6062463504464,
5.90808615117926));
#281878=CARTESIAN_POINT('Ctrl Pts',(-6.21212940551028,52.7562463504458,
8.55026260137164));
#281879=CARTESIAN_POINT('Ctrl Pts',(-3.10606470275516,52.9062463504452,
9.55948420107058));
#281880=CARTESIAN_POINT('Ctrl Pts',(-4.1091439905928E-14,53.0562463504446,
10.5687058007695));
#281881=CARTESIAN_POINT('Ctrl Pts',(3.10606470275508,53.206246350444,9.55948420107058));
#281882=CARTESIAN_POINT('Ctrl Pts',(6.2121294055102,53.3562463504434,8.55026260137164));
#281883=CARTESIAN_POINT('Ctrl Pts',(8.1317829630692,53.5062463504428,5.90808615117925));
#281884=CARTESIAN_POINT('Ctrl Pts',(10.0514365206282,53.6562463504422,3.26590970098687));
#281885=CARTESIAN_POINT('Ctrl Pts',(10.0514365206282,53.8062463504416,-1.23094595618202E-15));
#281886=CARTESIAN_POINT('Ctrl Pts',(10.0514365206282,53.956246350441,-3.26590970098687));
#281887=CARTESIAN_POINT('Ctrl Pts',(8.1317829630692,54.1062463504404,-5.90808615117926));
#281888=CARTESIAN_POINT('Ctrl Pts',(6.2121294055102,54.2562463504398,-8.55026260137164));
#281889=CARTESIAN_POINT('Ctrl Pts',(3.10606470275508,54.4062463504392,-9.55948420107058));
#281890=CARTESIAN_POINT('Ctrl Pts',(-4.45438808877674E-14,54.5562463504386,
-10.5687058007695));
#281891=CARTESIAN_POINT('Ctrl Pts',(-3.10606470275517,54.706246350438,-9.55948420107058));
#281892=CARTESIAN_POINT('Ctrl Pts',(-6.21212940551029,54.8562463504374,
-8.55026260137164));
#281893=CARTESIAN_POINT('Ctrl Pts',(-8.13178296306929,55.0062463504368,
-5.90808615117925));
#281894=CARTESIAN_POINT('Ctrl Pts',(-10.0514365206283,55.1562463504362,
-3.26590970098687));
#281895=CARTESIAN_POINT('Ctrl Pts',(-10.0514365206283,55.3062463504356,
2.46189191236404E-15));
#281896=CARTESIAN_POINT('Ctrl Pts',(-10.0514365206283,55.456246350435,3.26590970098687));
#281897=CARTESIAN_POINT('Ctrl Pts',(-8.13178296306929,55.6062463504344,
5.90808615117926));
#281898=CARTESIAN_POINT('Ctrl Pts',(-6.21212940551028,55.7562463504338,
8.55026260137164));
#281899=CARTESIAN_POINT('Ctrl Pts',(-3.10606470275516,55.9062463504332,
9.55948420107058));
#281900=CARTESIAN_POINT('Ctrl Pts',(-4.28191491775899E-14,56.0562463504326,
10.5687058007695));
#281901=CARTESIAN_POINT('Ctrl Pts',(3.10606470275508,56.206246350432,9.55948420107058));
#281902=CARTESIAN_POINT('Ctrl Pts',(6.2121294055102,56.3562463504314,8.55026260137164));
#281903=CARTESIAN_POINT('Ctrl Pts',(8.1317829630692,56.5062463504308,5.90808615117925));
#281904=CARTESIAN_POINT('Ctrl Pts',(10.0514365206282,56.6562463504302,3.26590970098687));
#281905=CARTESIAN_POINT('Ctrl Pts',(10.0514365206282,56.8062463504296,-1.23094595618202E-15));
#281906=CARTESIAN_POINT('Ctrl Pts',(10.0514365206282,56.956246350429,-3.26590970098687));
#281907=CARTESIAN_POINT('Ctrl Pts',(8.1317829630692,57.1062463504284,-5.90808615117926));
#281908=CARTESIAN_POINT('Ctrl Pts',(6.2121294055102,57.2562463504278,-8.55026260137164));
#281909=CARTESIAN_POINT('Ctrl Pts',(3.10606470275507,57.4062463504272,-9.55948420107058));
#281910=CARTESIAN_POINT('Ctrl Pts',(-4.62715901594293E-14,57.5562463504266,
-10.5687058007695));
#281911=CARTESIAN_POINT('Ctrl Pts',(-3.10606470275517,57.706246350426,-9.55948420107058));
#281912=CARTESIAN_POINT('Ctrl Pts',(-6.21212940551029,57.8562463504254,
-8.55026260137164));
#281913=CARTESIAN_POINT('Ctrl Pts',(-8.13178296306929,58.0062463504248,
-5.90808615117925));
#281914=CARTESIAN_POINT('Ctrl Pts',(-10.0514365206283,58.1562463504242,
-3.26590970098687));
#281915=CARTESIAN_POINT('Ctrl Pts',(-10.0514365206283,58.3062463504236,
2.46189191236404E-15));
#281916=CARTESIAN_POINT('Ctrl Pts',(-10.0514365206283,58.456246350423,3.26590970098687));
#281917=CARTESIAN_POINT('Ctrl Pts',(-8.13178296306929,58.6062463504224,
5.90808615117926));
#281918=CARTESIAN_POINT('Ctrl Pts',(-6.21212940551029,58.7562463504218,
8.55026260137164));
#281919=CARTESIAN_POINT('Ctrl Pts',(-3.10606470275517,58.9062463504212,
9.55948420107058));
#281920=CARTESIAN_POINT('Ctrl Pts',(-4.45468584492517E-14,59.0562463504206,
10.5687058007695));
#281921=CARTESIAN_POINT('Ctrl Pts',(3.10606470275508,59.20624635042,9.55948420107058));
#281922=CARTESIAN_POINT('Ctrl Pts',(6.2121294055102,59.3562463504194,8.55026260137164));
#281923=CARTESIAN_POINT('Ctrl Pts',(8.1317829630692,59.5062463504188,5.90808615117925));
#281924=CARTESIAN_POINT('Ctrl Pts',(10.0514365206282,59.6562463504182,3.26590970098687));
#281925=CARTESIAN_POINT('Ctrl Pts',(10.0514365206282,59.8062463504176,-1.23094595618202E-15));
#281926=CARTESIAN_POINT('Ctrl Pts',(10.0514365206282,59.956246350417,-3.26590970098687));
#281927=CARTESIAN_POINT('Ctrl Pts',(8.1317829630692,60.1062463504164,-5.90808615117926));
#281928=CARTESIAN_POINT('Ctrl Pts',(6.2121294055102,60.2562463504158,-8.55026260137164));
#281929=CARTESIAN_POINT('Ctrl Pts',(3.10606470275507,60.4062463504152,-9.55948420107058));
#281930=CARTESIAN_POINT('Ctrl Pts',(-4.79992994310911E-14,60.5562463504146,
-10.5687058007695));
#281931=CARTESIAN_POINT('Ctrl Pts',(-3.10606470275517,60.706246350414,-9.55948420107058));
#281932=CARTESIAN_POINT('Ctrl Pts',(-6.21212940551029,60.8562463504134,
-8.55026260137164));
#281933=CARTESIAN_POINT('Ctrl Pts',(-8.13178296306929,61.0062463504128,
-5.90808615117925));
#281934=CARTESIAN_POINT('Ctrl Pts',(-10.0514365206283,61.1562463504122,
-3.26590970098687));
#281935=CARTESIAN_POINT('Ctrl Pts',(-10.0514365206283,61.3062463504116,
2.46189191236404E-15));
#281936=CARTESIAN_POINT('Ctrl Pts',(-10.0514365206283,61.456246350411,3.26590970098687));
#281937=CARTESIAN_POINT('Ctrl Pts',(-8.13178296306929,61.6062463504104,
5.90808615117926));
#281938=CARTESIAN_POINT('Ctrl Pts',(-6.21212940551029,61.7562463504098,
8.55026260137164));
#281939=CARTESIAN_POINT('Ctrl Pts',(-3.10606470275517,61.9062463504092,
9.55948420107058));
#281940=CARTESIAN_POINT('Ctrl Pts',(-4.62745677209135E-14,62.0562463504086,
10.5687058007695));
#281941=CARTESIAN_POINT('Ctrl Pts',(3.10606470275507,62.206246350408,9.55948420107058));
#281942=CARTESIAN_POINT('Ctrl Pts',(6.2121294055102,62.3562463504074,8.55026260137164));
#281943=CARTESIAN_POINT('Ctrl Pts',(8.1317829630692,62.5062463504068,5.90808615117925));
#281944=CARTESIAN_POINT('Ctrl Pts',(10.0514365206282,62.6562463504062,3.26590970098687));
#281945=CARTESIAN_POINT('Ctrl Pts',(10.0514365206282,62.8062463504056,-1.23094595618202E-15));
#281946=CARTESIAN_POINT('Ctrl Pts',(10.0514365206282,62.956246350405,-3.26590970098687));
#281947=CARTESIAN_POINT('Ctrl Pts',(8.1317829630692,63.1062463504044,-5.90808615117926));
#281948=CARTESIAN_POINT('Ctrl Pts',(6.21212940551019,63.2562463504038,-8.55026260137164));
#281949=CARTESIAN_POINT('Ctrl Pts',(3.10606470275507,63.4062463504032,-9.55948420107058));
#281950=CARTESIAN_POINT('Ctrl Pts',(-4.9727008702753E-14,63.5562463504026,
-10.5687058007695));
#281951=CARTESIAN_POINT('Ctrl Pts',(-3.10606470275517,63.706246350402,-9.55948420107058));
#281952=CARTESIAN_POINT('Ctrl Pts',(-6.21212940551029,63.8562463504014,
-8.55026260137164));
#281953=CARTESIAN_POINT('Ctrl Pts',(-8.1317829630693,64.0062463504008,-5.90808615117925));
#281954=CARTESIAN_POINT('Ctrl Pts',(-10.0514365206283,64.1562463504002,
-3.26590970098687));
#281955=CARTESIAN_POINT('Ctrl Pts',(-10.0514365206283,64.3062463503996,
2.46189191236404E-15));
#281956=CARTESIAN_POINT('Ctrl Pts',(-10.0514365206283,64.456246350399,3.26590970098687));
#281957=CARTESIAN_POINT('Ctrl Pts',(-8.1317829630693,64.6062463503984,5.90808615117926));
#281958=CARTESIAN_POINT('Ctrl Pts',(-6.21212940551029,64.7562463503978,
8.55026260137164));
#281959=CARTESIAN_POINT('Ctrl Pts',(-3.10606470275517,64.9062463503972,
9.55948420107058));
#281960=CARTESIAN_POINT('Ctrl Pts',(-4.80022769925754E-14,65.0562463503966,
10.5687058007695));
#281961=CARTESIAN_POINT('Ctrl Pts',(3.10606470275507,65.206246350396,9.55948420107058));
#281962=CARTESIAN_POINT('Ctrl Pts',(6.21212940551019,65.3562463503954,8.55026260137164));
#281963=CARTESIAN_POINT('Ctrl Pts',(8.1317829630692,65.5062463503948,5.90808615117925));
#281964=CARTESIAN_POINT('Ctrl Pts',(10.0514365206282,65.6562463503942,3.26590970098687));
#281965=CARTESIAN_POINT('Ctrl Pts',(10.0514365206282,65.8062463503936,-1.23094595618202E-15));
#281966=CARTESIAN_POINT('Ctrl Pts',(10.0514365206282,65.956246350393,-3.26590970098687));
#281967=CARTESIAN_POINT('Ctrl Pts',(8.13178296306919,66.1062463503924,-5.90808615117926));
#281968=CARTESIAN_POINT('Ctrl Pts',(6.21212940551019,66.2562463503918,-8.55026260137164));
#281969=CARTESIAN_POINT('Ctrl Pts',(3.10606470275507,66.4062463503912,-9.55948420107058));
#281970=CARTESIAN_POINT('Ctrl Pts',(-5.14547179744148E-14,66.5562463503906,
-10.5687058007695));
#281971=CARTESIAN_POINT('Ctrl Pts',(-3.10606470275517,66.70624635039,-9.55948420107058));
#281972=CARTESIAN_POINT('Ctrl Pts',(-6.21212940551029,66.8562463503894,
-8.55026260137164));
#281973=CARTESIAN_POINT('Ctrl Pts',(-8.1317829630693,67.0062463503888,-5.90808615117925));
#281974=CARTESIAN_POINT('Ctrl Pts',(-10.0514365206283,67.1562463503882,
-3.26590970098687));
#281975=CARTESIAN_POINT('Ctrl Pts',(-10.0514365206283,67.3062463503876,
2.46189191236404E-15));
#281976=CARTESIAN_POINT('Ctrl Pts',(-10.0514365206283,67.456246350387,3.26590970098687));
#281977=CARTESIAN_POINT('Ctrl Pts',(-8.1317829630693,67.6062463503864,5.90808615117926));
#281978=CARTESIAN_POINT('Ctrl Pts',(-6.21212940551029,67.7562463503858,
8.55026260137164));
#281979=CARTESIAN_POINT('Ctrl Pts',(-3.10606470275517,67.9062463503852,
9.55948420107058));
#281980=CARTESIAN_POINT('Ctrl Pts',(-4.97299862642372E-14,68.0562463503846,
10.5687058007695));
#281981=CARTESIAN_POINT('Ctrl Pts',(3.10606470275507,68.206246350384,9.55948420107058));
#281982=CARTESIAN_POINT('Ctrl Pts',(6.21212940551019,68.3562463503834,8.55026260137164));
#281983=CARTESIAN_POINT('Ctrl Pts',(8.13178296306919,68.5062463503828,5.90808615117925));
#281984=CARTESIAN_POINT('Ctrl Pts',(10.0514365206282,68.6562463503822,3.26590970098687));
#281985=CARTESIAN_POINT('Ctrl Pts',(10.0514365206282,68.8062463503816,-1.23094595618202E-15));
#281986=CARTESIAN_POINT('Ctrl Pts',(10.0514365206282,68.956246350381,-3.26590970098687));
#281987=CARTESIAN_POINT('Ctrl Pts',(8.13178296306919,69.1062463503804,-5.90808615117926));
#281988=CARTESIAN_POINT('Ctrl Pts',(6.21212940551019,69.2562463503798,-8.55026260137164));
#281989=CARTESIAN_POINT('Ctrl Pts',(3.10606470275507,69.4062463503792,-9.55948420107058));
#281990=CARTESIAN_POINT('Ctrl Pts',(-5.31824272460766E-14,69.5562463503786,
-10.5687058007695));
#281991=CARTESIAN_POINT('Ctrl Pts',(-3.10606470275517,69.706246350378,-9.55948420107058));
#281992=CARTESIAN_POINT('Ctrl Pts',(-6.21212940551029,69.8562463503774,
-8.55026260137164));
#281993=CARTESIAN_POINT('Ctrl Pts',(-8.1317829630693,70.0062463503768,-5.90808615117925));
#281994=CARTESIAN_POINT('Ctrl Pts',(-10.0514365206283,70.1562463503762,
-3.26590970098687));
#281995=CARTESIAN_POINT('Ctrl Pts',(-10.0514365206283,70.3062463503756,
2.46189191236404E-15));
#281996=CARTESIAN_POINT('Ctrl Pts',(-10.0514365206283,70.456246350375,3.26590970098687));
#281997=CARTESIAN_POINT('Ctrl Pts',(-8.1317829630693,70.6062463503744,5.90808615117926));
#281998=CARTESIAN_POINT('Ctrl Pts',(-6.21212940551029,70.7562463503738,
8.55026260137164));
#281999=CARTESIAN_POINT('Ctrl Pts',(-3.10606470275517,70.9062463503732,
9.55948420107058));
#282000=CARTESIAN_POINT('Ctrl Pts',(-5.1457695535899E-14,71.0562463503726,
10.5687058007695));
#282001=CARTESIAN_POINT('Ctrl Pts',(3.10606470275507,71.206246350372,9.55948420107058));
#282002=CARTESIAN_POINT('Ctrl Pts',(6.21212940551019,71.3562463503714,8.55026260137164));
#282003=CARTESIAN_POINT('Ctrl Pts',(8.13178296306919,71.5062463503708,5.90808615117925));
#282004=CARTESIAN_POINT('Ctrl Pts',(10.0514365206282,71.6562463503702,3.26590970098687));
#282005=CARTESIAN_POINT('Ctrl Pts',(10.0514365206282,71.8062463503696,-1.23094595618202E-15));
#282006=CARTESIAN_POINT('Ctrl Pts',(10.0514365206282,71.956246350369,-3.26590970098687));
#282007=CARTESIAN_POINT('Ctrl Pts',(8.13178296306919,72.1062463503684,-5.90808615117926));
#282008=CARTESIAN_POINT('Ctrl Pts',(6.21212940551019,72.2562463503678,-8.55026260137164));
#282009=CARTESIAN_POINT('Ctrl Pts',(3.10606470275507,72.4062463503672,-9.55948420107058));
#282010=CARTESIAN_POINT('Ctrl Pts',(-5.49101365177385E-14,72.5562463503666,
-10.5687058007695));
#282011=CARTESIAN_POINT('Ctrl Pts',(-3.10606470275518,72.706246350366,-9.55948420107058));
#282012=CARTESIAN_POINT('Ctrl Pts',(-6.2121294055103,72.8562463503654,-8.55026260137164));
#282013=CARTESIAN_POINT('Ctrl Pts',(-8.1317829630693,73.0062463503648,-5.90808615117925));
#282014=CARTESIAN_POINT('Ctrl Pts',(-10.0514365206283,73.1562463503642,
-3.26590970098687));
#282015=CARTESIAN_POINT('Ctrl Pts',(-10.0514365206283,73.3062463503636,
2.46189191236404E-15));
#282016=CARTESIAN_POINT('Ctrl Pts',(-10.0514365206283,73.456246350363,3.26590970098687));
#282017=CARTESIAN_POINT('Ctrl Pts',(-8.1317829630693,73.6062463503624,5.90808615117926));
#282018=CARTESIAN_POINT('Ctrl Pts',(-6.21212940551029,73.7562463503618,
8.55026260137164));
#282019=CARTESIAN_POINT('Ctrl Pts',(-3.10606470275517,73.9062463503612,
9.55948420107058));
#282020=CARTESIAN_POINT('Ctrl Pts',(-5.31854048075609E-14,74.0562463503606,
10.5687058007695));
#282021=CARTESIAN_POINT('Ctrl Pts',(3.10606470275507,74.20624635036,9.55948420107058));
#282022=CARTESIAN_POINT('Ctrl Pts',(6.21212940551019,74.3562463503594,8.55026260137164));
#282023=CARTESIAN_POINT('Ctrl Pts',(8.13178296306919,74.5062463503588,5.90808615117925));
#282024=CARTESIAN_POINT('Ctrl Pts',(10.0514365206282,74.6562463503582,3.26590970098687));
#282025=CARTESIAN_POINT('Ctrl Pts',(10.0514365206282,74.8062463503576,-1.23094595618202E-15));
#282026=CARTESIAN_POINT('Ctrl Pts',(10.0514365206282,74.956246350357,-3.26590970098687));
#282027=CARTESIAN_POINT('Ctrl Pts',(8.13178296306919,75.1062463503564,-5.90808615117926));
#282028=CARTESIAN_POINT('Ctrl Pts',(6.21212940551018,75.2562463503558,-8.55026260137164));
#282029=CARTESIAN_POINT('Ctrl Pts',(3.10606470275506,75.4062463503552,-9.55948420107058));
#282030=CARTESIAN_POINT('Ctrl Pts',(-5.66378457894003E-14,75.5562463503546,
-10.5687058007695));
#282031=CARTESIAN_POINT('Ctrl Pts',(-3.10606470275518,75.706246350354,-9.55948420107058));
#282032=CARTESIAN_POINT('Ctrl Pts',(-6.2121294055103,75.8562463503534,-8.55026260137164));
#282033=CARTESIAN_POINT('Ctrl Pts',(-8.1317829630693,76.0062463503528,-5.90808615117925));
#282034=CARTESIAN_POINT('Ctrl Pts',(-10.0514365206283,76.1562463503522,
-3.26590970098687));
#282035=CARTESIAN_POINT('Ctrl Pts',(-10.0514365206283,76.3062463503516,
2.46189191236404E-15));
#282036=CARTESIAN_POINT('Ctrl Pts',(-10.0514365206283,76.456246350351,3.26590970098687));
#282037=CARTESIAN_POINT('Ctrl Pts',(-8.1317829630693,76.6062463503504,5.90808615117926));
#282038=CARTESIAN_POINT('Ctrl Pts',(-6.21212940551029,76.7562463503498,
8.55026260137164));
#282039=CARTESIAN_POINT('Ctrl Pts',(-3.10606470275518,76.9062463503492,
9.55948420107058));
#282040=CARTESIAN_POINT('Ctrl Pts',(-5.49131140792227E-14,77.0562463503486,
10.5687058007695));
#282041=CARTESIAN_POINT('Ctrl Pts',(3.10606470275506,77.206246350348,9.55948420107058));
#282042=CARTESIAN_POINT('Ctrl Pts',(6.21212940551019,77.3562463503474,8.55026260137164));
#282043=CARTESIAN_POINT('Ctrl Pts',(8.13178296306919,77.5062463503468,5.90808615117925));
#282044=CARTESIAN_POINT('Ctrl Pts',(10.0514365206282,77.6562463503462,3.26590970098687));
#282045=CARTESIAN_POINT('Ctrl Pts',(10.0514365206282,77.8062463503456,-1.23094595618202E-15));
#282046=CARTESIAN_POINT('Ctrl Pts',(10.0514365206282,77.956246350345,-3.26590970098687));
#282047=CARTESIAN_POINT('Ctrl Pts',(8.13178296306919,78.1062463503444,-5.90808615117926));
#282048=CARTESIAN_POINT('Ctrl Pts',(6.21212940551018,78.2562463503438,-8.55026260137164));
#282049=CARTESIAN_POINT('Ctrl Pts',(3.10606470275506,78.4062463503432,-9.55948420107058));
#282050=CARTESIAN_POINT('Ctrl Pts',(-5.83655550610621E-14,78.5562463503426,
-10.5687058007695));
#282051=CARTESIAN_POINT('Ctrl Pts',(-3.10606470275518,78.706246350342,-9.55948420107058));
#282052=CARTESIAN_POINT('Ctrl Pts',(-6.2121294055103,78.8562463503414,-8.55026260137164));
#282053=CARTESIAN_POINT('Ctrl Pts',(-8.13178296306931,79.0062463503408,
-5.90808615117925));
#282054=CARTESIAN_POINT('Ctrl Pts',(-10.0514365206283,79.1562463503402,
-3.26590970098687));
#282055=CARTESIAN_POINT('Ctrl Pts',(-10.0514365206283,79.3062463503396,
2.46189191236404E-15));
#282056=CARTESIAN_POINT('Ctrl Pts',(-10.0514365206283,79.456246350339,3.26590970098687));
#282057=CARTESIAN_POINT('Ctrl Pts',(-8.13178296306931,79.6062463503384,
5.90808615117926));
#282058=CARTESIAN_POINT('Ctrl Pts',(-6.2121294055103,79.7562463503378,8.55026260137164));
#282059=CARTESIAN_POINT('Ctrl Pts',(-3.10606470275518,79.9062463503372,
9.55948420107058));
#282060=CARTESIAN_POINT('Ctrl Pts',(-5.66408233508846E-14,80.0562463503366,
10.5687058007695));
#282061=CARTESIAN_POINT('Ctrl Pts',(3.10606470275506,80.206246350336,9.55948420107058));
#282062=CARTESIAN_POINT('Ctrl Pts',(6.21212940551018,80.3562463503354,8.55026260137164));
#282063=CARTESIAN_POINT('Ctrl Pts',(8.13178296306919,80.5062463503348,5.90808615117925));
#282064=CARTESIAN_POINT('Ctrl Pts',(10.0514365206282,80.6562463503342,3.26590970098687));
#282065=CARTESIAN_POINT('Ctrl Pts',(10.0514365206282,80.8062463503336,-1.23094595618202E-15));
#282066=CARTESIAN_POINT('Ctrl Pts',(10.0514365206282,80.956246350333,-3.26590970098687));
#282067=CARTESIAN_POINT('Ctrl Pts',(8.13178296306919,81.1062463503324,-5.90808615117926));
#282068=CARTESIAN_POINT('Ctrl Pts',(6.21212940551018,81.2562463503318,-8.55026260137164));
#282069=CARTESIAN_POINT('Ctrl Pts',(3.10606470275506,81.4062463503312,-9.55948420107058));
#282070=CARTESIAN_POINT('Ctrl Pts',(-6.0093264332724E-14,81.5562463503306,
-10.5687058007695));
#282071=CARTESIAN_POINT('Ctrl Pts',(-3.10606470275518,81.70624635033,-9.55948420107058));
#282072=CARTESIAN_POINT('Ctrl Pts',(-6.2121294055103,81.8562463503294,-8.55026260137164));
#282073=CARTESIAN_POINT('Ctrl Pts',(-8.13178296306931,82.0062463503288,
-5.90808615117925));
#282074=CARTESIAN_POINT('Ctrl Pts',(-10.0514365206283,82.1562463503282,
-3.26590970098687));
#282075=CARTESIAN_POINT('Ctrl Pts',(-10.0514365206283,82.3062463503276,
2.46189191236404E-15));
#282076=CARTESIAN_POINT('Ctrl Pts',(-10.0514365206283,82.456246350327,3.26590970098687));
#282077=CARTESIAN_POINT('Ctrl Pts',(-8.13178296306931,82.6062463503264,
5.90808615117926));
#282078=CARTESIAN_POINT('Ctrl Pts',(-6.2121294055103,82.7562463503258,8.55026260137164));
#282079=CARTESIAN_POINT('Ctrl Pts',(-3.10606470275518,82.9062463503252,
9.55948420107058));
#282080=CARTESIAN_POINT('Ctrl Pts',(-5.83685326225464E-14,83.0562463503246,
10.5687058007695));
#282081=CARTESIAN_POINT('Ctrl Pts',(3.10606470275506,83.206246350324,9.55948420107058));
#282082=CARTESIAN_POINT('Ctrl Pts',(6.21212940551018,83.3562463503234,8.55026260137164));
#282083=CARTESIAN_POINT('Ctrl Pts',(8.13178296306918,83.5062463503228,5.90808615117925));
#282084=CARTESIAN_POINT('Ctrl Pts',(10.0514365206282,83.6562463503222,3.26590970098687));
#282085=CARTESIAN_POINT('Ctrl Pts',(10.0514365206282,83.8062463503216,-1.23094595618202E-15));
#282086=CARTESIAN_POINT('Ctrl Pts',(10.0514365206282,83.956246350321,-3.26590970098687));
#282087=CARTESIAN_POINT('Ctrl Pts',(8.13178296306918,84.1062463503204,-5.90808615117926));
#282088=CARTESIAN_POINT('Ctrl Pts',(6.21212940551018,84.2562463503198,-8.55026260137164));
#282089=CARTESIAN_POINT('Ctrl Pts',(3.10606470275506,84.4062463503192,-9.55948420107058));
#282090=CARTESIAN_POINT('Ctrl Pts',(-6.18209736043858E-14,84.5562463503186,
-10.5687058007695));
#282091=CARTESIAN_POINT('Ctrl Pts',(-3.10606470275518,84.706246350318,-9.55948420107058));
#282092=CARTESIAN_POINT('Ctrl Pts',(-6.2121294055103,84.8562463503174,-8.55026260137164));
#282093=CARTESIAN_POINT('Ctrl Pts',(-8.13178296306931,85.0062463503168,
-5.90808615117925));
#282094=CARTESIAN_POINT('Ctrl Pts',(-10.0514365206283,85.1562463503162,
-3.26590970098687));
#282095=CARTESIAN_POINT('Ctrl Pts',(-10.0514365206283,85.3062463503156,
2.46189191236404E-15));
#282096=CARTESIAN_POINT('Ctrl Pts',(-10.0514365206283,85.456246350315,3.26590970098687));
#282097=CARTESIAN_POINT('Ctrl Pts',(-8.13178296306931,85.6062463503144,
5.90808615117926));
#282098=CARTESIAN_POINT('Ctrl Pts',(-6.2121294055103,85.7562463503138,8.55026260137164));
#282099=CARTESIAN_POINT('Ctrl Pts',(-3.10606470275518,85.9062463503132,
9.55948420107058));
#282100=CARTESIAN_POINT('Ctrl Pts',(-6.00962418942082E-14,86.0562463503126,
10.5687058007695));
#282101=CARTESIAN_POINT('Ctrl Pts',(3.10606470275506,86.206246350312,9.55948420107058));
#282102=CARTESIAN_POINT('Ctrl Pts',(6.21212940551018,86.3562463503114,8.55026260137164));
#282103=CARTESIAN_POINT('Ctrl Pts',(8.13178296306918,86.5062463503108,5.90808615117925));
#282104=CARTESIAN_POINT('Ctrl Pts',(10.0514365206282,86.6562463503102,3.26590970098687));
#282105=CARTESIAN_POINT('Ctrl Pts',(10.0514365206282,86.8062463503096,-1.23094595618202E-15));
#282106=CARTESIAN_POINT('Ctrl Pts',(10.0514365206282,86.956246350309,-3.26590970098687));
#282107=CARTESIAN_POINT('Ctrl Pts',(8.13178296306918,87.1062463503084,-5.90808615117926));
#282108=CARTESIAN_POINT('Ctrl Pts',(6.21212940551018,87.2562463503078,-8.55026260137164));
#282109=CARTESIAN_POINT('Ctrl Pts',(3.10606470275506,87.4062463503072,-9.55948420107058));
#282110=CARTESIAN_POINT('Ctrl Pts',(-6.35486828760476E-14,87.5562463503066,
-10.5687058007695));
#282111=CARTESIAN_POINT('Ctrl Pts',(-3.10606470275518,87.706246350306,-9.55948420107058));
#282112=CARTESIAN_POINT('Ctrl Pts',(-6.21212940551031,87.8562463503054,
-8.55026260137164));
#282113=CARTESIAN_POINT('Ctrl Pts',(-8.13178296306931,88.0062463503048,
-5.90808615117925));
#282114=CARTESIAN_POINT('Ctrl Pts',(-10.0514365206283,88.1562463503042,
-3.26590970098687));
#282115=CARTESIAN_POINT('Ctrl Pts',(-10.0514365206283,88.3062463503036,
2.46189191236404E-15));
#282116=CARTESIAN_POINT('Ctrl Pts',(-10.0514365206283,88.456246350303,3.26590970098687));
#282117=CARTESIAN_POINT('Ctrl Pts',(-8.13178296306931,88.6062463503024,
5.90808615117926));
#282118=CARTESIAN_POINT('Ctrl Pts',(-6.2121294055103,88.7562463503018,8.55026260137164));
#282119=CARTESIAN_POINT('Ctrl Pts',(-3.10606470275518,88.9062463503012,
9.55948420107058));
#282120=CARTESIAN_POINT('Ctrl Pts',(-6.18239511658701E-14,89.0562463503006,
10.5687058007695));
#282121=CARTESIAN_POINT('Ctrl Pts',(3.10606470275506,89.2062463503,9.55948420107058));
#282122=CARTESIAN_POINT('Ctrl Pts',(6.21212940551018,89.3562463502994,8.55026260137164));
#282123=CARTESIAN_POINT('Ctrl Pts',(8.13178296306918,89.5062463502988,5.90808615117925));
#282124=CARTESIAN_POINT('Ctrl Pts',(10.0514365206282,89.6562463502982,3.26590970098687));
#282125=CARTESIAN_POINT('Ctrl Pts',(10.0514365206282,89.8062463502976,-1.23094595618202E-15));
#282126=CARTESIAN_POINT('Ctrl Pts',(10.0514365206282,89.956246350297,-3.26590970098687));
#282127=CARTESIAN_POINT('Ctrl Pts',(8.13178296306918,90.1062463502964,-5.90808615117926));
#282128=CARTESIAN_POINT('Ctrl Pts',(6.21212940551018,90.2562463502958,-8.55026260137164));
#282129=CARTESIAN_POINT('Ctrl Pts',(3.10606470275506,90.4062463502952,-9.55948420107058));
#282130=CARTESIAN_POINT('Ctrl Pts',(-6.52763921477095E-14,90.5562463502946,
-10.5687058007695));
#282131=CARTESIAN_POINT('Ctrl Pts',(-3.10606470275519,90.706246350294,-9.55948420107058));
#282132=CARTESIAN_POINT('Ctrl Pts',(-6.21212940551031,90.8562463502934,
-8.55026260137164));
#282133=CARTESIAN_POINT('Ctrl Pts',(-8.13178296306931,91.0062463502928,
-5.90808615117925));
#282134=CARTESIAN_POINT('Ctrl Pts',(-10.0514365206283,91.1562463502922,
-3.26590970098687));
#282135=CARTESIAN_POINT('Ctrl Pts',(-10.0514365206283,91.3062463502916,
2.46189191236404E-15));
#282136=CARTESIAN_POINT('Ctrl Pts',(-10.0514365206283,91.456246350291,3.26590970098687));
#282137=CARTESIAN_POINT('Ctrl Pts',(-8.13178296306931,91.6062463502904,
5.90808615117926));
#282138=CARTESIAN_POINT('Ctrl Pts',(-6.21212940551031,91.7562463502898,
8.55026260137164));
#282139=CARTESIAN_POINT('Ctrl Pts',(-3.10606470275518,91.9062463502892,
9.55948420107058));
#282140=CARTESIAN_POINT('Ctrl Pts',(-6.35516604375319E-14,92.0562463502886,
10.5687058007695));
#282141=CARTESIAN_POINT('Ctrl Pts',(3.10606470275506,92.206246350288,9.55948420107058));
#282142=CARTESIAN_POINT('Ctrl Pts',(6.21212940551018,92.3562463502874,8.55026260137164));
#282143=CARTESIAN_POINT('Ctrl Pts',(8.13178296306918,92.5062463502868,5.90808615117925));
#282144=CARTESIAN_POINT('Ctrl Pts',(10.0514365206282,92.6562463502862,3.26590970098687));
#282145=CARTESIAN_POINT('Ctrl Pts',(10.0514365206282,92.8062463502856,-1.23094595618202E-15));
#282146=CARTESIAN_POINT('Ctrl Pts',(10.0514365206282,92.956246350285,-3.26590970098687));
#282147=CARTESIAN_POINT('Ctrl Pts',(8.13178296306918,93.1062463502844,-5.90808615117926));
#282148=CARTESIAN_POINT('Ctrl Pts',(6.21212940551018,93.2562463502838,-8.55026260137164));
#282149=CARTESIAN_POINT('Ctrl Pts',(3.10606470275505,93.4062463502832,-9.55948420107058));
#282150=CARTESIAN_POINT('Ctrl Pts',(-6.70041014193713E-14,93.5562463502826,
-10.5687058007695));
#282151=CARTESIAN_POINT('Ctrl Pts',(-3.10606470275519,93.706246350282,-9.55948420107058));
#282152=CARTESIAN_POINT('Ctrl Pts',(-6.21212940551031,93.8562463502814,
-8.55026260137164));
#282153=CARTESIAN_POINT('Ctrl Pts',(-8.13178296306931,94.0062463502808,
-5.90808615117925));
#282154=CARTESIAN_POINT('Ctrl Pts',(-10.0514365206283,94.1562463502802,
-3.26590970098687));
#282155=CARTESIAN_POINT('Ctrl Pts',(-10.0514365206283,94.3062463502796,
2.46189191236404E-15));
#282156=CARTESIAN_POINT('Ctrl Pts',(-10.0514365206283,94.456246350279,3.26590970098687));
#282157=CARTESIAN_POINT('Ctrl Pts',(-8.13178296306931,94.6062463502784,
5.90808615117926));
#282158=CARTESIAN_POINT('Ctrl Pts',(-6.21212940551031,94.7562463502778,
8.55026260137164));
#282159=CARTESIAN_POINT('Ctrl Pts',(-3.10606470275519,94.9062463502772,
9.55948420107058));
#282160=CARTESIAN_POINT('Ctrl Pts',(-6.52793697091937E-14,95.0562463502766,
10.5687058007695));
#282161=CARTESIAN_POINT('Ctrl Pts',(3.10606470275505,95.206246350276,9.55948420107058));
#282162=CARTESIAN_POINT('Ctrl Pts',(6.21212940551018,95.3562463502754,8.55026260137164));
#282163=CARTESIAN_POINT('Ctrl Pts',(8.13178296306918,95.5062463502748,5.90808615117925));
#282164=CARTESIAN_POINT('Ctrl Pts',(10.0514365206282,95.6562463502742,3.26590970098687));
#282165=CARTESIAN_POINT('Ctrl Pts',(10.0514365206282,95.8062463502736,-1.23094595618202E-15));
#282166=CARTESIAN_POINT('Ctrl Pts',(10.0514365206282,95.956246350273,-3.26590970098687));
#282167=CARTESIAN_POINT('Ctrl Pts',(8.13178296306918,96.1062463502724,-5.90808615117926));
#282168=CARTESIAN_POINT('Ctrl Pts',(6.21212940551017,96.2562463502718,-8.55026260137164));
#282169=CARTESIAN_POINT('Ctrl Pts',(3.10606470275505,96.4062463502712,-9.55948420107058));
#282170=CARTESIAN_POINT('Ctrl Pts',(-6.87318106910331E-14,96.5562463502706,
-10.5687058007695));
#282171=CARTESIAN_POINT('Ctrl Pts',(-3.10606470275519,96.70624635027,-9.55948420107058));
#282172=CARTESIAN_POINT('Ctrl Pts',(-6.21212940551031,96.8562463502694,
-8.55026260137164));
#282173=CARTESIAN_POINT('Ctrl Pts',(-8.13178296306931,97.0062463502688,
-5.90808615117925));
#282174=CARTESIAN_POINT('Ctrl Pts',(-10.0514365206283,97.1562463502682,
-3.26590970098687));
#282175=CARTESIAN_POINT('Ctrl Pts',(-10.0514365206283,97.3062463502676,
2.46189191236404E-15));
#282176=CARTESIAN_POINT('Ctrl Pts',(-10.0514365206283,97.456246350267,3.26590970098687));
#282177=CARTESIAN_POINT('Ctrl Pts',(-8.13178296306931,97.6062463502664,
5.90808615117926));
#282178=CARTESIAN_POINT('Ctrl Pts',(-6.21212940551031,97.7562463502658,
8.55026260137164));
#282179=CARTESIAN_POINT('Ctrl Pts',(-3.10606470275519,97.9062463502652,
9.55948420107058));
#282180=CARTESIAN_POINT('Ctrl Pts',(-6.70070789808556E-14,98.0562463502646,
10.5687058007695));
#282181=CARTESIAN_POINT('Ctrl Pts',(3.10606470275505,98.206246350264,9.55948420107058));
#282182=CARTESIAN_POINT('Ctrl Pts',(6.21212940551018,98.3562463502634,8.55026260137164));
#282183=CARTESIAN_POINT('Ctrl Pts',(8.13178296306918,98.5062463502628,5.90808615117925));
#282184=CARTESIAN_POINT('Ctrl Pts',(10.0514365206282,98.6562463502622,3.26590970098687));
#282185=CARTESIAN_POINT('Ctrl Pts',(10.0514365206282,98.8062463502616,-1.23094595618202E-15));
#282186=CARTESIAN_POINT('Ctrl Pts',(10.0514365206282,98.956246350261,-3.26590970098687));
#282187=CARTESIAN_POINT('Ctrl Pts',(8.13178296306918,99.1062463502604,-5.90808615117926));
#282188=CARTESIAN_POINT('Ctrl Pts',(6.21212940551017,99.2562463502598,-8.55026260137164));
#282189=CARTESIAN_POINT('Ctrl Pts',(3.10606470275505,99.4062463502592,-9.55948420107058));
#282190=CARTESIAN_POINT('Ctrl Pts',(-7.0459519962695E-14,99.5562463502586,
-10.5687058007695));
#282191=CARTESIAN_POINT('Ctrl Pts',(-3.10606470275519,99.706246350258,-9.55948420107058));
#282192=CARTESIAN_POINT('Ctrl Pts',(-6.21212940551031,99.8562463502574,
-8.55026260137164));
#282193=CARTESIAN_POINT('Ctrl Pts',(-8.13178296306931,100.006246350257,
-5.90808615117925));
#282194=CARTESIAN_POINT('Ctrl Pts',(-10.0514365206283,100.156246350256,
-3.26590970098687));
#282195=CARTESIAN_POINT('Ctrl Pts',(-10.0514365206283,100.306246350256,
2.46189191236404E-15));
#282196=CARTESIAN_POINT('Ctrl Pts',(-10.0514365206283,100.456246350255,
3.26590970098687));
#282197=CARTESIAN_POINT('Ctrl Pts',(-8.13178296306931,100.606246350254,
5.90808615117926));
#282198=CARTESIAN_POINT('Ctrl Pts',(-6.21212940551031,100.756246350254,
8.55026260137164));
#282199=CARTESIAN_POINT('Ctrl Pts',(-3.10606470275519,100.906246350253,
9.55948420107058));
#282200=CARTESIAN_POINT('Ctrl Pts',(-6.87347882525174E-14,101.056246350253,
10.5687058007695));
#282201=CARTESIAN_POINT('Ctrl Pts',(3.10606470275505,101.206246350252,9.55948420107058));
#282202=CARTESIAN_POINT('Ctrl Pts',(6.21212940551017,101.356246350251,8.55026260137164));
#282203=CARTESIAN_POINT('Ctrl Pts',(8.13178296306917,101.506246350251,5.90808615117925));
#282204=CARTESIAN_POINT('Ctrl Pts',(10.0514365206282,101.65624635025,3.26590970098687));
#282205=CARTESIAN_POINT('Ctrl Pts',(10.0514365206282,101.80624635025,-1.23094595618202E-15));
#282206=CARTESIAN_POINT('Ctrl Pts',(10.0514365206282,101.956246350249,-3.26590970098687));
#282207=CARTESIAN_POINT('Ctrl Pts',(8.13178296306917,102.106246350248,-5.90808615117926));
#282208=CARTESIAN_POINT('Ctrl Pts',(6.21212940551017,102.256246350248,-8.55026260137164));
#282209=CARTESIAN_POINT('Ctrl Pts',(3.10606470275505,102.406246350247,-9.55948420107058));
#282210=CARTESIAN_POINT('Ctrl Pts',(-7.21872292343569E-14,102.556246350247,
-10.5687058007695));
#282211=CARTESIAN_POINT('Ctrl Pts',(-3.10606470275519,102.706246350246,
-9.55948420107058));
#282212=CARTESIAN_POINT('Ctrl Pts',(-6.21212940551031,102.856246350245,
-8.55026260137164));
#282213=CARTESIAN_POINT('Ctrl Pts',(-8.13178296306932,103.006246350245,
-5.90808615117925));
#282214=CARTESIAN_POINT('Ctrl Pts',(-10.0514365206283,103.156246350244,
-3.26590970098687));
#282215=CARTESIAN_POINT('Ctrl Pts',(-10.0514365206283,103.306246350244,
2.46189191236404E-15));
#282216=CARTESIAN_POINT('Ctrl Pts',(-10.0514365206283,103.456246350243,
3.26590970098687));
#282217=CARTESIAN_POINT('Ctrl Pts',(-8.13178296306932,103.606246350242,
5.90808615117926));
#282218=CARTESIAN_POINT('Ctrl Pts',(-6.21212940551031,103.756246350242,
8.55026260137164));
#282219=CARTESIAN_POINT('Ctrl Pts',(-3.10606470275519,103.906246350241,
9.55948420107058));
#282220=CARTESIAN_POINT('Ctrl Pts',(-7.04624975241793E-14,104.056246350241,
10.5687058007695));
#282221=CARTESIAN_POINT('Ctrl Pts',(3.10606470275505,104.20624635024,9.55948420107058));
#282222=CARTESIAN_POINT('Ctrl Pts',(6.21212940551017,104.356246350239,8.55026260137164));
#282223=CARTESIAN_POINT('Ctrl Pts',(8.13178296306917,104.506246350239,5.90808615117925));
#282224=CARTESIAN_POINT('Ctrl Pts',(10.0514365206282,104.656246350238,3.26590970098687));
#282225=CARTESIAN_POINT('Ctrl Pts',(10.0514365206282,104.806246350238,-1.23094595618202E-15));
#282226=CARTESIAN_POINT('Ctrl Pts',(10.0514365206282,104.956246350237,-3.26590970098687));
#282227=CARTESIAN_POINT('Ctrl Pts',(8.13178296306917,105.106246350236,-5.90808615117926));
#282228=CARTESIAN_POINT('Ctrl Pts',(6.21212940551017,105.256246350236,-8.55026260137164));
#282229=CARTESIAN_POINT('Ctrl Pts',(3.10606470275505,105.406246350235,-9.55948420107058));
#282230=CARTESIAN_POINT('Ctrl Pts',(-7.39149385060187E-14,105.556246350235,
-10.5687058007695));
#282231=CARTESIAN_POINT('Ctrl Pts',(-3.1060647027552,105.706246350234,-9.55948420107058));
#282232=CARTESIAN_POINT('Ctrl Pts',(-6.21212940551032,105.856246350233,
-8.55026260137164));
#282233=CARTESIAN_POINT('Ctrl Pts',(-8.13178296306932,106.006246350233,
-5.90808615117925));
#282234=CARTESIAN_POINT('Ctrl Pts',(-10.0514365206283,106.156246350232,
-3.26590970098687));
#282235=CARTESIAN_POINT('Ctrl Pts',(-10.0514365206283,106.306246350232,
2.46189191236404E-15));
#282236=CARTESIAN_POINT('Ctrl Pts',(-10.0514365206283,106.456246350231,
3.26590970098687));
#282237=CARTESIAN_POINT('Ctrl Pts',(-8.13178296306932,106.60624635023,5.90808615117926));
#282238=CARTESIAN_POINT('Ctrl Pts',(-6.21212940551031,106.75624635023,8.55026260137164));
#282239=CARTESIAN_POINT('Ctrl Pts',(-3.10606470275519,106.906246350229,
9.55948420107058));
#282240=CARTESIAN_POINT('Ctrl Pts',(-7.21902067958411E-14,107.056246350229,
10.5687058007695));
#282241=CARTESIAN_POINT('Ctrl Pts',(3.10606470275505,107.206246350228,9.55948420107058));
#282242=CARTESIAN_POINT('Ctrl Pts',(6.21212940551017,107.356246350227,8.55026260137164));
#282243=CARTESIAN_POINT('Ctrl Pts',(8.13178296306917,107.506246350227,5.90808615117925));
#282244=CARTESIAN_POINT('Ctrl Pts',(10.0514365206282,107.656246350226,3.26590970098687));
#282245=CARTESIAN_POINT('Ctrl Pts',(10.0514365206282,107.806246350226,-1.23094595618202E-15));
#282246=CARTESIAN_POINT('Ctrl Pts',(10.0514365206282,107.956246350225,-3.26590970098687));
#282247=CARTESIAN_POINT('Ctrl Pts',(8.13178296306917,108.106246350224,-5.90808615117926));
#282248=CARTESIAN_POINT('Ctrl Pts',(6.21212940551017,108.256246350224,-8.55026260137164));
#282249=CARTESIAN_POINT('Ctrl Pts',(3.10606470275505,108.406246350223,-9.55948420107058));
#282250=CARTESIAN_POINT('Ctrl Pts',(-7.56426477776805E-14,108.556246350223,
-10.5687058007695));
#282251=CARTESIAN_POINT('Ctrl Pts',(-3.1060647027552,108.706246350222,-9.55948420107058));
#282252=CARTESIAN_POINT('Ctrl Pts',(-6.21212940551032,108.856246350221,
-8.55026260137164));
#282253=CARTESIAN_POINT('Ctrl Pts',(-8.13178296306932,109.006246350221,
-5.90808615117925));
#282254=CARTESIAN_POINT('Ctrl Pts',(-10.0514365206283,109.15624635022,-3.26590970098687));
#282255=CARTESIAN_POINT('Ctrl Pts',(-10.0514365206283,109.30624635022,2.46189191236404E-15));
#282256=CARTESIAN_POINT('Ctrl Pts',(-10.0514365206283,109.456246350219,
3.26590970098687));
#282257=CARTESIAN_POINT('Ctrl Pts',(-8.13178296306932,109.606246350218,
5.90808615117926));
#282258=CARTESIAN_POINT('Ctrl Pts',(-6.21212940551032,109.756246350218,
8.55026260137164));
#282259=CARTESIAN_POINT('Ctrl Pts',(-3.10606470275519,109.906246350217,
9.55948420107058));
#282260=CARTESIAN_POINT('Ctrl Pts',(-7.39179160675029E-14,110.056246350217,
10.5687058007695));
#282261=CARTESIAN_POINT('Ctrl Pts',(3.10606470275505,110.206246350216,9.55948420107058));
#282262=CARTESIAN_POINT('Ctrl Pts',(6.21212940551017,110.356246350215,8.55026260137164));
#282263=CARTESIAN_POINT('Ctrl Pts',(8.13178296306917,110.506246350215,5.90808615117925));
#282264=CARTESIAN_POINT('Ctrl Pts',(10.0514365206282,110.656246350214,3.26590970098687));
#282265=CARTESIAN_POINT('Ctrl Pts',(10.0514365206282,110.806246350214,-1.23094595618202E-15));
#282266=CARTESIAN_POINT('Ctrl Pts',(10.0514365206282,110.956246350213,-3.26590970098687));
#282267=CARTESIAN_POINT('Ctrl Pts',(8.13178296306917,111.106246350212,-5.90808615117926));
#282268=CARTESIAN_POINT('Ctrl Pts',(6.21212940551017,111.256246350212,-8.55026260137164));
#282269=CARTESIAN_POINT('Ctrl Pts',(3.10606470275504,111.406246350211,-9.55948420107058));
#282270=CARTESIAN_POINT('Ctrl Pts',(-7.73703570493424E-14,111.556246350211,
-10.5687058007695));
#282271=CARTESIAN_POINT('Ctrl Pts',(-3.1060647027552,111.70624635021,-9.55948420107058));
#282272=CARTESIAN_POINT('Ctrl Pts',(-6.21212940551032,111.856246350209,
-8.55026260137164));
#282273=CARTESIAN_POINT('Ctrl Pts',(-8.13178296306932,112.006246350209,
-5.90808615117925));
#282274=CARTESIAN_POINT('Ctrl Pts',(-10.0514365206283,112.156246350208,
-3.26590970098687));
#282275=CARTESIAN_POINT('Ctrl Pts',(-10.0514365206283,112.306246350208,
2.46189191236404E-15));
#282276=CARTESIAN_POINT('Ctrl Pts',(-10.0514365206283,112.456246350207,
3.26590970098687));
#282277=CARTESIAN_POINT('Ctrl Pts',(-8.13178296306932,112.606246350206,
5.90808615117926));
#282278=CARTESIAN_POINT('Ctrl Pts',(-6.21212940551032,112.756246350206,
8.55026260137164));
#282279=CARTESIAN_POINT('Ctrl Pts',(-3.1060647027552,112.906246350205,9.55948420107058));
#282280=CARTESIAN_POINT('Ctrl Pts',(-7.56456253391648E-14,113.056246350205,
10.5687058007695));
#282281=CARTESIAN_POINT('Ctrl Pts',(3.10606470275504,113.206246350204,9.55948420107058));
#282282=CARTESIAN_POINT('Ctrl Pts',(6.21212940551017,113.356246350203,8.55026260137164));
#282283=CARTESIAN_POINT('Ctrl Pts',(8.13178296306917,113.506246350203,5.90808615117925));
#282284=CARTESIAN_POINT('Ctrl Pts',(10.0514365206282,113.656246350202,3.26590970098687));
#282285=CARTESIAN_POINT('Ctrl Pts',(10.0514365206282,113.806246350202,-1.23094595618202E-15));
#282286=CARTESIAN_POINT('Ctrl Pts',(10.0514365206282,113.956246350201,-3.26590970098687));
#282287=CARTESIAN_POINT('Ctrl Pts',(8.13178296306917,114.1062463502,-5.90808615117926));
#282288=CARTESIAN_POINT('Ctrl Pts',(6.21212940551016,114.2562463502,-8.55026260137164));
#282289=CARTESIAN_POINT('Ctrl Pts',(3.10606470275504,114.406246350199,-9.55948420107058));
#282290=CARTESIAN_POINT('Ctrl Pts',(-7.90980663210042E-14,114.556246350199,
-10.5687058007695));
#282291=CARTESIAN_POINT('Ctrl Pts',(-3.1060647027552,114.706246350198,-9.55948420107058));
#282292=CARTESIAN_POINT('Ctrl Pts',(-6.21212940551032,114.856246350197,
-8.55026260137164));
#282293=CARTESIAN_POINT('Ctrl Pts',(-8.13178296306932,115.006246350197,
-5.90808615117925));
#282294=CARTESIAN_POINT('Ctrl Pts',(-10.0514365206283,115.156246350196,
-3.26590970098687));
#282295=CARTESIAN_POINT('Ctrl Pts',(-10.0514365206283,115.306246350196,
2.46189191236404E-15));
#282296=CARTESIAN_POINT('Ctrl Pts',(-10.0514365206283,115.456246350195,
3.26590970098687));
#282297=CARTESIAN_POINT('Ctrl Pts',(-8.13178296306932,115.606246350194,
5.90808615117926));
#282298=CARTESIAN_POINT('Ctrl Pts',(-6.21212940551032,115.756246350194,
8.55026260137164));
#282299=CARTESIAN_POINT('Ctrl Pts',(-3.1060647027552,115.906246350193,9.55948420107058));
#282300=CARTESIAN_POINT('Ctrl Pts',(-7.73733346108267E-14,116.056246350193,
10.5687058007695));
#282301=CARTESIAN_POINT('Ctrl Pts',(3.10606470275504,116.206246350192,9.55948420107058));
#282302=CARTESIAN_POINT('Ctrl Pts',(6.21212940551017,116.356246350191,8.55026260137164));
#282303=CARTESIAN_POINT('Ctrl Pts',(8.13178296306917,116.506246350191,5.90808615117925));
#282304=CARTESIAN_POINT('Ctrl Pts',(10.0514365206282,116.65624635019,3.26590970098687));
#282305=CARTESIAN_POINT('Ctrl Pts',(10.0514365206282,116.80624635019,-1.23094595618202E-15));
#282306=CARTESIAN_POINT('Ctrl Pts',(10.0514365206282,116.956246350189,-3.26590970098687));
#282307=CARTESIAN_POINT('Ctrl Pts',(8.13178296306917,117.106246350188,-5.90808615117926));
#282308=CARTESIAN_POINT('Ctrl Pts',(6.21212940551016,117.256246350188,-8.55026260137164));
#282309=CARTESIAN_POINT('Ctrl Pts',(3.10606470275504,117.406246350187,-9.55948420107058));
#282310=CARTESIAN_POINT('Ctrl Pts',(-8.0825775592666E-14,117.556246350187,
-10.5687058007695));
#282311=CARTESIAN_POINT('Ctrl Pts',(-3.1060647027552,117.706246350186,-9.55948420107058));
#282312=CARTESIAN_POINT('Ctrl Pts',(-6.21212940551032,117.856246350185,
-8.55026260137164));
#282313=CARTESIAN_POINT('Ctrl Pts',(-8.13178296306933,118.006246350185,
-5.90808615117925));
#282314=CARTESIAN_POINT('Ctrl Pts',(-10.0514365206283,118.156246350184,
-3.26590970098687));
#282315=CARTESIAN_POINT('Ctrl Pts',(-10.0514365206283,118.306246350184,
2.46189191236404E-15));
#282316=CARTESIAN_POINT('Ctrl Pts',(-10.0514365206283,118.456246350183,
3.26590970098687));
#282317=CARTESIAN_POINT('Ctrl Pts',(-8.13178296306933,118.606246350182,
5.90808615117926));
#282318=CARTESIAN_POINT('Ctrl Pts',(-6.21212940551032,118.756246350182,
8.55026260137164));
#282319=CARTESIAN_POINT('Ctrl Pts',(-3.1060647027552,118.906246350181,9.55948420107058));
#282320=CARTESIAN_POINT('Ctrl Pts',(-7.91010438824885E-14,119.056246350181,
10.5687058007695));
#282321=CARTESIAN_POINT('Ctrl Pts',(3.10606470275504,119.20624635018,9.55948420107058));
#282322=CARTESIAN_POINT('Ctrl Pts',(6.21212940551016,119.356246350179,8.55026260137164));
#282323=CARTESIAN_POINT('Ctrl Pts',(8.13178296306916,119.506246350179,5.90808615117925));
#282324=CARTESIAN_POINT('Ctrl Pts',(10.0514365206282,119.656246350178,3.26590970098687));
#282325=CARTESIAN_POINT('Ctrl Pts',(10.0514365206282,119.806246350178,-1.23094595618202E-15));
#282326=CARTESIAN_POINT('Ctrl Pts',(10.0514365206282,119.956246350177,-3.26590970098687));
#282327=CARTESIAN_POINT('Ctrl Pts',(8.13178296306916,120.106246350176,-5.90808615117926));
#282328=CARTESIAN_POINT('Ctrl Pts',(6.21212940551016,120.256246350176,-8.55026260137164));
#282329=CARTESIAN_POINT('Ctrl Pts',(3.10606470275504,120.406246350175,-9.55948420107058));
#282330=CARTESIAN_POINT('Ctrl Pts',(-8.25534848643279E-14,120.556246350175,
-10.5687058007695));
#282331=CARTESIAN_POINT('Ctrl Pts',(-3.1060647027552,120.706246350174,-9.55948420107058));
#282332=CARTESIAN_POINT('Ctrl Pts',(-6.21212940551032,120.856246350173,
-8.55026260137164));
#282333=CARTESIAN_POINT('Ctrl Pts',(-8.13178296306933,121.006246350173,
-5.90808615117925));
#282334=CARTESIAN_POINT('Ctrl Pts',(-10.0514365206283,121.156246350172,
-3.26590970098687));
#282335=CARTESIAN_POINT('Ctrl Pts',(-10.0514365206283,121.306246350172,
2.46189191236404E-15));
#282336=CARTESIAN_POINT('Ctrl Pts',(-10.0514365206283,121.456246350171,
3.26590970098687));
#282337=CARTESIAN_POINT('Ctrl Pts',(-8.13178296306933,121.60624635017,5.90808615117926));
#282338=CARTESIAN_POINT('Ctrl Pts',(-6.21212940551032,121.75624635017,8.55026260137164));
#282339=CARTESIAN_POINT('Ctrl Pts',(-3.1060647027552,121.906246350169,9.55948420107058));
#282340=CARTESIAN_POINT('Ctrl Pts',(-8.08287531541503E-14,122.056246350169,
10.5687058007695));
#282341=CARTESIAN_POINT('Ctrl Pts',(3.10606470275504,122.206246350168,9.55948420107058));
#282342=CARTESIAN_POINT('Ctrl Pts',(6.21212940551016,122.356246350167,8.55026260137164));
#282343=CARTESIAN_POINT('Ctrl Pts',(8.13178296306916,122.506246350167,5.90808615117925));
#282344=CARTESIAN_POINT('Ctrl Pts',(10.0514365206282,122.656246350166,3.26590970098687));
#282345=CARTESIAN_POINT('Ctrl Pts',(10.0514365206282,122.806246350166,-1.23094595618202E-15));
#282346=CARTESIAN_POINT('Ctrl Pts',(10.0514365206282,122.956246350165,-3.26590970098687));
#282347=CARTESIAN_POINT('Ctrl Pts',(8.13178296306916,123.106246350164,-5.90808615117926));
#282348=CARTESIAN_POINT('Ctrl Pts',(6.21212940551016,123.256246350164,-8.55026260137164));
#282349=CARTESIAN_POINT('Ctrl Pts',(3.10606470275504,123.406246350163,-9.55948420107058));
#282350=CARTESIAN_POINT('Ctrl Pts',(-8.42811941359897E-14,123.556246350163,
-10.5687058007695));
#282351=CARTESIAN_POINT('Ctrl Pts',(-3.10606470275521,123.706246350162,
-9.55948420107058));
#282352=CARTESIAN_POINT('Ctrl Pts',(-6.21212940551032,123.856246350161,
-8.55026260137164));
#282353=CARTESIAN_POINT('Ctrl Pts',(-8.13178296306933,124.006246350161,
-5.90808615117925));
#282354=CARTESIAN_POINT('Ctrl Pts',(-10.0514365206283,124.15624635016,-3.26590970098687));
#282355=CARTESIAN_POINT('Ctrl Pts',(-10.0514365206283,124.30624635016,2.46189191236404E-15));
#282356=CARTESIAN_POINT('Ctrl Pts',(-10.0514365206283,124.456246350159,
3.26590970098687));
#282357=CARTESIAN_POINT('Ctrl Pts',(-8.13178296306933,124.606246350158,
5.90808615117926));
#282358=CARTESIAN_POINT('Ctrl Pts',(-6.21212940551032,124.756246350158,
8.55026260137164));
#282359=CARTESIAN_POINT('Ctrl Pts',(-3.1060647027552,124.906246350157,9.55948420107058));
#282360=CARTESIAN_POINT('Ctrl Pts',(-8.25564624258121E-14,125.056246350157,
10.5687058007695));
#282361=CARTESIAN_POINT('Ctrl Pts',(3.10606470275504,125.206246350156,9.55948420107058));
#282362=CARTESIAN_POINT('Ctrl Pts',(6.21212940551016,125.356246350155,8.55026260137164));
#282363=CARTESIAN_POINT('Ctrl Pts',(8.13178296306916,125.506246350155,5.90808615117925));
#282364=CARTESIAN_POINT('Ctrl Pts',(10.0514365206282,125.656246350154,3.26590970098687));
#282365=CARTESIAN_POINT('Ctrl Pts',(10.0514365206282,125.806246350154,-1.23094595618202E-15));
#282366=CARTESIAN_POINT('Ctrl Pts',(10.0514365206282,125.956246350153,-3.26590970098687));
#282367=CARTESIAN_POINT('Ctrl Pts',(8.13178296306916,126.106246350152,-5.90808615117926));
#282368=CARTESIAN_POINT('Ctrl Pts',(6.21212940551016,126.256246350152,-8.55026260137164));
#282369=CARTESIAN_POINT('Ctrl Pts',(3.10606470275503,126.406246350151,-9.55948420107058));
#282370=CARTESIAN_POINT('Ctrl Pts',(-8.60089034076516E-14,126.556246350151,
-10.5687058007695));
#282371=CARTESIAN_POINT('Ctrl Pts',(-3.10606470275521,126.70624635015,-9.55948420107058));
#282372=CARTESIAN_POINT('Ctrl Pts',(-6.21212940551033,126.856246350149,
-8.55026260137164));
#282373=CARTESIAN_POINT('Ctrl Pts',(-8.13178296306933,127.006246350149,
-5.90808615117925));
#282374=CARTESIAN_POINT('Ctrl Pts',(-10.0514365206283,127.156246350148,
-3.26590970098687));
#282375=CARTESIAN_POINT('Ctrl Pts',(-10.0514365206283,127.306246350148,
2.46189191236404E-15));
#282376=CARTESIAN_POINT('Ctrl Pts',(-10.0514365206283,127.456246350147,
3.26590970098687));
#282377=CARTESIAN_POINT('Ctrl Pts',(-8.13178296306933,127.606246350146,
5.90808615117926));
#282378=CARTESIAN_POINT('Ctrl Pts',(-6.21212940551032,127.756246350146,
8.55026260137164));
#282379=CARTESIAN_POINT('Ctrl Pts',(-3.10606470275521,127.906246350145,
9.55948420107058));
#282380=CARTESIAN_POINT('Ctrl Pts',(-8.4284171697474E-14,128.056246350145,
10.5687058007695));
#282381=CARTESIAN_POINT('Ctrl Pts',(3.10606470275504,128.206246350144,9.55948420107058));
#282382=CARTESIAN_POINT('Ctrl Pts',(6.21212940551016,128.356246350143,8.55026260137164));
#282383=CARTESIAN_POINT('Ctrl Pts',(8.13178296306916,128.506246350143,5.90808615117925));
#282384=CARTESIAN_POINT('Ctrl Pts',(10.0514365206282,128.656246350142,3.26590970098687));
#282385=CARTESIAN_POINT('Ctrl Pts',(10.0514365206282,128.806246350142,-1.23094595618202E-15));
#282386=CARTESIAN_POINT('Ctrl Pts',(10.0514365206282,128.956246350141,-3.26590970098687));
#282387=CARTESIAN_POINT('Ctrl Pts',(8.13178296306916,129.10624635014,-5.90808615117926));
#282388=CARTESIAN_POINT('Ctrl Pts',(6.21212940551015,129.25624635014,-8.55026260137164));
#282389=CARTESIAN_POINT('Ctrl Pts',(3.10606470275503,129.406246350139,-9.55948420107058));
#282390=CARTESIAN_POINT('Ctrl Pts',(-8.77366126793134E-14,129.556246350139,
-10.5687058007695));
#282391=CARTESIAN_POINT('Ctrl Pts',(-3.10606470275521,129.706246350138,
-9.55948420107058));
#282392=CARTESIAN_POINT('Ctrl Pts',(-6.21212940551033,129.856246350137,
-8.55026260137164));
#282393=CARTESIAN_POINT('Ctrl Pts',(-8.13178296306933,130.006246350137,
-5.90808615117925));
#282394=CARTESIAN_POINT('Ctrl Pts',(-10.0514365206283,130.156246350136,
-3.26590970098687));
#282395=CARTESIAN_POINT('Ctrl Pts',(-10.0514365206283,130.306246350136,
2.46189191236404E-15));
#282396=CARTESIAN_POINT('Ctrl Pts',(-10.0514365206283,130.456246350135,
3.26590970098687));
#282397=CARTESIAN_POINT('Ctrl Pts',(-8.13178296306933,130.606246350134,
5.90808615117926));
#282398=CARTESIAN_POINT('Ctrl Pts',(-6.21212940551033,130.756246350134,
8.55026260137164));
#282399=CARTESIAN_POINT('Ctrl Pts',(-3.10606470275521,130.906246350133,
9.55948420107058));
#282400=CARTESIAN_POINT('Ctrl Pts',(-8.60118809691358E-14,131.056246350133,
10.5687058007695));
#282401=CARTESIAN_POINT('Ctrl Pts',(3.10606470275503,131.206246350132,9.55948420107058));
#282402=CARTESIAN_POINT('Ctrl Pts',(6.21212940551016,131.356246350131,8.55026260137164));
#282403=CARTESIAN_POINT('Ctrl Pts',(8.13178296306916,131.506246350131,5.90808615117925));
#282404=CARTESIAN_POINT('Ctrl Pts',(10.0514365206282,131.65624635013,3.26590970098687));
#282405=CARTESIAN_POINT('Ctrl Pts',(10.0514365206282,131.80624635013,-1.23094595618202E-15));
#282406=CARTESIAN_POINT('Ctrl Pts',(10.0514365206282,131.956246350129,-3.26590970098687));
#282407=CARTESIAN_POINT('Ctrl Pts',(8.13178296306916,132.106246350128,-5.90808615117926));
#282408=CARTESIAN_POINT('Ctrl Pts',(6.21212940551015,132.256246350128,-8.55026260137164));
#282409=CARTESIAN_POINT('Ctrl Pts',(3.10606470275503,132.406246350127,-9.55948420107058));
#282410=CARTESIAN_POINT('Ctrl Pts',(-8.94643219509752E-14,132.556246350127,
-10.5687058007695));
#282411=CARTESIAN_POINT('Ctrl Pts',(-3.10606470275521,132.706246350126,
-9.55948420107058));
#282412=CARTESIAN_POINT('Ctrl Pts',(-6.21212940551033,132.856246350125,
-8.55026260137164));
#282413=CARTESIAN_POINT('Ctrl Pts',(-8.13178296306934,133.006246350125,
-5.90808615117925));
#282414=CARTESIAN_POINT('Ctrl Pts',(-10.0514365206283,133.156246350124,
-3.26590970098687));
#282415=CARTESIAN_POINT('Ctrl Pts',(-10.0514365206283,133.306246350124,
2.46189191236404E-15));
#282416=CARTESIAN_POINT('Ctrl Pts',(-10.0514365206283,133.456246350123,
3.26590970098687));
#282417=CARTESIAN_POINT('Ctrl Pts',(-8.13178296306934,133.606246350122,
5.90808615117926));
#282418=CARTESIAN_POINT('Ctrl Pts',(-6.21212940551033,133.756246350122,
8.55026260137164));
#282419=CARTESIAN_POINT('Ctrl Pts',(-3.10606470275521,133.906246350121,
9.55948420107058));
#282420=CARTESIAN_POINT('Ctrl Pts',(-8.77395902407977E-14,134.056246350121,
10.5687058007695));
#282421=CARTESIAN_POINT('Ctrl Pts',(3.10606470275503,134.20624635012,9.55948420107058));
#282422=CARTESIAN_POINT('Ctrl Pts',(6.21212940551015,134.356246350119,8.55026260137164));
#282423=CARTESIAN_POINT('Ctrl Pts',(8.13178296306915,134.506246350119,5.90808615117925));
#282424=CARTESIAN_POINT('Ctrl Pts',(10.0514365206282,134.656246350118,3.26590970098687));
#282425=CARTESIAN_POINT('Ctrl Pts',(10.0514365206282,134.806246350118,-1.23094595618202E-15));
#282426=CARTESIAN_POINT('Ctrl Pts',(10.0514365206282,134.956246350117,-3.26590970098687));
#282427=CARTESIAN_POINT('Ctrl Pts',(8.13178296306915,135.106246350116,-5.90808615117926));
#282428=CARTESIAN_POINT('Ctrl Pts',(6.21212940551015,135.256246350116,-8.55026260137164));
#282429=CARTESIAN_POINT('Ctrl Pts',(3.10606470275503,135.406246350115,-9.55948420107058));
#282430=CARTESIAN_POINT('Ctrl Pts',(-9.11920312226371E-14,135.556246350115,
-10.5687058007695));
#282431=CARTESIAN_POINT('Ctrl Pts',(-3.10606470275521,135.706246350114,
-9.55948420107058));
#282432=CARTESIAN_POINT('Ctrl Pts',(-6.21212940551033,135.856246350113,
-8.55026260137164));
#282433=CARTESIAN_POINT('Ctrl Pts',(-8.13178296306934,136.006246350113,
-5.90808615117925));
#282434=CARTESIAN_POINT('Ctrl Pts',(-10.0514365206283,136.156246350112,
-3.26590970098687));
#282435=CARTESIAN_POINT('Ctrl Pts',(-10.0514365206283,136.306246350112,
2.46189191236404E-15));
#282436=CARTESIAN_POINT('Ctrl Pts',(-10.0514365206283,136.456246350111,
3.26590970098687));
#282437=CARTESIAN_POINT('Ctrl Pts',(-8.13178296306934,136.60624635011,5.90808615117926));
#282438=CARTESIAN_POINT('Ctrl Pts',(-6.21212940551033,136.75624635011,8.55026260137164));
#282439=CARTESIAN_POINT('Ctrl Pts',(-3.10606470275521,136.906246350109,
9.55948420107058));
#282440=CARTESIAN_POINT('Ctrl Pts',(-8.94672995124595E-14,137.056246350109,
10.5687058007695));
#282441=CARTESIAN_POINT('Ctrl Pts',(3.10606470275503,137.206246350108,9.55948420107058));
#282442=CARTESIAN_POINT('Ctrl Pts',(6.21212940551015,137.356246350107,8.55026260137164));
#282443=CARTESIAN_POINT('Ctrl Pts',(8.13178296306915,137.506246350107,5.90808615117925));
#282444=CARTESIAN_POINT('Ctrl Pts',(10.0514365206282,137.656246350106,3.26590970098687));
#282445=CARTESIAN_POINT('Ctrl Pts',(10.0514365206282,137.806246350106,-1.23094595618202E-15));
#282446=CARTESIAN_POINT('Ctrl Pts',(10.0514365206282,137.956246350105,-3.26590970098687));
#282447=CARTESIAN_POINT('Ctrl Pts',(8.13178296306915,138.106246350104,-5.90808615117926));
#282448=CARTESIAN_POINT('Ctrl Pts',(6.21212940551015,138.256246350104,-8.55026260137164));
#282449=CARTESIAN_POINT('Ctrl Pts',(3.10606470275503,138.406246350103,-9.55948420107058));
#282450=CARTESIAN_POINT('Ctrl Pts',(-9.29197404942989E-14,138.556246350103,
-10.5687058007695));
#282451=CARTESIAN_POINT('Ctrl Pts',(-3.10606470275521,138.706246350102,
-9.55948420107058));
#282452=CARTESIAN_POINT('Ctrl Pts',(-6.21212940551033,138.856246350101,
-8.55026260137164));
#282453=CARTESIAN_POINT('Ctrl Pts',(-8.13178296306934,139.006246350101,
-5.90808615117925));
#282454=CARTESIAN_POINT('Ctrl Pts',(-10.0514365206283,139.1562463501,-3.26590970098687));
#282455=CARTESIAN_POINT('Ctrl Pts',(-10.0514365206283,139.3062463501,2.46189191236404E-15));
#282456=CARTESIAN_POINT('Ctrl Pts',(-10.0514365206283,139.456246350099,
3.26590970098687));
#282457=CARTESIAN_POINT('Ctrl Pts',(-8.13178296306934,139.606246350098,
5.90808615117926));
#282458=CARTESIAN_POINT('Ctrl Pts',(-6.21212940551033,139.756246350098,
8.55026260137164));
#282459=CARTESIAN_POINT('Ctrl Pts',(-3.10606470275521,139.906246350097,
9.55948420107058));
#282460=CARTESIAN_POINT('Ctrl Pts',(-9.11950087841213E-14,140.056246350097,
10.5687058007695));
#282461=CARTESIAN_POINT('Ctrl Pts',(3.10606470275503,140.206246350096,9.55948420107058));
#282462=CARTESIAN_POINT('Ctrl Pts',(6.21212940551015,140.356246350095,8.55026260137164));
#282463=CARTESIAN_POINT('Ctrl Pts',(8.13178296306915,140.506246350095,5.90808615117925));
#282464=CARTESIAN_POINT('Ctrl Pts',(10.0514365206282,140.656246350094,3.26590970098687));
#282465=CARTESIAN_POINT('Ctrl Pts',(10.0514365206282,140.806246350094,-1.23094595618202E-15));
#282466=CARTESIAN_POINT('Ctrl Pts',(10.0514365206282,140.956246350093,-3.26590970098687));
#282467=CARTESIAN_POINT('Ctrl Pts',(8.13178296306915,141.106246350092,-5.90808615117926));
#282468=CARTESIAN_POINT('Ctrl Pts',(6.21212940551015,141.256246350092,-8.55026260137164));
#282469=CARTESIAN_POINT('Ctrl Pts',(3.10606470275503,141.406246350091,-9.55948420107058));
#282470=CARTESIAN_POINT('Ctrl Pts',(-9.46474497659607E-14,141.556246350091,
-10.5687058007695));
#282471=CARTESIAN_POINT('Ctrl Pts',(-3.10606470275522,141.70624635009,-9.55948420107058));
#282472=CARTESIAN_POINT('Ctrl Pts',(-6.21212940551034,141.856246350089,
-8.55026260137164));
#282473=CARTESIAN_POINT('Ctrl Pts',(-8.13178296306934,142.006246350089,
-5.90808615117925));
#282474=CARTESIAN_POINT('Ctrl Pts',(-10.0514365206283,142.156246350088,
-3.26590970098687));
#282475=CARTESIAN_POINT('Ctrl Pts',(-10.0514365206283,142.306246350088,
2.46189191236404E-15));
#282476=CARTESIAN_POINT('Ctrl Pts',(-10.0514365206283,142.456246350087,
3.26590970098687));
#282477=CARTESIAN_POINT('Ctrl Pts',(-8.13178296306934,142.606246350086,
5.90808615117926));
#282478=CARTESIAN_POINT('Ctrl Pts',(-6.21212940551033,142.756246350086,
8.55026260137164));
#282479=CARTESIAN_POINT('Ctrl Pts',(-3.10606470275521,142.906246350085,
9.55948420107058));
#282480=CARTESIAN_POINT('Ctrl Pts',(-9.29227180557832E-14,143.056246350085,
10.5687058007695));
#282481=CARTESIAN_POINT('Ctrl Pts',(3.10606470275503,143.206246350084,9.55948420107058));
#282482=CARTESIAN_POINT('Ctrl Pts',(6.21212940551015,143.356246350083,8.55026260137164));
#282483=CARTESIAN_POINT('Ctrl Pts',(8.13178296306915,143.506246350083,5.90808615117925));
#282484=CARTESIAN_POINT('Ctrl Pts',(10.0514365206282,143.656246350082,3.26590970098687));
#282485=CARTESIAN_POINT('Ctrl Pts',(10.0514365206282,143.806246350082,-1.23094595618202E-15));
#282486=CARTESIAN_POINT('Ctrl Pts',(10.0514365206282,143.956246350081,-3.26590970098687));
#282487=CARTESIAN_POINT('Ctrl Pts',(8.13178296306915,144.10624635008,-5.90808615117926));
#282488=CARTESIAN_POINT('Ctrl Pts',(6.21212940551015,144.25624635008,-8.55026260137164));
#282489=CARTESIAN_POINT('Ctrl Pts',(3.10606470275502,144.406246350079,-9.55948420107058));
#282490=CARTESIAN_POINT('Ctrl Pts',(-9.63751590376226E-14,144.556246350079,
-10.5687058007695));
#282491=CARTESIAN_POINT('Ctrl Pts',(-3.10606470275522,144.706246350078,
-9.55948420107058));
#282492=CARTESIAN_POINT('Ctrl Pts',(-6.21212940551034,144.856246350077,
-8.55026260137164));
#282493=CARTESIAN_POINT('Ctrl Pts',(-8.13178296306934,145.006246350077,
-5.90808615117925));
#282494=CARTESIAN_POINT('Ctrl Pts',(-10.0514365206283,145.156246350076,
-3.26590970098687));
#282495=CARTESIAN_POINT('Ctrl Pts',(-10.0514365206283,145.306246350076,
2.46189191236404E-15));
#282496=CARTESIAN_POINT('Ctrl Pts',(-10.0514365206283,145.456246350075,
3.26590970098687));
#282497=CARTESIAN_POINT('Ctrl Pts',(-8.13178296306934,145.606246350074,
5.90808615117926));
#282498=CARTESIAN_POINT('Ctrl Pts',(-6.21212940551034,145.756246350074,
8.55026260137164));
#282499=CARTESIAN_POINT('Ctrl Pts',(-3.10606470275522,145.906246350073,
9.55948420107058));
#282500=CARTESIAN_POINT('Ctrl Pts',(-9.4650427327445E-14,146.056246350073,
10.5687058007695));
#282501=CARTESIAN_POINT('Ctrl Pts',(3.10606470275503,146.206246350072,9.55948420107058));
#282502=CARTESIAN_POINT('Ctrl Pts',(6.21212940551015,146.356246350071,8.55026260137164));
#282503=CARTESIAN_POINT('Ctrl Pts',(8.13178296306915,146.506246350071,5.90808615117925));
#282504=CARTESIAN_POINT('Ctrl Pts',(10.0514365206282,146.65624635007,3.26590970098687));
#282505=CARTESIAN_POINT('Ctrl Pts',(10.0514365206281,146.80624635007,-1.23094595618202E-15));
#282506=CARTESIAN_POINT('Ctrl Pts',(10.0514365206282,146.956246350069,-3.26590970098687));
#282507=CARTESIAN_POINT('Ctrl Pts',(8.13178296306915,147.106246350068,-5.90808615117926));
#282508=CARTESIAN_POINT('Ctrl Pts',(6.21212940551014,147.256246350068,-8.55026260137164));
#282509=CARTESIAN_POINT('Ctrl Pts',(3.10606470275502,147.406246350067,-9.55948420107058));
#282510=CARTESIAN_POINT('Ctrl Pts',(-9.81028683092844E-14,147.556246350067,
-10.5687058007695));
#282511=CARTESIAN_POINT('Ctrl Pts',(-3.10606470275522,147.706246350066,
-9.55948420107058));
#282512=CARTESIAN_POINT('Ctrl Pts',(-6.21212940551034,147.856246350065,
-8.55026260137164));
#282513=CARTESIAN_POINT('Ctrl Pts',(-8.13178296306934,148.006246350065,
-5.90808615117925));
#282514=CARTESIAN_POINT('Ctrl Pts',(-10.0514365206283,148.156246350064,
-3.26590970098687));
#282515=CARTESIAN_POINT('Ctrl Pts',(-10.0514365206283,148.306246350064,
2.46189191236404E-15));
#282516=CARTESIAN_POINT('Ctrl Pts',(-10.0514365206283,148.456246350063,
3.26590970098687));
#282517=CARTESIAN_POINT('Ctrl Pts',(-8.13178296306934,148.606246350062,
5.90808615117926));
#282518=CARTESIAN_POINT('Ctrl Pts',(-6.21212940551034,148.756246350062,
8.55026260137164));
#282519=CARTESIAN_POINT('Ctrl Pts',(-3.10606470275522,148.906246350061,
9.55948420107058));
#282520=CARTESIAN_POINT('Ctrl Pts',(-9.63781365991068E-14,149.056246350061,
10.5687058007695));
#282521=CARTESIAN_POINT('Ctrl Pts',(3.10606470275502,149.20624635006,9.55948420107058));
#282522=CARTESIAN_POINT('Ctrl Pts',(6.21212940551015,149.356246350059,8.55026260137164));
#282523=CARTESIAN_POINT('Ctrl Pts',(8.13178296306915,149.506246350059,5.90808615117925));
#282524=CARTESIAN_POINT('Ctrl Pts',(10.0514365206282,149.656246350058,3.26590970098687));
#282525=CARTESIAN_POINT('Ctrl Pts',(10.0514365206281,149.806246350058,-1.23094595618202E-15));
#282526=CARTESIAN_POINT('Ctrl Pts',(10.0514365206281,149.956246350057,-3.26590970098687));
#282527=CARTESIAN_POINT('Ctrl Pts',(8.13178296306915,150.106246350056,-5.90808615117926));
#282528=CARTESIAN_POINT('Ctrl Pts',(6.21212940551014,150.256246350056,-8.55026260137164));
#282529=CARTESIAN_POINT('Ctrl Pts',(3.10606470275502,150.406246350055,-9.55948420107058));
#282530=CARTESIAN_POINT('Ctrl Pts',(-9.98305775809463E-14,150.556246350055,
-10.5687058007695));
#282531=CARTESIAN_POINT('Ctrl Pts',(-3.10606470275522,150.706246350054,
-9.55948420107058));
#282532=CARTESIAN_POINT('Ctrl Pts',(-6.21212940551034,150.856246350053,
-8.55026260137164));
#282533=CARTESIAN_POINT('Ctrl Pts',(-8.13178296306935,151.006246350053,
-5.90808615117925));
#282534=CARTESIAN_POINT('Ctrl Pts',(-10.0514365206283,151.156246350052,
-3.26590970098687));
#282535=CARTESIAN_POINT('Ctrl Pts',(-10.0514365206284,151.306246350052,
2.46189191236404E-15));
#282536=CARTESIAN_POINT('Ctrl Pts',(-10.0514365206283,151.456246350051,
3.26590970098687));
#282537=CARTESIAN_POINT('Ctrl Pts',(-8.13178296306935,151.60624635005,5.90808615117926));
#282538=CARTESIAN_POINT('Ctrl Pts',(-6.21212940551034,151.75624635005,8.55026260137164));
#282539=CARTESIAN_POINT('Ctrl Pts',(-3.10606470275522,151.906246350049,
9.55948420107058));
#282540=CARTESIAN_POINT('Ctrl Pts',(-9.81058458707687E-14,152.056246350049,
10.5687058007695));
#282541=CARTESIAN_POINT('Ctrl Pts',(3.10606470275502,152.206246350048,9.55948420107058));
#282542=CARTESIAN_POINT('Ctrl Pts',(6.21212940551014,152.356246350047,8.55026260137164));
#282543=CARTESIAN_POINT('Ctrl Pts',(8.13178296306915,152.506246350047,5.90808615117925));
#282544=CARTESIAN_POINT('Ctrl Pts',(10.0514365206281,152.656246350046,3.26590970098687));
#282545=CARTESIAN_POINT('Ctrl Pts',(10.0514365206281,152.806246350046,-1.23094595618202E-15));
#282546=CARTESIAN_POINT('Ctrl Pts',(10.0514365206281,152.956246350045,-3.26590970098687));
#282547=CARTESIAN_POINT('Ctrl Pts',(8.13178296306915,153.106246350044,-5.90808615117926));
#282548=CARTESIAN_POINT('Ctrl Pts',(6.21212940551014,153.256246350044,-8.55026260137164));
#282549=CARTESIAN_POINT('Ctrl Pts',(3.10606470275502,153.406246350043,-9.55948420107058));
#282550=CARTESIAN_POINT('Ctrl Pts',(-1.01558286852608E-13,153.556246350043,
-10.5687058007695));
#282551=CARTESIAN_POINT('Ctrl Pts',(-3.10606470275522,153.706246350042,
-9.55948420107058));
#282552=CARTESIAN_POINT('Ctrl Pts',(-12.1623797632097,-0.474999999988005,
2.97892388940585E-15));
#282553=CARTESIAN_POINT('Ctrl Pts',(-12.1623797632096,-0.324999999988605,
3.95179673813133));
#282554=CARTESIAN_POINT('Ctrl Pts',(-9.83957192047856,-0.174999999989203,
7.14886745759505));
#282555=CARTESIAN_POINT('Ctrl Pts',(-7.51676407774747,-0.0249999999898023,
10.3459381770588));
#282556=CARTESIAN_POINT('Ctrl Pts',(-3.75838203887374,0.1250000000096,11.5671105274568));
#282557=CARTESIAN_POINT('Ctrl Pts',(-1.02868273148643E-14,0.275000000009002,
12.7882828778549));
#282558=CARTESIAN_POINT('Ctrl Pts',(3.75838203887372,0.425000000008404,
11.5671105274568));
#282559=CARTESIAN_POINT('Ctrl Pts',(7.51676407774745,0.575000000007806,
10.3459381770588));
#282560=CARTESIAN_POINT('Ctrl Pts',(9.83957192047854,0.725000000007208,
7.14886745759505));
#282561=CARTESIAN_POINT('Ctrl Pts',(12.1623797632096,0.875000000006609,
3.95179673813132));
#282562=CARTESIAN_POINT('Ctrl Pts',(12.1623797632096,1.02500000000601,-1.48946194470292E-15));
#282563=CARTESIAN_POINT('Ctrl Pts',(12.1623797632096,1.17500000000541,-3.95179673813132));
#282564=CARTESIAN_POINT('Ctrl Pts',(9.83957192047853,1.32500000000481,-7.14886745759505));
#282565=CARTESIAN_POINT('Ctrl Pts',(7.51676407774744,1.47500000000421,-10.3459381770588));
#282566=CARTESIAN_POINT('Ctrl Pts',(3.75838203887371,1.6250000000036,-11.5671105274568));
#282567=CARTESIAN_POINT('Ctrl Pts',(-1.42829078892864E-14,1.775000000003,
-12.7882828778549));
#282568=CARTESIAN_POINT('Ctrl Pts',(-3.75838203887374,1.9250000000024,-11.5671105274568));
#282569=CARTESIAN_POINT('Ctrl Pts',(-7.51676407774747,2.0750000000018,-10.3459381770588));
#282570=CARTESIAN_POINT('Ctrl Pts',(-9.83957192047856,2.2250000000012,-7.14886745759505));
#282571=CARTESIAN_POINT('Ctrl Pts',(-12.1623797632097,2.37500000000059,
-3.95179673813132));
#282572=CARTESIAN_POINT('Ctrl Pts',(-12.1623797632097,2.525,2.97892388940585E-15));
#282573=CARTESIAN_POINT('Ctrl Pts',(-12.1623797632097,2.6749999999994,3.95179673813133));
#282574=CARTESIAN_POINT('Ctrl Pts',(-9.83957192047856,2.8249999999988,7.14886745759505));
#282575=CARTESIAN_POINT('Ctrl Pts',(-7.51676407774747,2.9749999999982,10.3459381770588));
#282576=CARTESIAN_POINT('Ctrl Pts',(-3.75838203887374,3.1249999999976,11.5671105274568));
#282577=CARTESIAN_POINT('Ctrl Pts',(-1.20145365865262E-14,3.274999999997,
12.7882828778549));
#282578=CARTESIAN_POINT('Ctrl Pts',(3.75838203887372,3.4249999999964,11.5671105274568));
#282579=CARTESIAN_POINT('Ctrl Pts',(7.51676407774744,3.57499999999581,10.3459381770588));
#282580=CARTESIAN_POINT('Ctrl Pts',(9.83957192047853,3.72499999999521,7.14886745759505));
#282581=CARTESIAN_POINT('Ctrl Pts',(12.1623797632096,3.87499999999461,3.95179673813132));
#282582=CARTESIAN_POINT('Ctrl Pts',(12.1623797632096,4.02499999999401,-1.48946194470292E-15));
#282583=CARTESIAN_POINT('Ctrl Pts',(12.1623797632096,4.17499999999341,-3.95179673813132));
#282584=CARTESIAN_POINT('Ctrl Pts',(9.83957192047853,4.32499999999281,-7.14886745759505));
#282585=CARTESIAN_POINT('Ctrl Pts',(7.51676407774744,4.47499999999221,-10.3459381770588));
#282586=CARTESIAN_POINT('Ctrl Pts',(3.75838203887371,4.6249999999916,-11.5671105274568));
#282587=CARTESIAN_POINT('Ctrl Pts',(-1.60106171609483E-14,4.774999999991,
-12.7882828778549));
#282588=CARTESIAN_POINT('Ctrl Pts',(-3.75838203887374,4.9249999999904,-11.5671105274568));
#282589=CARTESIAN_POINT('Ctrl Pts',(-7.51676407774747,5.0749999999898,-10.3459381770588));
#282590=CARTESIAN_POINT('Ctrl Pts',(-9.83957192047857,5.2249999999892,-7.14886745759505));
#282591=CARTESIAN_POINT('Ctrl Pts',(-12.1623797632097,5.3749999999886,-3.95179673813132));
#282592=CARTESIAN_POINT('Ctrl Pts',(-12.1623797632097,5.52499999998799,
2.97892388940585E-15));
#282593=CARTESIAN_POINT('Ctrl Pts',(-12.1623797632097,5.67499999998739,
3.95179673813133));
#282594=CARTESIAN_POINT('Ctrl Pts',(-9.83957192047857,5.8249999999868,7.14886745759505));
#282595=CARTESIAN_POINT('Ctrl Pts',(-7.51676407774747,5.9749999999862,10.3459381770588));
#282596=CARTESIAN_POINT('Ctrl Pts',(-3.75838203887374,6.1249999999856,11.5671105274568));
#282597=CARTESIAN_POINT('Ctrl Pts',(-1.3742245858188E-14,6.274999999985,
12.7882828778549));
#282598=CARTESIAN_POINT('Ctrl Pts',(3.75838203887371,6.4249999999844,11.5671105274568));
#282599=CARTESIAN_POINT('Ctrl Pts',(7.51676407774744,6.57499999998381,10.3459381770588));
#282600=CARTESIAN_POINT('Ctrl Pts',(9.83957192047853,6.72499999998321,7.14886745759505));
#282601=CARTESIAN_POINT('Ctrl Pts',(12.1623797632096,6.87499999998261,3.95179673813132));
#282602=CARTESIAN_POINT('Ctrl Pts',(12.1623797632096,7.02499999998201,-1.48946194470292E-15));
#282603=CARTESIAN_POINT('Ctrl Pts',(12.1623797632096,7.17499999998141,-3.95179673813132));
#282604=CARTESIAN_POINT('Ctrl Pts',(9.83957192047853,7.32499999998081,-7.14886745759505));
#282605=CARTESIAN_POINT('Ctrl Pts',(7.51676407774744,7.47499999998021,-10.3459381770588));
#282606=CARTESIAN_POINT('Ctrl Pts',(3.75838203887371,7.6249999999796,-11.5671105274568));
#282607=CARTESIAN_POINT('Ctrl Pts',(-1.77383264326101E-14,7.774999999979,
-12.7882828778549));
#282608=CARTESIAN_POINT('Ctrl Pts',(-3.75838203887375,7.9249999999784,-11.5671105274568));
#282609=CARTESIAN_POINT('Ctrl Pts',(-7.51676407774747,8.0749999999778,-10.3459381770588));
#282610=CARTESIAN_POINT('Ctrl Pts',(-9.83957192047857,8.2249999999772,-7.14886745759505));
#282611=CARTESIAN_POINT('Ctrl Pts',(-12.1623797632097,8.3749999999766,-3.95179673813132));
#282612=CARTESIAN_POINT('Ctrl Pts',(-12.1623797632097,8.52499999997599,
2.97892388940585E-15));
#282613=CARTESIAN_POINT('Ctrl Pts',(-12.1623797632097,8.6749999999754,3.95179673813133));
#282614=CARTESIAN_POINT('Ctrl Pts',(-9.83957192047857,8.8249999999748,7.14886745759505));
#282615=CARTESIAN_POINT('Ctrl Pts',(-7.51676407774747,8.9749999999742,10.3459381770588));
#282616=CARTESIAN_POINT('Ctrl Pts',(-3.75838203887374,9.1249999999736,11.5671105274568));
#282617=CARTESIAN_POINT('Ctrl Pts',(-1.54699551298498E-14,9.274999999973,
12.7882828778549));
#282618=CARTESIAN_POINT('Ctrl Pts',(3.75838203887371,9.4249999999724,11.5671105274568));
#282619=CARTESIAN_POINT('Ctrl Pts',(7.51676407774744,9.57499999997181,10.3459381770588));
#282620=CARTESIAN_POINT('Ctrl Pts',(9.83957192047853,9.72499999997121,7.14886745759505));
#282621=CARTESIAN_POINT('Ctrl Pts',(12.1623797632096,9.87499999997061,3.95179673813132));
#282622=CARTESIAN_POINT('Ctrl Pts',(12.1623797632096,10.02499999997,-1.48946194470292E-15));
#282623=CARTESIAN_POINT('Ctrl Pts',(12.1623797632096,10.1749999999694,-3.95179673813132));
#282624=CARTESIAN_POINT('Ctrl Pts',(9.83957192047853,10.3249999999688,-7.14886745759505));
#282625=CARTESIAN_POINT('Ctrl Pts',(7.51676407774744,10.4749999999682,-10.3459381770588));
#282626=CARTESIAN_POINT('Ctrl Pts',(3.75838203887371,10.6249999999676,-11.5671105274568));
#282627=CARTESIAN_POINT('Ctrl Pts',(-1.9466035704272E-14,10.774999999967,
-12.7882828778549));
#282628=CARTESIAN_POINT('Ctrl Pts',(-3.75838203887375,10.9249999999664,
-11.5671105274568));
#282629=CARTESIAN_POINT('Ctrl Pts',(-7.51676407774748,11.0749999999658,
-10.3459381770588));
#282630=CARTESIAN_POINT('Ctrl Pts',(-9.83957192047857,11.2249999999652,
-7.14886745759505));
#282631=CARTESIAN_POINT('Ctrl Pts',(-12.1623797632097,11.3749999999646,
-3.95179673813132));
#282632=CARTESIAN_POINT('Ctrl Pts',(-12.1623797632097,11.524999999964,2.97892388940585E-15));
#282633=CARTESIAN_POINT('Ctrl Pts',(-12.1623797632097,11.6749999999634,
3.95179673813133));
#282634=CARTESIAN_POINT('Ctrl Pts',(-9.83957192047857,11.8249999999628,
7.14886745759505));
#282635=CARTESIAN_POINT('Ctrl Pts',(-7.51676407774747,11.9749999999622,
10.3459381770588));
#282636=CARTESIAN_POINT('Ctrl Pts',(-3.75838203887375,12.1249999999616,
11.5671105274568));
#282637=CARTESIAN_POINT('Ctrl Pts',(-1.71976644015117E-14,12.274999999961,
12.7882828778549));
#282638=CARTESIAN_POINT('Ctrl Pts',(3.75838203887371,12.4249999999604,11.5671105274568));
#282639=CARTESIAN_POINT('Ctrl Pts',(7.51676407774744,12.5749999999598,10.3459381770588));
#282640=CARTESIAN_POINT('Ctrl Pts',(9.83957192047853,12.7249999999592,7.14886745759505));
#282641=CARTESIAN_POINT('Ctrl Pts',(12.1623797632096,12.8749999999586,3.95179673813132));
#282642=CARTESIAN_POINT('Ctrl Pts',(12.1623797632096,13.024999999958,-1.48946194470292E-15));
#282643=CARTESIAN_POINT('Ctrl Pts',(12.1623797632096,13.1749999999574,-3.95179673813132));
#282644=CARTESIAN_POINT('Ctrl Pts',(9.83957192047853,13.3249999999568,-7.14886745759505));
#282645=CARTESIAN_POINT('Ctrl Pts',(7.51676407774743,13.4749999999562,-10.3459381770588));
#282646=CARTESIAN_POINT('Ctrl Pts',(3.75838203887371,13.6249999999556,-11.5671105274568));
#282647=CARTESIAN_POINT('Ctrl Pts',(-2.11937449759338E-14,13.774999999955,
-12.7882828778549));
#282648=CARTESIAN_POINT('Ctrl Pts',(-3.75838203887375,13.9249999999544,
-11.5671105274568));
#282649=CARTESIAN_POINT('Ctrl Pts',(-7.51676407774748,14.0749999999538,
-10.3459381770588));
#282650=CARTESIAN_POINT('Ctrl Pts',(-9.83957192047857,14.2249999999532,
-7.14886745759505));
#282651=CARTESIAN_POINT('Ctrl Pts',(-12.1623797632097,14.3749999999526,
-3.95179673813132));
#282652=CARTESIAN_POINT('Ctrl Pts',(-12.1623797632097,14.524999999952,2.97892388940585E-15));
#282653=CARTESIAN_POINT('Ctrl Pts',(-12.1623797632097,14.6749999999514,
3.95179673813133));
#282654=CARTESIAN_POINT('Ctrl Pts',(-9.83957192047857,14.8249999999508,
7.14886745759505));
#282655=CARTESIAN_POINT('Ctrl Pts',(-7.51676407774747,14.9749999999502,
10.3459381770588));
#282656=CARTESIAN_POINT('Ctrl Pts',(-3.75838203887375,15.1249999999496,
11.5671105274568));
#282657=CARTESIAN_POINT('Ctrl Pts',(-1.89253736731735E-14,15.274999999949,
12.7882828778549));
#282658=CARTESIAN_POINT('Ctrl Pts',(3.75838203887371,15.4249999999484,11.5671105274568));
#282659=CARTESIAN_POINT('Ctrl Pts',(7.51676407774744,15.5749999999478,10.3459381770588));
#282660=CARTESIAN_POINT('Ctrl Pts',(9.83957192047853,15.7249999999472,7.14886745759505));
#282661=CARTESIAN_POINT('Ctrl Pts',(12.1623797632096,15.8749999999466,3.95179673813132));
#282662=CARTESIAN_POINT('Ctrl Pts',(12.1623797632096,16.024999999946,-1.48946194470292E-15));
#282663=CARTESIAN_POINT('Ctrl Pts',(12.1623797632096,16.1749999999454,-3.95179673813132));
#282664=CARTESIAN_POINT('Ctrl Pts',(9.83957192047852,16.3249999999448,-7.14886745759505));
#282665=CARTESIAN_POINT('Ctrl Pts',(7.51676407774743,16.4749999999442,-10.3459381770588));
#282666=CARTESIAN_POINT('Ctrl Pts',(3.7583820388737,16.6249999999436,-11.5671105274568));
#282667=CARTESIAN_POINT('Ctrl Pts',(-2.29214542475956E-14,16.774999999943,
-12.7882828778549));
#282668=CARTESIAN_POINT('Ctrl Pts',(-3.75838203887375,16.9249999999424,
-11.5671105274568));
#282669=CARTESIAN_POINT('Ctrl Pts',(-7.51676407774748,17.0749999999418,
-10.3459381770588));
#282670=CARTESIAN_POINT('Ctrl Pts',(-9.83957192047857,17.2249999999412,
-7.14886745759505));
#282671=CARTESIAN_POINT('Ctrl Pts',(-12.1623797632097,17.3749999999406,
-3.95179673813132));
#282672=CARTESIAN_POINT('Ctrl Pts',(-12.1623797632097,17.52499999994,2.97892388940585E-15));
#282673=CARTESIAN_POINT('Ctrl Pts',(-12.1623797632097,17.6749999999394,
3.95179673813133));
#282674=CARTESIAN_POINT('Ctrl Pts',(-9.83957192047857,17.8249999999388,
7.14886745759505));
#282675=CARTESIAN_POINT('Ctrl Pts',(-7.51676407774748,17.9749999999382,
10.3459381770588));
#282676=CARTESIAN_POINT('Ctrl Pts',(-3.75838203887375,18.1249999999376,
11.5671105274568));
#282677=CARTESIAN_POINT('Ctrl Pts',(-2.06530829448354E-14,18.274999999937,
12.7882828778549));
#282678=CARTESIAN_POINT('Ctrl Pts',(3.75838203887371,18.4249999999364,11.5671105274568));
#282679=CARTESIAN_POINT('Ctrl Pts',(7.51676407774743,18.5749999999358,10.3459381770588));
#282680=CARTESIAN_POINT('Ctrl Pts',(9.83957192047852,18.7249999999352,7.14886745759505));
#282681=CARTESIAN_POINT('Ctrl Pts',(12.1623797632096,18.8749999999346,3.95179673813132));
#282682=CARTESIAN_POINT('Ctrl Pts',(12.1623797632096,19.024999999934,-1.48946194470292E-15));
#282683=CARTESIAN_POINT('Ctrl Pts',(12.1623797632096,19.1749999999334,-3.95179673813132));
#282684=CARTESIAN_POINT('Ctrl Pts',(9.83957192047852,19.3249999999328,-7.14886745759505));
#282685=CARTESIAN_POINT('Ctrl Pts',(7.51676407774743,19.4749999999322,-10.3459381770588));
#282686=CARTESIAN_POINT('Ctrl Pts',(3.7583820388737,19.6249999999316,-11.5671105274568));
#282687=CARTESIAN_POINT('Ctrl Pts',(-2.46491635192575E-14,19.774999999931,
-12.7882828778549));
#282688=CARTESIAN_POINT('Ctrl Pts',(-3.75838203887375,19.9249999999304,
-11.5671105274568));
#282689=CARTESIAN_POINT('Ctrl Pts',(-7.51676407774748,20.0749999999298,
-10.3459381770588));
#282690=CARTESIAN_POINT('Ctrl Pts',(-9.83957192047857,20.2249999999292,
-7.14886745759505));
#282691=CARTESIAN_POINT('Ctrl Pts',(-12.1623797632097,20.3749999999286,
-3.95179673813132));
#282692=CARTESIAN_POINT('Ctrl Pts',(-12.1623797632097,20.524999999928,2.97892388940585E-15));
#282693=CARTESIAN_POINT('Ctrl Pts',(-12.1623797632097,20.6749999999274,
3.95179673813133));
#282694=CARTESIAN_POINT('Ctrl Pts',(-9.83957192047857,20.8249999999268,
7.14886745759505));
#282695=CARTESIAN_POINT('Ctrl Pts',(-7.51676407774748,20.9749999999262,
10.3459381770588));
#282696=CARTESIAN_POINT('Ctrl Pts',(-3.75838203887375,21.1249999999256,
11.5671105274568));
#282697=CARTESIAN_POINT('Ctrl Pts',(-2.23807922164972E-14,21.274999999925,
12.7882828778549));
#282698=CARTESIAN_POINT('Ctrl Pts',(3.7583820388737,21.4249999999244,11.5671105274568));
#282699=CARTESIAN_POINT('Ctrl Pts',(7.51676407774743,21.5749999999238,10.3459381770588));
#282700=CARTESIAN_POINT('Ctrl Pts',(9.83957192047852,21.7249999999232,7.14886745759505));
#282701=CARTESIAN_POINT('Ctrl Pts',(12.1623797632096,21.8749999999226,3.95179673813132));
#282702=CARTESIAN_POINT('Ctrl Pts',(12.1623797632096,22.024999999922,-1.48946194470292E-15));
#282703=CARTESIAN_POINT('Ctrl Pts',(12.1623797632096,22.1749999999214,-3.95179673813132));
#282704=CARTESIAN_POINT('Ctrl Pts',(9.83957192047852,22.3249999999208,-7.14886745759505));
#282705=CARTESIAN_POINT('Ctrl Pts',(7.51676407774743,22.4749999999202,-10.3459381770588));
#282706=CARTESIAN_POINT('Ctrl Pts',(3.7583820388737,22.6249999999196,-11.5671105274568));
#282707=CARTESIAN_POINT('Ctrl Pts',(-2.63768727909193E-14,22.774999999919,
-12.7882828778549));
#282708=CARTESIAN_POINT('Ctrl Pts',(-3.75838203887375,22.9249999999184,
-11.5671105274568));
#282709=CARTESIAN_POINT('Ctrl Pts',(-7.51676407774748,23.0749999999178,
-10.3459381770588));
#282710=CARTESIAN_POINT('Ctrl Pts',(-9.83957192047857,23.2249999999172,
-7.14886745759505));
#282711=CARTESIAN_POINT('Ctrl Pts',(-12.1623797632097,23.3749999999166,
-3.95179673813132));
#282712=CARTESIAN_POINT('Ctrl Pts',(-12.1623797632097,23.524999999916,2.97892388940585E-15));
#282713=CARTESIAN_POINT('Ctrl Pts',(-12.1623797632097,23.6749999999154,
3.95179673813133));
#282714=CARTESIAN_POINT('Ctrl Pts',(-9.83957192047857,23.8249999999148,
7.14886745759505));
#282715=CARTESIAN_POINT('Ctrl Pts',(-7.51676407774748,23.9749999999142,
10.3459381770588));
#282716=CARTESIAN_POINT('Ctrl Pts',(-3.75838203887375,24.1249999999136,
11.5671105274568));
#282717=CARTESIAN_POINT('Ctrl Pts',(-2.4108501488159E-14,24.274999999913,
12.7882828778549));
#282718=CARTESIAN_POINT('Ctrl Pts',(3.7583820388737,24.4249999999124,11.5671105274568));
#282719=CARTESIAN_POINT('Ctrl Pts',(7.51676407774743,24.5749999999118,10.3459381770588));
#282720=CARTESIAN_POINT('Ctrl Pts',(9.83957192047852,24.7249999999112,7.14886745759505));
#282721=CARTESIAN_POINT('Ctrl Pts',(12.1623797632096,24.8749999999106,3.95179673813132));
#282722=CARTESIAN_POINT('Ctrl Pts',(12.1623797632096,25.02499999991,-1.48946194470292E-15));
#282723=CARTESIAN_POINT('Ctrl Pts',(12.1623797632096,25.1749999999094,-3.95179673813132));
#282724=CARTESIAN_POINT('Ctrl Pts',(9.83957192047852,25.3249999999088,-7.14886745759505));
#282725=CARTESIAN_POINT('Ctrl Pts',(7.51676407774743,25.4749999999082,-10.3459381770588));
#282726=CARTESIAN_POINT('Ctrl Pts',(3.7583820388737,25.6249999999076,-11.5671105274568));
#282727=CARTESIAN_POINT('Ctrl Pts',(-2.81045820625811E-14,25.774999999907,
-12.7882828778549));
#282728=CARTESIAN_POINT('Ctrl Pts',(-3.75838203887376,25.9249999999064,
-11.5671105274568));
#282729=CARTESIAN_POINT('Ctrl Pts',(-7.51676407774749,26.0749999999058,
-10.3459381770588));
#282730=CARTESIAN_POINT('Ctrl Pts',(-9.83957192047857,26.2249999999052,
-7.14886745759505));
#282731=CARTESIAN_POINT('Ctrl Pts',(-12.1623797632097,26.3749999999046,
-3.95179673813132));
#282732=CARTESIAN_POINT('Ctrl Pts',(-12.1623797632097,26.524999999904,2.97892388940585E-15));
#282733=CARTESIAN_POINT('Ctrl Pts',(-12.1623797632097,26.6749999999034,
3.95179673813133));
#282734=CARTESIAN_POINT('Ctrl Pts',(-9.83957192047857,26.8249999999028,
7.14886745759505));
#282735=CARTESIAN_POINT('Ctrl Pts',(-7.51676407774748,26.9749999999022,
10.3459381770588));
#282736=CARTESIAN_POINT('Ctrl Pts',(-3.75838203887375,27.1249999999016,
11.5671105274568));
#282737=CARTESIAN_POINT('Ctrl Pts',(-2.58362107598209E-14,27.274999999901,
12.7882828778549));
#282738=CARTESIAN_POINT('Ctrl Pts',(3.7583820388737,27.4249999999004,11.5671105274568));
#282739=CARTESIAN_POINT('Ctrl Pts',(7.51676407774743,27.5749999998998,10.3459381770588));
#282740=CARTESIAN_POINT('Ctrl Pts',(9.83957192047852,27.7249999998992,7.14886745759505));
#282741=CARTESIAN_POINT('Ctrl Pts',(12.1623797632096,27.8749999998986,3.95179673813132));
#282742=CARTESIAN_POINT('Ctrl Pts',(12.1623797632096,28.024999999898,-1.48946194470292E-15));
#282743=CARTESIAN_POINT('Ctrl Pts',(12.1623797632096,28.1749999998974,-3.95179673813132));
#282744=CARTESIAN_POINT('Ctrl Pts',(9.83957192047852,28.3249999998968,-7.14886745759505));
#282745=CARTESIAN_POINT('Ctrl Pts',(7.51676407774743,28.4749999998962,-10.3459381770588));
#282746=CARTESIAN_POINT('Ctrl Pts',(3.7583820388737,28.6249999998956,-11.5671105274568));
#282747=CARTESIAN_POINT('Ctrl Pts',(-2.9832291334243E-14,28.774999999895,
-12.7882828778549));
#282748=CARTESIAN_POINT('Ctrl Pts',(-3.75838203887376,28.9249999998944,
-11.5671105274568));
#282749=CARTESIAN_POINT('Ctrl Pts',(-7.51676407774749,29.0749999998938,
-10.3459381770588));
#282750=CARTESIAN_POINT('Ctrl Pts',(-9.83957192047858,29.2249999998932,
-7.14886745759505));
#282751=CARTESIAN_POINT('Ctrl Pts',(-12.1623797632097,29.3749999998926,
-3.95179673813132));
#282752=CARTESIAN_POINT('Ctrl Pts',(-12.1623797632097,29.524999999892,2.97892388940585E-15));
#282753=CARTESIAN_POINT('Ctrl Pts',(-12.1623797632097,29.6749999998914,
3.95179673813133));
#282754=CARTESIAN_POINT('Ctrl Pts',(-9.83957192047858,29.8249999998908,
7.14886745759505));
#282755=CARTESIAN_POINT('Ctrl Pts',(-7.51676407774748,29.9749999998902,
10.3459381770588));
#282756=CARTESIAN_POINT('Ctrl Pts',(-3.75838203887376,30.1249999998896,
11.5671105274568));
#282757=CARTESIAN_POINT('Ctrl Pts',(-2.75639200314827E-14,30.274999999889,
12.7882828778549));
#282758=CARTESIAN_POINT('Ctrl Pts',(3.7583820388737,30.4249999998884,11.5671105274568));
#282759=CARTESIAN_POINT('Ctrl Pts',(7.51676407774743,30.5749999998878,10.3459381770588));
#282760=CARTESIAN_POINT('Ctrl Pts',(9.83957192047852,30.7249999998872,7.14886745759505));
#282761=CARTESIAN_POINT('Ctrl Pts',(12.1623797632096,30.8749999998866,3.95179673813132));
#282762=CARTESIAN_POINT('Ctrl Pts',(12.1623797632096,31.024999999886,-1.48946194470292E-15));
#282763=CARTESIAN_POINT('Ctrl Pts',(12.1623797632096,31.1749999998854,-3.95179673813132));
#282764=CARTESIAN_POINT('Ctrl Pts',(9.83957192047852,31.3249999998848,-7.14886745759505));
#282765=CARTESIAN_POINT('Ctrl Pts',(7.51676407774742,31.4749999998842,-10.3459381770588));
#282766=CARTESIAN_POINT('Ctrl Pts',(3.7583820388737,31.6249999998836,-11.5671105274568));
#282767=CARTESIAN_POINT('Ctrl Pts',(-3.15600006059048E-14,31.774999999883,
-12.7882828778549));
#282768=CARTESIAN_POINT('Ctrl Pts',(-3.75838203887376,31.9249999998824,
-11.5671105274568));
#282769=CARTESIAN_POINT('Ctrl Pts',(-7.51676407774749,32.0749999998818,
-10.3459381770588));
#282770=CARTESIAN_POINT('Ctrl Pts',(-9.83957192047858,32.2249999998812,
-7.14886745759505));
#282771=CARTESIAN_POINT('Ctrl Pts',(-12.1623797632097,32.3749999998806,
-3.95179673813132));
#282772=CARTESIAN_POINT('Ctrl Pts',(-12.1623797632097,32.52499999988,2.97892388940585E-15));
#282773=CARTESIAN_POINT('Ctrl Pts',(-12.1623797632097,32.6749999998794,
3.95179673813133));
#282774=CARTESIAN_POINT('Ctrl Pts',(-9.83957192047858,32.8249999998788,
7.14886745759505));
#282775=CARTESIAN_POINT('Ctrl Pts',(-7.51676407774749,32.9749999998782,
10.3459381770588));
#282776=CARTESIAN_POINT('Ctrl Pts',(-3.75838203887376,33.1249999998776,
11.5671105274568));
#282777=CARTESIAN_POINT('Ctrl Pts',(-2.92916293031446E-14,33.274999999877,
12.7882828778549));
#282778=CARTESIAN_POINT('Ctrl Pts',(3.7583820388737,33.4249999998764,11.5671105274568));
#282779=CARTESIAN_POINT('Ctrl Pts',(7.51676407774743,33.5749999998758,10.3459381770588));
#282780=CARTESIAN_POINT('Ctrl Pts',(9.83957192047852,33.7249999998752,7.14886745759505));
#282781=CARTESIAN_POINT('Ctrl Pts',(12.1623797632096,33.8749999998746,3.95179673813132));
#282782=CARTESIAN_POINT('Ctrl Pts',(12.1623797632096,34.024999999874,-1.48946194470292E-15));
#282783=CARTESIAN_POINT('Ctrl Pts',(12.1623797632096,34.1749999998734,-3.95179673813132));
#282784=CARTESIAN_POINT('Ctrl Pts',(9.83957192047851,34.3249999998728,-7.14886745759505));
#282785=CARTESIAN_POINT('Ctrl Pts',(7.51676407774742,34.4749999998722,-10.3459381770588));
#282786=CARTESIAN_POINT('Ctrl Pts',(3.7583820388737,34.6249999998716,-11.5671105274568));
#282787=CARTESIAN_POINT('Ctrl Pts',(-3.32877098775667E-14,34.774999999871,
-12.7882828778549));
#282788=CARTESIAN_POINT('Ctrl Pts',(-3.75838203887376,34.9249999998704,
-11.5671105274568));
#282789=CARTESIAN_POINT('Ctrl Pts',(-7.51676407774749,35.0749999998698,
-10.3459381770588));
#282790=CARTESIAN_POINT('Ctrl Pts',(-9.83957192047858,35.2249999998692,
-7.14886745759505));
#282791=CARTESIAN_POINT('Ctrl Pts',(-12.1623797632097,35.3749999998686,
-3.95179673813132));
#282792=CARTESIAN_POINT('Ctrl Pts',(-12.1623797632097,35.524999999868,2.97892388940585E-15));
#282793=CARTESIAN_POINT('Ctrl Pts',(-12.1623797632097,35.6749999998674,
3.95179673813133));
#282794=CARTESIAN_POINT('Ctrl Pts',(-9.83957192047858,35.8249999998668,
7.14886745759505));
#282795=CARTESIAN_POINT('Ctrl Pts',(-7.51676407774749,35.9749999998662,
10.3459381770588));
#282796=CARTESIAN_POINT('Ctrl Pts',(-3.75838203887376,36.1249999998656,
11.5671105274568));
#282797=CARTESIAN_POINT('Ctrl Pts',(-3.10193385748064E-14,36.274999999865,
12.7882828778549));
#282798=CARTESIAN_POINT('Ctrl Pts',(3.7583820388737,36.4249999998644,11.5671105274568));
#282799=CARTESIAN_POINT('Ctrl Pts',(7.51676407774742,36.5749999998638,10.3459381770588));
#282800=CARTESIAN_POINT('Ctrl Pts',(9.83957192047851,36.7249999998632,7.14886745759505));
#282801=CARTESIAN_POINT('Ctrl Pts',(12.1623797632096,36.8749999998626,3.95179673813132));
#282802=CARTESIAN_POINT('Ctrl Pts',(12.1623797632096,37.024999999862,-1.48946194470292E-15));
#282803=CARTESIAN_POINT('Ctrl Pts',(12.1623797632096,37.1749999998614,-3.95179673813132));
#282804=CARTESIAN_POINT('Ctrl Pts',(9.83957192047851,37.3249999998608,-7.14886745759505));
#282805=CARTESIAN_POINT('Ctrl Pts',(7.51676407774742,37.4749999998602,-10.3459381770588));
#282806=CARTESIAN_POINT('Ctrl Pts',(3.75838203887369,37.6249999998596,-11.5671105274568));
#282807=CARTESIAN_POINT('Ctrl Pts',(-3.50154191492285E-14,37.774999999859,
-12.7882828778549));
#282808=CARTESIAN_POINT('Ctrl Pts',(-3.75838203887376,37.9249999998584,
-11.5671105274568));
#282809=CARTESIAN_POINT('Ctrl Pts',(-7.51676407774749,38.0749999998578,
-10.3459381770588));
#282810=CARTESIAN_POINT('Ctrl Pts',(-9.83957192047858,38.2249999998572,
-7.14886745759505));
#282811=CARTESIAN_POINT('Ctrl Pts',(-12.1623797632097,38.3749999998566,
-3.95179673813132));
#282812=CARTESIAN_POINT('Ctrl Pts',(-12.1623797632097,38.524999999856,2.97892388940585E-15));
#282813=CARTESIAN_POINT('Ctrl Pts',(-12.1623797632097,38.6749999998554,
3.95179673813133));
#282814=CARTESIAN_POINT('Ctrl Pts',(-9.83957192047858,38.8249999998548,
7.14886745759505));
#282815=CARTESIAN_POINT('Ctrl Pts',(-7.51676407774749,38.9749999998542,
10.3459381770588));
#282816=CARTESIAN_POINT('Ctrl Pts',(-3.75838203887376,39.1249999998536,
11.5671105274568));
#282817=CARTESIAN_POINT('Ctrl Pts',(-3.27470478464682E-14,39.274999999853,
12.7882828778549));
#282818=CARTESIAN_POINT('Ctrl Pts',(3.7583820388737,39.4249999998524,11.5671105274568));
#282819=CARTESIAN_POINT('Ctrl Pts',(7.51676407774742,39.5749999998518,10.3459381770588));
#282820=CARTESIAN_POINT('Ctrl Pts',(9.83957192047851,39.7249999998512,7.14886745759505));
#282821=CARTESIAN_POINT('Ctrl Pts',(12.1623797632096,39.8749999998506,3.95179673813132));
#282822=CARTESIAN_POINT('Ctrl Pts',(12.1623797632096,40.02499999985,-1.48946194470292E-15));
#282823=CARTESIAN_POINT('Ctrl Pts',(12.1623797632096,40.1749999998494,-3.95179673813132));
#282824=CARTESIAN_POINT('Ctrl Pts',(9.83957192047851,40.3249999998488,-7.14886745759505));
#282825=CARTESIAN_POINT('Ctrl Pts',(7.51676407774742,40.4749999998482,-10.3459381770588));
#282826=CARTESIAN_POINT('Ctrl Pts',(3.75838203887369,40.6249999998476,-11.5671105274568));
#282827=CARTESIAN_POINT('Ctrl Pts',(-3.67431284208903E-14,40.774999999847,
-12.7882828778549));
#282828=CARTESIAN_POINT('Ctrl Pts',(-3.75838203887376,40.9249999998464,
-11.5671105274568));
#282829=CARTESIAN_POINT('Ctrl Pts',(-7.51676407774749,41.0749999998458,
-10.3459381770588));
#282830=CARTESIAN_POINT('Ctrl Pts',(-9.83957192047858,41.2249999998452,
-7.14886745759505));
#282831=CARTESIAN_POINT('Ctrl Pts',(-12.1623797632097,41.3749999998446,
-3.95179673813132));
#282832=CARTESIAN_POINT('Ctrl Pts',(-12.1623797632097,41.524999999844,2.97892388940585E-15));
#282833=CARTESIAN_POINT('Ctrl Pts',(-12.1623797632097,41.6749999998434,
3.95179673813133));
#282834=CARTESIAN_POINT('Ctrl Pts',(-9.83957192047858,41.8249999998428,
7.14886745759505));
#282835=CARTESIAN_POINT('Ctrl Pts',(-7.51676407774749,41.9749999998422,
10.3459381770588));
#282836=CARTESIAN_POINT('Ctrl Pts',(-3.75838203887376,42.1249999998416,
11.5671105274568));
#282837=CARTESIAN_POINT('Ctrl Pts',(-3.44747571181301E-14,42.274999999841,
12.7882828778549));
#282838=CARTESIAN_POINT('Ctrl Pts',(3.75838203887369,42.4249999998404,11.5671105274568));
#282839=CARTESIAN_POINT('Ctrl Pts',(7.51676407774742,42.5749999998398,10.3459381770588));
#282840=CARTESIAN_POINT('Ctrl Pts',(9.83957192047851,42.7249999998392,7.14886745759505));
#282841=CARTESIAN_POINT('Ctrl Pts',(12.1623797632096,42.8749999998386,3.95179673813132));
#282842=CARTESIAN_POINT('Ctrl Pts',(12.1623797632096,43.024999999838,-1.48946194470292E-15));
#282843=CARTESIAN_POINT('Ctrl Pts',(12.1623797632096,43.1749999998374,-3.95179673813132));
#282844=CARTESIAN_POINT('Ctrl Pts',(9.83957192047851,43.3249999998368,-7.14886745759505));
#282845=CARTESIAN_POINT('Ctrl Pts',(7.51676407774742,43.4749999998362,-10.3459381770588));
#282846=CARTESIAN_POINT('Ctrl Pts',(3.75838203887369,43.6249999998356,-11.5671105274568));
#282847=CARTESIAN_POINT('Ctrl Pts',(-3.84708376925522E-14,43.774999999835,
-12.7882828778549));
#282848=CARTESIAN_POINT('Ctrl Pts',(-3.75838203887377,43.9249999998344,
-11.5671105274568));
#282849=CARTESIAN_POINT('Ctrl Pts',(-7.51676407774749,44.0749999998338,
-10.3459381770588));
#282850=CARTESIAN_POINT('Ctrl Pts',(-9.83957192047859,44.2249999998332,
-7.14886745759505));
#282851=CARTESIAN_POINT('Ctrl Pts',(-12.1623797632097,44.3749999998326,
-3.95179673813132));
#282852=CARTESIAN_POINT('Ctrl Pts',(-12.1623797632097,44.524999999832,2.97892388940585E-15));
#282853=CARTESIAN_POINT('Ctrl Pts',(-12.1623797632097,44.6749999998314,
3.95179673813133));
#282854=CARTESIAN_POINT('Ctrl Pts',(-9.83957192047859,44.8249999998308,
7.14886745759505));
#282855=CARTESIAN_POINT('Ctrl Pts',(-7.51676407774749,44.9749999998302,
10.3459381770588));
#282856=CARTESIAN_POINT('Ctrl Pts',(-3.75838203887376,45.1249999998296,
11.5671105274568));
#282857=CARTESIAN_POINT('Ctrl Pts',(-3.62024663897919E-14,45.274999999829,
12.7882828778549));
#282858=CARTESIAN_POINT('Ctrl Pts',(3.75838203887369,45.4249999998284,11.5671105274568));
#282859=CARTESIAN_POINT('Ctrl Pts',(7.51676407774742,45.5749999998278,10.3459381770588));
#282860=CARTESIAN_POINT('Ctrl Pts',(9.83957192047851,45.7249999998272,7.14886745759505));
#282861=CARTESIAN_POINT('Ctrl Pts',(12.1623797632096,45.8749999998266,3.95179673813132));
#282862=CARTESIAN_POINT('Ctrl Pts',(12.1623797632096,46.024999999826,-1.48946194470292E-15));
#282863=CARTESIAN_POINT('Ctrl Pts',(12.1623797632096,46.1749999998254,-3.95179673813132));
#282864=CARTESIAN_POINT('Ctrl Pts',(9.83957192047851,46.3249999998248,-7.14886745759505));
#282865=CARTESIAN_POINT('Ctrl Pts',(7.51676407774742,46.4749999998242,-10.3459381770588));
#282866=CARTESIAN_POINT('Ctrl Pts',(3.75838203887369,46.6249999998236,-11.5671105274568));
#282867=CARTESIAN_POINT('Ctrl Pts',(-4.0198546964214E-14,46.774999999823,
-12.7882828778549));
#282868=CARTESIAN_POINT('Ctrl Pts',(-3.75838203887377,46.9249999998224,
-11.5671105274568));
#282869=CARTESIAN_POINT('Ctrl Pts',(-7.5167640777475,47.0749999998218,-10.3459381770588));
#282870=CARTESIAN_POINT('Ctrl Pts',(-9.83957192047859,47.2249999998212,
-7.14886745759505));
#282871=CARTESIAN_POINT('Ctrl Pts',(-12.1623797632097,47.3749999998206,
-3.95179673813132));
#282872=CARTESIAN_POINT('Ctrl Pts',(-12.1623797632097,47.52499999982,2.97892388940585E-15));
#282873=CARTESIAN_POINT('Ctrl Pts',(-12.1623797632097,47.6749999998194,
3.95179673813133));
#282874=CARTESIAN_POINT('Ctrl Pts',(-9.83957192047859,47.8249999998188,
7.14886745759505));
#282875=CARTESIAN_POINT('Ctrl Pts',(-7.51676407774749,47.9749999998182,
10.3459381770588));
#282876=CARTESIAN_POINT('Ctrl Pts',(-3.75838203887377,48.1249999998176,
11.5671105274568));
#282877=CARTESIAN_POINT('Ctrl Pts',(-3.79301756614538E-14,48.274999999817,
12.7882828778549));
#282878=CARTESIAN_POINT('Ctrl Pts',(3.75838203887369,48.4249999998164,11.5671105274568));
#282879=CARTESIAN_POINT('Ctrl Pts',(7.51676407774742,48.5749999998158,10.3459381770588));
#282880=CARTESIAN_POINT('Ctrl Pts',(9.83957192047851,48.7249999998152,7.14886745759505));
#282881=CARTESIAN_POINT('Ctrl Pts',(12.1623797632096,48.8749999998146,3.95179673813132));
#282882=CARTESIAN_POINT('Ctrl Pts',(12.1623797632096,49.024999999814,-1.48946194470292E-15));
#282883=CARTESIAN_POINT('Ctrl Pts',(12.1623797632096,49.1749999998134,-3.95179673813132));
#282884=CARTESIAN_POINT('Ctrl Pts',(9.83957192047851,49.3249999998128,-7.14886745759505));
#282885=CARTESIAN_POINT('Ctrl Pts',(7.51676407774741,49.4749999998122,-10.3459381770588));
#282886=CARTESIAN_POINT('Ctrl Pts',(3.75838203887369,49.6249999998116,-11.5671105274568));
#282887=CARTESIAN_POINT('Ctrl Pts',(-4.19262562358759E-14,49.774999999811,
-12.7882828778549));
#282888=CARTESIAN_POINT('Ctrl Pts',(-3.75838203887377,49.9249999998104,
-11.5671105274568));
#282889=CARTESIAN_POINT('Ctrl Pts',(-7.5167640777475,50.0749999998098,-10.3459381770588));
#282890=CARTESIAN_POINT('Ctrl Pts',(-9.83957192047859,50.2249999998092,
-7.14886745759505));
#282891=CARTESIAN_POINT('Ctrl Pts',(-12.1623797632097,50.3749999998086,
-3.95179673813132));
#282892=CARTESIAN_POINT('Ctrl Pts',(-12.1623797632097,50.524999999808,2.97892388940585E-15));
#282893=CARTESIAN_POINT('Ctrl Pts',(-12.1623797632097,50.6749999998074,
3.95179673813133));
#282894=CARTESIAN_POINT('Ctrl Pts',(-9.83957192047859,50.8249999998068,
7.14886745759505));
#282895=CARTESIAN_POINT('Ctrl Pts',(-7.51676407774749,50.9749999998062,
10.3459381770588));
#282896=CARTESIAN_POINT('Ctrl Pts',(-3.75838203887377,51.1249999998056,
11.5671105274568));
#282897=CARTESIAN_POINT('Ctrl Pts',(-3.96578849331156E-14,51.274999999805,
12.7882828778549));
#282898=CARTESIAN_POINT('Ctrl Pts',(3.75838203887369,51.4249999998044,11.5671105274568));
#282899=CARTESIAN_POINT('Ctrl Pts',(7.51676407774742,51.5749999998038,10.3459381770588));
#282900=CARTESIAN_POINT('Ctrl Pts',(9.83957192047851,51.7249999998032,7.14886745759505));
#282901=CARTESIAN_POINT('Ctrl Pts',(12.1623797632096,51.8749999998026,3.95179673813132));
#282902=CARTESIAN_POINT('Ctrl Pts',(12.1623797632096,52.024999999802,-1.48946194470292E-15));
#282903=CARTESIAN_POINT('Ctrl Pts',(12.1623797632096,52.1749999998014,-3.95179673813132));
#282904=CARTESIAN_POINT('Ctrl Pts',(9.8395719204785,52.3249999998008,-7.14886745759505));
#282905=CARTESIAN_POINT('Ctrl Pts',(7.51676407774741,52.4749999998002,-10.3459381770588));
#282906=CARTESIAN_POINT('Ctrl Pts',(3.75838203887368,52.6249999997996,-11.5671105274568));
#282907=CARTESIAN_POINT('Ctrl Pts',(-4.36539655075377E-14,52.774999999799,
-12.7882828778549));
#282908=CARTESIAN_POINT('Ctrl Pts',(-3.75838203887377,52.9249999997984,
-11.5671105274568));
#282909=CARTESIAN_POINT('Ctrl Pts',(-7.5167640777475,53.0749999997978,-10.3459381770588));
#282910=CARTESIAN_POINT('Ctrl Pts',(-9.83957192047859,53.2249999997972,
-7.14886745759505));
#282911=CARTESIAN_POINT('Ctrl Pts',(-12.1623797632097,53.3749999997966,
-3.95179673813132));
#282912=CARTESIAN_POINT('Ctrl Pts',(-12.1623797632097,53.524999999796,2.97892388940585E-15));
#282913=CARTESIAN_POINT('Ctrl Pts',(-12.1623797632097,53.6749999997954,
3.95179673813133));
#282914=CARTESIAN_POINT('Ctrl Pts',(-9.83957192047859,53.8249999997948,
7.14886745759505));
#282915=CARTESIAN_POINT('Ctrl Pts',(-7.5167640777475,53.9749999997942,10.3459381770588));
#282916=CARTESIAN_POINT('Ctrl Pts',(-3.75838203887377,54.1249999997936,
11.5671105274568));
#282917=CARTESIAN_POINT('Ctrl Pts',(-4.13855942047774E-14,54.274999999793,
12.7882828778549));
#282918=CARTESIAN_POINT('Ctrl Pts',(3.75838203887369,54.4249999997924,11.5671105274568));
#282919=CARTESIAN_POINT('Ctrl Pts',(7.51676407774741,54.5749999997918,10.3459381770588));
#282920=CARTESIAN_POINT('Ctrl Pts',(9.8395719204785,54.7249999997912,7.14886745759505));
#282921=CARTESIAN_POINT('Ctrl Pts',(12.1623797632096,54.8749999997906,3.95179673813132));
#282922=CARTESIAN_POINT('Ctrl Pts',(12.1623797632096,55.02499999979,-1.48946194470292E-15));
#282923=CARTESIAN_POINT('Ctrl Pts',(12.1623797632096,55.1749999997894,-3.95179673813132));
#282924=CARTESIAN_POINT('Ctrl Pts',(9.8395719204785,55.3249999997888,-7.14886745759505));
#282925=CARTESIAN_POINT('Ctrl Pts',(7.51676407774741,55.4749999997882,-10.3459381770588));
#282926=CARTESIAN_POINT('Ctrl Pts',(3.75838203887368,55.6249999997876,-11.5671105274568));
#282927=CARTESIAN_POINT('Ctrl Pts',(-4.53816747791995E-14,55.774999999787,
-12.7882828778549));
#282928=CARTESIAN_POINT('Ctrl Pts',(-3.75838203887377,55.9249999997864,
-11.5671105274568));
#282929=CARTESIAN_POINT('Ctrl Pts',(-7.5167640777475,56.0749999997858,-10.3459381770588));
#282930=CARTESIAN_POINT('Ctrl Pts',(-9.83957192047859,56.2249999997852,
-7.14886745759505));
#282931=CARTESIAN_POINT('Ctrl Pts',(-12.1623797632097,56.3749999997846,
-3.95179673813132));
#282932=CARTESIAN_POINT('Ctrl Pts',(-12.1623797632097,56.524999999784,2.97892388940585E-15));
#282933=CARTESIAN_POINT('Ctrl Pts',(-12.1623797632097,56.6749999997834,
3.95179673813133));
#282934=CARTESIAN_POINT('Ctrl Pts',(-9.83957192047859,56.8249999997828,
7.14886745759505));
#282935=CARTESIAN_POINT('Ctrl Pts',(-7.5167640777475,56.9749999997822,10.3459381770588));
#282936=CARTESIAN_POINT('Ctrl Pts',(-3.75838203887377,57.1249999997816,
11.5671105274568));
#282937=CARTESIAN_POINT('Ctrl Pts',(-4.31133034764393E-14,57.274999999781,
12.7882828778549));
#282938=CARTESIAN_POINT('Ctrl Pts',(3.75838203887368,57.4249999997804,11.5671105274568));
#282939=CARTESIAN_POINT('Ctrl Pts',(7.51676407774741,57.5749999997798,10.3459381770588));
#282940=CARTESIAN_POINT('Ctrl Pts',(9.8395719204785,57.7249999997792,7.14886745759505));
#282941=CARTESIAN_POINT('Ctrl Pts',(12.1623797632096,57.8749999997786,3.95179673813132));
#282942=CARTESIAN_POINT('Ctrl Pts',(12.1623797632096,58.024999999778,-1.48946194470292E-15));
#282943=CARTESIAN_POINT('Ctrl Pts',(12.1623797632096,58.1749999997774,-3.95179673813132));
#282944=CARTESIAN_POINT('Ctrl Pts',(9.8395719204785,58.3249999997768,-7.14886745759505));
#282945=CARTESIAN_POINT('Ctrl Pts',(7.51676407774741,58.4749999997762,-10.3459381770588));
#282946=CARTESIAN_POINT('Ctrl Pts',(3.75838203887368,58.6249999997756,-11.5671105274568));
#282947=CARTESIAN_POINT('Ctrl Pts',(-4.71093840508614E-14,58.774999999775,
-12.7882828778549));
#282948=CARTESIAN_POINT('Ctrl Pts',(-3.75838203887377,58.9249999997744,
-11.5671105274568));
#282949=CARTESIAN_POINT('Ctrl Pts',(-7.5167640777475,59.0749999997738,-10.3459381770588));
#282950=CARTESIAN_POINT('Ctrl Pts',(-9.83957192047859,59.2249999997732,
-7.14886745759505));
#282951=CARTESIAN_POINT('Ctrl Pts',(-12.1623797632097,59.3749999997726,
-3.95179673813132));
#282952=CARTESIAN_POINT('Ctrl Pts',(-12.1623797632097,59.524999999772,2.97892388940585E-15));
#282953=CARTESIAN_POINT('Ctrl Pts',(-12.1623797632097,59.6749999997714,
3.95179673813133));
#282954=CARTESIAN_POINT('Ctrl Pts',(-9.83957192047859,59.8249999997708,
7.14886745759505));
#282955=CARTESIAN_POINT('Ctrl Pts',(-7.5167640777475,59.9749999997702,10.3459381770588));
#282956=CARTESIAN_POINT('Ctrl Pts',(-3.75838203887377,60.1249999997696,
11.5671105274568));
#282957=CARTESIAN_POINT('Ctrl Pts',(-4.48410127481011E-14,60.274999999769,
12.7882828778549));
#282958=CARTESIAN_POINT('Ctrl Pts',(3.75838203887368,60.4249999997684,11.5671105274568));
#282959=CARTESIAN_POINT('Ctrl Pts',(7.51676407774741,60.5749999997678,10.3459381770588));
#282960=CARTESIAN_POINT('Ctrl Pts',(9.8395719204785,60.7249999997672,7.14886745759505));
#282961=CARTESIAN_POINT('Ctrl Pts',(12.1623797632096,60.8749999997666,3.95179673813132));
#282962=CARTESIAN_POINT('Ctrl Pts',(12.1623797632096,61.024999999766,-1.48946194470292E-15));
#282963=CARTESIAN_POINT('Ctrl Pts',(12.1623797632096,61.1749999997654,-3.95179673813132));
#282964=CARTESIAN_POINT('Ctrl Pts',(9.8395719204785,61.3249999997648,-7.14886745759505));
#282965=CARTESIAN_POINT('Ctrl Pts',(7.51676407774741,61.4749999997642,-10.3459381770588));
#282966=CARTESIAN_POINT('Ctrl Pts',(3.75838203887368,61.6249999997636,-11.5671105274568));
#282967=CARTESIAN_POINT('Ctrl Pts',(-4.88370933225232E-14,61.774999999763,
-12.7882828778549));
#282968=CARTESIAN_POINT('Ctrl Pts',(-3.75838203887378,61.9249999997624,
-11.5671105274568));
#282969=CARTESIAN_POINT('Ctrl Pts',(-7.5167640777475,62.0749999997618,-10.3459381770588));
#282970=CARTESIAN_POINT('Ctrl Pts',(-9.8395719204786,62.2249999997612,-7.14886745759505));
#282971=CARTESIAN_POINT('Ctrl Pts',(-12.1623797632097,62.3749999997606,
-3.95179673813132));
#282972=CARTESIAN_POINT('Ctrl Pts',(-12.1623797632097,62.52499999976,2.97892388940585E-15));
#282973=CARTESIAN_POINT('Ctrl Pts',(-12.1623797632097,62.6749999997594,
3.95179673813133));
#282974=CARTESIAN_POINT('Ctrl Pts',(-9.8395719204786,62.8249999997588,7.14886745759505));
#282975=CARTESIAN_POINT('Ctrl Pts',(-7.5167640777475,62.9749999997582,10.3459381770588));
#282976=CARTESIAN_POINT('Ctrl Pts',(-3.75838203887377,63.1249999997576,
11.5671105274568));
#282977=CARTESIAN_POINT('Ctrl Pts',(-4.6568722019763E-14,63.274999999757,
12.7882828778549));
#282978=CARTESIAN_POINT('Ctrl Pts',(3.75838203887368,63.4249999997564,11.5671105274568));
#282979=CARTESIAN_POINT('Ctrl Pts',(7.51676407774741,63.5749999997558,10.3459381770588));
#282980=CARTESIAN_POINT('Ctrl Pts',(9.8395719204785,63.7249999997552,7.14886745759505));
#282981=CARTESIAN_POINT('Ctrl Pts',(12.1623797632096,63.8749999997546,3.95179673813132));
#282982=CARTESIAN_POINT('Ctrl Pts',(12.1623797632096,64.024999999754,-1.48946194470292E-15));
#282983=CARTESIAN_POINT('Ctrl Pts',(12.1623797632096,64.1749999997534,-3.95179673813132));
#282984=CARTESIAN_POINT('Ctrl Pts',(9.8395719204785,64.3249999997528,-7.14886745759505));
#282985=CARTESIAN_POINT('Ctrl Pts',(7.5167640777474,64.4749999997522,-10.3459381770588));
#282986=CARTESIAN_POINT('Ctrl Pts',(3.75838203887368,64.6249999997516,-11.5671105274568));
#282987=CARTESIAN_POINT('Ctrl Pts',(-5.05648025941851E-14,64.774999999751,
-12.7882828778549));
#282988=CARTESIAN_POINT('Ctrl Pts',(-3.75838203887378,64.9249999997504,
-11.5671105274568));
#282989=CARTESIAN_POINT('Ctrl Pts',(-7.51676407774751,65.0749999997498,
-10.3459381770588));
#282990=CARTESIAN_POINT('Ctrl Pts',(-9.8395719204786,65.2249999997492,-7.14886745759505));
#282991=CARTESIAN_POINT('Ctrl Pts',(-12.1623797632097,65.3749999997486,
-3.95179673813132));
#282992=CARTESIAN_POINT('Ctrl Pts',(-12.1623797632097,65.524999999748,2.97892388940585E-15));
#282993=CARTESIAN_POINT('Ctrl Pts',(-12.1623797632097,65.6749999997474,
3.95179673813133));
#282994=CARTESIAN_POINT('Ctrl Pts',(-9.8395719204786,65.8249999997468,7.14886745759505));
#282995=CARTESIAN_POINT('Ctrl Pts',(-7.5167640777475,65.9749999997462,10.3459381770588));
#282996=CARTESIAN_POINT('Ctrl Pts',(-3.75838203887378,66.1249999997456,
11.5671105274568));
#282997=CARTESIAN_POINT('Ctrl Pts',(-4.82964312914248E-14,66.274999999745,
12.7882828778549));
#282998=CARTESIAN_POINT('Ctrl Pts',(3.75838203887368,66.4249999997444,11.5671105274568));
#282999=CARTESIAN_POINT('Ctrl Pts',(7.51676407774741,66.5749999997438,10.3459381770588));
#283000=CARTESIAN_POINT('Ctrl Pts',(9.8395719204785,66.7249999997432,7.14886745759505));
#283001=CARTESIAN_POINT('Ctrl Pts',(12.1623797632096,66.8749999997426,3.95179673813132));
#283002=CARTESIAN_POINT('Ctrl Pts',(12.1623797632096,67.024999999742,-1.48946194470292E-15));
#283003=CARTESIAN_POINT('Ctrl Pts',(12.1623797632096,67.1749999997414,-3.95179673813132));
#283004=CARTESIAN_POINT('Ctrl Pts',(9.8395719204785,67.3249999997408,-7.14886745759505));
#283005=CARTESIAN_POINT('Ctrl Pts',(7.5167640777474,67.4749999997402,-10.3459381770588));
#283006=CARTESIAN_POINT('Ctrl Pts',(3.75838203887368,67.6249999997396,-11.5671105274568));
#283007=CARTESIAN_POINT('Ctrl Pts',(-5.22925118658469E-14,67.774999999739,
-12.7882828778549));
#283008=CARTESIAN_POINT('Ctrl Pts',(-3.75838203887378,67.9249999997384,
-11.5671105274568));
#283009=CARTESIAN_POINT('Ctrl Pts',(-7.51676407774751,68.0749999997378,
-10.3459381770588));
#283010=CARTESIAN_POINT('Ctrl Pts',(-9.8395719204786,68.2249999997372,-7.14886745759505));
#283011=CARTESIAN_POINT('Ctrl Pts',(-12.1623797632097,68.3749999997366,
-3.95179673813132));
#283012=CARTESIAN_POINT('Ctrl Pts',(-12.1623797632097,68.524999999736,2.97892388940585E-15));
#283013=CARTESIAN_POINT('Ctrl Pts',(-12.1623797632097,68.6749999997354,
3.95179673813133));
#283014=CARTESIAN_POINT('Ctrl Pts',(-9.8395719204786,68.8249999997348,7.14886745759505));
#283015=CARTESIAN_POINT('Ctrl Pts',(-7.51676407774751,68.9749999997342,
10.3459381770588));
#283016=CARTESIAN_POINT('Ctrl Pts',(-3.75838203887378,69.1249999997336,
11.5671105274568));
#283017=CARTESIAN_POINT('Ctrl Pts',(-5.00241405630866E-14,69.274999999733,
12.7882828778549));
#283018=CARTESIAN_POINT('Ctrl Pts',(3.75838203887368,69.4249999997324,11.5671105274568));
#283019=CARTESIAN_POINT('Ctrl Pts',(7.5167640777474,69.5749999997318,10.3459381770588));
#283020=CARTESIAN_POINT('Ctrl Pts',(9.8395719204785,69.7249999997312,7.14886745759505));
#283021=CARTESIAN_POINT('Ctrl Pts',(12.1623797632096,69.8749999997306,3.95179673813132));
#283022=CARTESIAN_POINT('Ctrl Pts',(12.1623797632096,70.02499999973,-1.48946194470292E-15));
#283023=CARTESIAN_POINT('Ctrl Pts',(12.1623797632096,70.1749999997294,-3.95179673813132));
#283024=CARTESIAN_POINT('Ctrl Pts',(9.83957192047849,70.3249999997288,-7.14886745759505));
#283025=CARTESIAN_POINT('Ctrl Pts',(7.5167640777474,70.4749999997282,-10.3459381770588));
#283026=CARTESIAN_POINT('Ctrl Pts',(3.75838203887367,70.6249999997276,-11.5671105274568));
#283027=CARTESIAN_POINT('Ctrl Pts',(-5.40202211375087E-14,70.774999999727,
-12.7882828778549));
#283028=CARTESIAN_POINT('Ctrl Pts',(-3.75838203887378,70.9249999997264,
-11.5671105274568));
#283029=CARTESIAN_POINT('Ctrl Pts',(-7.51676407774751,71.0749999997258,
-10.3459381770588));
#283030=CARTESIAN_POINT('Ctrl Pts',(-9.8395719204786,71.2249999997252,-7.14886745759505));
#283031=CARTESIAN_POINT('Ctrl Pts',(-12.1623797632097,71.3749999997246,
-3.95179673813132));
#283032=CARTESIAN_POINT('Ctrl Pts',(-12.1623797632097,71.524999999724,2.97892388940585E-15));
#283033=CARTESIAN_POINT('Ctrl Pts',(-12.1623797632097,71.6749999997234,
3.95179673813133));
#283034=CARTESIAN_POINT('Ctrl Pts',(-9.8395719204786,71.8249999997228,7.14886745759505));
#283035=CARTESIAN_POINT('Ctrl Pts',(-7.51676407774751,71.9749999997222,
10.3459381770588));
#283036=CARTESIAN_POINT('Ctrl Pts',(-3.75838203887378,72.1249999997216,
11.5671105274568));
#283037=CARTESIAN_POINT('Ctrl Pts',(-5.17518498347485E-14,72.274999999721,
12.7882828778549));
#283038=CARTESIAN_POINT('Ctrl Pts',(3.75838203887368,72.4249999997204,11.5671105274568));
#283039=CARTESIAN_POINT('Ctrl Pts',(7.5167640777474,72.5749999997198,10.3459381770588));
#283040=CARTESIAN_POINT('Ctrl Pts',(9.83957192047849,72.7249999997192,7.14886745759505));
#283041=CARTESIAN_POINT('Ctrl Pts',(12.1623797632096,72.8749999997186,3.95179673813132));
#283042=CARTESIAN_POINT('Ctrl Pts',(12.1623797632096,73.024999999718,-1.48946194470292E-15));
#283043=CARTESIAN_POINT('Ctrl Pts',(12.1623797632096,73.1749999997174,-3.95179673813132));
#283044=CARTESIAN_POINT('Ctrl Pts',(9.83957192047849,73.3249999997168,-7.14886745759505));
#283045=CARTESIAN_POINT('Ctrl Pts',(7.5167640777474,73.4749999997162,-10.3459381770588));
#283046=CARTESIAN_POINT('Ctrl Pts',(3.75838203887367,73.6249999997156,-11.5671105274568));
#283047=CARTESIAN_POINT('Ctrl Pts',(-5.57479304091706E-14,73.774999999715,
-12.7882828778549));
#283048=CARTESIAN_POINT('Ctrl Pts',(-3.75838203887378,73.9249999997144,
-11.5671105274568));
#283049=CARTESIAN_POINT('Ctrl Pts',(-7.51676407774751,74.0749999997138,
-10.3459381770588));
#283050=CARTESIAN_POINT('Ctrl Pts',(-9.8395719204786,74.2249999997132,-7.14886745759505));
#283051=CARTESIAN_POINT('Ctrl Pts',(-12.1623797632097,74.3749999997126,
-3.95179673813132));
#283052=CARTESIAN_POINT('Ctrl Pts',(-12.1623797632097,74.524999999712,2.97892388940585E-15));
#283053=CARTESIAN_POINT('Ctrl Pts',(-12.1623797632097,74.6749999997114,
3.95179673813133));
#283054=CARTESIAN_POINT('Ctrl Pts',(-9.8395719204786,74.8249999997108,7.14886745759505));
#283055=CARTESIAN_POINT('Ctrl Pts',(-7.51676407774751,74.9749999997102,
10.3459381770588));
#283056=CARTESIAN_POINT('Ctrl Pts',(-3.75838203887378,75.1249999997096,
11.5671105274568));
#283057=CARTESIAN_POINT('Ctrl Pts',(-5.34795591064103E-14,75.274999999709,
12.7882828778549));
#283058=CARTESIAN_POINT('Ctrl Pts',(3.75838203887367,75.4249999997084,11.5671105274568));
#283059=CARTESIAN_POINT('Ctrl Pts',(7.5167640777474,75.5749999997078,10.3459381770588));
#283060=CARTESIAN_POINT('Ctrl Pts',(9.83957192047849,75.7249999997072,7.14886745759505));
#283061=CARTESIAN_POINT('Ctrl Pts',(12.1623797632096,75.8749999997066,3.95179673813132));
#283062=CARTESIAN_POINT('Ctrl Pts',(12.1623797632096,76.024999999706,-1.48946194470292E-15));
#283063=CARTESIAN_POINT('Ctrl Pts',(12.1623797632096,76.1749999997054,-3.95179673813132));
#283064=CARTESIAN_POINT('Ctrl Pts',(9.83957192047849,76.3249999997048,-7.14886745759505));
#283065=CARTESIAN_POINT('Ctrl Pts',(7.5167640777474,76.4749999997042,-10.3459381770588));
#283066=CARTESIAN_POINT('Ctrl Pts',(3.75838203887367,76.6249999997036,-11.5671105274568));
#283067=CARTESIAN_POINT('Ctrl Pts',(-5.74756396808324E-14,76.774999999703,
-12.7882828778549));
#283068=CARTESIAN_POINT('Ctrl Pts',(-3.75838203887379,76.9249999997024,
-11.5671105274568));
#283069=CARTESIAN_POINT('Ctrl Pts',(-7.51676407774751,77.0749999997018,
-10.3459381770588));
#283070=CARTESIAN_POINT('Ctrl Pts',(-9.8395719204786,77.2249999997012,-7.14886745759505));
#283071=CARTESIAN_POINT('Ctrl Pts',(-12.1623797632097,77.3749999997006,
-3.95179673813132));
#283072=CARTESIAN_POINT('Ctrl Pts',(-12.1623797632097,77.5249999997,2.97892388940585E-15));
#283073=CARTESIAN_POINT('Ctrl Pts',(-12.1623797632097,77.6749999996994,
3.95179673813133));
#283074=CARTESIAN_POINT('Ctrl Pts',(-9.8395719204786,77.8249999996988,7.14886745759505));
#283075=CARTESIAN_POINT('Ctrl Pts',(-7.51676407774751,77.9749999996982,
10.3459381770588));
#283076=CARTESIAN_POINT('Ctrl Pts',(-3.75838203887378,78.1249999996976,
11.5671105274568));
#283077=CARTESIAN_POINT('Ctrl Pts',(-5.52072683780721E-14,78.274999999697,
12.7882828778549));
#283078=CARTESIAN_POINT('Ctrl Pts',(3.75838203887367,78.4249999996964,11.5671105274568));
#283079=CARTESIAN_POINT('Ctrl Pts',(7.5167640777474,78.5749999996958,10.3459381770588));
#283080=CARTESIAN_POINT('Ctrl Pts',(9.83957192047849,78.7249999996952,7.14886745759505));
#283081=CARTESIAN_POINT('Ctrl Pts',(12.1623797632096,78.8749999996946,3.95179673813132));
#283082=CARTESIAN_POINT('Ctrl Pts',(12.1623797632096,79.024999999694,-1.48946194470292E-15));
#283083=CARTESIAN_POINT('Ctrl Pts',(12.1623797632096,79.1749999996934,-3.95179673813132));
#283084=CARTESIAN_POINT('Ctrl Pts',(9.83957192047849,79.3249999996928,-7.14886745759505));
#283085=CARTESIAN_POINT('Ctrl Pts',(7.5167640777474,79.4749999996922,-10.3459381770588));
#283086=CARTESIAN_POINT('Ctrl Pts',(3.75838203887367,79.6249999996916,-11.5671105274568));
#283087=CARTESIAN_POINT('Ctrl Pts',(-5.92033489524943E-14,79.774999999691,
-12.7882828778549));
#283088=CARTESIAN_POINT('Ctrl Pts',(-3.75838203887379,79.9249999996904,
-11.5671105274568));
#283089=CARTESIAN_POINT('Ctrl Pts',(-7.51676407774751,80.0749999996898,
-10.3459381770588));
#283090=CARTESIAN_POINT('Ctrl Pts',(-9.83957192047861,80.2249999996892,
-7.14886745759505));
#283091=CARTESIAN_POINT('Ctrl Pts',(-12.1623797632097,80.3749999996886,
-3.95179673813132));
#283092=CARTESIAN_POINT('Ctrl Pts',(-12.1623797632097,80.524999999688,2.97892388940585E-15));
#283093=CARTESIAN_POINT('Ctrl Pts',(-12.1623797632097,80.6749999996874,
3.95179673813133));
#283094=CARTESIAN_POINT('Ctrl Pts',(-9.83957192047861,80.8249999996868,
7.14886745759505));
#283095=CARTESIAN_POINT('Ctrl Pts',(-7.51676407774751,80.9749999996862,
10.3459381770588));
#283096=CARTESIAN_POINT('Ctrl Pts',(-3.75838203887378,81.1249999996856,
11.5671105274568));
#283097=CARTESIAN_POINT('Ctrl Pts',(-5.6934977649734E-14,81.274999999685,
12.7882828778549));
#283098=CARTESIAN_POINT('Ctrl Pts',(3.75838203887367,81.4249999996844,11.5671105274568));
#283099=CARTESIAN_POINT('Ctrl Pts',(7.5167640777474,81.5749999996838,10.3459381770588));
#283100=CARTESIAN_POINT('Ctrl Pts',(9.83957192047849,81.7249999996832,7.14886745759505));
#283101=CARTESIAN_POINT('Ctrl Pts',(12.1623797632096,81.8749999996826,3.95179673813132));
#283102=CARTESIAN_POINT('Ctrl Pts',(12.1623797632096,82.024999999682,-1.48946194470292E-15));
#283103=CARTESIAN_POINT('Ctrl Pts',(12.1623797632096,82.1749999996814,-3.95179673813132));
#283104=CARTESIAN_POINT('Ctrl Pts',(9.83957192047849,82.3249999996808,-7.14886745759505));
#283105=CARTESIAN_POINT('Ctrl Pts',(7.5167640777474,82.4749999996802,-10.3459381770588));
#283106=CARTESIAN_POINT('Ctrl Pts',(3.75838203887367,82.6249999996796,-11.5671105274568));
#283107=CARTESIAN_POINT('Ctrl Pts',(-6.09310582241561E-14,82.774999999679,
-12.7882828778549));
#283108=CARTESIAN_POINT('Ctrl Pts',(-3.75838203887379,82.9249999996784,
-11.5671105274568));
#283109=CARTESIAN_POINT('Ctrl Pts',(-7.51676407774752,83.0749999996778,
-10.3459381770588));
#283110=CARTESIAN_POINT('Ctrl Pts',(-9.83957192047861,83.2249999996772,
-7.14886745759505));
#283111=CARTESIAN_POINT('Ctrl Pts',(-12.1623797632097,83.3749999996766,
-3.95179673813132));
#283112=CARTESIAN_POINT('Ctrl Pts',(-12.1623797632097,83.524999999676,2.97892388940585E-15));
#283113=CARTESIAN_POINT('Ctrl Pts',(-12.1623797632097,83.6749999996754,
3.95179673813133));
#283114=CARTESIAN_POINT('Ctrl Pts',(-9.83957192047861,83.8249999996748,
7.14886745759505));
#283115=CARTESIAN_POINT('Ctrl Pts',(-7.51676407774751,83.9749999996742,
10.3459381770588));
#283116=CARTESIAN_POINT('Ctrl Pts',(-3.75838203887379,84.1249999996736,
11.5671105274568));
#283117=CARTESIAN_POINT('Ctrl Pts',(-5.86626869213958E-14,84.274999999673,
12.7882828778549));
#283118=CARTESIAN_POINT('Ctrl Pts',(3.75838203887367,84.4249999996724,11.5671105274568));
#283119=CARTESIAN_POINT('Ctrl Pts',(7.5167640777474,84.5749999996718,10.3459381770588));
#283120=CARTESIAN_POINT('Ctrl Pts',(9.83957192047849,84.7249999996712,7.14886745759505));
#283121=CARTESIAN_POINT('Ctrl Pts',(12.1623797632096,84.8749999996706,3.95179673813132));
#283122=CARTESIAN_POINT('Ctrl Pts',(12.1623797632096,85.02499999967,-1.48946194470292E-15));
#283123=CARTESIAN_POINT('Ctrl Pts',(12.1623797632096,85.1749999996694,-3.95179673813132));
#283124=CARTESIAN_POINT('Ctrl Pts',(9.83957192047849,85.3249999996688,-7.14886745759505));
#283125=CARTESIAN_POINT('Ctrl Pts',(7.51676407774739,85.4749999996682,-10.3459381770588));
#283126=CARTESIAN_POINT('Ctrl Pts',(3.75838203887367,85.6249999996676,-11.5671105274568));
#283127=CARTESIAN_POINT('Ctrl Pts',(-6.26587674958179E-14,85.774999999667,
-12.7882828778549));
#283128=CARTESIAN_POINT('Ctrl Pts',(-3.75838203887379,85.9249999996664,
-11.5671105274568));
#283129=CARTESIAN_POINT('Ctrl Pts',(-7.51676407774752,86.0749999996658,
-10.3459381770588));
#283130=CARTESIAN_POINT('Ctrl Pts',(-9.83957192047861,86.2249999996652,
-7.14886745759505));
#283131=CARTESIAN_POINT('Ctrl Pts',(-12.1623797632097,86.3749999996646,
-3.95179673813132));
#283132=CARTESIAN_POINT('Ctrl Pts',(-12.1623797632097,86.524999999664,2.97892388940585E-15));
#283133=CARTESIAN_POINT('Ctrl Pts',(-12.1623797632097,86.6749999996634,
3.95179673813133));
#283134=CARTESIAN_POINT('Ctrl Pts',(-9.83957192047861,86.8249999996628,
7.14886745759505));
#283135=CARTESIAN_POINT('Ctrl Pts',(-7.51676407774752,86.9749999996622,
10.3459381770588));
#283136=CARTESIAN_POINT('Ctrl Pts',(-3.75838203887379,87.1249999996616,
11.5671105274568));
#283137=CARTESIAN_POINT('Ctrl Pts',(-6.03903961930577E-14,87.274999999661,
12.7882828778549));
#283138=CARTESIAN_POINT('Ctrl Pts',(3.75838203887367,87.4249999996604,11.5671105274568));
#283139=CARTESIAN_POINT('Ctrl Pts',(7.5167640777474,87.5749999996598,10.3459381770588));
#283140=CARTESIAN_POINT('Ctrl Pts',(9.83957192047849,87.7249999996592,7.14886745759505));
#283141=CARTESIAN_POINT('Ctrl Pts',(12.1623797632096,87.8749999996586,3.95179673813132));
#283142=CARTESIAN_POINT('Ctrl Pts',(12.1623797632096,88.024999999658,-1.48946194470292E-15));
#283143=CARTESIAN_POINT('Ctrl Pts',(12.1623797632096,88.1749999996574,-3.95179673813132));
#283144=CARTESIAN_POINT('Ctrl Pts',(9.83957192047849,88.3249999996568,-7.14886745759505));
#283145=CARTESIAN_POINT('Ctrl Pts',(7.51676407774739,88.4749999996562,-10.3459381770588));
#283146=CARTESIAN_POINT('Ctrl Pts',(3.75838203887366,88.6249999996556,-11.5671105274568));
#283147=CARTESIAN_POINT('Ctrl Pts',(-6.43864767674798E-14,88.774999999655,
-12.7882828778549));
#283148=CARTESIAN_POINT('Ctrl Pts',(-3.75838203887379,88.9249999996544,
-11.5671105274568));
#283149=CARTESIAN_POINT('Ctrl Pts',(-7.51676407774752,89.0749999996538,
-10.3459381770588));
#283150=CARTESIAN_POINT('Ctrl Pts',(-9.83957192047861,89.2249999996532,
-7.14886745759505));
#283151=CARTESIAN_POINT('Ctrl Pts',(-12.1623797632097,89.3749999996526,
-3.95179673813132));
#283152=CARTESIAN_POINT('Ctrl Pts',(-12.1623797632097,89.524999999652,2.97892388940585E-15));
#283153=CARTESIAN_POINT('Ctrl Pts',(-12.1623797632097,89.6749999996514,
3.95179673813133));
#283154=CARTESIAN_POINT('Ctrl Pts',(-9.83957192047861,89.8249999996508,
7.14886745759505));
#283155=CARTESIAN_POINT('Ctrl Pts',(-7.51676407774752,89.9749999996502,
10.3459381770588));
#283156=CARTESIAN_POINT('Ctrl Pts',(-3.75838203887379,90.1249999996496,
11.5671105274568));
#283157=CARTESIAN_POINT('Ctrl Pts',(-6.21181054647195E-14,90.274999999649,
12.7882828778549));
#283158=CARTESIAN_POINT('Ctrl Pts',(3.75838203887366,90.4249999996484,11.5671105274568));
#283159=CARTESIAN_POINT('Ctrl Pts',(7.51676407774739,90.5749999996478,10.3459381770588));
#283160=CARTESIAN_POINT('Ctrl Pts',(9.83957192047848,90.7249999996472,7.14886745759505));
#283161=CARTESIAN_POINT('Ctrl Pts',(12.1623797632096,90.8749999996466,3.95179673813132));
#283162=CARTESIAN_POINT('Ctrl Pts',(12.1623797632096,91.024999999646,-1.48946194470292E-15));
#283163=CARTESIAN_POINT('Ctrl Pts',(12.1623797632096,91.1749999996454,-3.95179673813132));
#283164=CARTESIAN_POINT('Ctrl Pts',(9.83957192047848,91.3249999996448,-7.14886745759505));
#283165=CARTESIAN_POINT('Ctrl Pts',(7.51676407774739,91.4749999996442,-10.3459381770588));
#283166=CARTESIAN_POINT('Ctrl Pts',(3.75838203887366,91.6249999996436,-11.5671105274568));
#283167=CARTESIAN_POINT('Ctrl Pts',(-6.61141860391416E-14,91.774999999643,
-12.7882828778549));
#283168=CARTESIAN_POINT('Ctrl Pts',(-3.75838203887379,91.9249999996424,
-11.5671105274568));
#283169=CARTESIAN_POINT('Ctrl Pts',(-7.51676407774752,92.0749999996418,
-10.3459381770588));
#283170=CARTESIAN_POINT('Ctrl Pts',(-9.83957192047861,92.2249999996412,
-7.14886745759505));
#283171=CARTESIAN_POINT('Ctrl Pts',(-12.1623797632097,92.3749999996406,
-3.95179673813132));
#283172=CARTESIAN_POINT('Ctrl Pts',(-12.1623797632097,92.52499999964,2.97892388940585E-15));
#283173=CARTESIAN_POINT('Ctrl Pts',(-12.1623797632097,92.6749999996394,
3.95179673813133));
#283174=CARTESIAN_POINT('Ctrl Pts',(-9.83957192047861,92.8249999996388,
7.14886745759505));
#283175=CARTESIAN_POINT('Ctrl Pts',(-7.51676407774752,92.9749999996382,
10.3459381770588));
#283176=CARTESIAN_POINT('Ctrl Pts',(-3.75838203887379,93.1249999996376,
11.5671105274568));
#283177=CARTESIAN_POINT('Ctrl Pts',(-6.38458147363813E-14,93.274999999637,
12.7882828778549));
#283178=CARTESIAN_POINT('Ctrl Pts',(3.75838203887366,93.4249999996364,11.5671105274568));
#283179=CARTESIAN_POINT('Ctrl Pts',(7.51676407774739,93.5749999996358,10.3459381770588));
#283180=CARTESIAN_POINT('Ctrl Pts',(9.83957192047848,93.7249999996352,7.14886745759505));
#283181=CARTESIAN_POINT('Ctrl Pts',(12.1623797632096,93.8749999996346,3.95179673813132));
#283182=CARTESIAN_POINT('Ctrl Pts',(12.1623797632096,94.024999999634,-1.48946194470292E-15));
#283183=CARTESIAN_POINT('Ctrl Pts',(12.1623797632096,94.1749999996334,-3.95179673813132));
#283184=CARTESIAN_POINT('Ctrl Pts',(9.83957192047848,94.3249999996328,-7.14886745759505));
#283185=CARTESIAN_POINT('Ctrl Pts',(7.51676407774739,94.4749999996322,-10.3459381770588));
#283186=CARTESIAN_POINT('Ctrl Pts',(3.75838203887366,94.6249999996316,-11.5671105274568));
#283187=CARTESIAN_POINT('Ctrl Pts',(-6.78418953108034E-14,94.774999999631,
-12.7882828778549));
#283188=CARTESIAN_POINT('Ctrl Pts',(-3.7583820388738,94.9249999996304,-11.5671105274568));
#283189=CARTESIAN_POINT('Ctrl Pts',(-7.51676407774752,95.0749999996298,
-10.3459381770588));
#283190=CARTESIAN_POINT('Ctrl Pts',(-9.83957192047862,95.2249999996292,
-7.14886745759505));
#283191=CARTESIAN_POINT('Ctrl Pts',(-12.1623797632097,95.3749999996286,
-3.95179673813132));
#283192=CARTESIAN_POINT('Ctrl Pts',(-12.1623797632097,95.524999999628,2.97892388940585E-15));
#283193=CARTESIAN_POINT('Ctrl Pts',(-12.1623797632097,95.6749999996274,
3.95179673813133));
#283194=CARTESIAN_POINT('Ctrl Pts',(-9.83957192047862,95.8249999996268,
7.14886745759505));
#283195=CARTESIAN_POINT('Ctrl Pts',(-7.51676407774752,95.9749999996262,
10.3459381770588));
#283196=CARTESIAN_POINT('Ctrl Pts',(-3.75838203887379,96.1249999996256,
11.5671105274568));
#283197=CARTESIAN_POINT('Ctrl Pts',(-6.55735240080432E-14,96.274999999625,
12.7882828778549));
#283198=CARTESIAN_POINT('Ctrl Pts',(3.75838203887366,96.4249999996244,11.5671105274568));
#283199=CARTESIAN_POINT('Ctrl Pts',(7.51676407774739,96.5749999996238,10.3459381770588));
#283200=CARTESIAN_POINT('Ctrl Pts',(9.83957192047848,96.7249999996232,7.14886745759505));
#283201=CARTESIAN_POINT('Ctrl Pts',(12.1623797632096,96.8749999996226,3.95179673813132));
#283202=CARTESIAN_POINT('Ctrl Pts',(12.1623797632096,97.024999999622,-1.48946194470292E-15));
#283203=CARTESIAN_POINT('Ctrl Pts',(12.1623797632096,97.1749999996214,-3.95179673813132));
#283204=CARTESIAN_POINT('Ctrl Pts',(9.83957192047848,97.3249999996208,-7.14886745759505));
#283205=CARTESIAN_POINT('Ctrl Pts',(7.51676407774739,97.4749999996202,-10.3459381770588));
#283206=CARTESIAN_POINT('Ctrl Pts',(3.75838203887366,97.6249999996196,-11.5671105274568));
#283207=CARTESIAN_POINT('Ctrl Pts',(-6.95696045824653E-14,97.774999999619,
-12.7882828778549));
#283208=CARTESIAN_POINT('Ctrl Pts',(-3.7583820388738,97.9249999996184,-11.5671105274568));
#283209=CARTESIAN_POINT('Ctrl Pts',(-7.51676407774752,98.0749999996178,
-10.3459381770588));
#283210=CARTESIAN_POINT('Ctrl Pts',(-9.83957192047862,98.2249999996172,
-7.14886745759505));
#283211=CARTESIAN_POINT('Ctrl Pts',(-12.1623797632097,98.3749999996166,
-3.95179673813132));
#283212=CARTESIAN_POINT('Ctrl Pts',(-12.1623797632097,98.524999999616,2.97892388940585E-15));
#283213=CARTESIAN_POINT('Ctrl Pts',(-12.1623797632097,98.6749999996154,
3.95179673813133));
#283214=CARTESIAN_POINT('Ctrl Pts',(-9.83957192047862,98.8249999996148,
7.14886745759505));
#283215=CARTESIAN_POINT('Ctrl Pts',(-7.51676407774752,98.9749999996142,
10.3459381770588));
#283216=CARTESIAN_POINT('Ctrl Pts',(-3.7583820388738,99.1249999996136,11.5671105274568));
#283217=CARTESIAN_POINT('Ctrl Pts',(-6.7301233279705E-14,99.274999999613,
12.7882828778549));
#283218=CARTESIAN_POINT('Ctrl Pts',(3.75838203887366,99.4249999996124,11.5671105274568));
#283219=CARTESIAN_POINT('Ctrl Pts',(7.51676407774739,99.5749999996118,10.3459381770588));
#283220=CARTESIAN_POINT('Ctrl Pts',(9.83957192047848,99.7249999996112,7.14886745759505));
#283221=CARTESIAN_POINT('Ctrl Pts',(12.1623797632096,99.8749999996106,3.95179673813132));
#283222=CARTESIAN_POINT('Ctrl Pts',(12.1623797632096,100.02499999961,-1.48946194470292E-15));
#283223=CARTESIAN_POINT('Ctrl Pts',(12.1623797632096,100.174999999609,-3.95179673813132));
#283224=CARTESIAN_POINT('Ctrl Pts',(9.83957192047848,100.324999999609,-7.14886745759505));
#283225=CARTESIAN_POINT('Ctrl Pts',(7.51676407774738,100.474999999608,-10.3459381770588));
#283226=CARTESIAN_POINT('Ctrl Pts',(3.75838203887366,100.624999999608,-11.5671105274568));
#283227=CARTESIAN_POINT('Ctrl Pts',(-7.12973138541271E-14,100.774999999607,
-12.7882828778549));
#283228=CARTESIAN_POINT('Ctrl Pts',(-3.7583820388738,100.924999999606,-11.5671105274568));
#283229=CARTESIAN_POINT('Ctrl Pts',(-7.51676407774753,101.074999999606,
-10.3459381770588));
#283230=CARTESIAN_POINT('Ctrl Pts',(-9.83957192047862,101.224999999605,
-7.14886745759505));
#283231=CARTESIAN_POINT('Ctrl Pts',(-12.1623797632097,101.374999999605,
-3.95179673813132));
#283232=CARTESIAN_POINT('Ctrl Pts',(-12.1623797632097,101.524999999604,
2.97892388940585E-15));
#283233=CARTESIAN_POINT('Ctrl Pts',(-12.1623797632097,101.674999999603,
3.95179673813133));
#283234=CARTESIAN_POINT('Ctrl Pts',(-9.83957192047862,101.824999999603,
7.14886745759505));
#283235=CARTESIAN_POINT('Ctrl Pts',(-7.51676407774752,101.974999999602,
10.3459381770588));
#283236=CARTESIAN_POINT('Ctrl Pts',(-3.7583820388738,102.124999999602,11.5671105274568));
#283237=CARTESIAN_POINT('Ctrl Pts',(-6.90289425513669E-14,102.274999999601,
12.7882828778549));
#283238=CARTESIAN_POINT('Ctrl Pts',(3.75838203887366,102.4249999996,11.5671105274568));
#283239=CARTESIAN_POINT('Ctrl Pts',(7.51676407774739,102.5749999996,10.3459381770588));
#283240=CARTESIAN_POINT('Ctrl Pts',(9.83957192047848,102.724999999599,7.14886745759505));
#283241=CARTESIAN_POINT('Ctrl Pts',(12.1623797632096,102.874999999599,3.95179673813132));
#283242=CARTESIAN_POINT('Ctrl Pts',(12.1623797632096,103.024999999598,-1.48946194470292E-15));
#283243=CARTESIAN_POINT('Ctrl Pts',(12.1623797632096,103.174999999597,-3.95179673813132));
#283244=CARTESIAN_POINT('Ctrl Pts',(9.83957192047848,103.324999999597,-7.14886745759505));
#283245=CARTESIAN_POINT('Ctrl Pts',(7.51676407774738,103.474999999596,-10.3459381770588));
#283246=CARTESIAN_POINT('Ctrl Pts',(3.75838203887366,103.624999999596,-11.5671105274568));
#283247=CARTESIAN_POINT('Ctrl Pts',(-7.3025023125789E-14,103.774999999595,
-12.7882828778549));
#283248=CARTESIAN_POINT('Ctrl Pts',(-3.7583820388738,103.924999999594,-11.5671105274568));
#283249=CARTESIAN_POINT('Ctrl Pts',(-7.51676407774753,104.074999999594,
-10.3459381770588));
#283250=CARTESIAN_POINT('Ctrl Pts',(-9.83957192047862,104.224999999593,
-7.14886745759505));
#283251=CARTESIAN_POINT('Ctrl Pts',(-12.1623797632097,104.374999999593,
-3.95179673813132));
#283252=CARTESIAN_POINT('Ctrl Pts',(-12.1623797632097,104.524999999592,
2.97892388940585E-15));
#283253=CARTESIAN_POINT('Ctrl Pts',(-12.1623797632097,104.674999999591,
3.95179673813133));
#283254=CARTESIAN_POINT('Ctrl Pts',(-9.83957192047862,104.824999999591,
7.14886745759505));
#283255=CARTESIAN_POINT('Ctrl Pts',(-7.51676407774753,104.97499999959,10.3459381770588));
#283256=CARTESIAN_POINT('Ctrl Pts',(-3.7583820388738,105.12499999959,11.5671105274568));
#283257=CARTESIAN_POINT('Ctrl Pts',(-7.07566518230287E-14,105.274999999589,
12.7882828778549));
#283258=CARTESIAN_POINT('Ctrl Pts',(3.75838203887366,105.424999999588,11.5671105274568));
#283259=CARTESIAN_POINT('Ctrl Pts',(7.51676407774738,105.574999999588,10.3459381770588));
#283260=CARTESIAN_POINT('Ctrl Pts',(9.83957192047848,105.724999999587,7.14886745759505));
#283261=CARTESIAN_POINT('Ctrl Pts',(12.1623797632096,105.874999999587,3.95179673813132));
#283262=CARTESIAN_POINT('Ctrl Pts',(12.1623797632096,106.024999999586,-1.48946194470292E-15));
#283263=CARTESIAN_POINT('Ctrl Pts',(12.1623797632096,106.174999999585,-3.95179673813132));
#283264=CARTESIAN_POINT('Ctrl Pts',(9.83957192047848,106.324999999585,-7.14886745759505));
#283265=CARTESIAN_POINT('Ctrl Pts',(7.51676407774738,106.474999999584,-10.3459381770588));
#283266=CARTESIAN_POINT('Ctrl Pts',(3.75838203887365,106.624999999584,-11.5671105274568));
#283267=CARTESIAN_POINT('Ctrl Pts',(-7.47527323974508E-14,106.774999999583,
-12.7882828778549));
#283268=CARTESIAN_POINT('Ctrl Pts',(-3.7583820388738,106.924999999582,-11.5671105274568));
#283269=CARTESIAN_POINT('Ctrl Pts',(-7.51676407774753,107.074999999582,
-10.3459381770588));
#283270=CARTESIAN_POINT('Ctrl Pts',(-9.83957192047862,107.224999999581,
-7.14886745759505));
#283271=CARTESIAN_POINT('Ctrl Pts',(-12.1623797632097,107.374999999581,
-3.95179673813132));
#283272=CARTESIAN_POINT('Ctrl Pts',(-12.1623797632097,107.52499999958,2.97892388940585E-15));
#283273=CARTESIAN_POINT('Ctrl Pts',(-12.1623797632097,107.674999999579,
3.95179673813133));
#283274=CARTESIAN_POINT('Ctrl Pts',(-9.83957192047862,107.824999999579,
7.14886745759505));
#283275=CARTESIAN_POINT('Ctrl Pts',(-7.51676407774753,107.974999999578,
10.3459381770588));
#283276=CARTESIAN_POINT('Ctrl Pts',(-3.7583820388738,108.124999999578,11.5671105274568));
#283277=CARTESIAN_POINT('Ctrl Pts',(-7.24843610946905E-14,108.274999999577,
12.7882828778549));
#283278=CARTESIAN_POINT('Ctrl Pts',(3.75838203887366,108.424999999576,11.5671105274568));
#283279=CARTESIAN_POINT('Ctrl Pts',(7.51676407774738,108.574999999576,10.3459381770588));
#283280=CARTESIAN_POINT('Ctrl Pts',(9.83957192047847,108.724999999575,7.14886745759505));
#283281=CARTESIAN_POINT('Ctrl Pts',(12.1623797632096,108.874999999575,3.95179673813132));
#283282=CARTESIAN_POINT('Ctrl Pts',(12.1623797632096,109.024999999574,-1.48946194470292E-15));
#283283=CARTESIAN_POINT('Ctrl Pts',(12.1623797632096,109.174999999573,-3.95179673813132));
#283284=CARTESIAN_POINT('Ctrl Pts',(9.83957192047847,109.324999999573,-7.14886745759505));
#283285=CARTESIAN_POINT('Ctrl Pts',(7.51676407774738,109.474999999572,-10.3459381770588));
#283286=CARTESIAN_POINT('Ctrl Pts',(3.75838203887365,109.624999999572,-11.5671105274568));
#283287=CARTESIAN_POINT('Ctrl Pts',(-7.64804416691126E-14,109.774999999571,
-12.7882828778549));
#283288=CARTESIAN_POINT('Ctrl Pts',(-3.7583820388738,109.92499999957,-11.5671105274568));
#283289=CARTESIAN_POINT('Ctrl Pts',(-7.51676407774753,110.07499999957,-10.3459381770588));
#283290=CARTESIAN_POINT('Ctrl Pts',(-9.83957192047862,110.224999999569,
-7.14886745759505));
#283291=CARTESIAN_POINT('Ctrl Pts',(-12.1623797632097,110.374999999569,
-3.95179673813132));
#283292=CARTESIAN_POINT('Ctrl Pts',(-12.1623797632097,110.524999999568,
2.97892388940585E-15));
#283293=CARTESIAN_POINT('Ctrl Pts',(-12.1623797632097,110.674999999567,
3.95179673813133));
#283294=CARTESIAN_POINT('Ctrl Pts',(-9.83957192047862,110.824999999567,
7.14886745759505));
#283295=CARTESIAN_POINT('Ctrl Pts',(-7.51676407774753,110.974999999566,
10.3459381770588));
#283296=CARTESIAN_POINT('Ctrl Pts',(-3.7583820388738,111.124999999566,11.5671105274568));
#283297=CARTESIAN_POINT('Ctrl Pts',(-7.42120703663524E-14,111.274999999565,
12.7882828778549));
#283298=CARTESIAN_POINT('Ctrl Pts',(3.75838203887365,111.424999999564,11.5671105274568));
#283299=CARTESIAN_POINT('Ctrl Pts',(7.51676407774738,111.574999999564,10.3459381770588));
#283300=CARTESIAN_POINT('Ctrl Pts',(9.83957192047847,111.724999999563,7.14886745759505));
#283301=CARTESIAN_POINT('Ctrl Pts',(12.1623797632096,111.874999999563,3.95179673813132));
#283302=CARTESIAN_POINT('Ctrl Pts',(12.1623797632096,112.024999999562,-1.48946194470292E-15));
#283303=CARTESIAN_POINT('Ctrl Pts',(12.1623797632096,112.174999999561,-3.95179673813132));
#283304=CARTESIAN_POINT('Ctrl Pts',(9.83957192047847,112.324999999561,-7.14886745759505));
#283305=CARTESIAN_POINT('Ctrl Pts',(7.51676407774738,112.47499999956,-10.3459381770588));
#283306=CARTESIAN_POINT('Ctrl Pts',(3.75838203887365,112.62499999956,-11.5671105274568));
#283307=CARTESIAN_POINT('Ctrl Pts',(-7.82081509407745E-14,112.774999999559,
-12.7882828778549));
#283308=CARTESIAN_POINT('Ctrl Pts',(-3.75838203887381,112.924999999558,
-11.5671105274568));
#283309=CARTESIAN_POINT('Ctrl Pts',(-7.51676407774753,113.074999999558,
-10.3459381770588));
#283310=CARTESIAN_POINT('Ctrl Pts',(-9.83957192047863,113.224999999557,
-7.14886745759505));
#283311=CARTESIAN_POINT('Ctrl Pts',(-12.1623797632097,113.374999999557,
-3.95179673813132));
#283312=CARTESIAN_POINT('Ctrl Pts',(-12.1623797632097,113.524999999556,
2.97892388940585E-15));
#283313=CARTESIAN_POINT('Ctrl Pts',(-12.1623797632097,113.674999999555,
3.95179673813133));
#283314=CARTESIAN_POINT('Ctrl Pts',(-9.83957192047863,113.824999999555,
7.14886745759505));
#283315=CARTESIAN_POINT('Ctrl Pts',(-7.51676407774753,113.974999999554,
10.3459381770588));
#283316=CARTESIAN_POINT('Ctrl Pts',(-3.7583820388738,114.124999999554,11.5671105274568));
#283317=CARTESIAN_POINT('Ctrl Pts',(-7.59397796380142E-14,114.274999999553,
12.7882828778549));
#283318=CARTESIAN_POINT('Ctrl Pts',(3.75838203887365,114.424999999552,11.5671105274568));
#283319=CARTESIAN_POINT('Ctrl Pts',(7.51676407774738,114.574999999552,10.3459381770588));
#283320=CARTESIAN_POINT('Ctrl Pts',(9.83957192047847,114.724999999551,7.14886745759505));
#283321=CARTESIAN_POINT('Ctrl Pts',(12.1623797632096,114.874999999551,3.95179673813132));
#283322=CARTESIAN_POINT('Ctrl Pts',(12.1623797632096,115.02499999955,-1.48946194470292E-15));
#283323=CARTESIAN_POINT('Ctrl Pts',(12.1623797632096,115.174999999549,-3.95179673813132));
#283324=CARTESIAN_POINT('Ctrl Pts',(9.83957192047847,115.324999999549,-7.14886745759505));
#283325=CARTESIAN_POINT('Ctrl Pts',(7.51676407774738,115.474999999548,-10.3459381770588));
#283326=CARTESIAN_POINT('Ctrl Pts',(3.75838203887365,115.624999999548,-11.5671105274568));
#283327=CARTESIAN_POINT('Ctrl Pts',(-7.99358602124363E-14,115.774999999547,
-12.7882828778549));
#283328=CARTESIAN_POINT('Ctrl Pts',(-3.75838203887381,115.924999999546,
-11.5671105274568));
#283329=CARTESIAN_POINT('Ctrl Pts',(-7.51676407774754,116.074999999546,
-10.3459381770588));
#283330=CARTESIAN_POINT('Ctrl Pts',(-9.83957192047863,116.224999999545,
-7.14886745759505));
#283331=CARTESIAN_POINT('Ctrl Pts',(-12.1623797632097,116.374999999545,
-3.95179673813132));
#283332=CARTESIAN_POINT('Ctrl Pts',(-12.1623797632097,116.524999999544,
2.97892388940585E-15));
#283333=CARTESIAN_POINT('Ctrl Pts',(-12.1623797632097,116.674999999543,
3.95179673813133));
#283334=CARTESIAN_POINT('Ctrl Pts',(-9.83957192047863,116.824999999543,
7.14886745759505));
#283335=CARTESIAN_POINT('Ctrl Pts',(-7.51676407774753,116.974999999542,
10.3459381770588));
#283336=CARTESIAN_POINT('Ctrl Pts',(-3.75838203887381,117.124999999542,
11.5671105274568));
#283337=CARTESIAN_POINT('Ctrl Pts',(-7.76674889096761E-14,117.274999999541,
12.7882828778549));
#283338=CARTESIAN_POINT('Ctrl Pts',(3.75838203887365,117.42499999954,11.5671105274568));
#283339=CARTESIAN_POINT('Ctrl Pts',(7.51676407774738,117.57499999954,10.3459381770588));
#283340=CARTESIAN_POINT('Ctrl Pts',(9.83957192047847,117.724999999539,7.14886745759505));
#283341=CARTESIAN_POINT('Ctrl Pts',(12.1623797632096,117.874999999539,3.95179673813132));
#283342=CARTESIAN_POINT('Ctrl Pts',(12.1623797632096,118.024999999538,-1.48946194470292E-15));
#283343=CARTESIAN_POINT('Ctrl Pts',(12.1623797632096,118.174999999537,-3.95179673813132));
#283344=CARTESIAN_POINT('Ctrl Pts',(9.83957192047847,118.324999999537,-7.14886745759505));
#283345=CARTESIAN_POINT('Ctrl Pts',(7.51676407774737,118.474999999536,-10.3459381770588));
#283346=CARTESIAN_POINT('Ctrl Pts',(3.75838203887365,118.624999999536,-11.5671105274568));
#283347=CARTESIAN_POINT('Ctrl Pts',(-8.16635694840981E-14,118.774999999535,
-12.7882828778549));
#283348=CARTESIAN_POINT('Ctrl Pts',(-3.75838203887381,118.924999999534,
-11.5671105274568));
#283349=CARTESIAN_POINT('Ctrl Pts',(-7.51676407774754,119.074999999534,
-10.3459381770588));
#283350=CARTESIAN_POINT('Ctrl Pts',(-9.83957192047863,119.224999999533,
-7.14886745759505));
#283351=CARTESIAN_POINT('Ctrl Pts',(-12.1623797632097,119.374999999533,
-3.95179673813132));
#283352=CARTESIAN_POINT('Ctrl Pts',(-12.1623797632097,119.524999999532,
2.97892388940585E-15));
#283353=CARTESIAN_POINT('Ctrl Pts',(-12.1623797632097,119.674999999531,
3.95179673813133));
#283354=CARTESIAN_POINT('Ctrl Pts',(-9.83957192047863,119.824999999531,
7.14886745759505));
#283355=CARTESIAN_POINT('Ctrl Pts',(-7.51676407774754,119.97499999953,10.3459381770588));
#283356=CARTESIAN_POINT('Ctrl Pts',(-3.75838203887381,120.12499999953,11.5671105274568));
#283357=CARTESIAN_POINT('Ctrl Pts',(-7.93951981813379E-14,120.274999999529,
12.7882828778549));
#283358=CARTESIAN_POINT('Ctrl Pts',(3.75838203887365,120.424999999528,11.5671105274568));
#283359=CARTESIAN_POINT('Ctrl Pts',(7.51676407774738,120.574999999528,10.3459381770588));
#283360=CARTESIAN_POINT('Ctrl Pts',(9.83957192047847,120.724999999527,7.14886745759505));
#283361=CARTESIAN_POINT('Ctrl Pts',(12.1623797632096,120.874999999527,3.95179673813132));
#283362=CARTESIAN_POINT('Ctrl Pts',(12.1623797632096,121.024999999526,-1.48946194470292E-15));
#283363=CARTESIAN_POINT('Ctrl Pts',(12.1623797632096,121.174999999525,-3.95179673813132));
#283364=CARTESIAN_POINT('Ctrl Pts',(9.83957192047847,121.324999999525,-7.14886745759505));
#283365=CARTESIAN_POINT('Ctrl Pts',(7.51676407774737,121.474999999524,-10.3459381770588));
#283366=CARTESIAN_POINT('Ctrl Pts',(3.75838203887364,121.624999999524,-11.5671105274568));
#283367=CARTESIAN_POINT('Ctrl Pts',(-8.339127875576E-14,121.774999999523,
-12.7882828778549));
#283368=CARTESIAN_POINT('Ctrl Pts',(-3.75838203887381,121.924999999522,
-11.5671105274568));
#283369=CARTESIAN_POINT('Ctrl Pts',(-7.51676407774754,122.074999999522,
-10.3459381770588));
#283370=CARTESIAN_POINT('Ctrl Pts',(-9.83957192047863,122.224999999521,
-7.14886745759505));
#283371=CARTESIAN_POINT('Ctrl Pts',(-12.1623797632097,122.374999999521,
-3.95179673813132));
#283372=CARTESIAN_POINT('Ctrl Pts',(-12.1623797632097,122.52499999952,2.97892388940585E-15));
#283373=CARTESIAN_POINT('Ctrl Pts',(-12.1623797632097,122.674999999519,
3.95179673813133));
#283374=CARTESIAN_POINT('Ctrl Pts',(-9.83957192047863,122.824999999519,
7.14886745759505));
#283375=CARTESIAN_POINT('Ctrl Pts',(-7.51676407774754,122.974999999518,
10.3459381770588));
#283376=CARTESIAN_POINT('Ctrl Pts',(-3.75838203887381,123.124999999518,
11.5671105274568));
#283377=CARTESIAN_POINT('Ctrl Pts',(-8.11229074529997E-14,123.274999999517,
12.7882828778549));
#283378=CARTESIAN_POINT('Ctrl Pts',(3.75838203887365,123.424999999516,11.5671105274568));
#283379=CARTESIAN_POINT('Ctrl Pts',(7.51676407774737,123.574999999516,10.3459381770588));
#283380=CARTESIAN_POINT('Ctrl Pts',(9.83957192047846,123.724999999515,7.14886745759505));
#283381=CARTESIAN_POINT('Ctrl Pts',(12.1623797632096,123.874999999515,3.95179673813132));
#283382=CARTESIAN_POINT('Ctrl Pts',(12.1623797632096,124.024999999514,-1.48946194470292E-15));
#283383=CARTESIAN_POINT('Ctrl Pts',(12.1623797632096,124.174999999513,-3.95179673813132));
#283384=CARTESIAN_POINT('Ctrl Pts',(9.83957192047846,124.324999999513,-7.14886745759505));
#283385=CARTESIAN_POINT('Ctrl Pts',(7.51676407774737,124.474999999512,-10.3459381770588));
#283386=CARTESIAN_POINT('Ctrl Pts',(3.75838203887364,124.624999999512,-11.5671105274568));
#283387=CARTESIAN_POINT('Ctrl Pts',(-8.51189880274219E-14,124.774999999511,
-12.7882828778549));
#283388=CARTESIAN_POINT('Ctrl Pts',(-3.75838203887381,124.92499999951,-11.5671105274568));
#283389=CARTESIAN_POINT('Ctrl Pts',(-7.51676407774754,125.07499999951,-10.3459381770588));
#283390=CARTESIAN_POINT('Ctrl Pts',(-9.83957192047863,125.224999999509,
-7.14886745759505));
#283391=CARTESIAN_POINT('Ctrl Pts',(-12.1623797632097,125.374999999509,
-3.95179673813132));
#283392=CARTESIAN_POINT('Ctrl Pts',(-12.1623797632097,125.524999999508,
2.97892388940585E-15));
#283393=CARTESIAN_POINT('Ctrl Pts',(-12.1623797632097,125.674999999507,
3.95179673813133));
#283394=CARTESIAN_POINT('Ctrl Pts',(-9.83957192047863,125.824999999507,
7.14886745759505));
#283395=CARTESIAN_POINT('Ctrl Pts',(-7.51676407774754,125.974999999506,
10.3459381770588));
#283396=CARTESIAN_POINT('Ctrl Pts',(-3.75838203887381,126.124999999506,
11.5671105274568));
#283397=CARTESIAN_POINT('Ctrl Pts',(-8.28506167246616E-14,126.274999999505,
12.7882828778549));
#283398=CARTESIAN_POINT('Ctrl Pts',(3.75838203887364,126.424999999504,11.5671105274568));
#283399=CARTESIAN_POINT('Ctrl Pts',(7.51676407774737,126.574999999504,10.3459381770588));
#283400=CARTESIAN_POINT('Ctrl Pts',(9.83957192047846,126.724999999503,7.14886745759505));
#283401=CARTESIAN_POINT('Ctrl Pts',(12.1623797632096,126.874999999503,3.95179673813132));
#283402=CARTESIAN_POINT('Ctrl Pts',(12.1623797632096,127.024999999502,-1.48946194470292E-15));
#283403=CARTESIAN_POINT('Ctrl Pts',(12.1623797632096,127.174999999501,-3.95179673813132));
#283404=CARTESIAN_POINT('Ctrl Pts',(9.83957192047846,127.324999999501,-7.14886745759505));
#283405=CARTESIAN_POINT('Ctrl Pts',(7.51676407774737,127.4749999995,-10.3459381770588));
#283406=CARTESIAN_POINT('Ctrl Pts',(3.75838203887364,127.6249999995,-11.5671105274568));
#283407=CARTESIAN_POINT('Ctrl Pts',(-8.68466972990837E-14,127.774999999499,
-12.7882828778549));
#283408=CARTESIAN_POINT('Ctrl Pts',(-3.75838203887381,127.924999999498,
-11.5671105274568));
#283409=CARTESIAN_POINT('Ctrl Pts',(-7.51676407774754,128.074999999498,
-10.3459381770588));
#283410=CARTESIAN_POINT('Ctrl Pts',(-9.83957192047864,128.224999999497,
-7.14886745759505));
#283411=CARTESIAN_POINT('Ctrl Pts',(-12.1623797632097,128.374999999497,
-3.95179673813132));
#283412=CARTESIAN_POINT('Ctrl Pts',(-12.1623797632097,128.524999999496,
2.97892388940585E-15));
#283413=CARTESIAN_POINT('Ctrl Pts',(-12.1623797632097,128.674999999495,
3.95179673813133));
#283414=CARTESIAN_POINT('Ctrl Pts',(-9.83957192047864,128.824999999495,
7.14886745759505));
#283415=CARTESIAN_POINT('Ctrl Pts',(-7.51676407774754,128.974999999494,
10.3459381770588));
#283416=CARTESIAN_POINT('Ctrl Pts',(-3.75838203887381,129.124999999494,
11.5671105274568));
#283417=CARTESIAN_POINT('Ctrl Pts',(-8.45783259963234E-14,129.274999999493,
12.7882828778549));
#283418=CARTESIAN_POINT('Ctrl Pts',(3.75838203887364,129.424999999492,11.5671105274568));
#283419=CARTESIAN_POINT('Ctrl Pts',(7.51676407774737,129.574999999492,10.3459381770588));
#283420=CARTESIAN_POINT('Ctrl Pts',(9.83957192047846,129.724999999491,7.14886745759505));
#283421=CARTESIAN_POINT('Ctrl Pts',(12.1623797632096,129.874999999491,3.95179673813132));
#283422=CARTESIAN_POINT('Ctrl Pts',(12.1623797632096,130.02499999949,-1.48946194470292E-15));
#283423=CARTESIAN_POINT('Ctrl Pts',(12.1623797632096,130.174999999489,-3.95179673813132));
#283424=CARTESIAN_POINT('Ctrl Pts',(9.83957192047846,130.324999999489,-7.14886745759505));
#283425=CARTESIAN_POINT('Ctrl Pts',(7.51676407774737,130.474999999488,-10.3459381770588));
#283426=CARTESIAN_POINT('Ctrl Pts',(3.75838203887364,130.624999999488,-11.5671105274568));
#283427=CARTESIAN_POINT('Ctrl Pts',(-8.85744065707455E-14,130.774999999487,
-12.7882828778549));
#283428=CARTESIAN_POINT('Ctrl Pts',(-3.75838203887382,130.924999999486,
-11.5671105274568));
#283429=CARTESIAN_POINT('Ctrl Pts',(-7.51676407774754,131.074999999486,
-10.3459381770588));
#283430=CARTESIAN_POINT('Ctrl Pts',(-9.83957192047864,131.224999999485,
-7.14886745759505));
#283431=CARTESIAN_POINT('Ctrl Pts',(-12.1623797632097,131.374999999485,
-3.95179673813132));
#283432=CARTESIAN_POINT('Ctrl Pts',(-12.1623797632097,131.524999999484,
2.97892388940585E-15));
#283433=CARTESIAN_POINT('Ctrl Pts',(-12.1623797632097,131.674999999483,
3.95179673813133));
#283434=CARTESIAN_POINT('Ctrl Pts',(-9.83957192047864,131.824999999483,
7.14886745759505));
#283435=CARTESIAN_POINT('Ctrl Pts',(-7.51676407774754,131.974999999482,
10.3459381770588));
#283436=CARTESIAN_POINT('Ctrl Pts',(-3.75838203887381,132.124999999482,
11.5671105274568));
#283437=CARTESIAN_POINT('Ctrl Pts',(-8.63060352679853E-14,132.274999999481,
12.7882828778549));
#283438=CARTESIAN_POINT('Ctrl Pts',(3.75838203887364,132.42499999948,11.5671105274568));
#283439=CARTESIAN_POINT('Ctrl Pts',(7.51676407774737,132.57499999948,10.3459381770588));
#283440=CARTESIAN_POINT('Ctrl Pts',(9.83957192047846,132.724999999479,7.14886745759505));
#283441=CARTESIAN_POINT('Ctrl Pts',(12.1623797632096,132.874999999479,3.95179673813132));
#283442=CARTESIAN_POINT('Ctrl Pts',(12.1623797632096,133.024999999478,-1.48946194470292E-15));
#283443=CARTESIAN_POINT('Ctrl Pts',(12.1623797632096,133.174999999477,-3.95179673813132));
#283444=CARTESIAN_POINT('Ctrl Pts',(9.83957192047846,133.324999999477,-7.14886745759505));
#283445=CARTESIAN_POINT('Ctrl Pts',(7.51676407774736,133.474999999476,-10.3459381770588));
#283446=CARTESIAN_POINT('Ctrl Pts',(3.75838203887364,133.624999999476,-11.5671105274568));
#283447=CARTESIAN_POINT('Ctrl Pts',(-9.03021158424074E-14,133.774999999475,
-12.7882828778549));
#283448=CARTESIAN_POINT('Ctrl Pts',(-3.75838203887382,133.924999999474,
-11.5671105274568));
#283449=CARTESIAN_POINT('Ctrl Pts',(-7.51676407774755,134.074999999474,
-10.3459381770588));
#283450=CARTESIAN_POINT('Ctrl Pts',(-9.83957192047864,134.224999999473,
-7.14886745759505));
#283451=CARTESIAN_POINT('Ctrl Pts',(-12.1623797632097,134.374999999473,
-3.95179673813132));
#283452=CARTESIAN_POINT('Ctrl Pts',(-12.1623797632097,134.524999999472,
2.97892388940585E-15));
#283453=CARTESIAN_POINT('Ctrl Pts',(-12.1623797632097,134.674999999471,
3.95179673813133));
#283454=CARTESIAN_POINT('Ctrl Pts',(-9.83957192047864,134.824999999471,
7.14886745759505));
#283455=CARTESIAN_POINT('Ctrl Pts',(-7.51676407774754,134.97499999947,10.3459381770588));
#283456=CARTESIAN_POINT('Ctrl Pts',(-3.75838203887382,135.12499999947,11.5671105274568));
#283457=CARTESIAN_POINT('Ctrl Pts',(-8.80337445396471E-14,135.274999999469,
12.7882828778549));
#283458=CARTESIAN_POINT('Ctrl Pts',(3.75838203887364,135.424999999468,11.5671105274568));
#283459=CARTESIAN_POINT('Ctrl Pts',(7.51676407774737,135.574999999468,10.3459381770588));
#283460=CARTESIAN_POINT('Ctrl Pts',(9.83957192047846,135.724999999467,7.14886745759505));
#283461=CARTESIAN_POINT('Ctrl Pts',(12.1623797632096,135.874999999467,3.95179673813132));
#283462=CARTESIAN_POINT('Ctrl Pts',(12.1623797632096,136.024999999466,-1.48946194470292E-15));
#283463=CARTESIAN_POINT('Ctrl Pts',(12.1623797632095,136.174999999465,-3.95179673813132));
#283464=CARTESIAN_POINT('Ctrl Pts',(9.83957192047846,136.324999999465,-7.14886745759505));
#283465=CARTESIAN_POINT('Ctrl Pts',(7.51676407774736,136.474999999464,-10.3459381770588));
#283466=CARTESIAN_POINT('Ctrl Pts',(3.75838203887364,136.624999999464,-11.5671105274568));
#283467=CARTESIAN_POINT('Ctrl Pts',(-9.20298251140692E-14,136.774999999463,
-12.7882828778549));
#283468=CARTESIAN_POINT('Ctrl Pts',(-3.75838203887382,136.924999999462,
-11.5671105274568));
#283469=CARTESIAN_POINT('Ctrl Pts',(-7.51676407774755,137.074999999462,
-10.3459381770588));
#283470=CARTESIAN_POINT('Ctrl Pts',(-9.83957192047864,137.224999999461,
-7.14886745759505));
#283471=CARTESIAN_POINT('Ctrl Pts',(-12.1623797632097,137.374999999461,
-3.95179673813132));
#283472=CARTESIAN_POINT('Ctrl Pts',(-12.1623797632097,137.52499999946,2.97892388940585E-15));
#283473=CARTESIAN_POINT('Ctrl Pts',(-12.1623797632097,137.674999999459,
3.95179673813133));
#283474=CARTESIAN_POINT('Ctrl Pts',(-9.83957192047864,137.824999999459,
7.14886745759505));
#283475=CARTESIAN_POINT('Ctrl Pts',(-7.51676407774755,137.974999999458,
10.3459381770588));
#283476=CARTESIAN_POINT('Ctrl Pts',(-3.75838203887382,138.124999999458,
11.5671105274568));
#283477=CARTESIAN_POINT('Ctrl Pts',(-8.97614538113089E-14,138.274999999457,
12.7882828778549));
#283478=CARTESIAN_POINT('Ctrl Pts',(3.75838203887364,138.424999999456,11.5671105274568));
#283479=CARTESIAN_POINT('Ctrl Pts',(7.51676407774736,138.574999999456,10.3459381770588));
#283480=CARTESIAN_POINT('Ctrl Pts',(9.83957192047846,138.724999999455,7.14886745759505));
#283481=CARTESIAN_POINT('Ctrl Pts',(12.1623797632096,138.874999999455,3.95179673813132));
#283482=CARTESIAN_POINT('Ctrl Pts',(12.1623797632096,139.024999999454,-1.48946194470292E-15));
#283483=CARTESIAN_POINT('Ctrl Pts',(12.1623797632095,139.174999999453,-3.95179673813132));
#283484=CARTESIAN_POINT('Ctrl Pts',(9.83957192047846,139.324999999453,-7.14886745759505));
#283485=CARTESIAN_POINT('Ctrl Pts',(7.51676407774736,139.474999999452,-10.3459381770588));
#283486=CARTESIAN_POINT('Ctrl Pts',(3.75838203887363,139.624999999452,-11.5671105274568));
#283487=CARTESIAN_POINT('Ctrl Pts',(-9.3757534385731E-14,139.774999999451,
-12.7882828778549));
#283488=CARTESIAN_POINT('Ctrl Pts',(-3.75838203887382,139.92499999945,-11.5671105274568));
#283489=CARTESIAN_POINT('Ctrl Pts',(-7.51676407774755,140.07499999945,-10.3459381770588));
#283490=CARTESIAN_POINT('Ctrl Pts',(-9.83957192047864,140.224999999449,
-7.14886745759505));
#283491=CARTESIAN_POINT('Ctrl Pts',(-12.1623797632097,140.374999999449,
-3.95179673813132));
#283492=CARTESIAN_POINT('Ctrl Pts',(-12.1623797632097,140.524999999448,
2.97892388940585E-15));
#283493=CARTESIAN_POINT('Ctrl Pts',(-12.1623797632097,140.674999999447,
3.95179673813133));
#283494=CARTESIAN_POINT('Ctrl Pts',(-9.83957192047864,140.824999999447,
7.14886745759505));
#283495=CARTESIAN_POINT('Ctrl Pts',(-7.51676407774755,140.974999999446,
10.3459381770588));
#283496=CARTESIAN_POINT('Ctrl Pts',(-3.75838203887382,141.124999999446,
11.5671105274568));
#283497=CARTESIAN_POINT('Ctrl Pts',(-9.14891630829708E-14,141.274999999445,
12.7882828778549));
#283498=CARTESIAN_POINT('Ctrl Pts',(3.75838203887364,141.424999999444,11.5671105274568));
#283499=CARTESIAN_POINT('Ctrl Pts',(7.51676407774736,141.574999999444,10.3459381770588));
#283500=CARTESIAN_POINT('Ctrl Pts',(9.83957192047845,141.724999999443,7.14886745759505));
#283501=CARTESIAN_POINT('Ctrl Pts',(12.1623797632095,141.874999999443,3.95179673813132));
#283502=CARTESIAN_POINT('Ctrl Pts',(12.1623797632095,142.024999999442,-1.48946194470292E-15));
#283503=CARTESIAN_POINT('Ctrl Pts',(12.1623797632095,142.174999999441,-3.95179673813132));
#283504=CARTESIAN_POINT('Ctrl Pts',(9.83957192047845,142.324999999441,-7.14886745759505));
#283505=CARTESIAN_POINT('Ctrl Pts',(7.51676407774736,142.47499999944,-10.3459381770588));
#283506=CARTESIAN_POINT('Ctrl Pts',(3.75838203887363,142.62499999944,-11.5671105274568));
#283507=CARTESIAN_POINT('Ctrl Pts',(-9.54852436573929E-14,142.774999999439,
-12.7882828778549));
#283508=CARTESIAN_POINT('Ctrl Pts',(-3.75838203887382,142.924999999438,
-11.5671105274568));
#283509=CARTESIAN_POINT('Ctrl Pts',(-7.51676407774755,143.074999999438,
-10.3459381770588));
#283510=CARTESIAN_POINT('Ctrl Pts',(-9.83957192047864,143.224999999437,
-7.14886745759505));
#283511=CARTESIAN_POINT('Ctrl Pts',(-12.1623797632097,143.374999999437,
-3.95179673813132));
#283512=CARTESIAN_POINT('Ctrl Pts',(-12.1623797632097,143.524999999436,
2.97892388940585E-15));
#283513=CARTESIAN_POINT('Ctrl Pts',(-12.1623797632097,143.674999999435,
3.95179673813133));
#283514=CARTESIAN_POINT('Ctrl Pts',(-9.83957192047864,143.824999999435,
7.14886745759505));
#283515=CARTESIAN_POINT('Ctrl Pts',(-7.51676407774755,143.974999999434,
10.3459381770588));
#283516=CARTESIAN_POINT('Ctrl Pts',(-3.75838203887382,144.124999999434,
11.5671105274568));
#283517=CARTESIAN_POINT('Ctrl Pts',(-9.32168723546326E-14,144.274999999433,
12.7882828778549));
#283518=CARTESIAN_POINT('Ctrl Pts',(3.75838203887363,144.424999999432,11.5671105274568));
#283519=CARTESIAN_POINT('Ctrl Pts',(7.51676407774736,144.574999999432,10.3459381770588));
#283520=CARTESIAN_POINT('Ctrl Pts',(9.83957192047845,144.724999999431,7.14886745759505));
#283521=CARTESIAN_POINT('Ctrl Pts',(12.1623797632095,144.874999999431,3.95179673813132));
#283522=CARTESIAN_POINT('Ctrl Pts',(12.1623797632095,145.02499999943,-1.48946194470292E-15));
#283523=CARTESIAN_POINT('Ctrl Pts',(12.1623797632095,145.174999999429,-3.95179673813132));
#283524=CARTESIAN_POINT('Ctrl Pts',(9.83957192047845,145.324999999429,-7.14886745759505));
#283525=CARTESIAN_POINT('Ctrl Pts',(7.51676407774736,145.474999999428,-10.3459381770588));
#283526=CARTESIAN_POINT('Ctrl Pts',(3.75838203887363,145.624999999428,-11.5671105274568));
#283527=CARTESIAN_POINT('Ctrl Pts',(-9.72129529290547E-14,145.774999999427,
-12.7882828778549));
#283528=CARTESIAN_POINT('Ctrl Pts',(-3.75838203887382,145.924999999426,
-11.5671105274568));
#283529=CARTESIAN_POINT('Ctrl Pts',(-7.51676407774755,146.074999999426,
-10.3459381770588));
#283530=CARTESIAN_POINT('Ctrl Pts',(-9.83957192047865,146.224999999425,
-7.14886745759505));
#283531=CARTESIAN_POINT('Ctrl Pts',(-12.1623797632097,146.374999999425,
-3.95179673813132));
#283532=CARTESIAN_POINT('Ctrl Pts',(-12.1623797632097,146.524999999424,
2.97892388940585E-15));
#283533=CARTESIAN_POINT('Ctrl Pts',(-12.1623797632097,146.674999999423,
3.95179673813133));
#283534=CARTESIAN_POINT('Ctrl Pts',(-9.83957192047865,146.824999999423,
7.14886745759505));
#283535=CARTESIAN_POINT('Ctrl Pts',(-7.51676407774755,146.974999999422,
10.3459381770588));
#283536=CARTESIAN_POINT('Ctrl Pts',(-3.75838203887382,147.124999999422,
11.5671105274568));
#283537=CARTESIAN_POINT('Ctrl Pts',(-9.49445816262944E-14,147.274999999421,
12.7882828778549));
#283538=CARTESIAN_POINT('Ctrl Pts',(3.75838203887363,147.42499999942,11.5671105274568));
#283539=CARTESIAN_POINT('Ctrl Pts',(7.51676407774736,147.57499999942,10.3459381770588));
#283540=CARTESIAN_POINT('Ctrl Pts',(9.83957192047845,147.724999999419,7.14886745759505));
#283541=CARTESIAN_POINT('Ctrl Pts',(12.1623797632095,147.874999999419,3.95179673813132));
#283542=CARTESIAN_POINT('Ctrl Pts',(12.1623797632095,148.024999999418,-1.48946194470292E-15));
#283543=CARTESIAN_POINT('Ctrl Pts',(12.1623797632095,148.174999999417,-3.95179673813132));
#283544=CARTESIAN_POINT('Ctrl Pts',(9.83957192047845,148.324999999417,-7.14886745759505));
#283545=CARTESIAN_POINT('Ctrl Pts',(7.51676407774736,148.474999999416,-10.3459381770588));
#283546=CARTESIAN_POINT('Ctrl Pts',(3.75838203887363,148.624999999416,-11.5671105274568));
#283547=CARTESIAN_POINT('Ctrl Pts',(-9.89406622007166E-14,148.774999999415,
-12.7882828778549));
#283548=CARTESIAN_POINT('Ctrl Pts',(-3.75838203887383,148.924999999414,
-11.5671105274568));
#283549=CARTESIAN_POINT('Ctrl Pts',(-7.51676407774756,149.074999999414,
-10.3459381770588));
#283550=CARTESIAN_POINT('Ctrl Pts',(-9.83957192047865,149.224999999413,
-7.14886745759505));
#283551=CARTESIAN_POINT('Ctrl Pts',(-12.1623797632097,149.374999999413,
-3.95179673813132));
#283552=CARTESIAN_POINT('Ctrl Pts',(-12.1623797632097,149.524999999412,
2.97892388940585E-15));
#283553=CARTESIAN_POINT('Ctrl Pts',(-12.1623797632097,149.674999999411,
3.95179673813133));
#283554=CARTESIAN_POINT('Ctrl Pts',(-9.83957192047865,149.824999999411,
7.14886745759505));
#283555=CARTESIAN_POINT('Ctrl Pts',(-7.51676407774755,149.97499999941,10.3459381770588));
#283556=CARTESIAN_POINT('Ctrl Pts',(-3.75838203887382,150.12499999941,11.5671105274568));
#283557=CARTESIAN_POINT('Ctrl Pts',(-9.66722908979563E-14,150.274999999409,
12.7882828778549));
#283558=CARTESIAN_POINT('Ctrl Pts',(3.75838203887363,150.424999999408,11.5671105274568));
#283559=CARTESIAN_POINT('Ctrl Pts',(7.51676407774736,150.574999999408,10.3459381770588));
#283560=CARTESIAN_POINT('Ctrl Pts',(9.83957192047845,150.724999999407,7.14886745759505));
#283561=CARTESIAN_POINT('Ctrl Pts',(12.1623797632095,150.874999999407,3.95179673813132));
#283562=CARTESIAN_POINT('Ctrl Pts',(12.1623797632095,151.024999999406,-1.48946194470292E-15));
#283563=CARTESIAN_POINT('Ctrl Pts',(12.1623797632095,151.174999999405,-3.95179673813132));
#283564=CARTESIAN_POINT('Ctrl Pts',(9.83957192047845,151.324999999405,-7.14886745759505));
#283565=CARTESIAN_POINT('Ctrl Pts',(7.51676407774736,151.474999999404,-10.3459381770588));
#283566=CARTESIAN_POINT('Ctrl Pts',(3.75838203887363,151.624999999404,-11.5671105274568));
#283567=CARTESIAN_POINT('Ctrl Pts',(-1.00668371472378E-13,151.774999999403,
-12.7882828778549));
#283568=CARTESIAN_POINT('Ctrl Pts',(-3.75838203887383,151.924999999402,
-11.5671105274568));
#283569=CARTESIAN_POINT('Ctrl Pts',(-7.51676407774756,152.074999999402,
-10.3459381770588));
#283570=CARTESIAN_POINT('Ctrl Pts',(-9.83957192047865,152.224999999401,
-7.14886745759505));
#283571=CARTESIAN_POINT('Ctrl Pts',(-12.1623797632097,152.374999999401,
-3.95179673813132));
#283572=CARTESIAN_POINT('Ctrl Pts',(-12.1623797632097,152.5249999994,2.97892388940585E-15));
#283573=CARTESIAN_POINT('Ctrl Pts',(-12.1623797632097,152.674999999399,
3.95179673813133));
#283574=CARTESIAN_POINT('Ctrl Pts',(-9.83957192047865,152.824999999399,
7.14886745759505));
#283575=CARTESIAN_POINT('Ctrl Pts',(-7.51676407774756,152.974999999398,
10.3459381770588));
#283576=CARTESIAN_POINT('Ctrl Pts',(-3.75838203887383,153.124999999398,
11.5671105274568));
#283577=CARTESIAN_POINT('Ctrl Pts',(-9.84000001696181E-14,153.274999999397,
12.7882828778549));
#283578=CARTESIAN_POINT('Ctrl Pts',(3.75838203887363,153.424999999396,11.5671105274568));
#283579=CARTESIAN_POINT('Ctrl Pts',(7.51676407774736,153.574999999396,10.3459381770588));
#283580=CARTESIAN_POINT('Ctrl Pts',(9.83957192047845,153.724999999395,7.14886745759505));
#283581=CARTESIAN_POINT('Ctrl Pts',(12.1623797632095,153.874999999395,3.95179673813132));
#283582=CARTESIAN_POINT('Ctrl Pts',(12.1623797632095,154.024999999394,-1.48946194470292E-15));
#283583=CARTESIAN_POINT('Ctrl Pts',(12.1623797632095,154.174999999393,-3.95179673813132));
#283584=CARTESIAN_POINT('Ctrl Pts',(9.83957192047845,154.324999999393,-7.14886745759505));
#283585=CARTESIAN_POINT('Ctrl Pts',(7.51676407774735,154.474999999392,-10.3459381770588));
#283586=CARTESIAN_POINT('Ctrl Pts',(3.75838203887363,154.624999999392,-11.5671105274568));
#283587=CARTESIAN_POINT('Ctrl Pts',(-1.0239608074404E-13,154.774999999391,
-12.7882828778549));
#283588=CARTESIAN_POINT('Ctrl Pts',(-3.75838203887383,154.92499999939,-11.5671105274568));
#283589=CARTESIAN_POINT('Ctrl Pts',(10.0514428414942,2.80624999999926,-1.23094673026484E-15));
#283590=CARTESIAN_POINT('Ctrl Pts',(10.0514428414941,2.95624999999866,-3.26591175476071));
#283591=CARTESIAN_POINT('Ctrl Pts',(8.13178807675718,3.10624999999806,-5.90808986649102));
#283592=CARTESIAN_POINT('Ctrl Pts',(6.2121333120202,3.25624999999746,-8.55026797822134));
#283593=CARTESIAN_POINT('Ctrl Pts',(3.10606665601009,3.40624999999685,-9.5594902125713));
#283594=CARTESIAN_POINT('Ctrl Pts',(-1.51728257781496E-14,3.55624999999625,
-10.5687124469213));
#283595=CARTESIAN_POINT('Ctrl Pts',(-3.10606665601012,3.70624999999565,
-9.5594902125713));
#283596=CARTESIAN_POINT('Ctrl Pts',(-6.21213331202023,3.85624999999505,
-8.55026797822134));
#283597=CARTESIAN_POINT('Ctrl Pts',(-8.13178807675721,4.00624999999445,
-5.90808986649102));
#283598=CARTESIAN_POINT('Ctrl Pts',(-10.0514428414942,4.15624999999385,
-3.2659117547607));
#283599=CARTESIAN_POINT('Ctrl Pts',(-10.0514428414942,4.30624999999325,
2.46189346052968E-15));
#283600=CARTESIAN_POINT('Ctrl Pts',(-10.0514428414942,4.45624999999265,
3.26591175476071));
#283601=CARTESIAN_POINT('Ctrl Pts',(-8.13178807675721,4.60624999999205,
5.90808986649102));
#283602=CARTESIAN_POINT('Ctrl Pts',(-6.21213331202023,4.75624999999145,
8.55026797822134));
#283603=CARTESIAN_POINT('Ctrl Pts',(-3.10606665601012,4.90624999999085,
9.5594902125713));
#283604=CARTESIAN_POINT('Ctrl Pts',(-1.34480924401344E-14,5.05624999999025,
10.5687124469213));
#283605=CARTESIAN_POINT('Ctrl Pts',(3.10606665601009,5.20624999998966,9.5594902125713));
#283606=CARTESIAN_POINT('Ctrl Pts',(6.2121333120202,5.35624999998906,8.55026797822134));
#283607=CARTESIAN_POINT('Ctrl Pts',(8.13178807675718,5.50624999998846,5.90808986649102));
#283608=CARTESIAN_POINT('Ctrl Pts',(10.0514428414941,5.65624999998786,3.2659117547607));
#283609=CARTESIAN_POINT('Ctrl Pts',(10.0514428414941,5.80624999998726,-1.23094673026484E-15));
#283610=CARTESIAN_POINT('Ctrl Pts',(-12.1623797632103,-3.28749999997638,
2.97892388940601E-15));
#283611=CARTESIAN_POINT('Ctrl Pts',(-12.1623797632103,-3.13749999997698,
3.95179673813154));
#283612=CARTESIAN_POINT('Ctrl Pts',(-9.83957192047908,-2.98749999997758,
7.14886745759543));
#283613=CARTESIAN_POINT('Ctrl Pts',(-7.51676407774787,-2.83749999997817,
10.3459381770593));
#283614=CARTESIAN_POINT('Ctrl Pts',(-3.75838203887394,-2.68749999997877,
11.5671105274575));
#283615=CARTESIAN_POINT('Ctrl Pts',(-8.66709987268145E-15,-2.53749999997937,
12.7882828778556));
#283616=CARTESIAN_POINT('Ctrl Pts',(3.75838203887392,-2.38749999997997,
11.5671105274575));
#283617=CARTESIAN_POINT('Ctrl Pts',(7.51676407774785,-2.23749999998057,
10.3459381770593));
#283618=CARTESIAN_POINT('Ctrl Pts',(9.83957192047906,-2.08749999998117,
7.14886745759543));
#283619=CARTESIAN_POINT('Ctrl Pts',(12.1623797632103,-1.93749999998176,
3.95179673813153));
#283620=CARTESIAN_POINT('Ctrl Pts',(12.1623797632103,-1.78749999998236,
-1.489461944703E-15));
#283621=CARTESIAN_POINT('Ctrl Pts',(12.1623797632103,-1.63749999998296,
-3.95179673813154));
#283622=CARTESIAN_POINT('Ctrl Pts',(9.83957192047906,-1.48749999998357,
-7.14886745759543));
#283623=CARTESIAN_POINT('Ctrl Pts',(7.51676407774784,-1.33749999998417,
-10.3459381770593));
#283624=CARTESIAN_POINT('Ctrl Pts',(3.75838203887392,-1.18749999998477,
-11.5671105274575));
#283625=CARTESIAN_POINT('Ctrl Pts',(-1.26631804471037E-14,-1.03749999998537,
-12.7882828778556));
#283626=CARTESIAN_POINT('Ctrl Pts',(-3.75838203887394,-0.887499999985973,
-11.5671105274575));
#283627=CARTESIAN_POINT('Ctrl Pts',(-7.51676407774787,-0.737499999986575,
-10.3459381770593));
#283628=CARTESIAN_POINT('Ctrl Pts',(-9.83957192047909,-0.587499999987176,
-7.14886745759543));
#283629=CARTESIAN_POINT('Ctrl Pts',(-12.1623797632103,-0.437499999987778,
-3.95179673813153));
#283630=CARTESIAN_POINT('Ctrl Pts',(-12.1623797632103,-0.287499999988378,
2.97892388940601E-15));
#283631=CARTESIAN_POINT('Ctrl Pts',(-12.1623797632103,-0.137499999988978,
3.95179673813154));
#283632=CARTESIAN_POINT('Ctrl Pts',(-9.83957192047909,0.0125000000104236,
7.14886745759543));
#283633=CARTESIAN_POINT('Ctrl Pts',(-7.51676407774787,0.162500000009825,
10.3459381770593));
#283634=CARTESIAN_POINT('Ctrl Pts',(-3.75838203887394,0.312500000009227,
11.5671105274575));
#283635=CARTESIAN_POINT('Ctrl Pts',(-1.03948091443433E-14,0.462500000008629,
12.7882828778556));
#283636=CARTESIAN_POINT('Ctrl Pts',(3.75838203887392,0.612500000008031,
11.5671105274575));
#283637=CARTESIAN_POINT('Ctrl Pts',(7.51676407774785,0.762500000007433,
10.3459381770593));
#283638=CARTESIAN_POINT('Ctrl Pts',(9.83957192047906,0.912500000006835,
7.14886745759543));
#283639=CARTESIAN_POINT('Ctrl Pts',(12.1623797632103,1.06250000000624,3.95179673813153));
#283640=CARTESIAN_POINT('Ctrl Pts',(12.1623797632103,1.21250000000564,-1.489461944703E-15));
#283641=CARTESIAN_POINT('Ctrl Pts',(12.1623797632103,1.36250000000504,-3.95179673813154));
#283642=CARTESIAN_POINT('Ctrl Pts',(9.83957192047906,1.51250000000444,-7.14886745759543));
#283643=CARTESIAN_POINT('Ctrl Pts',(7.51676407774784,1.66250000000383,-10.3459381770593));
#283644=CARTESIAN_POINT('Ctrl Pts',(3.75838203887391,1.81250000000323,-11.5671105274575));
#283645=CARTESIAN_POINT('Ctrl Pts',(-1.43908897187656E-14,1.96250000000263,
-12.7882828778556));
#283646=CARTESIAN_POINT('Ctrl Pts',(-3.75838203887394,2.11250000000203,
-11.5671105274575));
#283647=CARTESIAN_POINT('Ctrl Pts',(-7.51676407774787,2.26250000000143,
-10.3459381770593));
#283648=CARTESIAN_POINT('Ctrl Pts',(-9.83957192047909,2.41250000000082,
-7.14886745759543));
#283649=CARTESIAN_POINT('Ctrl Pts',(-12.1623797632103,2.56250000000022,
-3.95179673813153));
#283650=CARTESIAN_POINT('Ctrl Pts',(-12.1623797632103,2.71249999999962,
2.97892388940601E-15));
#283651=CARTESIAN_POINT('Ctrl Pts',(-12.1623797632103,2.86249999999902,
3.95179673813154));
#283652=CARTESIAN_POINT('Ctrl Pts',(-9.83957192047909,3.01249999999842,
7.14886745759543));
#283653=CARTESIAN_POINT('Ctrl Pts',(-7.51676407774787,3.16249999999782,
10.3459381770593));
#283654=CARTESIAN_POINT('Ctrl Pts',(-3.75838203887394,3.31249999999723,
11.5671105274575));
#283655=CARTESIAN_POINT('Ctrl Pts',(-1.21225184160051E-14,3.46249999999663,
12.7882828778556));
#283656=CARTESIAN_POINT('Ctrl Pts',(3.75838203887392,3.61249999999603,11.5671105274575));
#283657=CARTESIAN_POINT('Ctrl Pts',(7.51676407774784,3.76249999999543,10.3459381770593));
#283658=CARTESIAN_POINT('Ctrl Pts',(9.83957192047906,3.91249999999483,7.14886745759543));
#283659=CARTESIAN_POINT('Ctrl Pts',(12.1623797632103,4.06249999999424,3.95179673813153));
#283660=CARTESIAN_POINT('Ctrl Pts',(12.1623797632103,4.21249999999364,-1.489461944703E-15));
#283661=CARTESIAN_POINT('Ctrl Pts',(12.1623797632103,4.36249999999303,-3.95179673813154));
#283662=CARTESIAN_POINT('Ctrl Pts',(9.83957192047906,4.51249999999243,-7.14886745759543));
#283663=CARTESIAN_POINT('Ctrl Pts',(7.51676407774784,4.66249999999183,-10.3459381770593));
#283664=CARTESIAN_POINT('Ctrl Pts',(3.75838203887391,4.81249999999123,-11.5671105274575));
#283665=CARTESIAN_POINT('Ctrl Pts',(-1.61185989904274E-14,4.96249999999063,
-12.7882828778556));
#283666=CARTESIAN_POINT('Ctrl Pts',(-3.75838203887394,5.11249999999003,
-11.5671105274575));
#283667=CARTESIAN_POINT('Ctrl Pts',(-7.51676407774788,5.26249999998942,
-10.3459381770593));
#283668=CARTESIAN_POINT('Ctrl Pts',(-9.83957192047909,5.41249999998882,
-7.14886745759543));
#283669=CARTESIAN_POINT('Ctrl Pts',(-12.1623797632103,5.56249999998822,
-3.95179673813153));
#283670=CARTESIAN_POINT('Ctrl Pts',(-12.1623797632103,5.71249999998762,
2.97892388940601E-15));
#283671=CARTESIAN_POINT('Ctrl Pts',(-12.1623797632103,5.86249999998702,
3.95179673813154));
#283672=CARTESIAN_POINT('Ctrl Pts',(-9.83957192047909,6.01249999998642,
7.14886745759543));
#283673=CARTESIAN_POINT('Ctrl Pts',(-7.51676407774787,6.16249999998582,
10.3459381770593));
#283674=CARTESIAN_POINT('Ctrl Pts',(-3.75838203887394,6.31249999998523,
11.5671105274575));
#283675=CARTESIAN_POINT('Ctrl Pts',(-1.3850227687667E-14,6.46249999998463,
12.7882828778556));
#283676=CARTESIAN_POINT('Ctrl Pts',(3.75838203887392,6.61249999998403,11.5671105274575));
#283677=CARTESIAN_POINT('Ctrl Pts',(7.51676407774784,6.76249999998343,10.3459381770593));
#283678=CARTESIAN_POINT('Ctrl Pts',(9.83957192047906,6.91249999998283,7.14886745759543));
#283679=CARTESIAN_POINT('Ctrl Pts',(12.1623797632103,7.06249999998224,3.95179673813153));
#283680=CARTESIAN_POINT('Ctrl Pts',(12.1623797632103,7.21249999998164,-1.489461944703E-15));
#283681=CARTESIAN_POINT('Ctrl Pts',(12.1623797632103,7.36249999998104,-3.95179673813154));
#283682=CARTESIAN_POINT('Ctrl Pts',(9.83957192047906,7.51249999998044,-7.14886745759543));
#283683=CARTESIAN_POINT('Ctrl Pts',(7.51676407774784,7.66249999997983,-10.3459381770593));
#283684=CARTESIAN_POINT('Ctrl Pts',(3.75838203887391,7.81249999997923,-11.5671105274575));
#283685=CARTESIAN_POINT('Ctrl Pts',(-1.78463082620892E-14,7.96249999997863,
-12.7882828778556));
#283686=CARTESIAN_POINT('Ctrl Pts',(-3.75838203887395,8.11249999997803,
-11.5671105274575));
#283687=CARTESIAN_POINT('Ctrl Pts',(-7.51676407774788,8.26249999997743,
-10.3459381770593));
#283688=CARTESIAN_POINT('Ctrl Pts',(-9.83957192047909,8.41249999997682,
-7.14886745759543));
#283689=CARTESIAN_POINT('Ctrl Pts',(-12.1623797632103,8.56249999997622,
-3.95179673813153));
#283690=CARTESIAN_POINT('Ctrl Pts',(-12.1623797632103,8.71249999997562,
2.97892388940601E-15));
#283691=CARTESIAN_POINT('Ctrl Pts',(-12.1623797632103,8.86249999997502,
3.95179673813154));
#283692=CARTESIAN_POINT('Ctrl Pts',(-9.83957192047909,9.01249999997442,
7.14886745759543));
#283693=CARTESIAN_POINT('Ctrl Pts',(-7.51676407774787,9.16249999997382,
10.3459381770593));
#283694=CARTESIAN_POINT('Ctrl Pts',(-3.75838203887394,9.31249999997323,
11.5671105274575));
#283695=CARTESIAN_POINT('Ctrl Pts',(-1.55779369593288E-14,9.46249999997263,
12.7882828778556));
#283696=CARTESIAN_POINT('Ctrl Pts',(3.75838203887391,9.61249999997203,11.5671105274575));
#283697=CARTESIAN_POINT('Ctrl Pts',(7.51676407774784,9.76249999997144,10.3459381770593));
#283698=CARTESIAN_POINT('Ctrl Pts',(9.83957192047906,9.91249999997084,7.14886745759543));
#283699=CARTESIAN_POINT('Ctrl Pts',(12.1623797632103,10.0624999999702,3.95179673813153));
#283700=CARTESIAN_POINT('Ctrl Pts',(12.1623797632103,10.2124999999696,-1.489461944703E-15));
#283701=CARTESIAN_POINT('Ctrl Pts',(12.1623797632103,10.362499999969,-3.95179673813154));
#283702=CARTESIAN_POINT('Ctrl Pts',(9.83957192047905,10.5124999999684,-7.14886745759543));
#283703=CARTESIAN_POINT('Ctrl Pts',(7.51676407774784,10.6624999999678,-10.3459381770593));
#283704=CARTESIAN_POINT('Ctrl Pts',(3.75838203887391,10.8124999999672,-11.5671105274575));
#283705=CARTESIAN_POINT('Ctrl Pts',(-1.95740175337511E-14,10.9624999999666,
-12.7882828778556));
#283706=CARTESIAN_POINT('Ctrl Pts',(-3.75838203887395,11.112499999966,-11.5671105274575));
#283707=CARTESIAN_POINT('Ctrl Pts',(-7.51676407774788,11.2624999999654,
-10.3459381770593));
#283708=CARTESIAN_POINT('Ctrl Pts',(-9.83957192047909,11.4124999999648,
-7.14886745759543));
#283709=CARTESIAN_POINT('Ctrl Pts',(-12.1623797632103,11.5624999999642,
-3.95179673813153));
#283710=CARTESIAN_POINT('Ctrl Pts',(-12.1623797632103,11.7124999999636,
2.97892388940601E-15));
#283711=CARTESIAN_POINT('Ctrl Pts',(-12.1623797632103,11.862499999963,3.95179673813154));
#283712=CARTESIAN_POINT('Ctrl Pts',(-9.83957192047909,12.0124999999624,
7.14886745759543));
#283713=CARTESIAN_POINT('Ctrl Pts',(-7.51676407774788,12.1624999999618,
10.3459381770593));
#283714=CARTESIAN_POINT('Ctrl Pts',(-3.75838203887395,12.3124999999612,
11.5671105274575));
#283715=CARTESIAN_POINT('Ctrl Pts',(-1.73056462309906E-14,12.4624999999606,
12.7882828778556));
#283716=CARTESIAN_POINT('Ctrl Pts',(3.75838203887391,12.61249999996,11.5671105274575));
#283717=CARTESIAN_POINT('Ctrl Pts',(7.51676407774784,12.7624999999594,10.3459381770593));
#283718=CARTESIAN_POINT('Ctrl Pts',(9.83957192047906,12.9124999999588,7.14886745759543));
#283719=CARTESIAN_POINT('Ctrl Pts',(12.1623797632103,13.0624999999582,3.95179673813153));
#283720=CARTESIAN_POINT('Ctrl Pts',(12.1623797632103,13.2124999999576,-1.489461944703E-15));
#283721=CARTESIAN_POINT('Ctrl Pts',(12.1623797632103,13.362499999957,-3.95179673813154));
#283722=CARTESIAN_POINT('Ctrl Pts',(9.83957192047905,13.5124999999564,-7.14886745759543));
#283723=CARTESIAN_POINT('Ctrl Pts',(7.51676407774784,13.6624999999558,-10.3459381770593));
#283724=CARTESIAN_POINT('Ctrl Pts',(3.75838203887391,13.8124999999552,-11.5671105274575));
#283725=CARTESIAN_POINT('Ctrl Pts',(-2.13017268054129E-14,13.9624999999546,
-12.7882828778556));
#283726=CARTESIAN_POINT('Ctrl Pts',(-3.75838203887395,14.112499999954,-11.5671105274575));
#283727=CARTESIAN_POINT('Ctrl Pts',(-7.51676407774788,14.2624999999534,
-10.3459381770593));
#283728=CARTESIAN_POINT('Ctrl Pts',(-9.8395719204791,14.4124999999528,-7.14886745759543));
#283729=CARTESIAN_POINT('Ctrl Pts',(-12.1623797632103,14.5624999999522,
-3.95179673813153));
#283730=CARTESIAN_POINT('Ctrl Pts',(-12.1623797632103,14.7124999999516,
2.97892388940601E-15));
#283731=CARTESIAN_POINT('Ctrl Pts',(-12.1623797632103,14.862499999951,3.95179673813154));
#283732=CARTESIAN_POINT('Ctrl Pts',(-9.83957192047909,15.0124999999504,
7.14886745759543));
#283733=CARTESIAN_POINT('Ctrl Pts',(-7.51676407774788,15.1624999999498,
10.3459381770593));
#283734=CARTESIAN_POINT('Ctrl Pts',(-3.75838203887395,15.3124999999492,
11.5671105274575));
#283735=CARTESIAN_POINT('Ctrl Pts',(-1.90333555026525E-14,15.4624999999486,
12.7882828778556));
#283736=CARTESIAN_POINT('Ctrl Pts',(3.75838203887391,15.612499999948,11.5671105274575));
#283737=CARTESIAN_POINT('Ctrl Pts',(7.51676407774784,15.7624999999474,10.3459381770593));
#283738=CARTESIAN_POINT('Ctrl Pts',(9.83957192047905,15.9124999999468,7.14886745759543));
#283739=CARTESIAN_POINT('Ctrl Pts',(12.1623797632103,16.0624999999462,3.95179673813153));
#283740=CARTESIAN_POINT('Ctrl Pts',(12.1623797632103,16.2124999999456,-1.489461944703E-15));
#283741=CARTESIAN_POINT('Ctrl Pts',(12.1623797632103,16.362499999945,-3.95179673813154));
#283742=CARTESIAN_POINT('Ctrl Pts',(9.83957192047905,16.5124999999444,-7.14886745759543));
#283743=CARTESIAN_POINT('Ctrl Pts',(7.51676407774784,16.6624999999438,-10.3459381770593));
#283744=CARTESIAN_POINT('Ctrl Pts',(3.75838203887391,16.8124999999432,-11.5671105274575));
#283745=CARTESIAN_POINT('Ctrl Pts',(-2.30294360770748E-14,16.9624999999426,
-12.7882828778556));
#283746=CARTESIAN_POINT('Ctrl Pts',(-3.75838203887395,17.112499999942,-11.5671105274575));
#283747=CARTESIAN_POINT('Ctrl Pts',(-7.51676407774788,17.2624999999414,
-10.3459381770593));
#283748=CARTESIAN_POINT('Ctrl Pts',(-9.8395719204791,17.4124999999408,-7.14886745759543));
#283749=CARTESIAN_POINT('Ctrl Pts',(-12.1623797632103,17.5624999999402,
-3.95179673813153));
#283750=CARTESIAN_POINT('Ctrl Pts',(-12.1623797632103,17.7124999999396,
2.97892388940601E-15));
#283751=CARTESIAN_POINT('Ctrl Pts',(-12.1623797632103,17.862499999939,3.95179673813154));
#283752=CARTESIAN_POINT('Ctrl Pts',(-9.8395719204791,18.0124999999384,7.14886745759543));
#283753=CARTESIAN_POINT('Ctrl Pts',(-7.51676407774788,18.1624999999378,
10.3459381770593));
#283754=CARTESIAN_POINT('Ctrl Pts',(-3.75838203887395,18.3124999999372,
11.5671105274575));
#283755=CARTESIAN_POINT('Ctrl Pts',(-2.07610647743143E-14,18.4624999999366,
12.7882828778556));
#283756=CARTESIAN_POINT('Ctrl Pts',(3.75838203887391,18.612499999936,11.5671105274575));
#283757=CARTESIAN_POINT('Ctrl Pts',(7.51676407774784,18.7624999999354,10.3459381770593));
#283758=CARTESIAN_POINT('Ctrl Pts',(9.83957192047905,18.9124999999348,7.14886745759543));
#283759=CARTESIAN_POINT('Ctrl Pts',(12.1623797632103,19.0624999999342,3.95179673813153));
#283760=CARTESIAN_POINT('Ctrl Pts',(12.1623797632103,19.2124999999336,-1.489461944703E-15));
#283761=CARTESIAN_POINT('Ctrl Pts',(12.1623797632103,19.362499999933,-3.95179673813154));
#283762=CARTESIAN_POINT('Ctrl Pts',(9.83957192047905,19.5124999999324,-7.14886745759543));
#283763=CARTESIAN_POINT('Ctrl Pts',(7.51676407774784,19.6624999999318,-10.3459381770593));
#283764=CARTESIAN_POINT('Ctrl Pts',(3.7583820388739,19.8124999999312,-11.5671105274575));
#283765=CARTESIAN_POINT('Ctrl Pts',(-2.47571453487366E-14,19.9624999999306,
-12.7882828778556));
#283766=CARTESIAN_POINT('Ctrl Pts',(-3.75838203887395,20.11249999993,-11.5671105274575));
#283767=CARTESIAN_POINT('Ctrl Pts',(-7.51676407774788,20.2624999999294,
-10.3459381770593));
#283768=CARTESIAN_POINT('Ctrl Pts',(-9.8395719204791,20.4124999999288,-7.14886745759543));
#283769=CARTESIAN_POINT('Ctrl Pts',(-12.1623797632103,20.5624999999282,
-3.95179673813153));
#283770=CARTESIAN_POINT('Ctrl Pts',(-12.1623797632103,20.7124999999276,
2.97892388940601E-15));
#283771=CARTESIAN_POINT('Ctrl Pts',(-12.1623797632103,20.862499999927,3.95179673813154));
#283772=CARTESIAN_POINT('Ctrl Pts',(-9.8395719204791,21.0124999999264,7.14886745759543));
#283773=CARTESIAN_POINT('Ctrl Pts',(-7.51676407774788,21.1624999999258,
10.3459381770593));
#283774=CARTESIAN_POINT('Ctrl Pts',(-3.75838203887395,21.3124999999252,
11.5671105274575));
#283775=CARTESIAN_POINT('Ctrl Pts',(-2.24887740459762E-14,21.4624999999246,
12.7882828778556));
#283776=CARTESIAN_POINT('Ctrl Pts',(3.75838203887391,21.612499999924,11.5671105274575));
#283777=CARTESIAN_POINT('Ctrl Pts',(7.51676407774784,21.7624999999234,10.3459381770593));
#283778=CARTESIAN_POINT('Ctrl Pts',(9.83957192047905,21.9124999999228,7.14886745759543));
#283779=CARTESIAN_POINT('Ctrl Pts',(12.1623797632103,22.0624999999222,3.95179673813153));
#283780=CARTESIAN_POINT('Ctrl Pts',(12.1623797632103,22.2124999999216,-1.489461944703E-15));
#283781=CARTESIAN_POINT('Ctrl Pts',(12.1623797632103,22.362499999921,-3.95179673813154));
#283782=CARTESIAN_POINT('Ctrl Pts',(9.83957192047905,22.5124999999204,-7.14886745759543));
#283783=CARTESIAN_POINT('Ctrl Pts',(7.51676407774783,22.6624999999198,-10.3459381770593));
#283784=CARTESIAN_POINT('Ctrl Pts',(3.7583820388739,22.8124999999192,-11.5671105274575));
#283785=CARTESIAN_POINT('Ctrl Pts',(-2.64848546203984E-14,22.9624999999186,
-12.7882828778556));
#283786=CARTESIAN_POINT('Ctrl Pts',(-3.75838203887396,23.112499999918,-11.5671105274575));
#283787=CARTESIAN_POINT('Ctrl Pts',(-7.51676407774788,23.2624999999174,
-10.3459381770593));
#283788=CARTESIAN_POINT('Ctrl Pts',(-9.8395719204791,23.4124999999168,-7.14886745759543));
#283789=CARTESIAN_POINT('Ctrl Pts',(-12.1623797632103,23.5624999999162,
-3.95179673813153));
#283790=CARTESIAN_POINT('Ctrl Pts',(-12.1623797632103,23.7124999999156,
2.97892388940601E-15));
#283791=CARTESIAN_POINT('Ctrl Pts',(-12.1623797632103,23.862499999915,3.95179673813154));
#283792=CARTESIAN_POINT('Ctrl Pts',(-9.8395719204791,24.0124999999144,7.14886745759543));
#283793=CARTESIAN_POINT('Ctrl Pts',(-7.51676407774788,24.1624999999138,
10.3459381770593));
#283794=CARTESIAN_POINT('Ctrl Pts',(-3.75838203887395,24.3124999999132,
11.5671105274575));
#283795=CARTESIAN_POINT('Ctrl Pts',(-2.4216483317638E-14,24.4624999999126,
12.7882828778556));
#283796=CARTESIAN_POINT('Ctrl Pts',(3.7583820388739,24.612499999912,11.5671105274575));
#283797=CARTESIAN_POINT('Ctrl Pts',(7.51676407774783,24.7624999999114,10.3459381770593));
#283798=CARTESIAN_POINT('Ctrl Pts',(9.83957192047905,24.9124999999108,7.14886745759543));
#283799=CARTESIAN_POINT('Ctrl Pts',(12.1623797632103,25.0624999999102,3.95179673813153));
#283800=CARTESIAN_POINT('Ctrl Pts',(12.1623797632103,25.2124999999096,-1.489461944703E-15));
#283801=CARTESIAN_POINT('Ctrl Pts',(12.1623797632103,25.362499999909,-3.95179673813154));
#283802=CARTESIAN_POINT('Ctrl Pts',(9.83957192047905,25.5124999999084,-7.14886745759543));
#283803=CARTESIAN_POINT('Ctrl Pts',(7.51676407774783,25.6624999999078,-10.3459381770593));
#283804=CARTESIAN_POINT('Ctrl Pts',(3.7583820388739,25.8124999999072,-11.5671105274575));
#283805=CARTESIAN_POINT('Ctrl Pts',(-2.82125638920603E-14,25.9624999999066,
-12.7882828778556));
#283806=CARTESIAN_POINT('Ctrl Pts',(-3.75838203887396,26.112499999906,-11.5671105274575));
#283807=CARTESIAN_POINT('Ctrl Pts',(-7.51676407774788,26.2624999999054,
-10.3459381770593));
#283808=CARTESIAN_POINT('Ctrl Pts',(-9.8395719204791,26.4124999999048,-7.14886745759543));
#283809=CARTESIAN_POINT('Ctrl Pts',(-12.1623797632103,26.5624999999042,
-3.95179673813153));
#283810=CARTESIAN_POINT('Ctrl Pts',(-12.1623797632103,26.7124999999036,
2.97892388940601E-15));
#283811=CARTESIAN_POINT('Ctrl Pts',(-12.1623797632103,26.862499999903,3.95179673813154));
#283812=CARTESIAN_POINT('Ctrl Pts',(-9.8395719204791,27.0124999999024,7.14886745759543));
#283813=CARTESIAN_POINT('Ctrl Pts',(-7.51676407774788,27.1624999999018,
10.3459381770593));
#283814=CARTESIAN_POINT('Ctrl Pts',(-3.75838203887396,27.3124999999012,
11.5671105274575));
#283815=CARTESIAN_POINT('Ctrl Pts',(-2.59441925892998E-14,27.4624999999006,
12.7882828778556));
#283816=CARTESIAN_POINT('Ctrl Pts',(3.7583820388739,27.6124999999,11.5671105274575));
#283817=CARTESIAN_POINT('Ctrl Pts',(7.51676407774783,27.7624999998994,10.3459381770593));
#283818=CARTESIAN_POINT('Ctrl Pts',(9.83957192047905,27.9124999998988,7.14886745759543));
#283819=CARTESIAN_POINT('Ctrl Pts',(12.1623797632103,28.0624999998982,3.95179673813153));
#283820=CARTESIAN_POINT('Ctrl Pts',(12.1623797632103,28.2124999998976,-1.489461944703E-15));
#283821=CARTESIAN_POINT('Ctrl Pts',(12.1623797632103,28.362499999897,-3.95179673813154));
#283822=CARTESIAN_POINT('Ctrl Pts',(9.83957192047905,28.5124999998964,-7.14886745759543));
#283823=CARTESIAN_POINT('Ctrl Pts',(7.51676407774783,28.6624999998958,-10.3459381770593));
#283824=CARTESIAN_POINT('Ctrl Pts',(3.7583820388739,28.8124999998952,-11.5671105274575));
#283825=CARTESIAN_POINT('Ctrl Pts',(-2.99402731637221E-14,28.9624999998946,
-12.7882828778556));
#283826=CARTESIAN_POINT('Ctrl Pts',(-3.75838203887396,29.112499999894,-11.5671105274575));
#283827=CARTESIAN_POINT('Ctrl Pts',(-7.51676407774789,29.2624999998934,
-10.3459381770593));
#283828=CARTESIAN_POINT('Ctrl Pts',(-9.8395719204791,29.4124999998928,-7.14886745759543));
#283829=CARTESIAN_POINT('Ctrl Pts',(-12.1623797632103,29.5624999998922,
-3.95179673813153));
#283830=CARTESIAN_POINT('Ctrl Pts',(-12.1623797632103,29.7124999998916,
2.97892388940601E-15));
#283831=CARTESIAN_POINT('Ctrl Pts',(-12.1623797632103,29.862499999891,3.95179673813154));
#283832=CARTESIAN_POINT('Ctrl Pts',(-9.8395719204791,30.0124999998904,7.14886745759543));
#283833=CARTESIAN_POINT('Ctrl Pts',(-7.51676407774788,30.1624999998898,
10.3459381770593));
#283834=CARTESIAN_POINT('Ctrl Pts',(-3.75838203887396,30.3124999998892,
11.5671105274575));
#283835=CARTESIAN_POINT('Ctrl Pts',(-2.76719018609617E-14,30.4624999998886,
12.7882828778556));
#283836=CARTESIAN_POINT('Ctrl Pts',(3.7583820388739,30.612499999888,11.5671105274575));
#283837=CARTESIAN_POINT('Ctrl Pts',(7.51676407774783,30.7624999998874,10.3459381770593));
#283838=CARTESIAN_POINT('Ctrl Pts',(9.83957192047905,30.9124999998868,7.14886745759543));
#283839=CARTESIAN_POINT('Ctrl Pts',(12.1623797632103,31.0624999998862,3.95179673813153));
#283840=CARTESIAN_POINT('Ctrl Pts',(12.1623797632103,31.2124999998856,-1.489461944703E-15));
#283841=CARTESIAN_POINT('Ctrl Pts',(12.1623797632103,31.362499999885,-3.95179673813154));
#283842=CARTESIAN_POINT('Ctrl Pts',(9.83957192047904,31.5124999998844,-7.14886745759543));
#283843=CARTESIAN_POINT('Ctrl Pts',(7.51676407774783,31.6624999998838,-10.3459381770593));
#283844=CARTESIAN_POINT('Ctrl Pts',(3.7583820388739,31.8124999998832,-11.5671105274575));
#283845=CARTESIAN_POINT('Ctrl Pts',(-3.16679824353839E-14,31.9624999998826,
-12.7882828778556));
#283846=CARTESIAN_POINT('Ctrl Pts',(-3.75838203887396,32.112499999882,-11.5671105274575));
#283847=CARTESIAN_POINT('Ctrl Pts',(-7.51676407774789,32.2624999998814,
-10.3459381770593));
#283848=CARTESIAN_POINT('Ctrl Pts',(-9.83957192047911,32.4124999998808,
-7.14886745759543));
#283849=CARTESIAN_POINT('Ctrl Pts',(-12.1623797632103,32.5624999998802,
-3.95179673813153));
#283850=CARTESIAN_POINT('Ctrl Pts',(-12.1623797632103,32.7124999998796,
2.97892388940601E-15));
#283851=CARTESIAN_POINT('Ctrl Pts',(-12.1623797632103,32.862499999879,3.95179673813154));
#283852=CARTESIAN_POINT('Ctrl Pts',(-9.8395719204791,33.0124999998784,7.14886745759543));
#283853=CARTESIAN_POINT('Ctrl Pts',(-7.51676407774789,33.1624999998778,
10.3459381770593));
#283854=CARTESIAN_POINT('Ctrl Pts',(-3.75838203887396,33.3124999998772,
11.5671105274575));
#283855=CARTESIAN_POINT('Ctrl Pts',(-2.93996111326235E-14,33.4624999998766,
12.7882828778556));
#283856=CARTESIAN_POINT('Ctrl Pts',(3.7583820388739,33.612499999876,11.5671105274575));
#283857=CARTESIAN_POINT('Ctrl Pts',(7.51676407774783,33.7624999998754,10.3459381770593));
#283858=CARTESIAN_POINT('Ctrl Pts',(9.83957192047905,33.9124999998748,7.14886745759543));
#283859=CARTESIAN_POINT('Ctrl Pts',(12.1623797632103,34.0624999998742,3.95179673813153));
#283860=CARTESIAN_POINT('Ctrl Pts',(12.1623797632103,34.2124999998736,-1.489461944703E-15));
#283861=CARTESIAN_POINT('Ctrl Pts',(12.1623797632103,34.362499999873,-3.95179673813154));
#283862=CARTESIAN_POINT('Ctrl Pts',(9.83957192047904,34.5124999998724,-7.14886745759543));
#283863=CARTESIAN_POINT('Ctrl Pts',(7.51676407774783,34.6624999998718,-10.3459381770593));
#283864=CARTESIAN_POINT('Ctrl Pts',(3.7583820388739,34.8124999998712,-11.5671105274575));
#283865=CARTESIAN_POINT('Ctrl Pts',(-3.33956917070458E-14,34.9624999998706,
-12.7882828778556));
#283866=CARTESIAN_POINT('Ctrl Pts',(-3.75838203887396,35.11249999987,-11.5671105274575));
#283867=CARTESIAN_POINT('Ctrl Pts',(-7.51676407774789,35.2624999998694,
-10.3459381770593));
#283868=CARTESIAN_POINT('Ctrl Pts',(-9.83957192047911,35.4124999998688,
-7.14886745759543));
#283869=CARTESIAN_POINT('Ctrl Pts',(-12.1623797632103,35.5624999998682,
-3.95179673813153));
#283870=CARTESIAN_POINT('Ctrl Pts',(-12.1623797632103,35.7124999998676,
2.97892388940601E-15));
#283871=CARTESIAN_POINT('Ctrl Pts',(-12.1623797632103,35.862499999867,3.95179673813154));
#283872=CARTESIAN_POINT('Ctrl Pts',(-9.83957192047911,36.0124999998664,
7.14886745759543));
#283873=CARTESIAN_POINT('Ctrl Pts',(-7.51676407774789,36.1624999998658,
10.3459381770593));
#283874=CARTESIAN_POINT('Ctrl Pts',(-3.75838203887396,36.3124999998652,
11.5671105274575));
#283875=CARTESIAN_POINT('Ctrl Pts',(-3.11273204042854E-14,36.4624999998646,
12.7882828778556));
#283876=CARTESIAN_POINT('Ctrl Pts',(3.7583820388739,36.612499999864,11.5671105274575));
#283877=CARTESIAN_POINT('Ctrl Pts',(7.51676407774783,36.7624999998634,10.3459381770593));
#283878=CARTESIAN_POINT('Ctrl Pts',(9.83957192047904,36.9124999998628,7.14886745759543));
#283879=CARTESIAN_POINT('Ctrl Pts',(12.1623797632103,37.0624999998622,3.95179673813153));
#283880=CARTESIAN_POINT('Ctrl Pts',(12.1623797632103,37.2124999998616,-1.489461944703E-15));
#283881=CARTESIAN_POINT('Ctrl Pts',(12.1623797632103,37.362499999861,-3.95179673813154));
#283882=CARTESIAN_POINT('Ctrl Pts',(9.83957192047904,37.5124999998604,-7.14886745759543));
#283883=CARTESIAN_POINT('Ctrl Pts',(7.51676407774782,37.6624999998598,-10.3459381770593));
#283884=CARTESIAN_POINT('Ctrl Pts',(3.75838203887389,37.8124999998592,-11.5671105274575));
#283885=CARTESIAN_POINT('Ctrl Pts',(-3.51234009787076E-14,37.9624999998586,
-12.7882828778556));
#283886=CARTESIAN_POINT('Ctrl Pts',(-3.75838203887396,38.112499999858,-11.5671105274575));
#283887=CARTESIAN_POINT('Ctrl Pts',(-7.51676407774789,38.2624999998574,
-10.3459381770593));
#283888=CARTESIAN_POINT('Ctrl Pts',(-9.83957192047911,38.4124999998568,
-7.14886745759543));
#283889=CARTESIAN_POINT('Ctrl Pts',(-12.1623797632103,38.5624999998562,
-3.95179673813153));
#283890=CARTESIAN_POINT('Ctrl Pts',(-12.1623797632103,38.7124999998556,
2.97892388940601E-15));
#283891=CARTESIAN_POINT('Ctrl Pts',(-12.1623797632103,38.862499999855,3.95179673813154));
#283892=CARTESIAN_POINT('Ctrl Pts',(-9.83957192047911,39.0124999998544,
7.14886745759543));
#283893=CARTESIAN_POINT('Ctrl Pts',(-7.51676407774789,39.1624999998538,
10.3459381770593));
#283894=CARTESIAN_POINT('Ctrl Pts',(-3.75838203887396,39.3124999998532,
11.5671105274575));
#283895=CARTESIAN_POINT('Ctrl Pts',(-3.28550296759472E-14,39.4624999998526,
12.7882828778556));
#283896=CARTESIAN_POINT('Ctrl Pts',(3.7583820388739,39.612499999852,11.5671105274575));
#283897=CARTESIAN_POINT('Ctrl Pts',(7.51676407774782,39.7624999998514,10.3459381770593));
#283898=CARTESIAN_POINT('Ctrl Pts',(9.83957192047904,39.9124999998508,7.14886745759543));
#283899=CARTESIAN_POINT('Ctrl Pts',(12.1623797632103,40.0624999998502,3.95179673813153));
#283900=CARTESIAN_POINT('Ctrl Pts',(12.1623797632103,40.2124999998496,-1.489461944703E-15));
#283901=CARTESIAN_POINT('Ctrl Pts',(12.1623797632103,40.362499999849,-3.95179673813154));
#283902=CARTESIAN_POINT('Ctrl Pts',(9.83957192047904,40.5124999998484,-7.14886745759543));
#283903=CARTESIAN_POINT('Ctrl Pts',(7.51676407774782,40.6624999998478,-10.3459381770593));
#283904=CARTESIAN_POINT('Ctrl Pts',(3.75838203887389,40.8124999998472,-11.5671105274575));
#283905=CARTESIAN_POINT('Ctrl Pts',(-3.68511102503695E-14,40.9624999998466,
-12.7882828778556));
#283906=CARTESIAN_POINT('Ctrl Pts',(-3.75838203887397,41.112499999846,-11.5671105274575));
#283907=CARTESIAN_POINT('Ctrl Pts',(-7.51676407774789,41.2624999998454,
-10.3459381770593));
#283908=CARTESIAN_POINT('Ctrl Pts',(-9.83957192047911,41.4124999998448,
-7.14886745759543));
#283909=CARTESIAN_POINT('Ctrl Pts',(-12.1623797632103,41.5624999998442,
-3.95179673813153));
#283910=CARTESIAN_POINT('Ctrl Pts',(-12.1623797632103,41.7124999998436,
2.97892388940601E-15));
#283911=CARTESIAN_POINT('Ctrl Pts',(-12.1623797632103,41.862499999843,3.95179673813154));
#283912=CARTESIAN_POINT('Ctrl Pts',(-9.83957192047911,42.0124999998424,
7.14886745759543));
#283913=CARTESIAN_POINT('Ctrl Pts',(-7.51676407774789,42.1624999998418,
10.3459381770593));
#283914=CARTESIAN_POINT('Ctrl Pts',(-3.75838203887396,42.3124999998412,
11.5671105274575));
#283915=CARTESIAN_POINT('Ctrl Pts',(-3.4582738947609E-14,42.4624999998406,
12.7882828778556));
#283916=CARTESIAN_POINT('Ctrl Pts',(3.75838203887389,42.61249999984,11.5671105274575));
#283917=CARTESIAN_POINT('Ctrl Pts',(7.51676407774782,42.7624999998394,10.3459381770593));
#283918=CARTESIAN_POINT('Ctrl Pts',(9.83957192047904,42.9124999998388,7.14886745759543));
#283919=CARTESIAN_POINT('Ctrl Pts',(12.1623797632103,43.0624999998382,3.95179673813153));
#283920=CARTESIAN_POINT('Ctrl Pts',(12.1623797632103,43.2124999998376,-1.489461944703E-15));
#283921=CARTESIAN_POINT('Ctrl Pts',(12.1623797632103,43.362499999837,-3.95179673813154));
#283922=CARTESIAN_POINT('Ctrl Pts',(9.83957192047903,43.5124999998364,-7.14886745759543));
#283923=CARTESIAN_POINT('Ctrl Pts',(7.51676407774782,43.6624999998358,-10.3459381770593));
#283924=CARTESIAN_POINT('Ctrl Pts',(3.75838203887389,43.8124999998352,-11.5671105274575));
#283925=CARTESIAN_POINT('Ctrl Pts',(-3.85788195220313E-14,43.9624999998346,
-12.7882828778556));
#283926=CARTESIAN_POINT('Ctrl Pts',(-3.75838203887397,44.112499999834,-11.5671105274575));
#283927=CARTESIAN_POINT('Ctrl Pts',(-7.5167640777479,44.2624999998334,-10.3459381770593));
#283928=CARTESIAN_POINT('Ctrl Pts',(-9.83957192047911,44.4124999998328,
-7.14886745759543));
#283929=CARTESIAN_POINT('Ctrl Pts',(-12.1623797632103,44.5624999998322,
-3.95179673813153));
#283930=CARTESIAN_POINT('Ctrl Pts',(-12.1623797632103,44.7124999998316,
2.97892388940601E-15));
#283931=CARTESIAN_POINT('Ctrl Pts',(-12.1623797632103,44.862499999831,3.95179673813154));
#283932=CARTESIAN_POINT('Ctrl Pts',(-9.83957192047911,45.0124999998304,
7.14886745759543));
#283933=CARTESIAN_POINT('Ctrl Pts',(-7.51676407774789,45.1624999998298,
10.3459381770593));
#283934=CARTESIAN_POINT('Ctrl Pts',(-3.75838203887397,45.3124999998292,
11.5671105274575));
#283935=CARTESIAN_POINT('Ctrl Pts',(-3.63104482192709E-14,45.4624999998286,
12.7882828778556));
#283936=CARTESIAN_POINT('Ctrl Pts',(3.75838203887389,45.612499999828,11.5671105274575));
#283937=CARTESIAN_POINT('Ctrl Pts',(7.51676407774782,45.7624999998274,10.3459381770593));
#283938=CARTESIAN_POINT('Ctrl Pts',(9.83957192047904,45.9124999998268,7.14886745759543));
#283939=CARTESIAN_POINT('Ctrl Pts',(12.1623797632103,46.0624999998262,3.95179673813153));
#283940=CARTESIAN_POINT('Ctrl Pts',(12.1623797632103,46.2124999998256,-1.489461944703E-15));
#283941=CARTESIAN_POINT('Ctrl Pts',(12.1623797632103,46.362499999825,-3.95179673813154));
#283942=CARTESIAN_POINT('Ctrl Pts',(9.83957192047903,46.5124999998244,-7.14886745759543));
#283943=CARTESIAN_POINT('Ctrl Pts',(7.51676407774782,46.6624999998238,-10.3459381770593));
#283944=CARTESIAN_POINT('Ctrl Pts',(3.75838203887389,46.8124999998232,-11.5671105274575));
#283945=CARTESIAN_POINT('Ctrl Pts',(-4.03065287936931E-14,46.9624999998226,
-12.7882828778556));
#283946=CARTESIAN_POINT('Ctrl Pts',(-3.75838203887397,47.112499999822,-11.5671105274575));
#283947=CARTESIAN_POINT('Ctrl Pts',(-7.5167640777479,47.2624999998214,-10.3459381770593));
#283948=CARTESIAN_POINT('Ctrl Pts',(-9.83957192047912,47.4124999998208,
-7.14886745759543));
#283949=CARTESIAN_POINT('Ctrl Pts',(-12.1623797632103,47.5624999998202,
-3.95179673813153));
#283950=CARTESIAN_POINT('Ctrl Pts',(-12.1623797632103,47.7124999998196,
2.97892388940601E-15));
#283951=CARTESIAN_POINT('Ctrl Pts',(-12.1623797632103,47.862499999819,3.95179673813154));
#283952=CARTESIAN_POINT('Ctrl Pts',(-9.83957192047911,48.0124999998184,
7.14886745759543));
#283953=CARTESIAN_POINT('Ctrl Pts',(-7.51676407774789,48.1624999998178,
10.3459381770593));
#283954=CARTESIAN_POINT('Ctrl Pts',(-3.75838203887397,48.3124999998172,
11.5671105274575));
#283955=CARTESIAN_POINT('Ctrl Pts',(-3.80381574909327E-14,48.4624999998166,
12.7882828778556));
#283956=CARTESIAN_POINT('Ctrl Pts',(3.75838203887389,48.612499999816,11.5671105274575));
#283957=CARTESIAN_POINT('Ctrl Pts',(7.51676407774782,48.7624999998154,10.3459381770593));
#283958=CARTESIAN_POINT('Ctrl Pts',(9.83957192047903,48.9124999998148,7.14886745759543));
#283959=CARTESIAN_POINT('Ctrl Pts',(12.1623797632103,49.0624999998142,3.95179673813153));
#283960=CARTESIAN_POINT('Ctrl Pts',(12.1623797632103,49.2124999998136,-1.489461944703E-15));
#283961=CARTESIAN_POINT('Ctrl Pts',(12.1623797632103,49.362499999813,-3.95179673813154));
#283962=CARTESIAN_POINT('Ctrl Pts',(9.83957192047903,49.5124999998124,-7.14886745759543));
#283963=CARTESIAN_POINT('Ctrl Pts',(7.51676407774782,49.6624999998118,-10.3459381770593));
#283964=CARTESIAN_POINT('Ctrl Pts',(3.75838203887389,49.8124999998112,-11.5671105274575));
#283965=CARTESIAN_POINT('Ctrl Pts',(-4.2034238065355E-14,49.9624999998106,
-12.7882828778556));
#283966=CARTESIAN_POINT('Ctrl Pts',(-3.75838203887397,50.11249999981,-11.5671105274575));
#283967=CARTESIAN_POINT('Ctrl Pts',(-7.5167640777479,50.2624999998094,-10.3459381770593));
#283968=CARTESIAN_POINT('Ctrl Pts',(-9.83957192047912,50.4124999998088,
-7.14886745759543));
#283969=CARTESIAN_POINT('Ctrl Pts',(-12.1623797632103,50.5624999998082,
-3.95179673813153));
#283970=CARTESIAN_POINT('Ctrl Pts',(-12.1623797632103,50.7124999998076,
2.97892388940601E-15));
#283971=CARTESIAN_POINT('Ctrl Pts',(-12.1623797632103,50.862499999807,3.95179673813154));
#283972=CARTESIAN_POINT('Ctrl Pts',(-9.83957192047912,51.0124999998064,
7.14886745759543));
#283973=CARTESIAN_POINT('Ctrl Pts',(-7.5167640777479,51.1624999998058,10.3459381770593));
#283974=CARTESIAN_POINT('Ctrl Pts',(-3.75838203887397,51.3124999998052,
11.5671105274575));
#283975=CARTESIAN_POINT('Ctrl Pts',(-3.97658667625946E-14,51.4624999998046,
12.7882828778556));
#283976=CARTESIAN_POINT('Ctrl Pts',(3.75838203887389,51.612499999804,11.5671105274575));
#283977=CARTESIAN_POINT('Ctrl Pts',(7.51676407774782,51.7624999998034,10.3459381770593));
#283978=CARTESIAN_POINT('Ctrl Pts',(9.83957192047903,51.9124999998028,7.14886745759543));
#283979=CARTESIAN_POINT('Ctrl Pts',(12.1623797632103,52.0624999998022,3.95179673813153));
#283980=CARTESIAN_POINT('Ctrl Pts',(12.1623797632103,52.2124999998016,-1.489461944703E-15));
#283981=CARTESIAN_POINT('Ctrl Pts',(12.1623797632103,52.362499999801,-3.95179673813154));
#283982=CARTESIAN_POINT('Ctrl Pts',(9.83957192047903,52.5124999998004,-7.14886745759543));
#283983=CARTESIAN_POINT('Ctrl Pts',(7.51676407774781,52.6624999997998,-10.3459381770593));
#283984=CARTESIAN_POINT('Ctrl Pts',(3.75838203887388,52.8124999997992,-11.5671105274575));
#283985=CARTESIAN_POINT('Ctrl Pts',(-4.37619473370168E-14,52.9624999997986,
-12.7882828778556));
#283986=CARTESIAN_POINT('Ctrl Pts',(-3.75838203887397,53.112499999798,-11.5671105274575));
#283987=CARTESIAN_POINT('Ctrl Pts',(-7.5167640777479,53.2624999997974,-10.3459381770593));
#283988=CARTESIAN_POINT('Ctrl Pts',(-9.83957192047912,53.4124999997968,
-7.14886745759543));
#283989=CARTESIAN_POINT('Ctrl Pts',(-12.1623797632103,53.5624999997962,
-3.95179673813153));
#283990=CARTESIAN_POINT('Ctrl Pts',(-12.1623797632103,53.7124999997956,
2.97892388940601E-15));
#283991=CARTESIAN_POINT('Ctrl Pts',(-12.1623797632103,53.862499999795,3.95179673813154));
#283992=CARTESIAN_POINT('Ctrl Pts',(-9.83957192047912,54.0124999997944,
7.14886745759543));
#283993=CARTESIAN_POINT('Ctrl Pts',(-7.5167640777479,54.1624999997938,10.3459381770593));
#283994=CARTESIAN_POINT('Ctrl Pts',(-3.75838203887397,54.3124999997932,
11.5671105274575));
#283995=CARTESIAN_POINT('Ctrl Pts',(-4.14935760342564E-14,54.4624999997926,
12.7882828778556));
#283996=CARTESIAN_POINT('Ctrl Pts',(3.75838203887389,54.612499999792,11.5671105274575));
#283997=CARTESIAN_POINT('Ctrl Pts',(7.51676407774782,54.7624999997914,10.3459381770593));
#283998=CARTESIAN_POINT('Ctrl Pts',(9.83957192047903,54.9124999997908,7.14886745759543));
#283999=CARTESIAN_POINT('Ctrl Pts',(12.1623797632103,55.0624999997902,3.95179673813153));
#284000=CARTESIAN_POINT('Ctrl Pts',(12.1623797632103,55.2124999997896,-1.489461944703E-15));
#284001=CARTESIAN_POINT('Ctrl Pts',(12.1623797632103,55.362499999789,-3.95179673813154));
#284002=CARTESIAN_POINT('Ctrl Pts',(9.83957192047903,55.5124999997884,-7.14886745759543));
#284003=CARTESIAN_POINT('Ctrl Pts',(7.51676407774781,55.6624999997878,-10.3459381770593));
#284004=CARTESIAN_POINT('Ctrl Pts',(3.75838203887388,55.8124999997872,-11.5671105274575));
#284005=CARTESIAN_POINT('Ctrl Pts',(-4.54896566086787E-14,55.9624999997866,
-12.7882828778556));
#284006=CARTESIAN_POINT('Ctrl Pts',(-3.75838203887397,56.112499999786,-11.5671105274575));
#284007=CARTESIAN_POINT('Ctrl Pts',(-7.5167640777479,56.2624999997854,-10.3459381770593));
#284008=CARTESIAN_POINT('Ctrl Pts',(-9.83957192047912,56.4124999997848,
-7.14886745759543));
#284009=CARTESIAN_POINT('Ctrl Pts',(-12.1623797632103,56.5624999997842,
-3.95179673813153));
#284010=CARTESIAN_POINT('Ctrl Pts',(-12.1623797632103,56.7124999997836,
2.97892388940601E-15));
#284011=CARTESIAN_POINT('Ctrl Pts',(-12.1623797632103,56.862499999783,3.95179673813154));
#284012=CARTESIAN_POINT('Ctrl Pts',(-9.83957192047912,57.0124999997824,
7.14886745759543));
#284013=CARTESIAN_POINT('Ctrl Pts',(-7.5167640777479,57.1624999997818,10.3459381770593));
#284014=CARTESIAN_POINT('Ctrl Pts',(-3.75838203887397,57.3124999997812,
11.5671105274575));
#284015=CARTESIAN_POINT('Ctrl Pts',(-4.32212853059182E-14,57.4624999997806,
12.7882828778556));
#284016=CARTESIAN_POINT('Ctrl Pts',(3.75838203887389,57.61249999978,11.5671105274575));
#284017=CARTESIAN_POINT('Ctrl Pts',(7.51676407774781,57.7624999997794,10.3459381770593));
#284018=CARTESIAN_POINT('Ctrl Pts',(9.83957192047903,57.9124999997788,7.14886745759543));
#284019=CARTESIAN_POINT('Ctrl Pts',(12.1623797632103,58.0624999997782,3.95179673813153));
#284020=CARTESIAN_POINT('Ctrl Pts',(12.1623797632102,58.2124999997776,-1.489461944703E-15));
#284021=CARTESIAN_POINT('Ctrl Pts',(12.1623797632102,58.362499999777,-3.95179673813154));
#284022=CARTESIAN_POINT('Ctrl Pts',(9.83957192047903,58.5124999997764,-7.14886745759543));
#284023=CARTESIAN_POINT('Ctrl Pts',(7.51676407774781,58.6624999997758,-10.3459381770593));
#284024=CARTESIAN_POINT('Ctrl Pts',(3.75838203887388,58.8124999997752,-11.5671105274575));
#284025=CARTESIAN_POINT('Ctrl Pts',(-4.72173658803405E-14,58.9624999997746,
-12.7882828778556));
#284026=CARTESIAN_POINT('Ctrl Pts',(-3.75838203887398,59.112499999774,-11.5671105274575));
#284027=CARTESIAN_POINT('Ctrl Pts',(-7.51676407774791,59.2624999997734,
-10.3459381770593));
#284028=CARTESIAN_POINT('Ctrl Pts',(-9.83957192047912,59.4124999997728,
-7.14886745759543));
#284029=CARTESIAN_POINT('Ctrl Pts',(-12.1623797632103,59.5624999997722,
-3.95179673813153));
#284030=CARTESIAN_POINT('Ctrl Pts',(-12.1623797632103,59.7124999997716,
2.97892388940601E-15));
#284031=CARTESIAN_POINT('Ctrl Pts',(-12.1623797632103,59.862499999771,3.95179673813154));
#284032=CARTESIAN_POINT('Ctrl Pts',(-9.83957192047912,60.0124999997704,
7.14886745759543));
#284033=CARTESIAN_POINT('Ctrl Pts',(-7.5167640777479,60.1624999997698,10.3459381770593));
#284034=CARTESIAN_POINT('Ctrl Pts',(-3.75838203887397,60.3124999997692,
11.5671105274575));
#284035=CARTESIAN_POINT('Ctrl Pts',(-4.49489945775801E-14,60.4624999997686,
12.7882828778556));
#284036=CARTESIAN_POINT('Ctrl Pts',(3.75838203887388,60.612499999768,11.5671105274575));
#284037=CARTESIAN_POINT('Ctrl Pts',(7.51676407774781,60.7624999997674,10.3459381770593));
#284038=CARTESIAN_POINT('Ctrl Pts',(9.83957192047903,60.9124999997668,7.14886745759543));
#284039=CARTESIAN_POINT('Ctrl Pts',(12.1623797632103,61.0624999997662,3.95179673813153));
#284040=CARTESIAN_POINT('Ctrl Pts',(12.1623797632102,61.2124999997656,-1.489461944703E-15));
#284041=CARTESIAN_POINT('Ctrl Pts',(12.1623797632102,61.362499999765,-3.95179673813154));
#284042=CARTESIAN_POINT('Ctrl Pts',(9.83957192047902,61.5124999997644,-7.14886745759543));
#284043=CARTESIAN_POINT('Ctrl Pts',(7.51676407774781,61.6624999997638,-10.3459381770593));
#284044=CARTESIAN_POINT('Ctrl Pts',(3.75838203887388,61.8124999997632,-11.5671105274575));
#284045=CARTESIAN_POINT('Ctrl Pts',(-4.89450751520023E-14,61.9624999997626,
-12.7882828778556));
#284046=CARTESIAN_POINT('Ctrl Pts',(-3.75838203887398,62.112499999762,-11.5671105274575));
#284047=CARTESIAN_POINT('Ctrl Pts',(-7.51676407774791,62.2624999997614,
-10.3459381770593));
#284048=CARTESIAN_POINT('Ctrl Pts',(-9.83957192047912,62.4124999997608,
-7.14886745759543));
#284049=CARTESIAN_POINT('Ctrl Pts',(-12.1623797632103,62.5624999997602,
-3.95179673813153));
#284050=CARTESIAN_POINT('Ctrl Pts',(-12.1623797632103,62.7124999997596,
2.97892388940601E-15));
#284051=CARTESIAN_POINT('Ctrl Pts',(-12.1623797632103,62.862499999759,3.95179673813154));
#284052=CARTESIAN_POINT('Ctrl Pts',(-9.83957192047912,63.0124999997584,
7.14886745759543));
#284053=CARTESIAN_POINT('Ctrl Pts',(-7.5167640777479,63.1624999997578,10.3459381770593));
#284054=CARTESIAN_POINT('Ctrl Pts',(-3.75838203887398,63.3124999997572,
11.5671105274575));
#284055=CARTESIAN_POINT('Ctrl Pts',(-4.66767038492419E-14,63.4624999997566,
12.7882828778556));
#284056=CARTESIAN_POINT('Ctrl Pts',(3.75838203887388,63.612499999756,11.5671105274575));
#284057=CARTESIAN_POINT('Ctrl Pts',(7.51676407774781,63.7624999997554,10.3459381770593));
#284058=CARTESIAN_POINT('Ctrl Pts',(9.83957192047903,63.9124999997548,7.14886745759543));
#284059=CARTESIAN_POINT('Ctrl Pts',(12.1623797632102,64.0624999997542,3.95179673813153));
#284060=CARTESIAN_POINT('Ctrl Pts',(12.1623797632102,64.2124999997536,-1.489461944703E-15));
#284061=CARTESIAN_POINT('Ctrl Pts',(12.1623797632102,64.362499999753,-3.95179673813154));
#284062=CARTESIAN_POINT('Ctrl Pts',(9.83957192047902,64.5124999997524,-7.14886745759543));
#284063=CARTESIAN_POINT('Ctrl Pts',(7.51676407774781,64.6624999997518,-10.3459381770593));
#284064=CARTESIAN_POINT('Ctrl Pts',(3.75838203887388,64.8124999997512,-11.5671105274575));
#284065=CARTESIAN_POINT('Ctrl Pts',(-5.06727844236642E-14,64.9624999997506,
-12.7882828778556));
#284066=CARTESIAN_POINT('Ctrl Pts',(-3.75838203887398,65.11249999975,-11.5671105274575));
#284067=CARTESIAN_POINT('Ctrl Pts',(-7.51676407774791,65.2624999997494,
-10.3459381770593));
#284068=CARTESIAN_POINT('Ctrl Pts',(-9.83957192047913,65.4124999997488,
-7.14886745759543));
#284069=CARTESIAN_POINT('Ctrl Pts',(-12.1623797632103,65.5624999997482,
-3.95179673813153));
#284070=CARTESIAN_POINT('Ctrl Pts',(-12.1623797632103,65.7124999997476,
2.97892388940601E-15));
#284071=CARTESIAN_POINT('Ctrl Pts',(-12.1623797632103,65.862499999747,3.95179673813154));
#284072=CARTESIAN_POINT('Ctrl Pts',(-9.83957192047912,66.0124999997464,
7.14886745759543));
#284073=CARTESIAN_POINT('Ctrl Pts',(-7.51676407774791,66.1624999997458,
10.3459381770593));
#284074=CARTESIAN_POINT('Ctrl Pts',(-3.75838203887398,66.3124999997452,
11.5671105274575));
#284075=CARTESIAN_POINT('Ctrl Pts',(-4.84044131209037E-14,66.4624999997446,
12.7882828778556));
#284076=CARTESIAN_POINT('Ctrl Pts',(3.75838203887388,66.612499999744,11.5671105274575));
#284077=CARTESIAN_POINT('Ctrl Pts',(7.51676407774781,66.7624999997434,10.3459381770593));
#284078=CARTESIAN_POINT('Ctrl Pts',(9.83957192047902,66.9124999997428,7.14886745759543));
#284079=CARTESIAN_POINT('Ctrl Pts',(12.1623797632102,67.0624999997422,3.95179673813153));
#284080=CARTESIAN_POINT('Ctrl Pts',(12.1623797632102,67.2124999997416,-1.489461944703E-15));
#284081=CARTESIAN_POINT('Ctrl Pts',(12.1623797632102,67.362499999741,-3.95179673813154));
#284082=CARTESIAN_POINT('Ctrl Pts',(9.83957192047902,67.5124999997404,-7.14886745759543));
#284083=CARTESIAN_POINT('Ctrl Pts',(7.51676407774781,67.6624999997398,-10.3459381770593));
#284084=CARTESIAN_POINT('Ctrl Pts',(3.75838203887388,67.8124999997392,-11.5671105274575));
#284085=CARTESIAN_POINT('Ctrl Pts',(-5.2400493695326E-14,67.9624999997386,
-12.7882828778556));
#284086=CARTESIAN_POINT('Ctrl Pts',(-3.75838203887398,68.112499999738,-11.5671105274575));
#284087=CARTESIAN_POINT('Ctrl Pts',(-7.51676407774791,68.2624999997374,
-10.3459381770593));
#284088=CARTESIAN_POINT('Ctrl Pts',(-9.83957192047913,68.4124999997368,
-7.14886745759543));
#284089=CARTESIAN_POINT('Ctrl Pts',(-12.1623797632103,68.5624999997362,
-3.95179673813153));
#284090=CARTESIAN_POINT('Ctrl Pts',(-12.1623797632103,68.7124999997356,
2.97892388940601E-15));
#284091=CARTESIAN_POINT('Ctrl Pts',(-12.1623797632103,68.862499999735,3.95179673813154));
#284092=CARTESIAN_POINT('Ctrl Pts',(-9.83957192047913,69.0124999997344,
7.14886745759543));
#284093=CARTESIAN_POINT('Ctrl Pts',(-7.51676407774791,69.1624999997338,
10.3459381770593));
#284094=CARTESIAN_POINT('Ctrl Pts',(-3.75838203887398,69.3124999997332,
11.5671105274575));
#284095=CARTESIAN_POINT('Ctrl Pts',(-5.01321223925656E-14,69.4624999997326,
12.7882828778556));
#284096=CARTESIAN_POINT('Ctrl Pts',(3.75838203887388,69.612499999732,11.5671105274575));
#284097=CARTESIAN_POINT('Ctrl Pts',(7.51676407774781,69.7624999997314,10.3459381770593));
#284098=CARTESIAN_POINT('Ctrl Pts',(9.83957192047902,69.9124999997308,7.14886745759543));
#284099=CARTESIAN_POINT('Ctrl Pts',(12.1623797632102,70.0624999997302,3.95179673813153));
#284100=CARTESIAN_POINT('Ctrl Pts',(12.1623797632102,70.2124999997296,-1.489461944703E-15));
#284101=CARTESIAN_POINT('Ctrl Pts',(12.1623797632102,70.362499999729,-3.95179673813154));
#284102=CARTESIAN_POINT('Ctrl Pts',(9.83957192047902,70.5124999997284,-7.14886745759543));
#284103=CARTESIAN_POINT('Ctrl Pts',(7.5167640777478,70.6624999997278,-10.3459381770593));
#284104=CARTESIAN_POINT('Ctrl Pts',(3.75838203887388,70.8124999997272,-11.5671105274575));
#284105=CARTESIAN_POINT('Ctrl Pts',(-5.41282029669879E-14,70.9624999997266,
-12.7882828778556));
#284106=CARTESIAN_POINT('Ctrl Pts',(-3.75838203887398,71.112499999726,-11.5671105274575));
#284107=CARTESIAN_POINT('Ctrl Pts',(-7.51676407774791,71.2624999997254,
-10.3459381770593));
#284108=CARTESIAN_POINT('Ctrl Pts',(-9.83957192047913,71.4124999997248,
-7.14886745759543));
#284109=CARTESIAN_POINT('Ctrl Pts',(-12.1623797632103,71.5624999997242,
-3.95179673813153));
#284110=CARTESIAN_POINT('Ctrl Pts',(-12.1623797632103,71.7124999997236,
2.97892388940601E-15));
#284111=CARTESIAN_POINT('Ctrl Pts',(-12.1623797632103,71.862499999723,3.95179673813154));
#284112=CARTESIAN_POINT('Ctrl Pts',(-9.83957192047913,72.0124999997224,
7.14886745759543));
#284113=CARTESIAN_POINT('Ctrl Pts',(-7.51676407774791,72.1624999997218,
10.3459381770593));
#284114=CARTESIAN_POINT('Ctrl Pts',(-3.75838203887398,72.3124999997212,
11.5671105274575));
#284115=CARTESIAN_POINT('Ctrl Pts',(-5.18598316642274E-14,72.4624999997206,
12.7882828778556));
#284116=CARTESIAN_POINT('Ctrl Pts',(3.75838203887388,72.61249999972,11.5671105274575));
#284117=CARTESIAN_POINT('Ctrl Pts',(7.51676407774781,72.7624999997194,10.3459381770593));
#284118=CARTESIAN_POINT('Ctrl Pts',(9.83957192047902,72.9124999997188,7.14886745759543));
#284119=CARTESIAN_POINT('Ctrl Pts',(12.1623797632102,73.0624999997182,3.95179673813153));
#284120=CARTESIAN_POINT('Ctrl Pts',(12.1623797632102,73.2124999997176,-1.489461944703E-15));
#284121=CARTESIAN_POINT('Ctrl Pts',(12.1623797632102,73.362499999717,-3.95179673813154));
#284122=CARTESIAN_POINT('Ctrl Pts',(9.83957192047902,73.5124999997164,-7.14886745759543));
#284123=CARTESIAN_POINT('Ctrl Pts',(7.5167640777478,73.6624999997158,-10.3459381770593));
#284124=CARTESIAN_POINT('Ctrl Pts',(3.75838203887387,73.8124999997152,-11.5671105274575));
#284125=CARTESIAN_POINT('Ctrl Pts',(-5.58559122386497E-14,73.9624999997146,
-12.7882828778556));
#284126=CARTESIAN_POINT('Ctrl Pts',(-3.75838203887398,74.112499999714,-11.5671105274575));
#284127=CARTESIAN_POINT('Ctrl Pts',(-7.51676407774791,74.2624999997134,
-10.3459381770593));
#284128=CARTESIAN_POINT('Ctrl Pts',(-9.83957192047913,74.4124999997128,
-7.14886745759543));
#284129=CARTESIAN_POINT('Ctrl Pts',(-12.1623797632103,74.5624999997122,
-3.95179673813153));
#284130=CARTESIAN_POINT('Ctrl Pts',(-12.1623797632103,74.7124999997116,
2.97892388940601E-15));
#284131=CARTESIAN_POINT('Ctrl Pts',(-12.1623797632103,74.862499999711,3.95179673813154));
#284132=CARTESIAN_POINT('Ctrl Pts',(-9.83957192047913,75.0124999997104,
7.14886745759543));
#284133=CARTESIAN_POINT('Ctrl Pts',(-7.51676407774791,75.1624999997098,
10.3459381770593));
#284134=CARTESIAN_POINT('Ctrl Pts',(-3.75838203887398,75.3124999997092,
11.5671105274575));
#284135=CARTESIAN_POINT('Ctrl Pts',(-5.35875409358893E-14,75.4624999997086,
12.7882828778556));
#284136=CARTESIAN_POINT('Ctrl Pts',(3.75838203887388,75.612499999708,11.5671105274575));
#284137=CARTESIAN_POINT('Ctrl Pts',(7.5167640777478,75.7624999997074,10.3459381770593));
#284138=CARTESIAN_POINT('Ctrl Pts',(9.83957192047902,75.9124999997068,7.14886745759543));
#284139=CARTESIAN_POINT('Ctrl Pts',(12.1623797632102,76.0624999997062,3.95179673813153));
#284140=CARTESIAN_POINT('Ctrl Pts',(12.1623797632102,76.2124999997056,-1.489461944703E-15));
#284141=CARTESIAN_POINT('Ctrl Pts',(12.1623797632102,76.362499999705,-3.95179673813154));
#284142=CARTESIAN_POINT('Ctrl Pts',(9.83957192047902,76.5124999997044,-7.14886745759543));
#284143=CARTESIAN_POINT('Ctrl Pts',(7.5167640777478,76.6624999997038,-10.3459381770593));
#284144=CARTESIAN_POINT('Ctrl Pts',(3.75838203887387,76.8124999997032,-11.5671105274575));
#284145=CARTESIAN_POINT('Ctrl Pts',(-5.75836215103115E-14,76.9624999997026,
-12.7882828778556));
#284146=CARTESIAN_POINT('Ctrl Pts',(-3.75838203887399,77.112499999702,-11.5671105274575));
#284147=CARTESIAN_POINT('Ctrl Pts',(-7.51676407774791,77.2624999997014,
-10.3459381770593));
#284148=CARTESIAN_POINT('Ctrl Pts',(-9.83957192047913,77.4124999997008,
-7.14886745759543));
#284149=CARTESIAN_POINT('Ctrl Pts',(-12.1623797632103,77.5624999997002,
-3.95179673813153));
#284150=CARTESIAN_POINT('Ctrl Pts',(-12.1623797632103,77.7124999996996,
2.97892388940601E-15));
#284151=CARTESIAN_POINT('Ctrl Pts',(-12.1623797632103,77.862499999699,3.95179673813154));
#284152=CARTESIAN_POINT('Ctrl Pts',(-9.83957192047913,78.0124999996984,
7.14886745759543));
#284153=CARTESIAN_POINT('Ctrl Pts',(-7.51676407774791,78.1624999996978,
10.3459381770593));
#284154=CARTESIAN_POINT('Ctrl Pts',(-3.75838203887398,78.3124999996972,
11.5671105274575));
#284155=CARTESIAN_POINT('Ctrl Pts',(-5.53152502075511E-14,78.4624999996966,
12.7882828778556));
#284156=CARTESIAN_POINT('Ctrl Pts',(3.75838203887387,78.612499999696,11.5671105274575));
#284157=CARTESIAN_POINT('Ctrl Pts',(7.5167640777478,78.7624999996954,10.3459381770593));
#284158=CARTESIAN_POINT('Ctrl Pts',(9.83957192047902,78.9124999996948,7.14886745759543));
#284159=CARTESIAN_POINT('Ctrl Pts',(12.1623797632102,79.0624999996942,3.95179673813153));
#284160=CARTESIAN_POINT('Ctrl Pts',(12.1623797632102,79.2124999996936,-1.489461944703E-15));
#284161=CARTESIAN_POINT('Ctrl Pts',(12.1623797632102,79.362499999693,-3.95179673813154));
#284162=CARTESIAN_POINT('Ctrl Pts',(9.83957192047902,79.5124999996924,-7.14886745759543));
#284163=CARTESIAN_POINT('Ctrl Pts',(7.5167640777478,79.6624999996918,-10.3459381770593));
#284164=CARTESIAN_POINT('Ctrl Pts',(3.75838203887387,79.8124999996912,-11.5671105274575));
#284165=CARTESIAN_POINT('Ctrl Pts',(-5.93113307819734E-14,79.9624999996906,
-12.7882828778556));
#284166=CARTESIAN_POINT('Ctrl Pts',(-3.75838203887399,80.11249999969,-11.5671105274575));
#284167=CARTESIAN_POINT('Ctrl Pts',(-7.51676407774791,80.2624999996894,
-10.3459381770593));
#284168=CARTESIAN_POINT('Ctrl Pts',(-9.83957192047913,80.4124999996888,
-7.14886745759543));
#284169=CARTESIAN_POINT('Ctrl Pts',(-12.1623797632104,80.5624999996882,
-3.95179673813153));
#284170=CARTESIAN_POINT('Ctrl Pts',(-12.1623797632104,80.7124999996876,
2.97892388940601E-15));
#284171=CARTESIAN_POINT('Ctrl Pts',(-12.1623797632104,80.862499999687,3.95179673813154));
#284172=CARTESIAN_POINT('Ctrl Pts',(-9.83957192047913,81.0124999996864,
7.14886745759543));
#284173=CARTESIAN_POINT('Ctrl Pts',(-7.51676407774791,81.1624999996858,
10.3459381770593));
#284174=CARTESIAN_POINT('Ctrl Pts',(-3.75838203887399,81.3124999996852,
11.5671105274575));
#284175=CARTESIAN_POINT('Ctrl Pts',(-5.70429594792129E-14,81.4624999996846,
12.7882828778556));
#284176=CARTESIAN_POINT('Ctrl Pts',(3.75838203887387,81.612499999684,11.5671105274575));
#284177=CARTESIAN_POINT('Ctrl Pts',(7.5167640777478,81.7624999996834,10.3459381770593));
#284178=CARTESIAN_POINT('Ctrl Pts',(9.83957192047902,81.9124999996828,7.14886745759543));
#284179=CARTESIAN_POINT('Ctrl Pts',(12.1623797632102,82.0624999996822,3.95179673813153));
#284180=CARTESIAN_POINT('Ctrl Pts',(12.1623797632102,82.2124999996816,-1.489461944703E-15));
#284181=CARTESIAN_POINT('Ctrl Pts',(12.1623797632102,82.362499999681,-3.95179673813154));
#284182=CARTESIAN_POINT('Ctrl Pts',(9.83957192047902,82.5124999996804,-7.14886745759543));
#284183=CARTESIAN_POINT('Ctrl Pts',(7.5167640777478,82.6624999996798,-10.3459381770593));
#284184=CARTESIAN_POINT('Ctrl Pts',(3.75838203887387,82.8124999996792,-11.5671105274575));
#284185=CARTESIAN_POINT('Ctrl Pts',(-6.10390400536352E-14,82.9624999996786,
-12.7882828778556));
#284186=CARTESIAN_POINT('Ctrl Pts',(-3.75838203887399,83.112499999678,-11.5671105274575));
#284187=CARTESIAN_POINT('Ctrl Pts',(-7.51676407774792,83.2624999996774,
-10.3459381770593));
#284188=CARTESIAN_POINT('Ctrl Pts',(-9.83957192047914,83.4124999996768,
-7.14886745759543));
#284189=CARTESIAN_POINT('Ctrl Pts',(-12.1623797632104,83.5624999996762,
-3.95179673813153));
#284190=CARTESIAN_POINT('Ctrl Pts',(-12.1623797632104,83.7124999996756,
2.97892388940601E-15));
#284191=CARTESIAN_POINT('Ctrl Pts',(-12.1623797632104,83.862499999675,3.95179673813154));
#284192=CARTESIAN_POINT('Ctrl Pts',(-9.83957192047913,84.0124999996744,
7.14886745759543));
#284193=CARTESIAN_POINT('Ctrl Pts',(-7.51676407774791,84.1624999996738,
10.3459381770593));
#284194=CARTESIAN_POINT('Ctrl Pts',(-3.75838203887399,84.3124999996732,
11.5671105274575));
#284195=CARTESIAN_POINT('Ctrl Pts',(-5.87706687508748E-14,84.4624999996726,
12.7882828778556));
#284196=CARTESIAN_POINT('Ctrl Pts',(3.75838203887387,84.6124999996721,11.5671105274575));
#284197=CARTESIAN_POINT('Ctrl Pts',(7.5167640777478,84.7624999996714,10.3459381770593));
#284198=CARTESIAN_POINT('Ctrl Pts',(9.83957192047902,84.9124999996708,7.14886745759543));
#284199=CARTESIAN_POINT('Ctrl Pts',(12.1623797632102,85.0624999996702,3.95179673813153));
#284200=CARTESIAN_POINT('Ctrl Pts',(12.1623797632102,85.2124999996696,-1.489461944703E-15));
#284201=CARTESIAN_POINT('Ctrl Pts',(12.1623797632102,85.362499999669,-3.95179673813154));
#284202=CARTESIAN_POINT('Ctrl Pts',(9.83957192047901,85.5124999996684,-7.14886745759543));
#284203=CARTESIAN_POINT('Ctrl Pts',(7.5167640777478,85.6624999996678,-10.3459381770593));
#284204=CARTESIAN_POINT('Ctrl Pts',(3.75838203887387,85.8124999996672,-11.5671105274575));
#284205=CARTESIAN_POINT('Ctrl Pts',(-6.27667493252971E-14,85.9624999996666,
-12.7882828778556));
#284206=CARTESIAN_POINT('Ctrl Pts',(-3.75838203887399,86.112499999666,-11.5671105274575));
#284207=CARTESIAN_POINT('Ctrl Pts',(-7.51676407774792,86.2624999996654,
-10.3459381770593));
#284208=CARTESIAN_POINT('Ctrl Pts',(-9.83957192047914,86.4124999996648,
-7.14886745759543));
#284209=CARTESIAN_POINT('Ctrl Pts',(-12.1623797632104,86.5624999996642,
-3.95179673813153));
#284210=CARTESIAN_POINT('Ctrl Pts',(-12.1623797632104,86.7124999996636,
2.97892388940601E-15));
#284211=CARTESIAN_POINT('Ctrl Pts',(-12.1623797632104,86.862499999663,3.95179673813154));
#284212=CARTESIAN_POINT('Ctrl Pts',(-9.83957192047914,87.0124999996624,
7.14886745759543));
#284213=CARTESIAN_POINT('Ctrl Pts',(-7.51676407774792,87.1624999996618,
10.3459381770593));
#284214=CARTESIAN_POINT('Ctrl Pts',(-3.75838203887399,87.3124999996612,
11.5671105274575));
#284215=CARTESIAN_POINT('Ctrl Pts',(-6.04983780225366E-14,87.4624999996606,
12.7882828778556));
#284216=CARTESIAN_POINT('Ctrl Pts',(3.75838203887387,87.61249999966,11.5671105274575));
#284217=CARTESIAN_POINT('Ctrl Pts',(7.5167640777478,87.7624999996594,10.3459381770593));
#284218=CARTESIAN_POINT('Ctrl Pts',(9.83957192047901,87.9124999996588,7.14886745759543));
#284219=CARTESIAN_POINT('Ctrl Pts',(12.1623797632102,88.0624999996582,3.95179673813153));
#284220=CARTESIAN_POINT('Ctrl Pts',(12.1623797632102,88.2124999996576,-1.489461944703E-15));
#284221=CARTESIAN_POINT('Ctrl Pts',(12.1623797632102,88.362499999657,-3.95179673813154));
#284222=CARTESIAN_POINT('Ctrl Pts',(9.83957192047901,88.5124999996564,-7.14886745759543));
#284223=CARTESIAN_POINT('Ctrl Pts',(7.51676407774779,88.6624999996558,-10.3459381770593));
#284224=CARTESIAN_POINT('Ctrl Pts',(3.75838203887386,88.8124999996552,-11.5671105274575));
#284225=CARTESIAN_POINT('Ctrl Pts',(-6.44944585969589E-14,88.9624999996546,
-12.7882828778556));
#284226=CARTESIAN_POINT('Ctrl Pts',(-3.75838203887399,89.112499999654,-11.5671105274575));
#284227=CARTESIAN_POINT('Ctrl Pts',(-7.51676407774792,89.2624999996534,
-10.3459381770593));
#284228=CARTESIAN_POINT('Ctrl Pts',(-9.83957192047914,89.4124999996528,
-7.14886745759543));
#284229=CARTESIAN_POINT('Ctrl Pts',(-12.1623797632104,89.5624999996522,
-3.95179673813153));
#284230=CARTESIAN_POINT('Ctrl Pts',(-12.1623797632104,89.7124999996516,
2.97892388940601E-15));
#284231=CARTESIAN_POINT('Ctrl Pts',(-12.1623797632104,89.862499999651,3.95179673813154));
#284232=CARTESIAN_POINT('Ctrl Pts',(-9.83957192047914,90.0124999996504,
7.14886745759543));
#284233=CARTESIAN_POINT('Ctrl Pts',(-7.51676407774792,90.1624999996498,
10.3459381770593));
#284234=CARTESIAN_POINT('Ctrl Pts',(-3.75838203887399,90.3124999996492,
11.5671105274575));
#284235=CARTESIAN_POINT('Ctrl Pts',(-6.22260872941985E-14,90.4624999996486,
12.7882828778556));
#284236=CARTESIAN_POINT('Ctrl Pts',(3.75838203887387,90.612499999648,11.5671105274575));
#284237=CARTESIAN_POINT('Ctrl Pts',(7.5167640777478,90.7624999996474,10.3459381770593));
#284238=CARTESIAN_POINT('Ctrl Pts',(9.83957192047901,90.9124999996468,7.14886745759543));
#284239=CARTESIAN_POINT('Ctrl Pts',(12.1623797632102,91.0624999996462,3.95179673813153));
#284240=CARTESIAN_POINT('Ctrl Pts',(12.1623797632102,91.2124999996456,-1.489461944703E-15));
#284241=CARTESIAN_POINT('Ctrl Pts',(12.1623797632102,91.362499999645,-3.95179673813154));
#284242=CARTESIAN_POINT('Ctrl Pts',(9.83957192047901,91.5124999996444,-7.14886745759543));
#284243=CARTESIAN_POINT('Ctrl Pts',(7.51676407774779,91.6624999996438,-10.3459381770593));
#284244=CARTESIAN_POINT('Ctrl Pts',(3.75838203887386,91.8124999996432,-11.5671105274575));
#284245=CARTESIAN_POINT('Ctrl Pts',(-6.62221678686207E-14,91.9624999996426,
-12.7882828778556));
#284246=CARTESIAN_POINT('Ctrl Pts',(-3.75838203887399,92.112499999642,-11.5671105274575));
#284247=CARTESIAN_POINT('Ctrl Pts',(-7.51676407774792,92.2624999996414,
-10.3459381770593));
#284248=CARTESIAN_POINT('Ctrl Pts',(-9.83957192047914,92.4124999996408,
-7.14886745759543));
#284249=CARTESIAN_POINT('Ctrl Pts',(-12.1623797632104,92.5624999996402,
-3.95179673813153));
#284250=CARTESIAN_POINT('Ctrl Pts',(-12.1623797632104,92.7124999996396,
2.97892388940601E-15));
#284251=CARTESIAN_POINT('Ctrl Pts',(-12.1623797632104,92.862499999639,3.95179673813154));
#284252=CARTESIAN_POINT('Ctrl Pts',(-9.83957192047914,93.0124999996384,
7.14886745759543));
#284253=CARTESIAN_POINT('Ctrl Pts',(-7.51676407774792,93.1624999996378,
10.3459381770593));
#284254=CARTESIAN_POINT('Ctrl Pts',(-3.75838203887399,93.3124999996372,
11.5671105274575));
#284255=CARTESIAN_POINT('Ctrl Pts',(-6.39537965658603E-14,93.4624999996366,
12.7882828778556));
#284256=CARTESIAN_POINT('Ctrl Pts',(3.75838203887386,93.612499999636,11.5671105274575));
#284257=CARTESIAN_POINT('Ctrl Pts',(7.51676407774779,93.7624999996354,10.3459381770593));
#284258=CARTESIAN_POINT('Ctrl Pts',(9.83957192047901,93.9124999996348,7.14886745759543));
#284259=CARTESIAN_POINT('Ctrl Pts',(12.1623797632102,94.0624999996342,3.95179673813153));
#284260=CARTESIAN_POINT('Ctrl Pts',(12.1623797632102,94.2124999996336,-1.489461944703E-15));
#284261=CARTESIAN_POINT('Ctrl Pts',(12.1623797632102,94.362499999633,-3.95179673813154));
#284262=CARTESIAN_POINT('Ctrl Pts',(9.83957192047901,94.5124999996324,-7.14886745759543));
#284263=CARTESIAN_POINT('Ctrl Pts',(7.51676407774779,94.6624999996318,-10.3459381770593));
#284264=CARTESIAN_POINT('Ctrl Pts',(3.75838203887386,94.8124999996312,-11.5671105274575));
#284265=CARTESIAN_POINT('Ctrl Pts',(-6.79498771402825E-14,94.9624999996306,
-12.7882828778556));
#284266=CARTESIAN_POINT('Ctrl Pts',(-3.758382038874,95.11249999963,-11.5671105274575));
#284267=CARTESIAN_POINT('Ctrl Pts',(-7.51676407774792,95.2624999996294,
-10.3459381770593));
#284268=CARTESIAN_POINT('Ctrl Pts',(-9.83957192047914,95.4124999996288,
-7.14886745759543));
#284269=CARTESIAN_POINT('Ctrl Pts',(-12.1623797632104,95.5624999996282,
-3.95179673813153));
#284270=CARTESIAN_POINT('Ctrl Pts',(-12.1623797632104,95.7124999996276,
2.97892388940601E-15));
#284271=CARTESIAN_POINT('Ctrl Pts',(-12.1623797632104,95.862499999627,3.95179673813154));
#284272=CARTESIAN_POINT('Ctrl Pts',(-9.83957192047914,96.0124999996264,
7.14886745759543));
#284273=CARTESIAN_POINT('Ctrl Pts',(-7.51676407774792,96.1624999996258,
10.3459381770593));
#284274=CARTESIAN_POINT('Ctrl Pts',(-3.75838203887399,96.3124999996252,
11.5671105274575));
#284275=CARTESIAN_POINT('Ctrl Pts',(-6.56815058375222E-14,96.4624999996246,
12.7882828778556));
#284276=CARTESIAN_POINT('Ctrl Pts',(3.75838203887386,96.612499999624,11.5671105274575));
#284277=CARTESIAN_POINT('Ctrl Pts',(7.51676407774779,96.7624999996234,10.3459381770593));
#284278=CARTESIAN_POINT('Ctrl Pts',(9.83957192047901,96.9124999996228,7.14886745759543));
#284279=CARTESIAN_POINT('Ctrl Pts',(12.1623797632102,97.0624999996222,3.95179673813153));
#284280=CARTESIAN_POINT('Ctrl Pts',(12.1623797632102,97.2124999996216,-1.489461944703E-15));
#284281=CARTESIAN_POINT('Ctrl Pts',(12.1623797632102,97.3624999996211,-3.95179673813154));
#284282=CARTESIAN_POINT('Ctrl Pts',(9.83957192047901,97.5124999996204,-7.14886745759543));
#284283=CARTESIAN_POINT('Ctrl Pts',(7.51676407774779,97.6624999996198,-10.3459381770593));
#284284=CARTESIAN_POINT('Ctrl Pts',(3.75838203887386,97.8124999996192,-11.5671105274575));
#284285=CARTESIAN_POINT('Ctrl Pts',(-6.96775864119444E-14,97.9624999996187,
-12.7882828778556));
#284286=CARTESIAN_POINT('Ctrl Pts',(-3.758382038874,98.112499999618,-11.5671105274575));
#284287=CARTESIAN_POINT('Ctrl Pts',(-7.51676407774793,98.2624999996174,
-10.3459381770593));
#284288=CARTESIAN_POINT('Ctrl Pts',(-9.83957192047914,98.4124999996168,
-7.14886745759543));
#284289=CARTESIAN_POINT('Ctrl Pts',(-12.1623797632104,98.5624999996162,
-3.95179673813153));
#284290=CARTESIAN_POINT('Ctrl Pts',(-12.1623797632104,98.7124999996156,
2.97892388940601E-15));
#284291=CARTESIAN_POINT('Ctrl Pts',(-12.1623797632104,98.862499999615,3.95179673813154));
#284292=CARTESIAN_POINT('Ctrl Pts',(-9.83957192047914,99.0124999996144,
7.14886745759543));
#284293=CARTESIAN_POINT('Ctrl Pts',(-7.51676407774792,99.1624999996138,
10.3459381770593));
#284294=CARTESIAN_POINT('Ctrl Pts',(-3.758382038874,99.3124999996132,11.5671105274575));
#284295=CARTESIAN_POINT('Ctrl Pts',(-6.7409215109184E-14,99.4624999996126,
12.7882828778556));
#284296=CARTESIAN_POINT('Ctrl Pts',(3.75838203887386,99.612499999612,11.5671105274575));
#284297=CARTESIAN_POINT('Ctrl Pts',(7.51676407774779,99.7624999996114,10.3459381770593));
#284298=CARTESIAN_POINT('Ctrl Pts',(9.83957192047901,99.9124999996108,7.14886745759543));
#284299=CARTESIAN_POINT('Ctrl Pts',(12.1623797632102,100.06249999961,3.95179673813153));
#284300=CARTESIAN_POINT('Ctrl Pts',(12.1623797632102,100.21249999961,-1.489461944703E-15));
#284301=CARTESIAN_POINT('Ctrl Pts',(12.1623797632102,100.362499999609,-3.95179673813154));
#284302=CARTESIAN_POINT('Ctrl Pts',(9.839571920479,100.512499999608,-7.14886745759543));
#284303=CARTESIAN_POINT('Ctrl Pts',(7.51676407774779,100.662499999608,-10.3459381770593));
#284304=CARTESIAN_POINT('Ctrl Pts',(3.75838203887386,100.812499999607,-11.5671105274575));
#284305=CARTESIAN_POINT('Ctrl Pts',(-7.14052956836063E-14,100.962499999607,
-12.7882828778556));
#284306=CARTESIAN_POINT('Ctrl Pts',(-3.758382038874,101.112499999606,-11.5671105274575));
#284307=CARTESIAN_POINT('Ctrl Pts',(-7.51676407774793,101.262499999605,
-10.3459381770593));
#284308=CARTESIAN_POINT('Ctrl Pts',(-9.83957192047915,101.412499999605,
-7.14886745759543));
#284309=CARTESIAN_POINT('Ctrl Pts',(-12.1623797632104,101.562499999604,
-3.95179673813153));
#284310=CARTESIAN_POINT('Ctrl Pts',(-12.1623797632104,101.712499999604,
2.97892388940601E-15));
#284311=CARTESIAN_POINT('Ctrl Pts',(-12.1623797632104,101.862499999603,
3.95179673813154));
#284312=CARTESIAN_POINT('Ctrl Pts',(-9.83957192047914,102.012499999602,
7.14886745759543));
#284313=CARTESIAN_POINT('Ctrl Pts',(-7.51676407774793,102.162499999602,
10.3459381770593));
#284314=CARTESIAN_POINT('Ctrl Pts',(-3.758382038874,102.312499999601,11.5671105274575));
#284315=CARTESIAN_POINT('Ctrl Pts',(-6.91369243808458E-14,102.462499999601,
12.7882828778556));
#284316=CARTESIAN_POINT('Ctrl Pts',(3.75838203887386,102.6124999996,11.5671105274575));
#284317=CARTESIAN_POINT('Ctrl Pts',(7.51676407774779,102.762499999599,10.3459381770593));
#284318=CARTESIAN_POINT('Ctrl Pts',(9.839571920479,102.912499999599,7.14886745759543));
#284319=CARTESIAN_POINT('Ctrl Pts',(12.1623797632102,103.062499999598,3.95179673813153));
#284320=CARTESIAN_POINT('Ctrl Pts',(12.1623797632102,103.212499999598,-1.489461944703E-15));
#284321=CARTESIAN_POINT('Ctrl Pts',(12.1623797632102,103.362499999597,-3.95179673813154));
#284322=CARTESIAN_POINT('Ctrl Pts',(9.839571920479,103.512499999596,-7.14886745759543));
#284323=CARTESIAN_POINT('Ctrl Pts',(7.51676407774779,103.662499999596,-10.3459381770593));
#284324=CARTESIAN_POINT('Ctrl Pts',(3.75838203887386,103.812499999595,-11.5671105274575));
#284325=CARTESIAN_POINT('Ctrl Pts',(-7.31330049552681E-14,103.962499999595,
-12.7882828778556));
#284326=CARTESIAN_POINT('Ctrl Pts',(-3.758382038874,104.112499999594,-11.5671105274575));
#284327=CARTESIAN_POINT('Ctrl Pts',(-7.51676407774793,104.262499999593,
-10.3459381770593));
#284328=CARTESIAN_POINT('Ctrl Pts',(-9.83957192047915,104.412499999593,
-7.14886745759543));
#284329=CARTESIAN_POINT('Ctrl Pts',(-12.1623797632104,104.562499999592,
-3.95179673813153));
#284330=CARTESIAN_POINT('Ctrl Pts',(-12.1623797632104,104.712499999592,
2.97892388940601E-15));
#284331=CARTESIAN_POINT('Ctrl Pts',(-12.1623797632104,104.862499999591,
3.95179673813154));
#284332=CARTESIAN_POINT('Ctrl Pts',(-9.83957192047915,105.01249999959,7.14886745759543));
#284333=CARTESIAN_POINT('Ctrl Pts',(-7.51676407774793,105.16249999959,10.3459381770593));
#284334=CARTESIAN_POINT('Ctrl Pts',(-3.758382038874,105.312499999589,11.5671105274575));
#284335=CARTESIAN_POINT('Ctrl Pts',(-7.08646336525076E-14,105.462499999589,
12.7882828778556));
#284336=CARTESIAN_POINT('Ctrl Pts',(3.75838203887386,105.612499999588,11.5671105274575));
#284337=CARTESIAN_POINT('Ctrl Pts',(7.51676407774779,105.762499999587,10.3459381770593));
#284338=CARTESIAN_POINT('Ctrl Pts',(9.839571920479,105.912499999587,7.14886745759543));
#284339=CARTESIAN_POINT('Ctrl Pts',(12.1623797632102,106.062499999586,3.95179673813153));
#284340=CARTESIAN_POINT('Ctrl Pts',(12.1623797632102,106.212499999586,-1.489461944703E-15));
#284341=CARTESIAN_POINT('Ctrl Pts',(12.1623797632102,106.362499999585,-3.95179673813154));
#284342=CARTESIAN_POINT('Ctrl Pts',(9.839571920479,106.512499999584,-7.14886745759543));
#284343=CARTESIAN_POINT('Ctrl Pts',(7.51676407774778,106.662499999584,-10.3459381770593));
#284344=CARTESIAN_POINT('Ctrl Pts',(3.75838203887385,106.812499999583,-11.5671105274575));
#284345=CARTESIAN_POINT('Ctrl Pts',(-7.48607142269299E-14,106.962499999583,
-12.7882828778556));
#284346=CARTESIAN_POINT('Ctrl Pts',(-3.758382038874,107.112499999582,-11.5671105274575));
#284347=CARTESIAN_POINT('Ctrl Pts',(-7.51676407774793,107.262499999581,
-10.3459381770593));
#284348=CARTESIAN_POINT('Ctrl Pts',(-9.83957192047915,107.412499999581,
-7.14886745759543));
#284349=CARTESIAN_POINT('Ctrl Pts',(-12.1623797632104,107.56249999958,-3.95179673813153));
#284350=CARTESIAN_POINT('Ctrl Pts',(-12.1623797632104,107.71249999958,2.97892388940601E-15));
#284351=CARTESIAN_POINT('Ctrl Pts',(-12.1623797632104,107.862499999579,
3.95179673813154));
#284352=CARTESIAN_POINT('Ctrl Pts',(-9.83957192047915,108.012499999578,
7.14886745759543));
#284353=CARTESIAN_POINT('Ctrl Pts',(-7.51676407774793,108.162499999578,
10.3459381770593));
#284354=CARTESIAN_POINT('Ctrl Pts',(-3.758382038874,108.312499999577,11.5671105274575));
#284355=CARTESIAN_POINT('Ctrl Pts',(-7.25923429241695E-14,108.462499999577,
12.7882828778556));
#284356=CARTESIAN_POINT('Ctrl Pts',(3.75838203887386,108.612499999576,11.5671105274575));
#284357=CARTESIAN_POINT('Ctrl Pts',(7.51676407774779,108.762499999575,10.3459381770593));
#284358=CARTESIAN_POINT('Ctrl Pts',(9.839571920479,108.912499999575,7.14886745759543));
#284359=CARTESIAN_POINT('Ctrl Pts',(12.1623797632102,109.062499999574,3.95179673813153));
#284360=CARTESIAN_POINT('Ctrl Pts',(12.1623797632102,109.212499999574,-1.489461944703E-15));
#284361=CARTESIAN_POINT('Ctrl Pts',(12.1623797632102,109.362499999573,-3.95179673813154));
#284362=CARTESIAN_POINT('Ctrl Pts',(9.839571920479,109.512499999572,-7.14886745759543));
#284363=CARTESIAN_POINT('Ctrl Pts',(7.51676407774778,109.662499999572,-10.3459381770593));
#284364=CARTESIAN_POINT('Ctrl Pts',(3.75838203887385,109.812499999571,-11.5671105274575));
#284365=CARTESIAN_POINT('Ctrl Pts',(-7.65884234985918E-14,109.962499999571,
-12.7882828778556));
#284366=CARTESIAN_POINT('Ctrl Pts',(-3.75838203887401,110.11249999957,-11.5671105274575));
#284367=CARTESIAN_POINT('Ctrl Pts',(-7.51676407774793,110.262499999569,
-10.3459381770593));
#284368=CARTESIAN_POINT('Ctrl Pts',(-9.83957192047915,110.412499999569,
-7.14886745759543));
#284369=CARTESIAN_POINT('Ctrl Pts',(-12.1623797632104,110.562499999568,
-3.95179673813153));
#284370=CARTESIAN_POINT('Ctrl Pts',(-12.1623797632104,110.712499999568,
2.97892388940601E-15));
#284371=CARTESIAN_POINT('Ctrl Pts',(-12.1623797632104,110.862499999567,
3.95179673813154));
#284372=CARTESIAN_POINT('Ctrl Pts',(-9.83957192047915,111.012499999566,
7.14886745759543));
#284373=CARTESIAN_POINT('Ctrl Pts',(-7.51676407774793,111.162499999566,
10.3459381770593));
#284374=CARTESIAN_POINT('Ctrl Pts',(-3.758382038874,111.312499999565,11.5671105274575));
#284375=CARTESIAN_POINT('Ctrl Pts',(-7.43200521958313E-14,111.462499999565,
12.7882828778556));
#284376=CARTESIAN_POINT('Ctrl Pts',(3.75838203887385,111.612499999564,11.5671105274575));
#284377=CARTESIAN_POINT('Ctrl Pts',(7.51676407774778,111.762499999563,10.3459381770593));
#284378=CARTESIAN_POINT('Ctrl Pts',(9.839571920479,111.912499999563,7.14886745759543));
#284379=CARTESIAN_POINT('Ctrl Pts',(12.1623797632102,112.062499999562,3.95179673813153));
#284380=CARTESIAN_POINT('Ctrl Pts',(12.1623797632102,112.212499999562,-1.489461944703E-15));
#284381=CARTESIAN_POINT('Ctrl Pts',(12.1623797632102,112.362499999561,-3.95179673813154));
#284382=CARTESIAN_POINT('Ctrl Pts',(9.839571920479,112.51249999956,-7.14886745759543));
#284383=CARTESIAN_POINT('Ctrl Pts',(7.51676407774778,112.66249999956,-10.3459381770593));
#284384=CARTESIAN_POINT('Ctrl Pts',(3.75838203887385,112.812499999559,-11.5671105274575));
#284385=CARTESIAN_POINT('Ctrl Pts',(-7.83161327702536E-14,112.962499999559,
-12.7882828778556));
#284386=CARTESIAN_POINT('Ctrl Pts',(-3.75838203887401,113.112499999558,
-11.5671105274575));
#284387=CARTESIAN_POINT('Ctrl Pts',(-7.51676407774793,113.262499999557,
-10.3459381770593));
#284388=CARTESIAN_POINT('Ctrl Pts',(-9.83957192047915,113.412499999557,
-7.14886745759543));
#284389=CARTESIAN_POINT('Ctrl Pts',(-12.1623797632104,113.562499999556,
-3.95179673813153));
#284390=CARTESIAN_POINT('Ctrl Pts',(-12.1623797632104,113.712499999556,
2.97892388940601E-15));
#284391=CARTESIAN_POINT('Ctrl Pts',(-12.1623797632104,113.862499999555,
3.95179673813154));
#284392=CARTESIAN_POINT('Ctrl Pts',(-9.83957192047915,114.012499999554,
7.14886745759543));
#284393=CARTESIAN_POINT('Ctrl Pts',(-7.51676407774793,114.162499999554,
10.3459381770593));
#284394=CARTESIAN_POINT('Ctrl Pts',(-3.758382038874,114.312499999553,11.5671105274575));
#284395=CARTESIAN_POINT('Ctrl Pts',(-7.60477614674932E-14,114.462499999553,
12.7882828778556));
#284396=CARTESIAN_POINT('Ctrl Pts',(3.75838203887385,114.612499999552,11.5671105274575));
#284397=CARTESIAN_POINT('Ctrl Pts',(7.51676407774778,114.762499999551,10.3459381770593));
#284398=CARTESIAN_POINT('Ctrl Pts',(9.839571920479,114.912499999551,7.14886745759543));
#284399=CARTESIAN_POINT('Ctrl Pts',(12.1623797632102,115.06249999955,3.95179673813153));
#284400=CARTESIAN_POINT('Ctrl Pts',(12.1623797632102,115.21249999955,-1.489461944703E-15));
#284401=CARTESIAN_POINT('Ctrl Pts',(12.1623797632102,115.362499999549,-3.95179673813154));
#284402=CARTESIAN_POINT('Ctrl Pts',(9.839571920479,115.512499999548,-7.14886745759543));
#284403=CARTESIAN_POINT('Ctrl Pts',(7.51676407774778,115.662499999548,-10.3459381770593));
#284404=CARTESIAN_POINT('Ctrl Pts',(3.75838203887385,115.812499999547,-11.5671105274575));
#284405=CARTESIAN_POINT('Ctrl Pts',(-8.00438420419154E-14,115.962499999547,
-12.7882828778556));
#284406=CARTESIAN_POINT('Ctrl Pts',(-3.75838203887401,116.112499999546,
-11.5671105274575));
#284407=CARTESIAN_POINT('Ctrl Pts',(-7.51676407774794,116.262499999545,
-10.3459381770593));
#284408=CARTESIAN_POINT('Ctrl Pts',(-9.83957192047916,116.412499999545,
-7.14886745759543));
#284409=CARTESIAN_POINT('Ctrl Pts',(-12.1623797632104,116.562499999544,
-3.95179673813153));
#284410=CARTESIAN_POINT('Ctrl Pts',(-12.1623797632104,116.712499999544,
2.97892388940601E-15));
#284411=CARTESIAN_POINT('Ctrl Pts',(-12.1623797632104,116.862499999543,
3.95179673813154));
#284412=CARTESIAN_POINT('Ctrl Pts',(-9.83957192047915,117.012499999542,
7.14886745759543));
#284413=CARTESIAN_POINT('Ctrl Pts',(-7.51676407774793,117.162499999542,
10.3459381770593));
#284414=CARTESIAN_POINT('Ctrl Pts',(-3.75838203887401,117.312499999541,
11.5671105274575));
#284415=CARTESIAN_POINT('Ctrl Pts',(-7.7775470739155E-14,117.462499999541,
12.7882828778556));
#284416=CARTESIAN_POINT('Ctrl Pts',(3.75838203887385,117.61249999954,11.5671105274575));
#284417=CARTESIAN_POINT('Ctrl Pts',(7.51676407774778,117.762499999539,10.3459381770593));
#284418=CARTESIAN_POINT('Ctrl Pts',(9.839571920479,117.912499999539,7.14886745759543));
#284419=CARTESIAN_POINT('Ctrl Pts',(12.1623797632102,118.062499999538,3.95179673813153));
#284420=CARTESIAN_POINT('Ctrl Pts',(12.1623797632102,118.212499999538,-1.489461944703E-15));
#284421=CARTESIAN_POINT('Ctrl Pts',(12.1623797632102,118.362499999537,-3.95179673813154));
#284422=CARTESIAN_POINT('Ctrl Pts',(9.83957192047899,118.512499999536,-7.14886745759543));
#284423=CARTESIAN_POINT('Ctrl Pts',(7.51676407774778,118.662499999536,-10.3459381770593));
#284424=CARTESIAN_POINT('Ctrl Pts',(3.75838203887385,118.812499999535,-11.5671105274575));
#284425=CARTESIAN_POINT('Ctrl Pts',(-8.17715513135773E-14,118.962499999535,
-12.7882828778556));
#284426=CARTESIAN_POINT('Ctrl Pts',(-3.75838203887401,119.112499999534,
-11.5671105274575));
#284427=CARTESIAN_POINT('Ctrl Pts',(-7.51676407774794,119.262499999533,
-10.3459381770593));
#284428=CARTESIAN_POINT('Ctrl Pts',(-9.83957192047916,119.412499999533,
-7.14886745759543));
#284429=CARTESIAN_POINT('Ctrl Pts',(-12.1623797632104,119.562499999532,
-3.95179673813153));
#284430=CARTESIAN_POINT('Ctrl Pts',(-12.1623797632104,119.712499999532,
2.97892388940601E-15));
#284431=CARTESIAN_POINT('Ctrl Pts',(-12.1623797632104,119.862499999531,
3.95179673813154));
#284432=CARTESIAN_POINT('Ctrl Pts',(-9.83957192047916,120.01249999953,7.14886745759543));
#284433=CARTESIAN_POINT('Ctrl Pts',(-7.51676407774794,120.16249999953,10.3459381770593));
#284434=CARTESIAN_POINT('Ctrl Pts',(-3.75838203887401,120.312499999529,
11.5671105274575));
#284435=CARTESIAN_POINT('Ctrl Pts',(-7.95031800108169E-14,120.462499999529,
12.7882828778556));
#284436=CARTESIAN_POINT('Ctrl Pts',(3.75838203887385,120.612499999528,11.5671105274575));
#284437=CARTESIAN_POINT('Ctrl Pts',(7.51676407774778,120.762499999527,10.3459381770593));
#284438=CARTESIAN_POINT('Ctrl Pts',(9.83957192047899,120.912499999527,7.14886745759543));
#284439=CARTESIAN_POINT('Ctrl Pts',(12.1623797632102,121.062499999526,3.95179673813153));
#284440=CARTESIAN_POINT('Ctrl Pts',(12.1623797632102,121.212499999526,-1.489461944703E-15));
#284441=CARTESIAN_POINT('Ctrl Pts',(12.1623797632102,121.362499999525,-3.95179673813154));
#284442=CARTESIAN_POINT('Ctrl Pts',(9.83957192047899,121.512499999524,-7.14886745759543));
#284443=CARTESIAN_POINT('Ctrl Pts',(7.51676407774777,121.662499999524,-10.3459381770593));
#284444=CARTESIAN_POINT('Ctrl Pts',(3.75838203887385,121.812499999523,-11.5671105274575));
#284445=CARTESIAN_POINT('Ctrl Pts',(-8.34992605852391E-14,121.962499999523,
-12.7882828778556));
#284446=CARTESIAN_POINT('Ctrl Pts',(-3.75838203887401,122.112499999522,
-11.5671105274575));
#284447=CARTESIAN_POINT('Ctrl Pts',(-7.51676407774794,122.262499999521,
-10.3459381770593));
#284448=CARTESIAN_POINT('Ctrl Pts',(-9.83957192047916,122.412499999521,
-7.14886745759543));
#284449=CARTESIAN_POINT('Ctrl Pts',(-12.1623797632104,122.56249999952,-3.95179673813153));
#284450=CARTESIAN_POINT('Ctrl Pts',(-12.1623797632104,122.71249999952,2.97892388940601E-15));
#284451=CARTESIAN_POINT('Ctrl Pts',(-12.1623797632104,122.862499999519,
3.95179673813154));
#284452=CARTESIAN_POINT('Ctrl Pts',(-9.83957192047916,123.012499999518,
7.14886745759543));
#284453=CARTESIAN_POINT('Ctrl Pts',(-7.51676407774794,123.162499999518,
10.3459381770593));
#284454=CARTESIAN_POINT('Ctrl Pts',(-3.75838203887401,123.312499999517,
11.5671105274575));
#284455=CARTESIAN_POINT('Ctrl Pts',(-8.12308892824787E-14,123.462499999517,
12.7882828778556));
#284456=CARTESIAN_POINT('Ctrl Pts',(3.75838203887385,123.612499999516,11.5671105274575));
#284457=CARTESIAN_POINT('Ctrl Pts',(7.51676407774778,123.762499999515,10.3459381770593));
#284458=CARTESIAN_POINT('Ctrl Pts',(9.83957192047899,123.912499999515,7.14886745759543));
#284459=CARTESIAN_POINT('Ctrl Pts',(12.1623797632102,124.062499999514,3.95179673813153));
#284460=CARTESIAN_POINT('Ctrl Pts',(12.1623797632102,124.212499999514,-1.489461944703E-15));
#284461=CARTESIAN_POINT('Ctrl Pts',(12.1623797632102,124.362499999513,-3.95179673813154));
#284462=CARTESIAN_POINT('Ctrl Pts',(9.83957192047899,124.512499999512,-7.14886745759543));
#284463=CARTESIAN_POINT('Ctrl Pts',(7.51676407774777,124.662499999512,-10.3459381770593));
#284464=CARTESIAN_POINT('Ctrl Pts',(3.75838203887384,124.812499999511,-11.5671105274575));
#284465=CARTESIAN_POINT('Ctrl Pts',(-8.52269698569009E-14,124.962499999511,
-12.7882828778556));
#284466=CARTESIAN_POINT('Ctrl Pts',(-3.75838203887401,125.11249999951,-11.5671105274575));
#284467=CARTESIAN_POINT('Ctrl Pts',(-7.51676407774794,125.262499999509,
-10.3459381770593));
#284468=CARTESIAN_POINT('Ctrl Pts',(-9.83957192047916,125.412499999509,
-7.14886745759543));
#284469=CARTESIAN_POINT('Ctrl Pts',(-12.1623797632104,125.562499999508,
-3.95179673813153));
#284470=CARTESIAN_POINT('Ctrl Pts',(-12.1623797632104,125.712499999508,
2.97892388940601E-15));
#284471=CARTESIAN_POINT('Ctrl Pts',(-12.1623797632104,125.862499999507,
3.95179673813154));
#284472=CARTESIAN_POINT('Ctrl Pts',(-9.83957192047916,126.012499999506,
7.14886745759543));
#284473=CARTESIAN_POINT('Ctrl Pts',(-7.51676407774794,126.162499999506,
10.3459381770593));
#284474=CARTESIAN_POINT('Ctrl Pts',(-3.75838203887401,126.312499999505,
11.5671105274575));
#284475=CARTESIAN_POINT('Ctrl Pts',(-8.29585985541405E-14,126.462499999505,
12.7882828778556));
#284476=CARTESIAN_POINT('Ctrl Pts',(3.75838203887385,126.612499999504,11.5671105274575));
#284477=CARTESIAN_POINT('Ctrl Pts',(7.51676407774777,126.762499999503,10.3459381770593));
#284478=CARTESIAN_POINT('Ctrl Pts',(9.83957192047899,126.912499999503,7.14886745759543));
#284479=CARTESIAN_POINT('Ctrl Pts',(12.1623797632102,127.062499999502,3.95179673813153));
#284480=CARTESIAN_POINT('Ctrl Pts',(12.1623797632102,127.212499999502,-1.489461944703E-15));
#284481=CARTESIAN_POINT('Ctrl Pts',(12.1623797632102,127.362499999501,-3.95179673813154));
#284482=CARTESIAN_POINT('Ctrl Pts',(9.83957192047899,127.5124999995,-7.14886745759543));
#284483=CARTESIAN_POINT('Ctrl Pts',(7.51676407774777,127.6624999995,-10.3459381770593));
#284484=CARTESIAN_POINT('Ctrl Pts',(3.75838203887384,127.812499999499,-11.5671105274575));
#284485=CARTESIAN_POINT('Ctrl Pts',(-8.69546791285628E-14,127.962499999499,
-12.7882828778556));
#284486=CARTESIAN_POINT('Ctrl Pts',(-3.75838203887402,128.112499999498,
-11.5671105274575));
#284487=CARTESIAN_POINT('Ctrl Pts',(-7.51676407774795,128.262499999497,
-10.3459381770593));
#284488=CARTESIAN_POINT('Ctrl Pts',(-9.83957192047916,128.412499999497,
-7.14886745759543));
#284489=CARTESIAN_POINT('Ctrl Pts',(-12.1623797632104,128.562499999496,
-3.95179673813153));
#284490=CARTESIAN_POINT('Ctrl Pts',(-12.1623797632104,128.712499999496,
2.97892388940601E-15));
#284491=CARTESIAN_POINT('Ctrl Pts',(-12.1623797632104,128.862499999495,
3.95179673813154));
#284492=CARTESIAN_POINT('Ctrl Pts',(-9.83957192047916,129.012499999494,
7.14886745759543));
#284493=CARTESIAN_POINT('Ctrl Pts',(-7.51676407774794,129.162499999494,
10.3459381770593));
#284494=CARTESIAN_POINT('Ctrl Pts',(-3.75838203887401,129.312499999493,
11.5671105274575));
#284495=CARTESIAN_POINT('Ctrl Pts',(-8.46863078258024E-14,129.462499999493,
12.7882828778556));
#284496=CARTESIAN_POINT('Ctrl Pts',(3.75838203887384,129.612499999492,11.5671105274575));
#284497=CARTESIAN_POINT('Ctrl Pts',(7.51676407774777,129.762499999491,10.3459381770593));
#284498=CARTESIAN_POINT('Ctrl Pts',(9.83957192047899,129.912499999491,7.14886745759543));
#284499=CARTESIAN_POINT('Ctrl Pts',(12.1623797632102,130.06249999949,3.95179673813153));
#284500=CARTESIAN_POINT('Ctrl Pts',(12.1623797632102,130.21249999949,-1.489461944703E-15));
#284501=CARTESIAN_POINT('Ctrl Pts',(12.1623797632102,130.362499999489,-3.95179673813154));
#284502=CARTESIAN_POINT('Ctrl Pts',(9.83957192047899,130.512499999488,-7.14886745759543));
#284503=CARTESIAN_POINT('Ctrl Pts',(7.51676407774777,130.662499999488,-10.3459381770593));
#284504=CARTESIAN_POINT('Ctrl Pts',(3.75838203887384,130.812499999487,-11.5671105274575));
#284505=CARTESIAN_POINT('Ctrl Pts',(-8.86823884002247E-14,130.962499999487,
-12.7882828778556));
#284506=CARTESIAN_POINT('Ctrl Pts',(-3.75838203887402,131.112499999486,
-11.5671105274575));
#284507=CARTESIAN_POINT('Ctrl Pts',(-7.51676407774795,131.262499999485,
-10.3459381770593));
#284508=CARTESIAN_POINT('Ctrl Pts',(-9.83957192047916,131.412499999485,
-7.14886745759543));
#284509=CARTESIAN_POINT('Ctrl Pts',(-12.1623797632104,131.562499999484,
-3.95179673813153));
#284510=CARTESIAN_POINT('Ctrl Pts',(-12.1623797632104,131.712499999484,
2.97892388940601E-15));
#284511=CARTESIAN_POINT('Ctrl Pts',(-12.1623797632104,131.862499999483,
3.95179673813154));
#284512=CARTESIAN_POINT('Ctrl Pts',(-9.83957192047916,132.012499999482,
7.14886745759543));
#284513=CARTESIAN_POINT('Ctrl Pts',(-7.51676407774795,132.162499999482,
10.3459381770593));
#284514=CARTESIAN_POINT('Ctrl Pts',(-3.75838203887402,132.312499999481,
11.5671105274575));
#284515=CARTESIAN_POINT('Ctrl Pts',(-8.64140170974642E-14,132.462499999481,
12.7882828778556));
#284516=CARTESIAN_POINT('Ctrl Pts',(3.75838203887384,132.61249999948,11.5671105274575));
#284517=CARTESIAN_POINT('Ctrl Pts',(7.51676407774777,132.762499999479,10.3459381770593));
#284518=CARTESIAN_POINT('Ctrl Pts',(9.83957192047899,132.912499999479,7.14886745759543));
#284519=CARTESIAN_POINT('Ctrl Pts',(12.1623797632102,133.062499999478,3.95179673813153));
#284520=CARTESIAN_POINT('Ctrl Pts',(12.1623797632102,133.212499999478,-1.489461944703E-15));
#284521=CARTESIAN_POINT('Ctrl Pts',(12.1623797632102,133.362499999477,-3.95179673813154));
#284522=CARTESIAN_POINT('Ctrl Pts',(9.83957192047898,133.512499999476,-7.14886745759543));
#284523=CARTESIAN_POINT('Ctrl Pts',(7.51676407774777,133.662499999476,-10.3459381770593));
#284524=CARTESIAN_POINT('Ctrl Pts',(3.75838203887384,133.812499999475,-11.5671105274575));
#284525=CARTESIAN_POINT('Ctrl Pts',(-9.04100976718865E-14,133.962499999475,
-12.7882828778556));
#284526=CARTESIAN_POINT('Ctrl Pts',(-3.75838203887402,134.112499999474,
-11.5671105274575));
#284527=CARTESIAN_POINT('Ctrl Pts',(-7.51676407774795,134.262499999473,
-10.3459381770593));
#284528=CARTESIAN_POINT('Ctrl Pts',(-9.83957192047917,134.412499999473,
-7.14886745759543));
#284529=CARTESIAN_POINT('Ctrl Pts',(-12.1623797632104,134.562499999472,
-3.95179673813153));
#284530=CARTESIAN_POINT('Ctrl Pts',(-12.1623797632104,134.712499999472,
2.97892388940601E-15));
#284531=CARTESIAN_POINT('Ctrl Pts',(-12.1623797632104,134.862499999471,
3.95179673813154));
#284532=CARTESIAN_POINT('Ctrl Pts',(-9.83957192047916,135.01249999947,7.14886745759543));
#284533=CARTESIAN_POINT('Ctrl Pts',(-7.51676407774795,135.16249999947,10.3459381770593));
#284534=CARTESIAN_POINT('Ctrl Pts',(-3.75838203887402,135.312499999469,
11.5671105274575));
#284535=CARTESIAN_POINT('Ctrl Pts',(-8.8141726369126E-14,135.462499999469,
12.7882828778556));
#284536=CARTESIAN_POINT('Ctrl Pts',(3.75838203887384,135.612499999468,11.5671105274575));
#284537=CARTESIAN_POINT('Ctrl Pts',(7.51676407774777,135.762499999467,10.3459381770593));
#284538=CARTESIAN_POINT('Ctrl Pts',(9.83957192047898,135.912499999467,7.14886745759543));
#284539=CARTESIAN_POINT('Ctrl Pts',(12.1623797632102,136.062499999466,3.95179673813153));
#284540=CARTESIAN_POINT('Ctrl Pts',(12.1623797632102,136.212499999466,-1.489461944703E-15));
#284541=CARTESIAN_POINT('Ctrl Pts',(12.1623797632102,136.362499999465,-3.95179673813154));
#284542=CARTESIAN_POINT('Ctrl Pts',(9.83957192047898,136.512499999464,-7.14886745759543));
#284543=CARTESIAN_POINT('Ctrl Pts',(7.51676407774776,136.662499999464,-10.3459381770593));
#284544=CARTESIAN_POINT('Ctrl Pts',(3.75838203887384,136.812499999463,-11.5671105274575));
#284545=CARTESIAN_POINT('Ctrl Pts',(-9.21378069435483E-14,136.962499999463,
-12.7882828778556));
#284546=CARTESIAN_POINT('Ctrl Pts',(-3.75838203887402,137.112499999462,
-11.5671105274575));
#284547=CARTESIAN_POINT('Ctrl Pts',(-7.51676407774795,137.262499999461,
-10.3459381770593));
#284548=CARTESIAN_POINT('Ctrl Pts',(-9.83957192047917,137.412499999461,
-7.14886745759543));
#284549=CARTESIAN_POINT('Ctrl Pts',(-12.1623797632104,137.56249999946,-3.95179673813153));
#284550=CARTESIAN_POINT('Ctrl Pts',(-12.1623797632104,137.71249999946,2.97892388940601E-15));
#284551=CARTESIAN_POINT('Ctrl Pts',(-12.1623797632104,137.862499999459,
3.95179673813154));
#284552=CARTESIAN_POINT('Ctrl Pts',(-9.83957192047917,138.012499999458,
7.14886745759543));
#284553=CARTESIAN_POINT('Ctrl Pts',(-7.51676407774795,138.162499999458,
10.3459381770593));
#284554=CARTESIAN_POINT('Ctrl Pts',(-3.75838203887402,138.312499999457,
11.5671105274575));
#284555=CARTESIAN_POINT('Ctrl Pts',(-8.98694356407879E-14,138.462499999457,
12.7882828778556));
#284556=CARTESIAN_POINT('Ctrl Pts',(3.75838203887384,138.612499999456,11.5671105274575));
#284557=CARTESIAN_POINT('Ctrl Pts',(7.51676407774777,138.762499999455,10.3459381770593));
#284558=CARTESIAN_POINT('Ctrl Pts',(9.83957192047898,138.912499999455,7.14886745759543));
#284559=CARTESIAN_POINT('Ctrl Pts',(12.1623797632102,139.062499999454,3.95179673813153));
#284560=CARTESIAN_POINT('Ctrl Pts',(12.1623797632102,139.212499999454,-1.489461944703E-15));
#284561=CARTESIAN_POINT('Ctrl Pts',(12.1623797632102,139.362499999453,-3.95179673813154));
#284562=CARTESIAN_POINT('Ctrl Pts',(9.83957192047898,139.512499999452,-7.14886745759543));
#284563=CARTESIAN_POINT('Ctrl Pts',(7.51676407774776,139.662499999452,-10.3459381770593));
#284564=CARTESIAN_POINT('Ctrl Pts',(3.75838203887384,139.812499999451,-11.5671105274575));
#284565=CARTESIAN_POINT('Ctrl Pts',(-9.38655162152102E-14,139.962499999451,
-12.7882828778556));
#284566=CARTESIAN_POINT('Ctrl Pts',(-3.75838203887402,140.11249999945,-11.5671105274575));
#284567=CARTESIAN_POINT('Ctrl Pts',(-7.51676407774795,140.262499999449,
-10.3459381770593));
#284568=CARTESIAN_POINT('Ctrl Pts',(-9.83957192047917,140.412499999449,
-7.14886745759543));
#284569=CARTESIAN_POINT('Ctrl Pts',(-12.1623797632104,140.562499999448,
-3.95179673813153));
#284570=CARTESIAN_POINT('Ctrl Pts',(-12.1623797632104,140.712499999448,
2.97892388940601E-15));
#284571=CARTESIAN_POINT('Ctrl Pts',(-12.1623797632104,140.862499999447,
3.95179673813154));
#284572=CARTESIAN_POINT('Ctrl Pts',(-9.83957192047917,141.012499999446,
7.14886745759543));
#284573=CARTESIAN_POINT('Ctrl Pts',(-7.51676407774795,141.162499999446,
10.3459381770593));
#284574=CARTESIAN_POINT('Ctrl Pts',(-3.75838203887402,141.312499999445,
11.5671105274575));
#284575=CARTESIAN_POINT('Ctrl Pts',(-9.15971449124498E-14,141.462499999445,
12.7882828778556));
#284576=CARTESIAN_POINT('Ctrl Pts',(3.75838203887384,141.612499999444,11.5671105274575));
#284577=CARTESIAN_POINT('Ctrl Pts',(7.51676407774776,141.762499999443,10.3459381770593));
#284578=CARTESIAN_POINT('Ctrl Pts',(9.83957192047898,141.912499999443,7.14886745759543));
#284579=CARTESIAN_POINT('Ctrl Pts',(12.1623797632102,142.062499999442,3.95179673813153));
#284580=CARTESIAN_POINT('Ctrl Pts',(12.1623797632102,142.212499999442,-1.489461944703E-15));
#284581=CARTESIAN_POINT('Ctrl Pts',(12.1623797632102,142.362499999441,-3.95179673813154));
#284582=CARTESIAN_POINT('Ctrl Pts',(9.83957192047898,142.51249999944,-7.14886745759543));
#284583=CARTESIAN_POINT('Ctrl Pts',(7.51676407774776,142.66249999944,-10.3459381770593));
#284584=CARTESIAN_POINT('Ctrl Pts',(3.75838203887383,142.812499999439,-11.5671105274575));
#284585=CARTESIAN_POINT('Ctrl Pts',(-9.5593225486872E-14,142.962499999439,
-12.7882828778556));
#284586=CARTESIAN_POINT('Ctrl Pts',(-3.75838203887402,143.112499999438,
-11.5671105274575));
#284587=CARTESIAN_POINT('Ctrl Pts',(-7.51676407774795,143.262499999437,
-10.3459381770593));
#284588=CARTESIAN_POINT('Ctrl Pts',(-9.83957192047917,143.412499999437,
-7.14886745759543));
#284589=CARTESIAN_POINT('Ctrl Pts',(-12.1623797632104,143.562499999436,
-3.95179673813153));
#284590=CARTESIAN_POINT('Ctrl Pts',(-12.1623797632104,143.712499999436,
2.97892388940601E-15));
#284591=CARTESIAN_POINT('Ctrl Pts',(-12.1623797632104,143.862499999435,
3.95179673813154));
#284592=CARTESIAN_POINT('Ctrl Pts',(-9.83957192047917,144.012499999434,
7.14886745759543));
#284593=CARTESIAN_POINT('Ctrl Pts',(-7.51676407774795,144.162499999434,
10.3459381770593));
#284594=CARTESIAN_POINT('Ctrl Pts',(-3.75838203887402,144.312499999433,
11.5671105274575));
#284595=CARTESIAN_POINT('Ctrl Pts',(-9.33248541841116E-14,144.462499999433,
12.7882828778556));
#284596=CARTESIAN_POINT('Ctrl Pts',(3.75838203887384,144.612499999432,11.5671105274575));
#284597=CARTESIAN_POINT('Ctrl Pts',(7.51676407774776,144.762499999431,10.3459381770593));
#284598=CARTESIAN_POINT('Ctrl Pts',(9.83957192047898,144.912499999431,7.14886745759543));
#284599=CARTESIAN_POINT('Ctrl Pts',(12.1623797632102,145.06249999943,3.95179673813153));
#284600=CARTESIAN_POINT('Ctrl Pts',(12.1623797632102,145.21249999943,-1.489461944703E-15));
#284601=CARTESIAN_POINT('Ctrl Pts',(12.1623797632102,145.362499999429,-3.95179673813154));
#284602=CARTESIAN_POINT('Ctrl Pts',(9.83957192047898,145.512499999428,-7.14886745759543));
#284603=CARTESIAN_POINT('Ctrl Pts',(7.51676407774776,145.662499999428,-10.3459381770593));
#284604=CARTESIAN_POINT('Ctrl Pts',(3.75838203887383,145.812499999427,-11.5671105274575));
#284605=CARTESIAN_POINT('Ctrl Pts',(-9.73209347585338E-14,145.962499999427,
-12.7882828778556));
#284606=CARTESIAN_POINT('Ctrl Pts',(-3.75838203887403,146.112499999426,
-11.5671105274575));
#284607=CARTESIAN_POINT('Ctrl Pts',(-7.51676407774795,146.262499999425,
-10.3459381770593));
#284608=CARTESIAN_POINT('Ctrl Pts',(-9.83957192047917,146.412499999425,
-7.14886745759543));
#284609=CARTESIAN_POINT('Ctrl Pts',(-12.1623797632104,146.562499999424,
-3.95179673813153));
#284610=CARTESIAN_POINT('Ctrl Pts',(-12.1623797632104,146.712499999424,
2.97892388940601E-15));
#284611=CARTESIAN_POINT('Ctrl Pts',(-12.1623797632104,146.862499999423,
3.95179673813154));
#284612=CARTESIAN_POINT('Ctrl Pts',(-9.83957192047917,147.012499999422,
7.14886745759543));
#284613=CARTESIAN_POINT('Ctrl Pts',(-7.51676407774795,147.162499999422,
10.3459381770593));
#284614=CARTESIAN_POINT('Ctrl Pts',(-3.75838203887402,147.312499999421,
11.5671105274575));
#284615=CARTESIAN_POINT('Ctrl Pts',(-9.50525634557734E-14,147.462499999421,
12.7882828778556));
#284616=CARTESIAN_POINT('Ctrl Pts',(3.75838203887383,147.61249999942,11.5671105274575));
#284617=CARTESIAN_POINT('Ctrl Pts',(7.51676407774776,147.762499999419,10.3459381770593));
#284618=CARTESIAN_POINT('Ctrl Pts',(9.83957192047898,147.912499999419,7.14886745759543));
#284619=CARTESIAN_POINT('Ctrl Pts',(12.1623797632102,148.062499999418,3.95179673813153));
#284620=CARTESIAN_POINT('Ctrl Pts',(12.1623797632102,148.212499999418,-1.489461944703E-15));
#284621=CARTESIAN_POINT('Ctrl Pts',(12.1623797632102,148.362499999417,-3.95179673813154));
#284622=CARTESIAN_POINT('Ctrl Pts',(9.83957192047898,148.512499999416,-7.14886745759543));
#284623=CARTESIAN_POINT('Ctrl Pts',(7.51676407774776,148.662499999416,-10.3459381770593));
#284624=CARTESIAN_POINT('Ctrl Pts',(3.75838203887383,148.812499999415,-11.5671105274575));
#284625=CARTESIAN_POINT('Ctrl Pts',(-9.90486440301957E-14,148.962499999415,
-12.7882828778556));
#284626=CARTESIAN_POINT('Ctrl Pts',(-3.75838203887403,149.112499999414,
-11.5671105274575));
#284627=CARTESIAN_POINT('Ctrl Pts',(-7.51676407774795,149.262499999413,
-10.3459381770593));
#284628=CARTESIAN_POINT('Ctrl Pts',(-9.83957192047917,149.412499999413,
-7.14886745759543));
#284629=CARTESIAN_POINT('Ctrl Pts',(-12.1623797632104,149.562499999412,
-3.95179673813153));
#284630=CARTESIAN_POINT('Ctrl Pts',(-12.1623797632104,149.712499999412,
2.97892388940601E-15));
#284631=CARTESIAN_POINT('Ctrl Pts',(-12.1623797632104,149.862499999411,
3.95179673813154));
#284632=CARTESIAN_POINT('Ctrl Pts',(-9.83957192047917,150.01249999941,7.14886745759543));
#284633=CARTESIAN_POINT('Ctrl Pts',(-7.51676407774795,150.16249999941,10.3459381770593));
#284634=CARTESIAN_POINT('Ctrl Pts',(-3.75838203887403,150.312499999409,
11.5671105274575));
#284635=CARTESIAN_POINT('Ctrl Pts',(-9.67802727274353E-14,150.462499999409,
12.7882828778556));
#284636=CARTESIAN_POINT('Ctrl Pts',(3.75838203887383,150.612499999408,11.5671105274575));
#284637=CARTESIAN_POINT('Ctrl Pts',(7.51676407774776,150.762499999407,10.3459381770593));
#284638=CARTESIAN_POINT('Ctrl Pts',(9.83957192047898,150.912499999407,7.14886745759543));
#284639=CARTESIAN_POINT('Ctrl Pts',(12.1623797632102,151.062499999406,3.95179673813153));
#284640=CARTESIAN_POINT('Ctrl Pts',(12.1623797632102,151.212499999406,-1.489461944703E-15));
#284641=CARTESIAN_POINT('Ctrl Pts',(12.1623797632102,151.362499999405,-3.95179673813154));
#284642=CARTESIAN_POINT('Ctrl Pts',(9.83957192047897,151.512499999404,-7.14886745759543));
#284643=CARTESIAN_POINT('Ctrl Pts',(7.51676407774776,151.662499999404,-10.3459381770593));
#284644=CARTESIAN_POINT('Ctrl Pts',(3.75838203887383,151.812499999403,-11.5671105274575));
#284645=CARTESIAN_POINT('Ctrl Pts',(-1.00776353301858E-13,151.962499999403,
-12.7882828778556));
#284646=CARTESIAN_POINT('Ctrl Pts',(-3.75838203887403,152.112499999402,
-11.5671105274575));
#284647=CARTESIAN_POINT('Ctrl Pts',(-10.0514333556354,-2.06874452331816,
2.46189113716437E-15));
#284648=CARTESIAN_POINT('Ctrl Pts',(-10.0514333556354,-1.91874452331876,
3.26590867261837));
#284649=CARTESIAN_POINT('Ctrl Pts',(-8.13178040253628,-1.76874452331936,
5.90808429084315));
#284650=CARTESIAN_POINT('Ctrl Pts',(-6.21212744943711,-1.61874452331995,
8.55025990906793));
#284651=CARTESIAN_POINT('Ctrl Pts',(-3.10606372471856,-1.46874452332055,
9.55948119098353));
#284652=CARTESIAN_POINT('Ctrl Pts',(-9.77671522407829E-15,-1.31874452332115,
10.5687024728991));
#284653=CARTESIAN_POINT('Ctrl Pts',(3.10606372471854,-1.16874452332175,
9.55948119098353));
#284654=CARTESIAN_POINT('Ctrl Pts',(6.21212744943709,-1.01874452332235,
8.55025990906793));
#284655=CARTESIAN_POINT('Ctrl Pts',(8.13178040253625,-0.868744523322946,
5.90808429084315));
#284656=CARTESIAN_POINT('Ctrl Pts',(10.0514333556354,-0.718744523323545,
3.26590867261836));
#284657=CARTESIAN_POINT('Ctrl Pts',(10.0514333556354,-0.568744523324145,
-1.23094556858219E-15));
#284658=CARTESIAN_POINT('Ctrl Pts',(10.0514333556354,-0.418744523324745,
-3.26590867261837));
#284659=CARTESIAN_POINT('Ctrl Pts',(8.13178040253625,-0.268744523325346,
-5.90808429084315));
#284660=CARTESIAN_POINT('Ctrl Pts',(6.21212744943709,-0.118744523325947,
-8.55025990906793));
#284661=CARTESIAN_POINT('Ctrl Pts',(3.10606372471854,0.0312554766734513,
-9.55948119098353));
#284662=CARTESIAN_POINT('Ctrl Pts',(-1.32291553908245E-14,0.181255476672849,
-10.5687024728991));
#284663=CARTESIAN_POINT('Ctrl Pts',(-3.10606372471856,0.331255476672248,
-9.55948119098353));
#284664=CARTESIAN_POINT('Ctrl Pts',(-6.21212744943711,0.481255476671646,
-8.55025990906793));
#284665=CARTESIAN_POINT('Ctrl Pts',(-8.13178040253628,0.631255476671045,
-5.90808429084315));
#284666=CARTESIAN_POINT('Ctrl Pts',(-10.0514333556354,0.781255476670443,
-3.26590867261836));
#284667=CARTESIAN_POINT('Ctrl Pts',(-10.0514333556354,0.931255476669843,
2.46189113716437E-15));
#284668=CARTESIAN_POINT('Ctrl Pts',(-10.0514333556354,1.08125547666924,
3.26590867261837));
#284669=CARTESIAN_POINT('Ctrl Pts',(-8.13178040253628,1.23125547666864,
5.90808429084315));
#284670=CARTESIAN_POINT('Ctrl Pts',(-6.21212744943711,1.38125547666805,
8.55025990906793));
#284671=CARTESIAN_POINT('Ctrl Pts',(-3.10606372471856,1.53125547666745,
9.55948119098353));
#284672=CARTESIAN_POINT('Ctrl Pts',(-1.15044244957401E-14,1.68125547666685,
10.5687024728991));
#284673=CARTESIAN_POINT('Ctrl Pts',(3.10606372471854,1.83125547666625,9.55948119098353));
#284674=CARTESIAN_POINT('Ctrl Pts',(6.21212744943709,1.98125547666565,8.55025990906793));
#284675=CARTESIAN_POINT('Ctrl Pts',(8.13178040253625,2.13125547666505,5.90808429084315));
#284676=CARTESIAN_POINT('Ctrl Pts',(10.0514333556354,2.28125547666446,3.26590867261836));
#284677=CARTESIAN_POINT('Ctrl Pts',(10.0514333556354,2.43125547666386,-1.23094556858219E-15));
#284678=CARTESIAN_POINT('Ctrl Pts',(10.0514333556354,2.58125547666326,-3.26590867261837));
#284679=CARTESIAN_POINT('Ctrl Pts',(8.13178040253625,2.73125547666265,-5.90808429084315));
#284680=CARTESIAN_POINT('Ctrl Pts',(6.21212744943709,2.88125547666205,-8.55025990906793));
#284681=CARTESIAN_POINT('Ctrl Pts',(3.10606372471854,3.03125547666145,-9.55948119098353));
#284682=CARTESIAN_POINT('Ctrl Pts',(-1.49568646624864E-14,3.18125547666085,
-10.5687024728991));
#284683=CARTESIAN_POINT('Ctrl Pts',(-3.10606372471857,3.33125547666025,
-9.55948119098353));
#284684=CARTESIAN_POINT('Ctrl Pts',(-6.21212744943712,3.48125547665965,
-8.55025990906793));
#284685=CARTESIAN_POINT('Ctrl Pts',(-8.13178040253628,3.63125547665905,
-5.90808429084315));
#284686=CARTESIAN_POINT('Ctrl Pts',(-10.0514333556354,3.78125547665844,
-3.26590867261836));
#284687=CARTESIAN_POINT('Ctrl Pts',(-10.0514333556354,3.93125547665784,
2.46189113716437E-15));
#284688=CARTESIAN_POINT('Ctrl Pts',(-10.0514333556354,4.08125547665724,
3.26590867261837));
#284689=CARTESIAN_POINT('Ctrl Pts',(-8.13178040253628,4.23125547665664,
5.90808429084315));
#284690=CARTESIAN_POINT('Ctrl Pts',(-6.21212744943711,4.38125547665605,
8.55025990906793));
#284691=CARTESIAN_POINT('Ctrl Pts',(-3.10606372471856,4.53125547665545,
9.55948119098353));
#284692=CARTESIAN_POINT('Ctrl Pts',(-1.3232133767402E-14,4.68125547665485,
10.5687024728991));
#284693=CARTESIAN_POINT('Ctrl Pts',(3.10606372471854,4.83125547665425,9.55948119098353));
#284694=CARTESIAN_POINT('Ctrl Pts',(6.21212744943709,4.98125547665365,8.55025990906793));
#284695=CARTESIAN_POINT('Ctrl Pts',(8.13178040253625,5.13125547665306,5.90808429084315));
#284696=CARTESIAN_POINT('Ctrl Pts',(10.0514333556354,5.28125547665245,3.26590867261836));
#284697=CARTESIAN_POINT('Ctrl Pts',(10.0514333556354,5.43125547665185,-1.23094556858219E-15));
#284698=CARTESIAN_POINT('Ctrl Pts',(10.0514333556354,5.58125547665125,-3.26590867261837));
#284699=CARTESIAN_POINT('Ctrl Pts',(8.13178040253625,5.73125547665065,-5.90808429084315));
#284700=CARTESIAN_POINT('Ctrl Pts',(6.21212744943708,5.88125547665005,-8.55025990906793));
#284701=CARTESIAN_POINT('Ctrl Pts',(3.10606372471853,6.03125547664945,-9.55948119098353));
#284702=CARTESIAN_POINT('Ctrl Pts',(-1.66845739341482E-14,6.18125547664885,
-10.5687024728991));
#284703=CARTESIAN_POINT('Ctrl Pts',(-3.10606372471857,6.33125547664825,
-9.55948119098353));
#284704=CARTESIAN_POINT('Ctrl Pts',(-6.21212744943712,6.48125547664765,
-8.55025990906793));
#284705=CARTESIAN_POINT('Ctrl Pts',(-8.13178040253628,6.63125547664705,
-5.90808429084315));
#284706=CARTESIAN_POINT('Ctrl Pts',(-10.0514333556354,6.78125547664644,
-3.26590867261836));
#284707=CARTESIAN_POINT('Ctrl Pts',(-10.0514333556354,6.93125547664584,
2.46189113716437E-15));
#284708=CARTESIAN_POINT('Ctrl Pts',(-10.0514333556354,7.08125547664524,
3.26590867261837));
#284709=CARTESIAN_POINT('Ctrl Pts',(-8.13178040253628,7.23125547664465,
5.90808429084315));
#284710=CARTESIAN_POINT('Ctrl Pts',(-6.21212744943711,7.38125547664405,
8.55025990906793));
#284711=CARTESIAN_POINT('Ctrl Pts',(-3.10606372471857,7.53125547664345,
9.55948119098353));
#284712=CARTESIAN_POINT('Ctrl Pts',(-1.49598430390638E-14,7.68125547664285,
10.5687024728991));
#284713=CARTESIAN_POINT('Ctrl Pts',(3.10606372471854,7.83125547664225,9.55948119098353));
#284714=CARTESIAN_POINT('Ctrl Pts',(6.21212744943708,7.98125547664165,8.55025990906793));
#284715=CARTESIAN_POINT('Ctrl Pts',(8.13178040253625,8.13125547664105,5.90808429084315));
#284716=CARTESIAN_POINT('Ctrl Pts',(10.0514333556354,8.28125547664046,3.26590867261836));
#284717=CARTESIAN_POINT('Ctrl Pts',(10.0514333556354,8.43125547663985,-1.23094556858219E-15));
#284718=CARTESIAN_POINT('Ctrl Pts',(10.0514333556354,8.58125547663926,-3.26590867261837));
#284719=CARTESIAN_POINT('Ctrl Pts',(8.13178040253625,8.73125547663865,-5.90808429084315));
#284720=CARTESIAN_POINT('Ctrl Pts',(6.21212744943708,8.88125547663805,-8.55025990906793));
#284721=CARTESIAN_POINT('Ctrl Pts',(3.10606372471853,9.03125547663745,-9.55948119098353));
#284722=CARTESIAN_POINT('Ctrl Pts',(-1.84122832058101E-14,9.18125547663685,
-10.5687024728991));
#284723=CARTESIAN_POINT('Ctrl Pts',(-3.10606372471857,9.33125547663625,
-9.55948119098353));
#284724=CARTESIAN_POINT('Ctrl Pts',(-6.21212744943712,9.48125547663565,
-8.55025990906793));
#284725=CARTESIAN_POINT('Ctrl Pts',(-8.13178040253628,9.63125547663505,
-5.90808429084315));
#284726=CARTESIAN_POINT('Ctrl Pts',(-10.0514333556354,9.78125547663444,
-3.26590867261836));
#284727=CARTESIAN_POINT('Ctrl Pts',(-10.0514333556354,9.93125547663384,
2.46189113716437E-15));
#284728=CARTESIAN_POINT('Ctrl Pts',(-10.0514333556354,10.0812554766332,
3.26590867261837));
#284729=CARTESIAN_POINT('Ctrl Pts',(-8.13178040253628,10.2312554766326,
5.90808429084315));
#284730=CARTESIAN_POINT('Ctrl Pts',(-6.21212744943712,10.381255476632,8.55025990906793));
#284731=CARTESIAN_POINT('Ctrl Pts',(-3.10606372471857,10.5312554766314,
9.55948119098353));
#284732=CARTESIAN_POINT('Ctrl Pts',(-1.66875523107256E-14,10.6812554766309,
10.5687024728991));
#284733=CARTESIAN_POINT('Ctrl Pts',(3.10606372471853,10.8312554766303,9.55948119098353));
#284734=CARTESIAN_POINT('Ctrl Pts',(6.21212744943708,10.9812554766297,8.55025990906793));
#284735=CARTESIAN_POINT('Ctrl Pts',(8.13178040253625,11.1312554766291,5.90808429084315));
#284736=CARTESIAN_POINT('Ctrl Pts',(10.0514333556354,11.2812554766285,3.26590867261836));
#284737=CARTESIAN_POINT('Ctrl Pts',(10.0514333556354,11.4312554766279,-1.23094556858219E-15));
#284738=CARTESIAN_POINT('Ctrl Pts',(10.0514333556354,11.5812554766273,-3.26590867261837));
#284739=CARTESIAN_POINT('Ctrl Pts',(8.13178040253624,11.7312554766267,-5.90808429084315));
#284740=CARTESIAN_POINT('Ctrl Pts',(6.21212744943708,11.8812554766261,-8.55025990906793));
#284741=CARTESIAN_POINT('Ctrl Pts',(3.10606372471853,12.0312554766255,-9.55948119098353));
#284742=CARTESIAN_POINT('Ctrl Pts',(-2.01399924774719E-14,12.1812554766248,
-10.5687024728991));
#284743=CARTESIAN_POINT('Ctrl Pts',(-3.10606372471857,12.3312554766242,
-9.55948119098353));
#284744=CARTESIAN_POINT('Ctrl Pts',(-6.21212744943712,12.4812554766236,
-8.55025990906793));
#284745=CARTESIAN_POINT('Ctrl Pts',(-8.13178040253628,12.631255476623,-5.90808429084315));
#284746=CARTESIAN_POINT('Ctrl Pts',(-10.0514333556354,12.7812554766224,
-3.26590867261836));
#284747=CARTESIAN_POINT('Ctrl Pts',(-10.0514333556354,12.9312554766218,
2.46189113716437E-15));
#284748=CARTESIAN_POINT('Ctrl Pts',(-10.0514333556354,13.0812554766212,
3.26590867261837));
#284749=CARTESIAN_POINT('Ctrl Pts',(-8.13178040253628,13.2312554766206,
5.90808429084315));
#284750=CARTESIAN_POINT('Ctrl Pts',(-6.21212744943712,13.38125547662,8.55025990906793));
#284751=CARTESIAN_POINT('Ctrl Pts',(-3.10606372471857,13.5312554766194,
9.55948119098353));
#284752=CARTESIAN_POINT('Ctrl Pts',(-1.84152615823875E-14,13.6812554766188,
10.5687024728991));
#284753=CARTESIAN_POINT('Ctrl Pts',(3.10606372471853,13.8312554766182,9.55948119098353));
#284754=CARTESIAN_POINT('Ctrl Pts',(6.21212744943708,13.9812554766177,8.55025990906793));
#284755=CARTESIAN_POINT('Ctrl Pts',(8.13178040253624,14.1312554766171,5.90808429084315));
#284756=CARTESIAN_POINT('Ctrl Pts',(10.0514333556354,14.2812554766165,3.26590867261836));
#284757=CARTESIAN_POINT('Ctrl Pts',(10.0514333556354,14.4312554766159,-1.23094556858219E-15));
#284758=CARTESIAN_POINT('Ctrl Pts',(10.0514333556354,14.5812554766153,-3.26590867261837));
#284759=CARTESIAN_POINT('Ctrl Pts',(8.13178040253624,14.7312554766147,-5.90808429084315));
#284760=CARTESIAN_POINT('Ctrl Pts',(6.21212744943708,14.8812554766141,-8.55025990906793));
#284761=CARTESIAN_POINT('Ctrl Pts',(3.10606372471853,15.0312554766134,-9.55948119098353));
#284762=CARTESIAN_POINT('Ctrl Pts',(-2.18677017491337E-14,15.1812554766128,
-10.5687024728991));
#284763=CARTESIAN_POINT('Ctrl Pts',(-3.10606372471857,15.3312554766122,
-9.55948119098353));
#284764=CARTESIAN_POINT('Ctrl Pts',(-6.21212744943712,15.4812554766116,
-8.55025990906793));
#284765=CARTESIAN_POINT('Ctrl Pts',(-8.13178040253629,15.631255476611,-5.90808429084315));
#284766=CARTESIAN_POINT('Ctrl Pts',(-10.0514333556354,15.7812554766104,
-3.26590867261836));
#284767=CARTESIAN_POINT('Ctrl Pts',(-10.0514333556355,15.9312554766098,
2.46189113716437E-15));
#284768=CARTESIAN_POINT('Ctrl Pts',(-10.0514333556354,16.0812554766092,
3.26590867261837));
#284769=CARTESIAN_POINT('Ctrl Pts',(-8.13178040253629,16.2312554766086,
5.90808429084315));
#284770=CARTESIAN_POINT('Ctrl Pts',(-6.21212744943712,16.381255476608,8.55025990906793));
#284771=CARTESIAN_POINT('Ctrl Pts',(-3.10606372471857,16.5312554766074,
9.55948119098353));
#284772=CARTESIAN_POINT('Ctrl Pts',(-2.01429708540493E-14,16.6812554766069,
10.5687024728991));
#284773=CARTESIAN_POINT('Ctrl Pts',(3.10606372471853,16.8312554766063,9.55948119098353));
#284774=CARTESIAN_POINT('Ctrl Pts',(6.21212744943708,16.9812554766057,8.55025990906793));
#284775=CARTESIAN_POINT('Ctrl Pts',(8.13178040253624,17.1312554766051,5.90808429084315));
#284776=CARTESIAN_POINT('Ctrl Pts',(10.0514333556354,17.2812554766045,3.26590867261836));
#284777=CARTESIAN_POINT('Ctrl Pts',(10.0514333556354,17.4312554766039,-1.23094556858219E-15));
#284778=CARTESIAN_POINT('Ctrl Pts',(10.0514333556354,17.5812554766033,-3.26590867261837));
#284779=CARTESIAN_POINT('Ctrl Pts',(8.13178040253624,17.7312554766027,-5.90808429084315));
#284780=CARTESIAN_POINT('Ctrl Pts',(6.21212744943708,17.881255476602,-8.55025990906793));
#284781=CARTESIAN_POINT('Ctrl Pts',(3.10606372471853,18.0312554766015,-9.55948119098353));
#284782=CARTESIAN_POINT('Ctrl Pts',(-2.35954110207956E-14,18.1812554766008,
-10.5687024728991));
#284783=CARTESIAN_POINT('Ctrl Pts',(-3.10606372471857,18.3312554766002,
-9.55948119098353));
#284784=CARTESIAN_POINT('Ctrl Pts',(-6.21212744943713,18.4812554765996,
-8.55025990906793));
#284785=CARTESIAN_POINT('Ctrl Pts',(-8.13178040253629,18.631255476599,-5.90808429084315));
#284786=CARTESIAN_POINT('Ctrl Pts',(-10.0514333556354,18.7812554765984,
-3.26590867261836));
#284787=CARTESIAN_POINT('Ctrl Pts',(-10.0514333556355,18.9312554765978,
2.46189113716437E-15));
#284788=CARTESIAN_POINT('Ctrl Pts',(-10.0514333556354,19.0812554765972,
3.26590867261837));
#284789=CARTESIAN_POINT('Ctrl Pts',(-8.13178040253629,19.2312554765966,
5.90808429084315));
#284790=CARTESIAN_POINT('Ctrl Pts',(-6.21212744943712,19.381255476596,8.55025990906793));
#284791=CARTESIAN_POINT('Ctrl Pts',(-3.10606372471857,19.5312554765954,
9.55948119098353));
#284792=CARTESIAN_POINT('Ctrl Pts',(-2.18706801257112E-14,19.6812554765949,
10.5687024728991));
#284793=CARTESIAN_POINT('Ctrl Pts',(3.10606372471853,19.8312554765942,9.55948119098353));
#284794=CARTESIAN_POINT('Ctrl Pts',(6.21212744943708,19.9812554765937,8.55025990906793));
#284795=CARTESIAN_POINT('Ctrl Pts',(8.13178040253624,20.1312554765931,5.90808429084315));
#284796=CARTESIAN_POINT('Ctrl Pts',(10.0514333556354,20.2812554765925,3.26590867261836));
#284797=CARTESIAN_POINT('Ctrl Pts',(10.0514333556354,20.4312554765919,-1.23094556858219E-15));
#284798=CARTESIAN_POINT('Ctrl Pts',(10.0514333556354,20.5812554765913,-3.26590867261837));
#284799=CARTESIAN_POINT('Ctrl Pts',(8.13178040253624,20.7312554765907,-5.90808429084315));
#284800=CARTESIAN_POINT('Ctrl Pts',(6.21212744943708,20.88125547659,-8.55025990906793));
#284801=CARTESIAN_POINT('Ctrl Pts',(3.10606372471852,21.0312554765894,-9.55948119098353));
#284802=CARTESIAN_POINT('Ctrl Pts',(-2.53231202924574E-14,21.1812554765889,
-10.5687024728991));
#284803=CARTESIAN_POINT('Ctrl Pts',(-3.10606372471858,21.3312554765882,
-9.55948119098353));
#284804=CARTESIAN_POINT('Ctrl Pts',(-6.21212744943713,21.4812554765876,
-8.55025990906793));
#284805=CARTESIAN_POINT('Ctrl Pts',(-8.13178040253629,21.631255476587,-5.90808429084315));
#284806=CARTESIAN_POINT('Ctrl Pts',(-10.0514333556354,21.7812554765864,
-3.26590867261836));
#284807=CARTESIAN_POINT('Ctrl Pts',(-10.0514333556355,21.9312554765858,
2.46189113716437E-15));
#284808=CARTESIAN_POINT('Ctrl Pts',(-10.0514333556354,22.0812554765852,
3.26590867261837));
#284809=CARTESIAN_POINT('Ctrl Pts',(-8.13178040253629,22.2312554765846,
5.90808429084315));
#284810=CARTESIAN_POINT('Ctrl Pts',(-6.21212744943713,22.381255476584,8.55025990906793));
#284811=CARTESIAN_POINT('Ctrl Pts',(-3.10606372471857,22.5312554765834,
9.55948119098353));
#284812=CARTESIAN_POINT('Ctrl Pts',(-2.3598389397373E-14,22.6812554765828,
10.5687024728991));
#284813=CARTESIAN_POINT('Ctrl Pts',(3.10606372471853,22.8312554765822,9.55948119098353));
#284814=CARTESIAN_POINT('Ctrl Pts',(6.21212744943708,22.9812554765817,8.55025990906793));
#284815=CARTESIAN_POINT('Ctrl Pts',(8.13178040253624,23.1312554765811,5.90808429084315));
#284816=CARTESIAN_POINT('Ctrl Pts',(10.0514333556354,23.2812554765805,3.26590867261836));
#284817=CARTESIAN_POINT('Ctrl Pts',(10.0514333556354,23.4312554765799,-1.23094556858219E-15));
#284818=CARTESIAN_POINT('Ctrl Pts',(10.0514333556354,23.5812554765793,-3.26590867261837));
#284819=CARTESIAN_POINT('Ctrl Pts',(8.13178040253624,23.7312554765787,-5.90808429084315));
#284820=CARTESIAN_POINT('Ctrl Pts',(6.21212744943707,23.8812554765781,-8.55025990906793));
#284821=CARTESIAN_POINT('Ctrl Pts',(3.10606372471852,24.0312554765774,-9.55948119098353));
#284822=CARTESIAN_POINT('Ctrl Pts',(-2.70508295641193E-14,24.1812554765769,
-10.5687024728991));
#284823=CARTESIAN_POINT('Ctrl Pts',(-3.10606372471858,24.3312554765762,
-9.55948119098353));
#284824=CARTESIAN_POINT('Ctrl Pts',(-6.21212744943713,24.4812554765756,
-8.55025990906793));
#284825=CARTESIAN_POINT('Ctrl Pts',(-8.13178040253629,24.631255476575,-5.90808429084315));
#284826=CARTESIAN_POINT('Ctrl Pts',(-10.0514333556355,24.7812554765744,
-3.26590867261836));
#284827=CARTESIAN_POINT('Ctrl Pts',(-10.0514333556355,24.9312554765738,
2.46189113716437E-15));
#284828=CARTESIAN_POINT('Ctrl Pts',(-10.0514333556355,25.0812554765733,
3.26590867261837));
#284829=CARTESIAN_POINT('Ctrl Pts',(-8.13178040253629,25.2312554765726,
5.90808429084315));
#284830=CARTESIAN_POINT('Ctrl Pts',(-6.21212744943713,25.3812554765721,
8.55025990906793));
#284831=CARTESIAN_POINT('Ctrl Pts',(-3.10606372471858,25.5312554765715,
9.55948119098353));
#284832=CARTESIAN_POINT('Ctrl Pts',(-2.53260986690348E-14,25.6812554765709,
10.5687024728991));
#284833=CARTESIAN_POINT('Ctrl Pts',(3.10606372471852,25.8312554765702,9.55948119098353));
#284834=CARTESIAN_POINT('Ctrl Pts',(6.21212744943708,25.9812554765697,8.55025990906793));
#284835=CARTESIAN_POINT('Ctrl Pts',(8.13178040253624,26.1312554765691,5.90808429084315));
#284836=CARTESIAN_POINT('Ctrl Pts',(10.0514333556354,26.2812554765685,3.26590867261836));
#284837=CARTESIAN_POINT('Ctrl Pts',(10.0514333556354,26.4312554765679,-1.23094556858219E-15));
#284838=CARTESIAN_POINT('Ctrl Pts',(10.0514333556354,26.5812554765673,-3.26590867261837));
#284839=CARTESIAN_POINT('Ctrl Pts',(8.13178040253623,26.7312554765667,-5.90808429084315));
#284840=CARTESIAN_POINT('Ctrl Pts',(6.21212744943707,26.8812554765661,-8.55025990906793));
#284841=CARTESIAN_POINT('Ctrl Pts',(3.10606372471852,27.0312554765654,-9.55948119098353));
#284842=CARTESIAN_POINT('Ctrl Pts',(-2.87785388357811E-14,27.1812554765649,
-10.5687024728991));
#284843=CARTESIAN_POINT('Ctrl Pts',(-3.10606372471858,27.3312554765642,
-9.55948119098353));
#284844=CARTESIAN_POINT('Ctrl Pts',(-6.21212744943713,27.4812554765636,
-8.55025990906793));
#284845=CARTESIAN_POINT('Ctrl Pts',(-8.13178040253629,27.631255476563,-5.90808429084315));
#284846=CARTESIAN_POINT('Ctrl Pts',(-10.0514333556355,27.7812554765624,
-3.26590867261836));
#284847=CARTESIAN_POINT('Ctrl Pts',(-10.0514333556355,27.9312554765618,
2.46189113716437E-15));
#284848=CARTESIAN_POINT('Ctrl Pts',(-10.0514333556355,28.0812554765612,
3.26590867261837));
#284849=CARTESIAN_POINT('Ctrl Pts',(-8.13178040253629,28.2312554765606,
5.90808429084315));
#284850=CARTESIAN_POINT('Ctrl Pts',(-6.21212744943713,28.38125547656,8.55025990906793));
#284851=CARTESIAN_POINT('Ctrl Pts',(-3.10606372471858,28.5312554765595,
9.55948119098353));
#284852=CARTESIAN_POINT('Ctrl Pts',(-2.70538079406967E-14,28.6812554765589,
10.5687024728991));
#284853=CARTESIAN_POINT('Ctrl Pts',(3.10606372471852,28.8312554765583,9.55948119098353));
#284854=CARTESIAN_POINT('Ctrl Pts',(6.21212744943707,28.9812554765577,8.55025990906793));
#284855=CARTESIAN_POINT('Ctrl Pts',(8.13178040253623,29.1312554765571,5.90808429084315));
#284856=CARTESIAN_POINT('Ctrl Pts',(10.0514333556354,29.2812554765565,3.26590867261836));
#284857=CARTESIAN_POINT('Ctrl Pts',(10.0514333556354,29.4312554765559,-1.23094556858219E-15));
#284858=CARTESIAN_POINT('Ctrl Pts',(10.0514333556354,29.5812554765553,-3.26590867261837));
#284859=CARTESIAN_POINT('Ctrl Pts',(8.13178040253623,29.7312554765547,-5.90808429084315));
#284860=CARTESIAN_POINT('Ctrl Pts',(6.21212744943707,29.881255476554,-8.55025990906793));
#284861=CARTESIAN_POINT('Ctrl Pts',(3.10606372471852,30.0312554765534,-9.55948119098353));
#284862=CARTESIAN_POINT('Ctrl Pts',(-3.05062481074429E-14,30.1812554765528,
-10.5687024728991));
#284863=CARTESIAN_POINT('Ctrl Pts',(-3.10606372471858,30.3312554765522,
-9.55948119098353));
#284864=CARTESIAN_POINT('Ctrl Pts',(-6.21212744943713,30.4812554765516,
-8.55025990906793));
#284865=CARTESIAN_POINT('Ctrl Pts',(-8.13178040253629,30.631255476551,-5.90808429084315));
#284866=CARTESIAN_POINT('Ctrl Pts',(-10.0514333556355,30.7812554765504,
-3.26590867261836));
#284867=CARTESIAN_POINT('Ctrl Pts',(-10.0514333556355,30.9312554765498,
2.46189113716437E-15));
#284868=CARTESIAN_POINT('Ctrl Pts',(-10.0514333556355,31.0812554765492,
3.26590867261837));
#284869=CARTESIAN_POINT('Ctrl Pts',(-8.13178040253629,31.2312554765487,
5.90808429084315));
#284870=CARTESIAN_POINT('Ctrl Pts',(-6.21212744943713,31.381255476548,8.55025990906793));
#284871=CARTESIAN_POINT('Ctrl Pts',(-3.10606372471858,31.5312554765474,
9.55948119098353));
#284872=CARTESIAN_POINT('Ctrl Pts',(-2.87815172123585E-14,31.6812554765468,
10.5687024728991));
#284873=CARTESIAN_POINT('Ctrl Pts',(3.10606372471852,31.8312554765463,9.55948119098353));
#284874=CARTESIAN_POINT('Ctrl Pts',(6.21212744943707,31.9812554765457,8.55025990906793));
#284875=CARTESIAN_POINT('Ctrl Pts',(8.13178040253623,32.1312554765451,5.90808429084315));
#284876=CARTESIAN_POINT('Ctrl Pts',(10.0514333556354,32.2812554765445,3.26590867261836));
#284877=CARTESIAN_POINT('Ctrl Pts',(10.0514333556354,32.4312554765439,-1.23094556858219E-15));
#284878=CARTESIAN_POINT('Ctrl Pts',(10.0514333556354,32.5812554765433,-3.26590867261837));
#284879=CARTESIAN_POINT('Ctrl Pts',(8.13178040253623,32.7312554765427,-5.90808429084315));
#284880=CARTESIAN_POINT('Ctrl Pts',(6.21212744943707,32.881255476542,-8.55025990906793));
#284881=CARTESIAN_POINT('Ctrl Pts',(3.10606372471852,33.0312554765415,-9.55948119098353));
#284882=CARTESIAN_POINT('Ctrl Pts',(-3.22339573791048E-14,33.1812554765408,
-10.5687024728991));
#284883=CARTESIAN_POINT('Ctrl Pts',(-3.10606372471858,33.3312554765402,
-9.55948119098353));
#284884=CARTESIAN_POINT('Ctrl Pts',(-6.21212744943713,33.4812554765397,
-8.55025990906793));
#284885=CARTESIAN_POINT('Ctrl Pts',(-8.1317804025363,33.631255476539,-5.90808429084315));
#284886=CARTESIAN_POINT('Ctrl Pts',(-10.0514333556355,33.7812554765384,
-3.26590867261836));
#284887=CARTESIAN_POINT('Ctrl Pts',(-10.0514333556355,33.9312554765378,
2.46189113716437E-15));
#284888=CARTESIAN_POINT('Ctrl Pts',(-10.0514333556355,34.0812554765372,
3.26590867261837));
#284889=CARTESIAN_POINT('Ctrl Pts',(-8.1317804025363,34.2312554765366,5.90808429084315));
#284890=CARTESIAN_POINT('Ctrl Pts',(-6.21212744943713,34.381255476536,8.55025990906793));
#284891=CARTESIAN_POINT('Ctrl Pts',(-3.10606372471858,34.5312554765354,
9.55948119098353));
#284892=CARTESIAN_POINT('Ctrl Pts',(-3.05092264840204E-14,34.6812554765349,
10.5687024728991));
#284893=CARTESIAN_POINT('Ctrl Pts',(3.10606372471852,34.8312554765343,9.55948119098353));
#284894=CARTESIAN_POINT('Ctrl Pts',(6.21212744943707,34.9812554765337,8.55025990906793));
#284895=CARTESIAN_POINT('Ctrl Pts',(8.13178040253623,35.1312554765331,5.90808429084315));
#284896=CARTESIAN_POINT('Ctrl Pts',(10.0514333556354,35.2812554765325,3.26590867261836));
#284897=CARTESIAN_POINT('Ctrl Pts',(10.0514333556354,35.4312554765319,-1.23094556858219E-15));
#284898=CARTESIAN_POINT('Ctrl Pts',(10.0514333556354,35.5812554765313,-3.26590867261837));
#284899=CARTESIAN_POINT('Ctrl Pts',(8.13178040253623,35.7312554765307,-5.90808429084315));
#284900=CARTESIAN_POINT('Ctrl Pts',(6.21212744943707,35.8812554765301,-8.55025990906793));
#284901=CARTESIAN_POINT('Ctrl Pts',(3.10606372471852,36.0312554765295,-9.55948119098353));
#284902=CARTESIAN_POINT('Ctrl Pts',(-3.39616666507666E-14,36.1812554765289,
-10.5687024728991));
#284903=CARTESIAN_POINT('Ctrl Pts',(-3.10606372471859,36.3312554765282,
-9.55948119098353));
#284904=CARTESIAN_POINT('Ctrl Pts',(-6.21212744943714,36.4812554765277,
-8.55025990906793));
#284905=CARTESIAN_POINT('Ctrl Pts',(-8.1317804025363,36.631255476527,-5.90808429084315));
#284906=CARTESIAN_POINT('Ctrl Pts',(-10.0514333556355,36.7812554765265,
-3.26590867261836));
#284907=CARTESIAN_POINT('Ctrl Pts',(-10.0514333556355,36.9312554765258,
2.46189113716437E-15));
#284908=CARTESIAN_POINT('Ctrl Pts',(-10.0514333556355,37.0812554765252,
3.26590867261837));
#284909=CARTESIAN_POINT('Ctrl Pts',(-8.1317804025363,37.2312554765246,5.90808429084315));
#284910=CARTESIAN_POINT('Ctrl Pts',(-6.21212744943713,37.381255476524,8.55025990906793));
#284911=CARTESIAN_POINT('Ctrl Pts',(-3.10606372471858,37.5312554765234,
9.55948119098353));
#284912=CARTESIAN_POINT('Ctrl Pts',(-3.22369357556822E-14,37.6812554765228,
10.5687024728991));
#284913=CARTESIAN_POINT('Ctrl Pts',(3.10606372471852,37.8312554765223,9.55948119098353));
#284914=CARTESIAN_POINT('Ctrl Pts',(6.21212744943707,37.9812554765217,8.55025990906793));
#284915=CARTESIAN_POINT('Ctrl Pts',(8.13178040253623,38.1312554765211,5.90808429084315));
#284916=CARTESIAN_POINT('Ctrl Pts',(10.0514333556354,38.2812554765204,3.26590867261836));
#284917=CARTESIAN_POINT('Ctrl Pts',(10.0514333556354,38.4312554765199,-1.23094556858219E-15));
#284918=CARTESIAN_POINT('Ctrl Pts',(10.0514333556354,38.5812554765193,-3.26590867261837));
#284919=CARTESIAN_POINT('Ctrl Pts',(8.13178040253623,38.7312554765187,-5.90808429084315));
#284920=CARTESIAN_POINT('Ctrl Pts',(6.21212744943707,38.881255476518,-8.55025990906793));
#284921=CARTESIAN_POINT('Ctrl Pts',(3.10606372471851,39.0312554765174,-9.55948119098353));
#284922=CARTESIAN_POINT('Ctrl Pts',(-3.56893759224285E-14,39.1812554765169,
-10.5687024728991));
#284923=CARTESIAN_POINT('Ctrl Pts',(-3.10606372471859,39.3312554765162,
-9.55948119098353));
#284924=CARTESIAN_POINT('Ctrl Pts',(-6.21212744943714,39.4812554765156,
-8.55025990906793));
#284925=CARTESIAN_POINT('Ctrl Pts',(-8.1317804025363,39.631255476515,-5.90808429084315));
#284926=CARTESIAN_POINT('Ctrl Pts',(-10.0514333556355,39.7812554765145,
-3.26590867261836));
#284927=CARTESIAN_POINT('Ctrl Pts',(-10.0514333556355,39.9312554765138,
2.46189113716437E-15));
#284928=CARTESIAN_POINT('Ctrl Pts',(-10.0514333556355,40.0812554765132,
3.26590867261837));
#284929=CARTESIAN_POINT('Ctrl Pts',(-8.1317804025363,40.2312554765126,5.90808429084315));
#284930=CARTESIAN_POINT('Ctrl Pts',(-6.21212744943714,40.381255476512,8.55025990906793));
#284931=CARTESIAN_POINT('Ctrl Pts',(-3.10606372471859,40.5312554765114,
9.55948119098353));
#284932=CARTESIAN_POINT('Ctrl Pts',(-3.39646450273441E-14,40.6812554765108,
10.5687024728991));
#284933=CARTESIAN_POINT('Ctrl Pts',(3.10606372471852,40.8312554765103,9.55948119098353));
#284934=CARTESIAN_POINT('Ctrl Pts',(6.21212744943707,40.9812554765097,8.55025990906793));
#284935=CARTESIAN_POINT('Ctrl Pts',(8.13178040253623,41.1312554765091,5.90808429084315));
#284936=CARTESIAN_POINT('Ctrl Pts',(10.0514333556354,41.2812554765085,3.26590867261836));
#284937=CARTESIAN_POINT('Ctrl Pts',(10.0514333556354,41.4312554765079,-1.23094556858219E-15));
#284938=CARTESIAN_POINT('Ctrl Pts',(10.0514333556354,41.5812554765073,-3.26590867261837));
#284939=CARTESIAN_POINT('Ctrl Pts',(8.13178040253623,41.7312554765067,-5.90808429084315));
#284940=CARTESIAN_POINT('Ctrl Pts',(6.21212744943706,41.8812554765061,-8.55025990906793));
#284941=CARTESIAN_POINT('Ctrl Pts',(3.10606372471851,42.0312554765054,-9.55948119098353));
#284942=CARTESIAN_POINT('Ctrl Pts',(-3.74170851940903E-14,42.1812554765049,
-10.5687024728991));
#284943=CARTESIAN_POINT('Ctrl Pts',(-3.10606372471859,42.3312554765042,
-9.55948119098353));
#284944=CARTESIAN_POINT('Ctrl Pts',(-6.21212744943714,42.4812554765036,
-8.55025990906793));
#284945=CARTESIAN_POINT('Ctrl Pts',(-8.1317804025363,42.631255476503,-5.90808429084315));
#284946=CARTESIAN_POINT('Ctrl Pts',(-10.0514333556355,42.7812554765024,
-3.26590867261836));
#284947=CARTESIAN_POINT('Ctrl Pts',(-10.0514333556355,42.9312554765018,
2.46189113716437E-15));
#284948=CARTESIAN_POINT('Ctrl Pts',(-10.0514333556355,43.0812554765012,
3.26590867261837));
#284949=CARTESIAN_POINT('Ctrl Pts',(-8.1317804025363,43.2312554765006,5.90808429084315));
#284950=CARTESIAN_POINT('Ctrl Pts',(-6.21212744943714,43.3812554765001,
8.55025990906793));
#284951=CARTESIAN_POINT('Ctrl Pts',(-3.10606372471859,43.5312554764994,
9.55948119098353));
#284952=CARTESIAN_POINT('Ctrl Pts',(-3.56923542990059E-14,43.6812554764988,
10.5687024728991));
#284953=CARTESIAN_POINT('Ctrl Pts',(3.10606372471851,43.8312554764982,9.55948119098353));
#284954=CARTESIAN_POINT('Ctrl Pts',(6.21212744943706,43.9812554764976,8.55025990906793));
#284955=CARTESIAN_POINT('Ctrl Pts',(8.13178040253623,44.1312554764971,5.90808429084315));
#284956=CARTESIAN_POINT('Ctrl Pts',(10.0514333556354,44.2812554764965,3.26590867261836));
#284957=CARTESIAN_POINT('Ctrl Pts',(10.0514333556354,44.4312554764959,-1.23094556858219E-15));
#284958=CARTESIAN_POINT('Ctrl Pts',(10.0514333556354,44.5812554764953,-3.26590867261837));
#284959=CARTESIAN_POINT('Ctrl Pts',(8.13178040253622,44.7312554764947,-5.90808429084315));
#284960=CARTESIAN_POINT('Ctrl Pts',(6.21212744943706,44.881255476494,-8.55025990906793));
#284961=CARTESIAN_POINT('Ctrl Pts',(3.10606372471851,45.0312554764935,-9.55948119098353));
#284962=CARTESIAN_POINT('Ctrl Pts',(-3.91447944657521E-14,45.1812554764929,
-10.5687024728991));
#284963=CARTESIAN_POINT('Ctrl Pts',(-3.10606372471859,45.3312554764922,
-9.55948119098353));
#284964=CARTESIAN_POINT('Ctrl Pts',(-6.21212744943714,45.4812554764916,
-8.55025990906793));
#284965=CARTESIAN_POINT('Ctrl Pts',(-8.1317804025363,45.631255476491,-5.90808429084315));
#284966=CARTESIAN_POINT('Ctrl Pts',(-10.0514333556355,45.7812554764904,
-3.26590867261836));
#284967=CARTESIAN_POINT('Ctrl Pts',(-10.0514333556355,45.9312554764898,
2.46189113716437E-15));
#284968=CARTESIAN_POINT('Ctrl Pts',(-10.0514333556355,46.0812554764892,
3.26590867261837));
#284969=CARTESIAN_POINT('Ctrl Pts',(-8.1317804025363,46.2312554764886,5.90808429084315));
#284970=CARTESIAN_POINT('Ctrl Pts',(-6.21212744943714,46.381255476488,8.55025990906793));
#284971=CARTESIAN_POINT('Ctrl Pts',(-3.10606372471859,46.5312554764875,
9.55948119098353));
#284972=CARTESIAN_POINT('Ctrl Pts',(-3.74200635706677E-14,46.6812554764869,
10.5687024728991));
#284973=CARTESIAN_POINT('Ctrl Pts',(3.10606372471851,46.8312554764862,9.55948119098353));
#284974=CARTESIAN_POINT('Ctrl Pts',(6.21212744943706,46.9812554764857,8.55025990906793));
#284975=CARTESIAN_POINT('Ctrl Pts',(8.13178040253622,47.1312554764851,5.90808429084315));
#284976=CARTESIAN_POINT('Ctrl Pts',(10.0514333556354,47.2812554764845,3.26590867261836));
#284977=CARTESIAN_POINT('Ctrl Pts',(10.0514333556354,47.4312554764839,-1.23094556858219E-15));
#284978=CARTESIAN_POINT('Ctrl Pts',(10.0514333556354,47.5812554764833,-3.26590867261837));
#284979=CARTESIAN_POINT('Ctrl Pts',(8.13178040253622,47.7312554764826,-5.90808429084315));
#284980=CARTESIAN_POINT('Ctrl Pts',(6.21212744943706,47.8812554764821,-8.55025990906793));
#284981=CARTESIAN_POINT('Ctrl Pts',(3.10606372471851,48.0312554764814,-9.55948119098353));
#284982=CARTESIAN_POINT('Ctrl Pts',(-4.0872503737414E-14,48.1812554764809,
-10.5687024728991));
#284983=CARTESIAN_POINT('Ctrl Pts',(-3.10606372471859,48.3312554764803,
-9.55948119098353));
#284984=CARTESIAN_POINT('Ctrl Pts',(-6.21212744943714,48.4812554764797,
-8.55025990906793));
#284985=CARTESIAN_POINT('Ctrl Pts',(-8.13178040253631,48.631255476479,-5.90808429084315));
#284986=CARTESIAN_POINT('Ctrl Pts',(-10.0514333556355,48.7812554764784,
-3.26590867261836));
#284987=CARTESIAN_POINT('Ctrl Pts',(-10.0514333556355,48.9312554764778,
2.46189113716437E-15));
#284988=CARTESIAN_POINT('Ctrl Pts',(-10.0514333556355,49.0812554764772,
3.26590867261837));
#284989=CARTESIAN_POINT('Ctrl Pts',(-8.13178040253631,49.2312554764766,
5.90808429084315));
#284990=CARTESIAN_POINT('Ctrl Pts',(-6.21212744943714,49.381255476476,8.55025990906793));
#284991=CARTESIAN_POINT('Ctrl Pts',(-3.10606372471859,49.5312554764755,
9.55948119098353));
#284992=CARTESIAN_POINT('Ctrl Pts',(-3.91477728423295E-14,49.6812554764748,
10.5687024728991));
#284993=CARTESIAN_POINT('Ctrl Pts',(3.10606372471851,49.8312554764742,9.55948119098353));
#284994=CARTESIAN_POINT('Ctrl Pts',(6.21212744943706,49.9812554764736,8.55025990906793));
#284995=CARTESIAN_POINT('Ctrl Pts',(8.13178040253622,50.1312554764731,5.90808429084315));
#284996=CARTESIAN_POINT('Ctrl Pts',(10.0514333556354,50.2812554764725,3.26590867261836));
#284997=CARTESIAN_POINT('Ctrl Pts',(10.0514333556354,50.4312554764719,-1.23094556858219E-15));
#284998=CARTESIAN_POINT('Ctrl Pts',(10.0514333556354,50.5812554764713,-3.26590867261837));
#284999=CARTESIAN_POINT('Ctrl Pts',(8.13178040253622,50.7312554764707,-5.90808429084315));
#285000=CARTESIAN_POINT('Ctrl Pts',(6.21212744943706,50.88125547647,-8.55025990906793));
#285001=CARTESIAN_POINT('Ctrl Pts',(3.10606372471851,51.0312554764695,-9.55948119098353));
#285002=CARTESIAN_POINT('Ctrl Pts',(-4.26002130090758E-14,51.1812554764689,
-10.5687024728991));
#285003=CARTESIAN_POINT('Ctrl Pts',(-3.10606372471859,51.3312554764683,
-9.55948119098353));
#285004=CARTESIAN_POINT('Ctrl Pts',(-6.21212744943715,51.4812554764676,
-8.55025990906793));
#285005=CARTESIAN_POINT('Ctrl Pts',(-8.13178040253631,51.6312554764671,
-5.90808429084315));
#285006=CARTESIAN_POINT('Ctrl Pts',(-10.0514333556355,51.7812554764664,
-3.26590867261836));
#285007=CARTESIAN_POINT('Ctrl Pts',(-10.0514333556355,51.9312554764658,
2.46189113716437E-15));
#285008=CARTESIAN_POINT('Ctrl Pts',(-10.0514333556355,52.0812554764652,
3.26590867261837));
#285009=CARTESIAN_POINT('Ctrl Pts',(-8.13178040253631,52.2312554764646,
5.90808429084315));
#285010=CARTESIAN_POINT('Ctrl Pts',(-6.21212744943714,52.381255476464,8.55025990906793));
#285011=CARTESIAN_POINT('Ctrl Pts',(-3.10606372471859,52.5312554764634,
9.55948119098353));
#285012=CARTESIAN_POINT('Ctrl Pts',(-4.08754821139914E-14,52.6812554764629,
10.5687024728991));
#285013=CARTESIAN_POINT('Ctrl Pts',(3.10606372471851,52.8312554764622,9.55948119098353));
#285014=CARTESIAN_POINT('Ctrl Pts',(6.21212744943706,52.9812554764617,8.55025990906793));
#285015=CARTESIAN_POINT('Ctrl Pts',(8.13178040253622,53.1312554764611,5.90808429084315));
#285016=CARTESIAN_POINT('Ctrl Pts',(10.0514333556354,53.2812554764605,3.26590867261836));
#285017=CARTESIAN_POINT('Ctrl Pts',(10.0514333556354,53.4312554764599,-1.23094556858219E-15));
#285018=CARTESIAN_POINT('Ctrl Pts',(10.0514333556354,53.5812554764593,-3.26590867261837));
#285019=CARTESIAN_POINT('Ctrl Pts',(8.13178040253622,53.7312554764587,-5.90808429084315));
#285020=CARTESIAN_POINT('Ctrl Pts',(6.21212744943706,53.8812554764581,-8.55025990906793));
#285021=CARTESIAN_POINT('Ctrl Pts',(3.10606372471851,54.0312554764574,-9.55948119098353));
#285022=CARTESIAN_POINT('Ctrl Pts',(-4.43279222807376E-14,54.1812554764569,
-10.5687024728991));
#285023=CARTESIAN_POINT('Ctrl Pts',(-3.1060637247186,54.3312554764562,-9.55948119098353));
#285024=CARTESIAN_POINT('Ctrl Pts',(-6.21212744943715,54.4812554764556,
-8.55025990906793));
#285025=CARTESIAN_POINT('Ctrl Pts',(-8.13178040253631,54.631255476455,-5.90808429084315));
#285026=CARTESIAN_POINT('Ctrl Pts',(-10.0514333556355,54.7812554764544,
-3.26590867261836));
#285027=CARTESIAN_POINT('Ctrl Pts',(-10.0514333556355,54.9312554764538,
2.46189113716437E-15));
#285028=CARTESIAN_POINT('Ctrl Pts',(-10.0514333556355,55.0812554764532,
3.26590867261837));
#285029=CARTESIAN_POINT('Ctrl Pts',(-8.13178040253631,55.2312554764526,
5.90808429084315));
#285030=CARTESIAN_POINT('Ctrl Pts',(-6.21212744943715,55.381255476452,8.55025990906793));
#285031=CARTESIAN_POINT('Ctrl Pts',(-3.10606372471859,55.5312554764514,
9.55948119098353));
#285032=CARTESIAN_POINT('Ctrl Pts',(-4.26031913856532E-14,55.6812554764508,
10.5687024728991));
#285033=CARTESIAN_POINT('Ctrl Pts',(3.10606372471851,55.8312554764502,9.55948119098353));
#285034=CARTESIAN_POINT('Ctrl Pts',(6.21212744943706,55.9812554764496,8.55025990906793));
#285035=CARTESIAN_POINT('Ctrl Pts',(8.13178040253622,56.1312554764491,5.90808429084315));
#285036=CARTESIAN_POINT('Ctrl Pts',(10.0514333556354,56.2812554764485,3.26590867261836));
#285037=CARTESIAN_POINT('Ctrl Pts',(10.0514333556354,56.4312554764479,-1.23094556858219E-15));
#285038=CARTESIAN_POINT('Ctrl Pts',(10.0514333556354,56.5812554764473,-3.26590867261837));
#285039=CARTESIAN_POINT('Ctrl Pts',(8.13178040253622,56.7312554764467,-5.90808429084315));
#285040=CARTESIAN_POINT('Ctrl Pts',(6.21212744943706,56.881255476446,-8.55025990906793));
#285041=CARTESIAN_POINT('Ctrl Pts',(3.10606372471851,57.0312554764455,-9.55948119098353));
#285042=CARTESIAN_POINT('Ctrl Pts',(-4.60556315523995E-14,57.1812554764448,
-10.5687024728991));
#285043=CARTESIAN_POINT('Ctrl Pts',(-3.1060637247186,57.3312554764443,-9.55948119098353));
#285044=CARTESIAN_POINT('Ctrl Pts',(-6.21212744943715,57.4812554764436,
-8.55025990906793));
#285045=CARTESIAN_POINT('Ctrl Pts',(-8.13178040253631,57.631255476443,-5.90808429084315));
#285046=CARTESIAN_POINT('Ctrl Pts',(-10.0514333556355,57.7812554764424,
-3.26590867261836));
#285047=CARTESIAN_POINT('Ctrl Pts',(-10.0514333556355,57.9312554764418,
2.46189113716437E-15));
#285048=CARTESIAN_POINT('Ctrl Pts',(-10.0514333556355,58.0812554764412,
3.26590867261837));
#285049=CARTESIAN_POINT('Ctrl Pts',(-8.13178040253631,58.2312554764406,
5.90808429084315));
#285050=CARTESIAN_POINT('Ctrl Pts',(-6.21212744943715,58.38125547644,8.55025990906793));
#285051=CARTESIAN_POINT('Ctrl Pts',(-3.10606372471859,58.5312554764394,
9.55948119098353));
#285052=CARTESIAN_POINT('Ctrl Pts',(-4.43309006573151E-14,58.6812554764388,
10.5687024728991));
#285053=CARTESIAN_POINT('Ctrl Pts',(3.10606372471851,58.8312554764382,9.55948119098353));
#285054=CARTESIAN_POINT('Ctrl Pts',(6.21212744943706,58.9812554764377,8.55025990906793));
#285055=CARTESIAN_POINT('Ctrl Pts',(8.13178040253622,59.1312554764371,5.90808429084315));
#285056=CARTESIAN_POINT('Ctrl Pts',(10.0514333556354,59.2812554764365,3.26590867261836));
#285057=CARTESIAN_POINT('Ctrl Pts',(10.0514333556354,59.4312554764359,-1.23094556858219E-15));
#285058=CARTESIAN_POINT('Ctrl Pts',(10.0514333556354,59.5812554764353,-3.26590867261837));
#285059=CARTESIAN_POINT('Ctrl Pts',(8.13178040253622,59.7312554764347,-5.90808429084315));
#285060=CARTESIAN_POINT('Ctrl Pts',(6.21212744943706,59.8812554764341,-8.55025990906793));
#285061=CARTESIAN_POINT('Ctrl Pts',(3.1060637247185,60.0312554764335,-9.55948119098353));
#285062=CARTESIAN_POINT('Ctrl Pts',(-4.77833408240613E-14,60.1812554764329,
-10.5687024728991));
#285063=CARTESIAN_POINT('Ctrl Pts',(-3.1060637247186,60.3312554764322,-9.55948119098353));
#285064=CARTESIAN_POINT('Ctrl Pts',(-6.21212744943715,60.4812554764316,
-8.55025990906793));
#285065=CARTESIAN_POINT('Ctrl Pts',(-8.13178040253631,60.631255476431,-5.90808429084315));
#285066=CARTESIAN_POINT('Ctrl Pts',(-10.0514333556355,60.7812554764304,
-3.26590867261836));
#285067=CARTESIAN_POINT('Ctrl Pts',(-10.0514333556355,60.9312554764298,
2.46189113716437E-15));
#285068=CARTESIAN_POINT('Ctrl Pts',(-10.0514333556355,61.0812554764292,
3.26590867261837));
#285069=CARTESIAN_POINT('Ctrl Pts',(-8.13178040253631,61.2312554764286,
5.90808429084315));
#285070=CARTESIAN_POINT('Ctrl Pts',(-6.21212744943715,61.381255476428,8.55025990906793));
#285071=CARTESIAN_POINT('Ctrl Pts',(-3.1060637247186,61.5312554764274,9.55948119098353));
#285072=CARTESIAN_POINT('Ctrl Pts',(-4.60586099289769E-14,61.6812554764268,
10.5687024728991));
#285073=CARTESIAN_POINT('Ctrl Pts',(3.1060637247185,61.8312554764263,9.55948119098353));
#285074=CARTESIAN_POINT('Ctrl Pts',(6.21212744943706,61.9812554764256,8.55025990906793));
#285075=CARTESIAN_POINT('Ctrl Pts',(8.13178040253622,62.1312554764251,5.90808429084315));
#285076=CARTESIAN_POINT('Ctrl Pts',(10.0514333556354,62.2812554764245,3.26590867261836));
#285077=CARTESIAN_POINT('Ctrl Pts',(10.0514333556354,62.4312554764238,-1.23094556858219E-15));
#285078=CARTESIAN_POINT('Ctrl Pts',(10.0514333556354,62.5812554764233,-3.26590867261837));
#285079=CARTESIAN_POINT('Ctrl Pts',(8.13178040253621,62.7312554764227,-5.90808429084315));
#285080=CARTESIAN_POINT('Ctrl Pts',(6.21212744943705,62.8812554764221,-8.55025990906793));
#285081=CARTESIAN_POINT('Ctrl Pts',(3.1060637247185,63.0312554764215,-9.55948119098353));
#285082=CARTESIAN_POINT('Ctrl Pts',(-4.95110500957232E-14,63.1812554764208,
-10.5687024728991));
#285083=CARTESIAN_POINT('Ctrl Pts',(-3.1060637247186,63.3312554764203,-9.55948119098353));
#285084=CARTESIAN_POINT('Ctrl Pts',(-6.21212744943715,63.4812554764196,
-8.55025990906793));
#285085=CARTESIAN_POINT('Ctrl Pts',(-8.13178040253631,63.631255476419,-5.90808429084315));
#285086=CARTESIAN_POINT('Ctrl Pts',(-10.0514333556355,63.7812554764184,
-3.26590867261836));
#285087=CARTESIAN_POINT('Ctrl Pts',(-10.0514333556355,63.9312554764178,
2.46189113716437E-15));
#285088=CARTESIAN_POINT('Ctrl Pts',(-10.0514333556355,64.0812554764173,
3.26590867261837));
#285089=CARTESIAN_POINT('Ctrl Pts',(-8.13178040253631,64.2312554764166,
5.90808429084315));
#285090=CARTESIAN_POINT('Ctrl Pts',(-6.21212744943715,64.3812554764161,
8.55025990906793));
#285091=CARTESIAN_POINT('Ctrl Pts',(-3.1060637247186,64.5312554764155,9.55948119098353));
#285092=CARTESIAN_POINT('Ctrl Pts',(-4.77863192006388E-14,64.6812554764149,
10.5687024728991));
#285093=CARTESIAN_POINT('Ctrl Pts',(3.1060637247185,64.8312554764142,9.55948119098353));
#285094=CARTESIAN_POINT('Ctrl Pts',(6.21212744943705,64.9812554764137,8.55025990906793));
#285095=CARTESIAN_POINT('Ctrl Pts',(8.13178040253621,65.1312554764131,5.90808429084315));
#285096=CARTESIAN_POINT('Ctrl Pts',(10.0514333556354,65.2812554764124,3.26590867261836));
#285097=CARTESIAN_POINT('Ctrl Pts',(10.0514333556354,65.4312554764118,-1.23094556858219E-15));
#285098=CARTESIAN_POINT('Ctrl Pts',(10.0514333556354,65.5812554764112,-3.26590867261837));
#285099=CARTESIAN_POINT('Ctrl Pts',(8.13178040253621,65.7312554764107,-5.90808429084315));
#285100=CARTESIAN_POINT('Ctrl Pts',(6.21212744943705,65.8812554764101,-8.55025990906793));
#285101=CARTESIAN_POINT('Ctrl Pts',(3.1060637247185,66.0312554764095,-9.55948119098353));
#285102=CARTESIAN_POINT('Ctrl Pts',(-5.1238759367385E-14,66.1812554764089,
-10.5687024728991));
#285103=CARTESIAN_POINT('Ctrl Pts',(-3.1060637247186,66.3312554764082,-9.55948119098353));
#285104=CARTESIAN_POINT('Ctrl Pts',(-6.21212744943715,66.4812554764077,
-8.55025990906793));
#285105=CARTESIAN_POINT('Ctrl Pts',(-8.13178040253632,66.631255476407,-5.90808429084315));
#285106=CARTESIAN_POINT('Ctrl Pts',(-10.0514333556355,66.7812554764064,
-3.26590867261836));
#285107=CARTESIAN_POINT('Ctrl Pts',(-10.0514333556355,66.9312554764059,
2.46189113716437E-15));
#285108=CARTESIAN_POINT('Ctrl Pts',(-10.0514333556355,67.0812554764052,
3.26590867261837));
#285109=CARTESIAN_POINT('Ctrl Pts',(-8.13178040253632,67.2312554764047,
5.90808429084315));
#285110=CARTESIAN_POINT('Ctrl Pts',(-6.21212744943715,67.381255476404,8.55025990906793));
#285111=CARTESIAN_POINT('Ctrl Pts',(-3.1060637247186,67.5312554764035,9.55948119098353));
#285112=CARTESIAN_POINT('Ctrl Pts',(-4.95140284723006E-14,67.6812554764028,
10.5687024728991));
#285113=CARTESIAN_POINT('Ctrl Pts',(3.1060637247185,67.8312554764022,9.55948119098353));
#285114=CARTESIAN_POINT('Ctrl Pts',(6.21212744943705,67.9812554764016,8.55025990906793));
#285115=CARTESIAN_POINT('Ctrl Pts',(8.13178040253621,68.131255476401,5.90808429084315));
#285116=CARTESIAN_POINT('Ctrl Pts',(10.0514333556354,68.2812554764004,3.26590867261836));
#285117=CARTESIAN_POINT('Ctrl Pts',(10.0514333556354,68.4312554763998,-1.23094556858219E-15));
#285118=CARTESIAN_POINT('Ctrl Pts',(10.0514333556354,68.5812554763992,-3.26590867261837));
#285119=CARTESIAN_POINT('Ctrl Pts',(8.13178040253621,68.7312554763986,-5.90808429084315));
#285120=CARTESIAN_POINT('Ctrl Pts',(6.21212744943705,68.8812554763981,-8.55025990906793));
#285121=CARTESIAN_POINT('Ctrl Pts',(3.1060637247185,69.0312554763974,-9.55948119098353));
#285122=CARTESIAN_POINT('Ctrl Pts',(-5.29664686390469E-14,69.1812554763968,
-10.5687024728991));
#285123=CARTESIAN_POINT('Ctrl Pts',(-3.1060637247186,69.3312554763963,-9.55948119098353));
#285124=CARTESIAN_POINT('Ctrl Pts',(-6.21212744943715,69.4812554763957,
-8.55025990906793));
#285125=CARTESIAN_POINT('Ctrl Pts',(-8.13178040253632,69.6312554763951,
-5.90808429084315));
#285126=CARTESIAN_POINT('Ctrl Pts',(-10.0514333556355,69.7812554763944,
-3.26590867261836));
#285127=CARTESIAN_POINT('Ctrl Pts',(-10.0514333556355,69.9312554763938,
2.46189113716437E-15));
#285128=CARTESIAN_POINT('Ctrl Pts',(-10.0514333556355,70.0812554763932,
3.26590867261837));
#285129=CARTESIAN_POINT('Ctrl Pts',(-8.13178040253632,70.2312554763926,
5.90808429084315));
#285130=CARTESIAN_POINT('Ctrl Pts',(-6.21212744943715,70.381255476392,8.55025990906793));
#285131=CARTESIAN_POINT('Ctrl Pts',(-3.1060637247186,70.5312554763914,9.55948119098353));
#285132=CARTESIAN_POINT('Ctrl Pts',(-5.12417377439624E-14,70.6812554763908,
10.5687024728991));
#285133=CARTESIAN_POINT('Ctrl Pts',(3.1060637247185,70.8312554763903,9.55948119098353));
#285134=CARTESIAN_POINT('Ctrl Pts',(6.21212744943705,70.9812554763896,8.55025990906793));
#285135=CARTESIAN_POINT('Ctrl Pts',(8.13178040253621,71.131255476389,5.90808429084315));
#285136=CARTESIAN_POINT('Ctrl Pts',(10.0514333556354,71.2812554763884,3.26590867261836));
#285137=CARTESIAN_POINT('Ctrl Pts',(10.0514333556354,71.4312554763879,-1.23094556858219E-15));
#285138=CARTESIAN_POINT('Ctrl Pts',(10.0514333556354,71.5812554763872,-3.26590867261837));
#285139=CARTESIAN_POINT('Ctrl Pts',(8.13178040253621,71.7312554763867,-5.90808429084315));
#285140=CARTESIAN_POINT('Ctrl Pts',(6.21212744943705,71.881255476386,-8.55025990906793));
#285141=CARTESIAN_POINT('Ctrl Pts',(3.1060637247185,72.0312554763855,-9.55948119098353));
#285142=CARTESIAN_POINT('Ctrl Pts',(-5.46941779107087E-14,72.1812554763848,
-10.5687024728991));
#285143=CARTESIAN_POINT('Ctrl Pts',(-3.10606372471861,72.3312554763843,
-9.55948119098353));
#285144=CARTESIAN_POINT('Ctrl Pts',(-6.21212744943716,72.4812554763837,
-8.55025990906793));
#285145=CARTESIAN_POINT('Ctrl Pts',(-8.13178040253632,72.6312554763831,
-5.90808429084315));
#285146=CARTESIAN_POINT('Ctrl Pts',(-10.0514333556355,72.7812554763825,
-3.26590867261836));
#285147=CARTESIAN_POINT('Ctrl Pts',(-10.0514333556355,72.9312554763818,
2.46189113716437E-15));
#285148=CARTESIAN_POINT('Ctrl Pts',(-10.0514333556355,73.0812554763812,
3.26590867261837));
#285149=CARTESIAN_POINT('Ctrl Pts',(-8.13178040253632,73.2312554763807,
5.90808429084315));
#285150=CARTESIAN_POINT('Ctrl Pts',(-6.21212744943715,73.3812554763801,
8.55025990906793));
#285151=CARTESIAN_POINT('Ctrl Pts',(-3.1060637247186,73.5312554763795,9.55948119098353));
#285152=CARTESIAN_POINT('Ctrl Pts',(-5.29694470156243E-14,73.6812554763789,
10.5687024728991));
#285153=CARTESIAN_POINT('Ctrl Pts',(3.1060637247185,73.8312554763782,9.55948119098353));
#285154=CARTESIAN_POINT('Ctrl Pts',(6.21212744943705,73.9812554763777,8.55025990906793));
#285155=CARTESIAN_POINT('Ctrl Pts',(8.13178040253621,74.131255476377,5.90808429084315));
#285156=CARTESIAN_POINT('Ctrl Pts',(10.0514333556354,74.2812554763765,3.26590867261836));
#285157=CARTESIAN_POINT('Ctrl Pts',(10.0514333556354,74.4312554763758,-1.23094556858219E-15));
#285158=CARTESIAN_POINT('Ctrl Pts',(10.0514333556354,74.5812554763752,-3.26590867261837));
#285159=CARTESIAN_POINT('Ctrl Pts',(8.13178040253621,74.7312554763746,-5.90808429084315));
#285160=CARTESIAN_POINT('Ctrl Pts',(6.21212744943704,74.8812554763741,-8.55025990906793));
#285161=CARTESIAN_POINT('Ctrl Pts',(3.10606372471849,75.0312554763734,-9.55948119098353));
#285162=CARTESIAN_POINT('Ctrl Pts',(-5.64218871823705E-14,75.1812554763729,
-10.5687024728991));
#285163=CARTESIAN_POINT('Ctrl Pts',(-3.10606372471861,75.3312554763722,
-9.55948119098353));
#285164=CARTESIAN_POINT('Ctrl Pts',(-6.21212744943716,75.4812554763717,
-8.55025990906793));
#285165=CARTESIAN_POINT('Ctrl Pts',(-8.13178040253632,75.6312554763711,
-5.90808429084315));
#285166=CARTESIAN_POINT('Ctrl Pts',(-10.0514333556355,75.7812554763704,
-3.26590867261836));
#285167=CARTESIAN_POINT('Ctrl Pts',(-10.0514333556355,75.9312554763699,
2.46189113716437E-15));
#285168=CARTESIAN_POINT('Ctrl Pts',(-10.0514333556355,76.0812554763693,
3.26590867261837));
#285169=CARTESIAN_POINT('Ctrl Pts',(-8.13178040253632,76.2312554763686,
5.90808429084315));
#285170=CARTESIAN_POINT('Ctrl Pts',(-6.21212744943715,76.3812554763681,
8.55025990906793));
#285171=CARTESIAN_POINT('Ctrl Pts',(-3.1060637247186,76.5312554763674,9.55948119098353));
#285172=CARTESIAN_POINT('Ctrl Pts',(-5.46971562872861E-14,76.6812554763668,
10.5687024728991));
#285173=CARTESIAN_POINT('Ctrl Pts',(3.1060637247185,76.8312554763662,9.55948119098353));
#285174=CARTESIAN_POINT('Ctrl Pts',(6.21212744943705,76.9812554763656,8.55025990906793));
#285175=CARTESIAN_POINT('Ctrl Pts',(8.13178040253621,77.1312554763651,5.90808429084315));
#285176=CARTESIAN_POINT('Ctrl Pts',(10.0514333556354,77.2812554763644,3.26590867261836));
#285177=CARTESIAN_POINT('Ctrl Pts',(10.0514333556354,77.4312554763638,-1.23094556858219E-15));
#285178=CARTESIAN_POINT('Ctrl Pts',(10.0514333556354,77.5812554763632,-3.26590867261837));
#285179=CARTESIAN_POINT('Ctrl Pts',(8.13178040253621,77.7312554763626,-5.90808429084315));
#285180=CARTESIAN_POINT('Ctrl Pts',(6.21212744943704,77.881255476362,-8.55025990906793));
#285181=CARTESIAN_POINT('Ctrl Pts',(3.10606372471849,78.0312554763615,-9.55948119098353));
#285182=CARTESIAN_POINT('Ctrl Pts',(-5.81495964540324E-14,78.1812554763608,
-10.5687024728991));
#285183=CARTESIAN_POINT('Ctrl Pts',(-3.10606372471861,78.3312554763603,
-9.55948119098353));
#285184=CARTESIAN_POINT('Ctrl Pts',(-6.21212744943716,78.4812554763596,
-8.55025990906793));
#285185=CARTESIAN_POINT('Ctrl Pts',(-8.13178040253632,78.6312554763591,
-5.90808429084315));
#285186=CARTESIAN_POINT('Ctrl Pts',(-10.0514333556355,78.7812554763585,
-3.26590867261836));
#285187=CARTESIAN_POINT('Ctrl Pts',(-10.0514333556355,78.9312554763579,
2.46189113716437E-15));
#285188=CARTESIAN_POINT('Ctrl Pts',(-10.0514333556355,79.0812554763573,
3.26590867261837));
#285189=CARTESIAN_POINT('Ctrl Pts',(-8.13178040253632,79.2312554763567,
5.90808429084315));
#285190=CARTESIAN_POINT('Ctrl Pts',(-6.21212744943716,79.3812554763561,
8.55025990906793));
#285191=CARTESIAN_POINT('Ctrl Pts',(-3.10606372471861,79.5312554763554,
9.55948119098353));
#285192=CARTESIAN_POINT('Ctrl Pts',(-5.6424865558948E-14,79.6812554763548,
10.5687024728991));
#285193=CARTESIAN_POINT('Ctrl Pts',(3.10606372471849,79.8312554763542,9.55948119098353));
#285194=CARTESIAN_POINT('Ctrl Pts',(6.21212744943704,79.9812554763537,8.55025990906793));
#285195=CARTESIAN_POINT('Ctrl Pts',(8.1317804025362,80.131255476353,5.90808429084315));
#285196=CARTESIAN_POINT('Ctrl Pts',(10.0514333556354,80.2812554763524,3.26590867261836));
#285197=CARTESIAN_POINT('Ctrl Pts',(10.0514333556354,80.4312554763519,-1.23094556858219E-15));
#285198=CARTESIAN_POINT('Ctrl Pts',(10.0514333556354,80.5812554763513,-3.26590867261837));
#285199=CARTESIAN_POINT('Ctrl Pts',(8.1317804025362,80.7312554763506,-5.90808429084315));
#285200=CARTESIAN_POINT('Ctrl Pts',(6.21212744943704,80.88125547635,-8.55025990906793));
#285201=CARTESIAN_POINT('Ctrl Pts',(3.10606372471849,81.0312554763494,-9.55948119098353));
#285202=CARTESIAN_POINT('Ctrl Pts',(-5.98773057256942E-14,81.1812554763489,
-10.5687024728991));
#285203=CARTESIAN_POINT('Ctrl Pts',(-3.10606372471861,81.3312554763482,
-9.55948119098353));
#285204=CARTESIAN_POINT('Ctrl Pts',(-6.21212744943716,81.4812554763476,
-8.55025990906793));
#285205=CARTESIAN_POINT('Ctrl Pts',(-8.13178040253633,81.631255476347,-5.90808429084315));
#285206=CARTESIAN_POINT('Ctrl Pts',(-10.0514333556355,81.7812554763464,
-3.26590867261836));
#285207=CARTESIAN_POINT('Ctrl Pts',(-10.0514333556355,81.9312554763458,
2.46189113716437E-15));
#285208=CARTESIAN_POINT('Ctrl Pts',(-10.0514333556355,82.0812554763452,
3.26590867261837));
#285209=CARTESIAN_POINT('Ctrl Pts',(-8.13178040253633,82.2312554763447,
5.90808429084315));
#285210=CARTESIAN_POINT('Ctrl Pts',(-6.21212744943716,82.3812554763441,
8.55025990906793));
#285211=CARTESIAN_POINT('Ctrl Pts',(-3.10606372471861,82.5312554763435,
9.55948119098353));
#285212=CARTESIAN_POINT('Ctrl Pts',(-5.81525748306098E-14,82.6812554763429,
10.5687024728991));
#285213=CARTESIAN_POINT('Ctrl Pts',(3.10606372471849,82.8312554763423,9.55948119098353));
#285214=CARTESIAN_POINT('Ctrl Pts',(6.21212744943704,82.9812554763416,8.55025990906793));
#285215=CARTESIAN_POINT('Ctrl Pts',(8.1317804025362,83.1312554763411,5.90808429084315));
#285216=CARTESIAN_POINT('Ctrl Pts',(10.0514333556354,83.2812554763404,3.26590867261836));
#285217=CARTESIAN_POINT('Ctrl Pts',(10.0514333556354,83.4312554763399,-1.23094556858219E-15));
#285218=CARTESIAN_POINT('Ctrl Pts',(10.0514333556354,83.5812554763393,-3.26590867261837));
#285219=CARTESIAN_POINT('Ctrl Pts',(8.1317804025362,83.7312554763386,-5.90808429084315));
#285220=CARTESIAN_POINT('Ctrl Pts',(6.21212744943704,83.881255476338,-8.55025990906793));
#285221=CARTESIAN_POINT('Ctrl Pts',(3.10606372471849,84.0312554763374,-9.55948119098353));
#285222=CARTESIAN_POINT('Ctrl Pts',(-6.1605014997356E-14,84.1812554763369,
-10.5687024728991));
#285223=CARTESIAN_POINT('Ctrl Pts',(-3.10606372471861,84.3312554763362,
-9.55948119098353));
#285224=CARTESIAN_POINT('Ctrl Pts',(-6.21212744943716,84.4812554763356,
-8.55025990906793));
#285225=CARTESIAN_POINT('Ctrl Pts',(-8.13178040253633,84.631255476335,-5.90808429084315));
#285226=CARTESIAN_POINT('Ctrl Pts',(-10.0514333556355,84.7812554763345,
-3.26590867261836));
#285227=CARTESIAN_POINT('Ctrl Pts',(-10.0514333556355,84.9312554763338,
2.46189113716437E-15));
#285228=CARTESIAN_POINT('Ctrl Pts',(-10.0514333556355,85.0812554763333,
3.26590867261837));
#285229=CARTESIAN_POINT('Ctrl Pts',(-8.13178040253633,85.2312554763326,
5.90808429084315));
#285230=CARTESIAN_POINT('Ctrl Pts',(-6.21212744943716,85.3812554763321,
8.55025990906793));
#285231=CARTESIAN_POINT('Ctrl Pts',(-3.10606372471861,85.5312554763315,
9.55948119098353));
#285232=CARTESIAN_POINT('Ctrl Pts',(-5.98802841022716E-14,85.6812554763308,
10.5687024728991));
#285233=CARTESIAN_POINT('Ctrl Pts',(3.10606372471849,85.8312554763303,9.55948119098353));
#285234=CARTESIAN_POINT('Ctrl Pts',(6.21212744943704,85.9812554763297,8.55025990906793));
#285235=CARTESIAN_POINT('Ctrl Pts',(8.1317804025362,86.131255476329,5.90808429084315));
#285236=CARTESIAN_POINT('Ctrl Pts',(10.0514333556354,86.2812554763284,3.26590867261836));
#285237=CARTESIAN_POINT('Ctrl Pts',(10.0514333556354,86.4312554763278,-1.23094556858219E-15));
#285238=CARTESIAN_POINT('Ctrl Pts',(10.0514333556354,86.5812554763272,-3.26590867261837));
#285239=CARTESIAN_POINT('Ctrl Pts',(8.1317804025362,86.7312554763266,-5.90808429084315));
#285240=CARTESIAN_POINT('Ctrl Pts',(6.21212744943704,86.881255476326,-8.55025990906793));
#285241=CARTESIAN_POINT('Ctrl Pts',(3.10606372471849,87.0312554763254,-9.55948119098353));
#285242=CARTESIAN_POINT('Ctrl Pts',(-6.33327242690179E-14,87.1812554763249,
-10.5687024728991));
#285243=CARTESIAN_POINT('Ctrl Pts',(-3.10606372471861,87.3312554763242,
-9.55948119098353));
#285244=CARTESIAN_POINT('Ctrl Pts',(-6.21212744943717,87.4812554763236,
-8.55025990906793));
#285245=CARTESIAN_POINT('Ctrl Pts',(-8.13178040253633,87.631255476323,-5.90808429084315));
#285246=CARTESIAN_POINT('Ctrl Pts',(-10.0514333556355,87.7812554763225,
-3.26590867261836));
#285247=CARTESIAN_POINT('Ctrl Pts',(-10.0514333556355,87.9312554763218,
2.46189113716437E-15));
#285248=CARTESIAN_POINT('Ctrl Pts',(-10.0514333556355,88.0812554763212,
3.26590867261837));
#285249=CARTESIAN_POINT('Ctrl Pts',(-8.13178040253633,88.2312554763207,
5.90808429084315));
#285250=CARTESIAN_POINT('Ctrl Pts',(-6.21212744943716,88.38125547632,8.55025990906793));
#285251=CARTESIAN_POINT('Ctrl Pts',(-3.10606372471861,88.5312554763195,
9.55948119098353));
#285252=CARTESIAN_POINT('Ctrl Pts',(-6.16079933739335E-14,88.6812554763188,
10.5687024728991));
#285253=CARTESIAN_POINT('Ctrl Pts',(3.10606372471849,88.8312554763183,9.55948119098353));
#285254=CARTESIAN_POINT('Ctrl Pts',(6.21212744943704,88.9812554763177,8.55025990906793));
#285255=CARTESIAN_POINT('Ctrl Pts',(8.1317804025362,89.1312554763171,5.90808429084315));
#285256=CARTESIAN_POINT('Ctrl Pts',(10.0514333556354,89.2812554763164,3.26590867261836));
#285257=CARTESIAN_POINT('Ctrl Pts',(10.0514333556354,89.4312554763158,-1.23094556858219E-15));
#285258=CARTESIAN_POINT('Ctrl Pts',(10.0514333556354,89.5812554763153,-3.26590867261837));
#285259=CARTESIAN_POINT('Ctrl Pts',(8.1317804025362,89.7312554763146,-5.90808429084315));
#285260=CARTESIAN_POINT('Ctrl Pts',(6.21212744943704,89.881255476314,-8.55025990906793));
#285261=CARTESIAN_POINT('Ctrl Pts',(3.10606372471849,90.0312554763134,-9.55948119098353));
#285262=CARTESIAN_POINT('Ctrl Pts',(-6.50604335406797E-14,90.1812554763128,
-10.5687024728991));
#285263=CARTESIAN_POINT('Ctrl Pts',(-3.10606372471862,90.3312554763122,
-9.55948119098353));
#285264=CARTESIAN_POINT('Ctrl Pts',(-6.21212744943717,90.4812554763116,
-8.55025990906793));
#285265=CARTESIAN_POINT('Ctrl Pts',(-8.13178040253633,90.631255476311,-5.90808429084315));
#285266=CARTESIAN_POINT('Ctrl Pts',(-10.0514333556355,90.7812554763104,
-3.26590867261836));
#285267=CARTESIAN_POINT('Ctrl Pts',(-10.0514333556355,90.9312554763098,
2.46189113716437E-15));
#285268=CARTESIAN_POINT('Ctrl Pts',(-10.0514333556355,91.0812554763092,
3.26590867261837));
#285269=CARTESIAN_POINT('Ctrl Pts',(-8.13178040253633,91.2312554763086,
5.90808429084315));
#285270=CARTESIAN_POINT('Ctrl Pts',(-6.21212744943717,91.3812554763081,
8.55025990906793));
#285271=CARTESIAN_POINT('Ctrl Pts',(-3.10606372471861,91.5312554763075,
9.55948119098353));
#285272=CARTESIAN_POINT('Ctrl Pts',(-6.33357026455953E-14,91.6812554763069,
10.5687024728991));
#285273=CARTESIAN_POINT('Ctrl Pts',(3.10606372471849,91.8312554763063,9.55948119098353));
#285274=CARTESIAN_POINT('Ctrl Pts',(6.21212744943704,91.9812554763056,8.55025990906793));
#285275=CARTESIAN_POINT('Ctrl Pts',(8.1317804025362,92.1312554763051,5.90808429084315));
#285276=CARTESIAN_POINT('Ctrl Pts',(10.0514333556354,92.2812554763045,3.26590867261836));
#285277=CARTESIAN_POINT('Ctrl Pts',(10.0514333556354,92.4312554763039,-1.23094556858219E-15));
#285278=CARTESIAN_POINT('Ctrl Pts',(10.0514333556354,92.5812554763033,-3.26590867261837));
#285279=CARTESIAN_POINT('Ctrl Pts',(8.1317804025362,92.7312554763026,-5.90808429084315));
#285280=CARTESIAN_POINT('Ctrl Pts',(6.21212744943704,92.881255476302,-8.55025990906793));
#285281=CARTESIAN_POINT('Ctrl Pts',(3.10606372471848,93.0312554763014,-9.55948119098353));
#285282=CARTESIAN_POINT('Ctrl Pts',(-6.67881428123416E-14,93.1812554763008,
-10.5687024728991));
#285283=CARTESIAN_POINT('Ctrl Pts',(-3.10606372471862,93.3312554763002,
-9.55948119098353));
#285284=CARTESIAN_POINT('Ctrl Pts',(-6.21212744943717,93.4812554762996,
-8.55025990906793));
#285285=CARTESIAN_POINT('Ctrl Pts',(-8.13178040253633,93.631255476299,-5.90808429084315));
#285286=CARTESIAN_POINT('Ctrl Pts',(-10.0514333556355,93.7812554762984,
-3.26590867261836));
#285287=CARTESIAN_POINT('Ctrl Pts',(-10.0514333556355,93.9312554762978,
2.46189113716437E-15));
#285288=CARTESIAN_POINT('Ctrl Pts',(-10.0514333556355,94.0812554762972,
3.26590867261837));
#285289=CARTESIAN_POINT('Ctrl Pts',(-8.13178040253633,94.2312554762967,
5.90808429084315));
#285290=CARTESIAN_POINT('Ctrl Pts',(-6.21212744943717,94.3812554762961,
8.55025990906793));
#285291=CARTESIAN_POINT('Ctrl Pts',(-3.10606372471862,94.5312554762955,
9.55948119098353));
#285292=CARTESIAN_POINT('Ctrl Pts',(-6.50634119172571E-14,94.6812554762948,
10.5687024728991));
#285293=CARTESIAN_POINT('Ctrl Pts',(3.10606372471849,94.8312554762943,9.55948119098353));
#285294=CARTESIAN_POINT('Ctrl Pts',(6.21212744943704,94.9812554762937,8.55025990906793));
#285295=CARTESIAN_POINT('Ctrl Pts',(8.1317804025362,95.1312554762931,5.90808429084315));
#285296=CARTESIAN_POINT('Ctrl Pts',(10.0514333556354,95.2812554762924,3.26590867261836));
#285297=CARTESIAN_POINT('Ctrl Pts',(10.0514333556354,95.4312554762919,-1.23094556858219E-15));
#285298=CARTESIAN_POINT('Ctrl Pts',(10.0514333556354,95.5812554762912,-3.26590867261837));
#285299=CARTESIAN_POINT('Ctrl Pts',(8.1317804025362,95.7312554762906,-5.90808429084315));
#285300=CARTESIAN_POINT('Ctrl Pts',(6.21212744943703,95.88125547629,-8.55025990906793));
#285301=CARTESIAN_POINT('Ctrl Pts',(3.10606372471848,96.0312554762895,-9.55948119098353));
#285302=CARTESIAN_POINT('Ctrl Pts',(-6.85158520840034E-14,96.1812554762889,
-10.5687024728991));
#285303=CARTESIAN_POINT('Ctrl Pts',(-3.10606372471862,96.3312554762882,
-9.55948119098353));
#285304=CARTESIAN_POINT('Ctrl Pts',(-6.21212744943717,96.4812554762876,
-8.55025990906793));
#285305=CARTESIAN_POINT('Ctrl Pts',(-8.13178040253633,96.631255476287,-5.90808429084315));
#285306=CARTESIAN_POINT('Ctrl Pts',(-10.0514333556355,96.7812554762864,
-3.26590867261836));
#285307=CARTESIAN_POINT('Ctrl Pts',(-10.0514333556355,96.9312554762858,
2.46189113716437E-15));
#285308=CARTESIAN_POINT('Ctrl Pts',(-10.0514333556355,97.0812554762852,
3.26590867261837));
#285309=CARTESIAN_POINT('Ctrl Pts',(-8.13178040253633,97.2312554762846,
5.90808429084315));
#285310=CARTESIAN_POINT('Ctrl Pts',(-6.21212744943717,97.3812554762841,
8.55025990906793));
#285311=CARTESIAN_POINT('Ctrl Pts',(-3.10606372471862,97.5312554762834,
9.55948119098353));
#285312=CARTESIAN_POINT('Ctrl Pts',(-6.6791121188919E-14,97.6812554762828,
10.5687024728991));
#285313=CARTESIAN_POINT('Ctrl Pts',(3.10606372471848,97.8312554762823,9.55948119098353));
#285314=CARTESIAN_POINT('Ctrl Pts',(6.21212744943704,97.9812554762817,8.55025990906793));
#285315=CARTESIAN_POINT('Ctrl Pts',(8.13178040253619,98.1312554762811,5.90808429084315));
#285316=CARTESIAN_POINT('Ctrl Pts',(10.0514333556354,98.2812554762804,3.26590867261836));
#285317=CARTESIAN_POINT('Ctrl Pts',(10.0514333556354,98.4312554762799,-1.23094556858219E-15));
#285318=CARTESIAN_POINT('Ctrl Pts',(10.0514333556354,98.5812554762793,-3.26590867261837));
#285319=CARTESIAN_POINT('Ctrl Pts',(8.13178040253619,98.7312554762786,-5.90808429084315));
#285320=CARTESIAN_POINT('Ctrl Pts',(6.21212744943703,98.8812554762781,-8.55025990906793));
#285321=CARTESIAN_POINT('Ctrl Pts',(3.10606372471848,99.0312554762774,-9.55948119098353));
#285322=CARTESIAN_POINT('Ctrl Pts',(-7.02435613556652E-14,99.1812554762769,
-10.5687024728991));
#285323=CARTESIAN_POINT('Ctrl Pts',(-3.10606372471862,99.3312554762762,
-9.55948119098353));
#285324=CARTESIAN_POINT('Ctrl Pts',(-6.21212744943717,99.4812554762756,
-8.55025990906793));
#285325=CARTESIAN_POINT('Ctrl Pts',(-8.13178040253633,99.631255476275,-5.90808429084315));
#285326=CARTESIAN_POINT('Ctrl Pts',(-10.0514333556355,99.7812554762745,
-3.26590867261836));
#285327=CARTESIAN_POINT('Ctrl Pts',(-10.0514333556355,99.9312554762739,
2.46189113716437E-15));
#285328=CARTESIAN_POINT('Ctrl Pts',(-10.0514333556355,100.081255476273,
3.26590867261837));
#285329=CARTESIAN_POINT('Ctrl Pts',(-8.13178040253633,100.231255476273,
5.90808429084315));
#285330=CARTESIAN_POINT('Ctrl Pts',(-6.21212744943717,100.381255476272,
8.55025990906793));
#285331=CARTESIAN_POINT('Ctrl Pts',(-3.10606372471862,100.531255476271,
9.55948119098353));
#285332=CARTESIAN_POINT('Ctrl Pts',(-6.85188304605808E-14,100.681255476271,
10.5687024728991));
#285333=CARTESIAN_POINT('Ctrl Pts',(3.10606372471848,100.83125547627,9.55948119098353));
#285334=CARTESIAN_POINT('Ctrl Pts',(6.21212744943703,100.98125547627,8.55025990906793));
#285335=CARTESIAN_POINT('Ctrl Pts',(8.13178040253619,101.131255476269,5.90808429084315));
#285336=CARTESIAN_POINT('Ctrl Pts',(10.0514333556354,101.281255476268,3.26590867261836));
#285337=CARTESIAN_POINT('Ctrl Pts',(10.0514333556354,101.431255476268,-1.23094556858219E-15));
#285338=CARTESIAN_POINT('Ctrl Pts',(10.0514333556353,101.581255476267,-3.26590867261837));
#285339=CARTESIAN_POINT('Ctrl Pts',(8.13178040253619,101.731255476267,-5.90808429084315));
#285340=CARTESIAN_POINT('Ctrl Pts',(6.21212744943703,101.881255476266,-8.55025990906793));
#285341=CARTESIAN_POINT('Ctrl Pts',(3.10606372471848,102.031255476265,-9.55948119098353));
#285342=CARTESIAN_POINT('Ctrl Pts',(-7.19712706273271E-14,102.181255476265,
-10.5687024728991));
#285343=CARTESIAN_POINT('Ctrl Pts',(-3.10606372471862,102.331255476264,
-9.55948119098353));
#285344=CARTESIAN_POINT('Ctrl Pts',(-6.21212744943717,102.481255476264,
-8.55025990906793));
#285345=CARTESIAN_POINT('Ctrl Pts',(-8.13178040253634,102.631255476263,
-5.90808429084315));
#285346=CARTESIAN_POINT('Ctrl Pts',(-10.0514333556355,102.781255476262,
-3.26590867261836));
#285347=CARTESIAN_POINT('Ctrl Pts',(-10.0514333556355,102.931255476262,
2.46189113716437E-15));
#285348=CARTESIAN_POINT('Ctrl Pts',(-10.0514333556355,103.081255476261,
3.26590867261837));
#285349=CARTESIAN_POINT('Ctrl Pts',(-8.13178040253634,103.231255476261,
5.90808429084315));
#285350=CARTESIAN_POINT('Ctrl Pts',(-6.21212744943717,103.38125547626,8.55025990906793));
#285351=CARTESIAN_POINT('Ctrl Pts',(-3.10606372471862,103.531255476259,
9.55948119098353));
#285352=CARTESIAN_POINT('Ctrl Pts',(-7.02465397322427E-14,103.681255476259,
10.5687024728991));
#285353=CARTESIAN_POINT('Ctrl Pts',(3.10606372471848,103.831255476258,9.55948119098353));
#285354=CARTESIAN_POINT('Ctrl Pts',(6.21212744943703,103.981255476258,8.55025990906793));
#285355=CARTESIAN_POINT('Ctrl Pts',(8.13178040253619,104.131255476257,5.90808429084315));
#285356=CARTESIAN_POINT('Ctrl Pts',(10.0514333556353,104.281255476256,3.26590867261836));
#285357=CARTESIAN_POINT('Ctrl Pts',(10.0514333556354,104.431255476256,-1.23094556858219E-15));
#285358=CARTESIAN_POINT('Ctrl Pts',(10.0514333556353,104.581255476255,-3.26590867261837));
#285359=CARTESIAN_POINT('Ctrl Pts',(8.13178040253619,104.731255476255,-5.90808429084315));
#285360=CARTESIAN_POINT('Ctrl Pts',(6.21212744943703,104.881255476254,-8.55025990906793));
#285361=CARTESIAN_POINT('Ctrl Pts',(3.10606372471848,105.031255476253,-9.55948119098353));
#285362=CARTESIAN_POINT('Ctrl Pts',(-7.36989798989889E-14,105.181255476253,
-10.5687024728991));
#285363=CARTESIAN_POINT('Ctrl Pts',(-3.10606372471862,105.331255476252,
-9.55948119098353));
#285364=CARTESIAN_POINT('Ctrl Pts',(-6.21212744943718,105.481255476252,
-8.55025990906793));
#285365=CARTESIAN_POINT('Ctrl Pts',(-8.13178040253634,105.631255476251,
-5.90808429084315));
#285366=CARTESIAN_POINT('Ctrl Pts',(-10.0514333556355,105.78125547625,-3.26590867261836));
#285367=CARTESIAN_POINT('Ctrl Pts',(-10.0514333556355,105.93125547625,2.46189113716437E-15));
#285368=CARTESIAN_POINT('Ctrl Pts',(-10.0514333556355,106.081255476249,
3.26590867261837));
#285369=CARTESIAN_POINT('Ctrl Pts',(-8.13178040253634,106.231255476249,
5.90808429084315));
#285370=CARTESIAN_POINT('Ctrl Pts',(-6.21212744943717,106.381255476248,
8.55025990906793));
#285371=CARTESIAN_POINT('Ctrl Pts',(-3.10606372471862,106.531255476247,
9.55948119098353));
#285372=CARTESIAN_POINT('Ctrl Pts',(-7.19742490039045E-14,106.681255476247,
10.5687024728991));
#285373=CARTESIAN_POINT('Ctrl Pts',(3.10606372471848,106.831255476246,9.55948119098353));
#285374=CARTESIAN_POINT('Ctrl Pts',(6.21212744943703,106.981255476246,8.55025990906793));
#285375=CARTESIAN_POINT('Ctrl Pts',(8.13178040253619,107.131255476245,5.90808429084315));
#285376=CARTESIAN_POINT('Ctrl Pts',(10.0514333556353,107.281255476244,3.26590867261836));
#285377=CARTESIAN_POINT('Ctrl Pts',(10.0514333556354,107.431255476244,-1.23094556858219E-15));
#285378=CARTESIAN_POINT('Ctrl Pts',(10.0514333556353,107.581255476243,-3.26590867261837));
#285379=CARTESIAN_POINT('Ctrl Pts',(8.13178040253619,107.731255476243,-5.90808429084315));
#285380=CARTESIAN_POINT('Ctrl Pts',(6.21212744943703,107.881255476242,-8.55025990906793));
#285381=CARTESIAN_POINT('Ctrl Pts',(3.10606372471848,108.031255476241,-9.55948119098353));
#285382=CARTESIAN_POINT('Ctrl Pts',(-7.54266891706507E-14,108.181255476241,
-10.5687024728991));
#285383=CARTESIAN_POINT('Ctrl Pts',(-3.10606372471863,108.33125547624,-9.55948119098353));
#285384=CARTESIAN_POINT('Ctrl Pts',(-6.21212744943718,108.48125547624,-8.55025990906793));
#285385=CARTESIAN_POINT('Ctrl Pts',(-8.13178040253634,108.631255476239,
-5.90808429084315));
#285386=CARTESIAN_POINT('Ctrl Pts',(-10.0514333556355,108.781255476238,
-3.26590867261836));
#285387=CARTESIAN_POINT('Ctrl Pts',(-10.0514333556355,108.931255476238,
2.46189113716437E-15));
#285388=CARTESIAN_POINT('Ctrl Pts',(-10.0514333556355,109.081255476237,
3.26590867261837));
#285389=CARTESIAN_POINT('Ctrl Pts',(-8.13178040253634,109.231255476237,
5.90808429084315));
#285390=CARTESIAN_POINT('Ctrl Pts',(-6.21212744943718,109.381255476236,
8.55025990906793));
#285391=CARTESIAN_POINT('Ctrl Pts',(-3.10606372471862,109.531255476235,
9.55948119098353));
#285392=CARTESIAN_POINT('Ctrl Pts',(-7.37019582755663E-14,109.681255476235,
10.5687024728991));
#285393=CARTESIAN_POINT('Ctrl Pts',(3.10606372471848,109.831255476234,9.55948119098353));
#285394=CARTESIAN_POINT('Ctrl Pts',(6.21212744943703,109.981255476234,8.55025990906793));
#285395=CARTESIAN_POINT('Ctrl Pts',(8.13178040253619,110.131255476233,5.90808429084315));
#285396=CARTESIAN_POINT('Ctrl Pts',(10.0514333556353,110.281255476232,3.26590867261836));
#285397=CARTESIAN_POINT('Ctrl Pts',(10.0514333556353,110.431255476232,-1.23094556858219E-15));
#285398=CARTESIAN_POINT('Ctrl Pts',(10.0514333556353,110.581255476231,-3.26590867261837));
#285399=CARTESIAN_POINT('Ctrl Pts',(8.13178040253619,110.731255476231,-5.90808429084315));
#285400=CARTESIAN_POINT('Ctrl Pts',(6.21212744943703,110.88125547623,-8.55025990906793));
#285401=CARTESIAN_POINT('Ctrl Pts',(3.10606372471847,111.031255476229,-9.55948119098353));
#285402=CARTESIAN_POINT('Ctrl Pts',(-7.71543984423126E-14,111.181255476229,
-10.5687024728991));
#285403=CARTESIAN_POINT('Ctrl Pts',(-3.10606372471863,111.331255476228,
-9.55948119098353));
#285404=CARTESIAN_POINT('Ctrl Pts',(-6.21212744943718,111.481255476228,
-8.55025990906793));
#285405=CARTESIAN_POINT('Ctrl Pts',(-8.13178040253634,111.631255476227,
-5.90808429084315));
#285406=CARTESIAN_POINT('Ctrl Pts',(-10.0514333556355,111.781255476226,
-3.26590867261836));
#285407=CARTESIAN_POINT('Ctrl Pts',(-10.0514333556355,111.931255476226,
2.46189113716437E-15));
#285408=CARTESIAN_POINT('Ctrl Pts',(-10.0514333556355,112.081255476225,
3.26590867261837));
#285409=CARTESIAN_POINT('Ctrl Pts',(-8.13178040253634,112.231255476225,
5.90808429084315));
#285410=CARTESIAN_POINT('Ctrl Pts',(-6.21212744943718,112.381255476224,
8.55025990906793));
#285411=CARTESIAN_POINT('Ctrl Pts',(-3.10606372471863,112.531255476223,
9.55948119098353));
#285412=CARTESIAN_POINT('Ctrl Pts',(-7.54296675472282E-14,112.681255476223,
10.5687024728991));
#285413=CARTESIAN_POINT('Ctrl Pts',(3.10606372471847,112.831255476222,9.55948119098353));
#285414=CARTESIAN_POINT('Ctrl Pts',(6.21212744943703,112.981255476222,8.55025990906793));
#285415=CARTESIAN_POINT('Ctrl Pts',(8.13178040253618,113.131255476221,5.90808429084315));
#285416=CARTESIAN_POINT('Ctrl Pts',(10.0514333556353,113.28125547622,3.26590867261836));
#285417=CARTESIAN_POINT('Ctrl Pts',(10.0514333556353,113.43125547622,-1.23094556858219E-15));
#285418=CARTESIAN_POINT('Ctrl Pts',(10.0514333556353,113.581255476219,-3.26590867261837));
#285419=CARTESIAN_POINT('Ctrl Pts',(8.13178040253618,113.731255476219,-5.90808429084315));
#285420=CARTESIAN_POINT('Ctrl Pts',(6.21212744943702,113.881255476218,-8.55025990906793));
#285421=CARTESIAN_POINT('Ctrl Pts',(3.10606372471847,114.031255476217,-9.55948119098353));
#285422=CARTESIAN_POINT('Ctrl Pts',(-7.88821077139744E-14,114.181255476217,
-10.5687024728991));
#285423=CARTESIAN_POINT('Ctrl Pts',(-3.10606372471863,114.331255476216,
-9.55948119098353));
#285424=CARTESIAN_POINT('Ctrl Pts',(-6.21212744943718,114.481255476216,
-8.55025990906793));
#285425=CARTESIAN_POINT('Ctrl Pts',(-8.13178040253634,114.631255476215,
-5.90808429084315));
#285426=CARTESIAN_POINT('Ctrl Pts',(-10.0514333556355,114.781255476214,
-3.26590867261836));
#285427=CARTESIAN_POINT('Ctrl Pts',(-10.0514333556355,114.931255476214,
2.46189113716437E-15));
#285428=CARTESIAN_POINT('Ctrl Pts',(-10.0514333556355,115.081255476213,
3.26590867261837));
#285429=CARTESIAN_POINT('Ctrl Pts',(-8.13178040253634,115.231255476213,
5.90808429084315));
#285430=CARTESIAN_POINT('Ctrl Pts',(-6.21212744943718,115.381255476212,
8.55025990906793));
#285431=CARTESIAN_POINT('Ctrl Pts',(-3.10606372471863,115.531255476211,
9.55948119098353));
#285432=CARTESIAN_POINT('Ctrl Pts',(-7.715737681889E-14,115.681255476211,
10.5687024728991));
#285433=CARTESIAN_POINT('Ctrl Pts',(3.10606372471847,115.83125547621,9.55948119098353));
#285434=CARTESIAN_POINT('Ctrl Pts',(6.21212744943703,115.98125547621,8.55025990906793));
#285435=CARTESIAN_POINT('Ctrl Pts',(8.13178040253618,116.131255476209,5.90808429084315));
#285436=CARTESIAN_POINT('Ctrl Pts',(10.0514333556353,116.281255476208,3.26590867261836));
#285437=CARTESIAN_POINT('Ctrl Pts',(10.0514333556353,116.431255476208,-1.23094556858219E-15));
#285438=CARTESIAN_POINT('Ctrl Pts',(10.0514333556353,116.581255476207,-3.26590867261837));
#285439=CARTESIAN_POINT('Ctrl Pts',(8.13178040253618,116.731255476207,-5.90808429084315));
#285440=CARTESIAN_POINT('Ctrl Pts',(6.21212744943702,116.881255476206,-8.55025990906793));
#285441=CARTESIAN_POINT('Ctrl Pts',(3.10606372471847,117.031255476205,-9.55948119098353));
#285442=CARTESIAN_POINT('Ctrl Pts',(-8.06098169856363E-14,117.181255476205,
-10.5687024728991));
#285443=CARTESIAN_POINT('Ctrl Pts',(-3.10606372471863,117.331255476204,
-9.55948119098353));
#285444=CARTESIAN_POINT('Ctrl Pts',(-6.21212744943718,117.481255476204,
-8.55025990906793));
#285445=CARTESIAN_POINT('Ctrl Pts',(-8.13178040253634,117.631255476203,
-5.90808429084315));
#285446=CARTESIAN_POINT('Ctrl Pts',(-10.0514333556355,117.781255476202,
-3.26590867261836));
#285447=CARTESIAN_POINT('Ctrl Pts',(-10.0514333556355,117.931255476202,
2.46189113716437E-15));
#285448=CARTESIAN_POINT('Ctrl Pts',(-10.0514333556355,118.081255476201,
3.26590867261837));
#285449=CARTESIAN_POINT('Ctrl Pts',(-8.13178040253634,118.231255476201,
5.90808429084315));
#285450=CARTESIAN_POINT('Ctrl Pts',(-6.21212744943718,118.3812554762,8.55025990906793));
#285451=CARTESIAN_POINT('Ctrl Pts',(-3.10606372471863,118.531255476199,
9.55948119098353));
#285452=CARTESIAN_POINT('Ctrl Pts',(-7.88850860905518E-14,118.681255476199,
10.5687024728991));
#285453=CARTESIAN_POINT('Ctrl Pts',(3.10606372471847,118.831255476198,9.55948119098353));
#285454=CARTESIAN_POINT('Ctrl Pts',(6.21212744943702,118.981255476198,8.55025990906793));
#285455=CARTESIAN_POINT('Ctrl Pts',(8.13178040253618,119.131255476197,5.90808429084315));
#285456=CARTESIAN_POINT('Ctrl Pts',(10.0514333556353,119.281255476196,3.26590867261836));
#285457=CARTESIAN_POINT('Ctrl Pts',(10.0514333556353,119.431255476196,-1.23094556858219E-15));
#285458=CARTESIAN_POINT('Ctrl Pts',(10.0514333556353,119.581255476195,-3.26590867261837));
#285459=CARTESIAN_POINT('Ctrl Pts',(8.13178040253618,119.731255476195,-5.90808429084315));
#285460=CARTESIAN_POINT('Ctrl Pts',(6.21212744943702,119.881255476194,-8.55025990906793));
#285461=CARTESIAN_POINT('Ctrl Pts',(3.10606372471847,120.031255476193,-9.55948119098353));
#285462=CARTESIAN_POINT('Ctrl Pts',(-8.23375262572981E-14,120.181255476193,
-10.5687024728991));
#285463=CARTESIAN_POINT('Ctrl Pts',(-3.10606372471863,120.331255476192,
-9.55948119098353));
#285464=CARTESIAN_POINT('Ctrl Pts',(-6.21212744943718,120.481255476192,
-8.55025990906793));
#285465=CARTESIAN_POINT('Ctrl Pts',(-8.13178040253635,120.631255476191,
-5.90808429084315));
#285466=CARTESIAN_POINT('Ctrl Pts',(-10.0514333556355,120.78125547619,-3.26590867261836));
#285467=CARTESIAN_POINT('Ctrl Pts',(-10.0514333556355,120.93125547619,2.46189113716437E-15));
#285468=CARTESIAN_POINT('Ctrl Pts',(-10.0514333556355,121.081255476189,
3.26590867261837));
#285469=CARTESIAN_POINT('Ctrl Pts',(-8.13178040253635,121.231255476189,
5.90808429084315));
#285470=CARTESIAN_POINT('Ctrl Pts',(-6.21212744943718,121.381255476188,
8.55025990906793));
#285471=CARTESIAN_POINT('Ctrl Pts',(-3.10606372471863,121.531255476187,
9.55948119098353));
#285472=CARTESIAN_POINT('Ctrl Pts',(-8.06127953622137E-14,121.681255476187,
10.5687024728991));
#285473=CARTESIAN_POINT('Ctrl Pts',(3.10606372471847,121.831255476186,9.55948119098353));
#285474=CARTESIAN_POINT('Ctrl Pts',(6.21212744943702,121.981255476186,8.55025990906793));
#285475=CARTESIAN_POINT('Ctrl Pts',(8.13178040253618,122.131255476185,5.90808429084315));
#285476=CARTESIAN_POINT('Ctrl Pts',(10.0514333556353,122.281255476184,3.26590867261836));
#285477=CARTESIAN_POINT('Ctrl Pts',(10.0514333556353,122.431255476184,-1.23094556858219E-15));
#285478=CARTESIAN_POINT('Ctrl Pts',(10.0514333556353,122.581255476183,-3.26590867261837));
#285479=CARTESIAN_POINT('Ctrl Pts',(8.13178040253618,122.731255476183,-5.90808429084315));
#285480=CARTESIAN_POINT('Ctrl Pts',(6.21212744943702,122.881255476182,-8.55025990906793));
#285481=CARTESIAN_POINT('Ctrl Pts',(3.10606372471847,123.031255476181,-9.55948119098353));
#285482=CARTESIAN_POINT('Ctrl Pts',(-8.40652355289599E-14,123.181255476181,
-10.5687024728991));
#285483=CARTESIAN_POINT('Ctrl Pts',(-3.10606372471864,123.33125547618,-9.55948119098353));
#285484=CARTESIAN_POINT('Ctrl Pts',(-6.21212744943718,123.48125547618,-8.55025990906793));
#285485=CARTESIAN_POINT('Ctrl Pts',(-8.13178040253635,123.631255476179,
-5.90808429084315));
#285486=CARTESIAN_POINT('Ctrl Pts',(-10.0514333556355,123.781255476178,
-3.26590867261836));
#285487=CARTESIAN_POINT('Ctrl Pts',(-10.0514333556355,123.931255476178,
2.46189113716437E-15));
#285488=CARTESIAN_POINT('Ctrl Pts',(-10.0514333556355,124.081255476177,
3.26590867261837));
#285489=CARTESIAN_POINT('Ctrl Pts',(-8.13178040253635,124.231255476177,
5.90808429084315));
#285490=CARTESIAN_POINT('Ctrl Pts',(-6.21212744943718,124.381255476176,
8.55025990906793));
#285491=CARTESIAN_POINT('Ctrl Pts',(-3.10606372471863,124.531255476175,
9.55948119098353));
#285492=CARTESIAN_POINT('Ctrl Pts',(-8.23405046338756E-14,124.681255476175,
10.5687024728991));
#285493=CARTESIAN_POINT('Ctrl Pts',(3.10606372471847,124.831255476174,9.55948119098353));
#285494=CARTESIAN_POINT('Ctrl Pts',(6.21212744943702,124.981255476174,8.55025990906793));
#285495=CARTESIAN_POINT('Ctrl Pts',(8.13178040253618,125.131255476173,5.90808429084315));
#285496=CARTESIAN_POINT('Ctrl Pts',(10.0514333556353,125.281255476172,3.26590867261836));
#285497=CARTESIAN_POINT('Ctrl Pts',(10.0514333556353,125.431255476172,-1.23094556858219E-15));
#285498=CARTESIAN_POINT('Ctrl Pts',(10.0514333556353,125.581255476171,-3.26590867261837));
#285499=CARTESIAN_POINT('Ctrl Pts',(8.13178040253618,125.731255476171,-5.90808429084315));
#285500=CARTESIAN_POINT('Ctrl Pts',(6.21212744943702,125.88125547617,-8.55025990906793));
#285501=CARTESIAN_POINT('Ctrl Pts',(3.10606372471847,126.031255476169,-9.55948119098353));
#285502=CARTESIAN_POINT('Ctrl Pts',(-8.57929448006218E-14,126.181255476169,
-10.5687024728991));
#285503=CARTESIAN_POINT('Ctrl Pts',(-3.10606372471864,126.331255476168,
-9.55948119098353));
#285504=CARTESIAN_POINT('Ctrl Pts',(-6.21212744943719,126.481255476168,
-8.55025990906793));
#285505=CARTESIAN_POINT('Ctrl Pts',(-8.13178040253635,126.631255476167,
-5.90808429084315));
#285506=CARTESIAN_POINT('Ctrl Pts',(-10.0514333556355,126.781255476166,
-3.26590867261836));
#285507=CARTESIAN_POINT('Ctrl Pts',(-10.0514333556355,126.931255476166,
2.46189113716437E-15));
#285508=CARTESIAN_POINT('Ctrl Pts',(-10.0514333556355,127.081255476165,
3.26590867261837));
#285509=CARTESIAN_POINT('Ctrl Pts',(-8.13178040253635,127.231255476165,
5.90808429084315));
#285510=CARTESIAN_POINT('Ctrl Pts',(-6.21212744943718,127.381255476164,
8.55025990906793));
#285511=CARTESIAN_POINT('Ctrl Pts',(-3.10606372471863,127.531255476163,
9.55948119098353));
#285512=CARTESIAN_POINT('Ctrl Pts',(-8.40682139055374E-14,127.681255476163,
10.5687024728991));
#285513=CARTESIAN_POINT('Ctrl Pts',(3.10606372471847,127.831255476162,9.55948119098353));
#285514=CARTESIAN_POINT('Ctrl Pts',(6.21212744943702,127.981255476162,8.55025990906793));
#285515=CARTESIAN_POINT('Ctrl Pts',(8.13178040253618,128.131255476161,5.90808429084315));
#285516=CARTESIAN_POINT('Ctrl Pts',(10.0514333556353,128.28125547616,3.26590867261836));
#285517=CARTESIAN_POINT('Ctrl Pts',(10.0514333556353,128.43125547616,-1.23094556858219E-15));
#285518=CARTESIAN_POINT('Ctrl Pts',(10.0514333556353,128.581255476159,-3.26590867261837));
#285519=CARTESIAN_POINT('Ctrl Pts',(8.13178040253618,128.731255476159,-5.90808429084315));
#285520=CARTESIAN_POINT('Ctrl Pts',(6.21212744943701,128.881255476158,-8.55025990906793));
#285521=CARTESIAN_POINT('Ctrl Pts',(3.10606372471846,129.031255476157,-9.55948119098353));
#285522=CARTESIAN_POINT('Ctrl Pts',(-8.75206540722836E-14,129.181255476157,
-10.5687024728991));
#285523=CARTESIAN_POINT('Ctrl Pts',(-3.10606372471864,129.331255476156,
-9.55948119098353));
#285524=CARTESIAN_POINT('Ctrl Pts',(-6.21212744943719,129.481255476156,
-8.55025990906793));
#285525=CARTESIAN_POINT('Ctrl Pts',(-8.13178040253635,129.631255476155,
-5.90808429084315));
#285526=CARTESIAN_POINT('Ctrl Pts',(-10.0514333556355,129.781255476154,
-3.26590867261836));
#285527=CARTESIAN_POINT('Ctrl Pts',(-10.0514333556355,129.931255476154,
2.46189113716437E-15));
#285528=CARTESIAN_POINT('Ctrl Pts',(-10.0514333556355,130.081255476153,
3.26590867261837));
#285529=CARTESIAN_POINT('Ctrl Pts',(-8.13178040253635,130.231255476153,
5.90808429084315));
#285530=CARTESIAN_POINT('Ctrl Pts',(-6.21212744943719,130.381255476152,
8.55025990906793));
#285531=CARTESIAN_POINT('Ctrl Pts',(-3.10606372471864,130.531255476151,
9.55948119098353));
#285532=CARTESIAN_POINT('Ctrl Pts',(-8.57959231771992E-14,130.681255476151,
10.5687024728991));
#285533=CARTESIAN_POINT('Ctrl Pts',(3.10606372471846,130.83125547615,9.55948119098353));
#285534=CARTESIAN_POINT('Ctrl Pts',(6.21212744943702,130.98125547615,8.55025990906793));
#285535=CARTESIAN_POINT('Ctrl Pts',(8.13178040253618,131.131255476149,5.90808429084315));
#285536=CARTESIAN_POINT('Ctrl Pts',(10.0514333556353,131.281255476148,3.26590867261836));
#285537=CARTESIAN_POINT('Ctrl Pts',(10.0514333556353,131.431255476148,-1.23094556858219E-15));
#285538=CARTESIAN_POINT('Ctrl Pts',(10.0514333556353,131.581255476147,-3.26590867261837));
#285539=CARTESIAN_POINT('Ctrl Pts',(8.13178040253618,131.731255476147,-5.90808429084315));
#285540=CARTESIAN_POINT('Ctrl Pts',(6.21212744943701,131.881255476146,-8.55025990906793));
#285541=CARTESIAN_POINT('Ctrl Pts',(3.10606372471846,132.031255476145,-9.55948119098353));
#285542=CARTESIAN_POINT('Ctrl Pts',(-8.92483633439455E-14,132.181255476145,
-10.5687024728991));
#285543=CARTESIAN_POINT('Ctrl Pts',(-3.10606372471864,132.331255476144,
-9.55948119098353));
#285544=CARTESIAN_POINT('Ctrl Pts',(-6.21212744943719,132.481255476144,
-8.55025990906793));
#285545=CARTESIAN_POINT('Ctrl Pts',(-8.13178040253635,132.631255476143,
-5.90808429084315));
#285546=CARTESIAN_POINT('Ctrl Pts',(-10.0514333556355,132.781255476142,
-3.26590867261836));
#285547=CARTESIAN_POINT('Ctrl Pts',(-10.0514333556355,132.931255476142,
2.46189113716437E-15));
#285548=CARTESIAN_POINT('Ctrl Pts',(-10.0514333556355,133.081255476141,
3.26590867261837));
#285549=CARTESIAN_POINT('Ctrl Pts',(-8.13178040253635,133.231255476141,
5.90808429084315));
#285550=CARTESIAN_POINT('Ctrl Pts',(-6.21212744943719,133.38125547614,8.55025990906793));
#285551=CARTESIAN_POINT('Ctrl Pts',(-3.10606372471864,133.531255476139,
9.55948119098353));
#285552=CARTESIAN_POINT('Ctrl Pts',(-8.7523632448861E-14,133.681255476139,
10.5687024728991));
#285553=CARTESIAN_POINT('Ctrl Pts',(3.10606372471846,133.831255476138,9.55948119098353));
#285554=CARTESIAN_POINT('Ctrl Pts',(6.21212744943701,133.981255476138,8.55025990906793));
#285555=CARTESIAN_POINT('Ctrl Pts',(8.13178040253617,134.131255476137,5.90808429084315));
#285556=CARTESIAN_POINT('Ctrl Pts',(10.0514333556353,134.281255476136,3.26590867261836));
#285557=CARTESIAN_POINT('Ctrl Pts',(10.0514333556353,134.431255476136,-1.23094556858219E-15));
#285558=CARTESIAN_POINT('Ctrl Pts',(10.0514333556353,134.581255476135,-3.26590867261837));
#285559=CARTESIAN_POINT('Ctrl Pts',(8.13178040253617,134.731255476135,-5.90808429084315));
#285560=CARTESIAN_POINT('Ctrl Pts',(6.21212744943701,134.881255476134,-8.55025990906793));
#285561=CARTESIAN_POINT('Ctrl Pts',(3.10606372471846,135.031255476133,-9.55948119098353));
#285562=CARTESIAN_POINT('Ctrl Pts',(-9.09760726156073E-14,135.181255476133,
-10.5687024728991));
#285563=CARTESIAN_POINT('Ctrl Pts',(-3.10606372471864,135.331255476132,
-9.55948119098353));
#285564=CARTESIAN_POINT('Ctrl Pts',(-6.21212744943719,135.481255476132,
-8.55025990906793));
#285565=CARTESIAN_POINT('Ctrl Pts',(-8.13178040253636,135.631255476131,
-5.90808429084315));
#285566=CARTESIAN_POINT('Ctrl Pts',(-10.0514333556355,135.78125547613,-3.26590867261836));
#285567=CARTESIAN_POINT('Ctrl Pts',(-10.0514333556355,135.93125547613,2.46189113716437E-15));
#285568=CARTESIAN_POINT('Ctrl Pts',(-10.0514333556355,136.081255476129,
3.26590867261837));
#285569=CARTESIAN_POINT('Ctrl Pts',(-8.13178040253636,136.231255476129,
5.90808429084315));
#285570=CARTESIAN_POINT('Ctrl Pts',(-6.21212744943719,136.381255476128,
8.55025990906793));
#285571=CARTESIAN_POINT('Ctrl Pts',(-3.10606372471864,136.531255476127,
9.55948119098353));
#285572=CARTESIAN_POINT('Ctrl Pts',(-8.92513417205229E-14,136.681255476127,
10.5687024728991));
#285573=CARTESIAN_POINT('Ctrl Pts',(3.10606372471846,136.831255476126,9.55948119098353));
#285574=CARTESIAN_POINT('Ctrl Pts',(6.21212744943701,136.981255476126,8.55025990906793));
#285575=CARTESIAN_POINT('Ctrl Pts',(8.13178040253617,137.131255476125,5.90808429084315));
#285576=CARTESIAN_POINT('Ctrl Pts',(10.0514333556353,137.281255476124,3.26590867261836));
#285577=CARTESIAN_POINT('Ctrl Pts',(10.0514333556353,137.431255476124,-1.23094556858219E-15));
#285578=CARTESIAN_POINT('Ctrl Pts',(10.0514333556353,137.581255476123,-3.26590867261837));
#285579=CARTESIAN_POINT('Ctrl Pts',(8.13178040253617,137.731255476123,-5.90808429084315));
#285580=CARTESIAN_POINT('Ctrl Pts',(6.21212744943701,137.881255476122,-8.55025990906793));
#285581=CARTESIAN_POINT('Ctrl Pts',(3.10606372471846,138.031255476121,-9.55948119098353));
#285582=CARTESIAN_POINT('Ctrl Pts',(-9.27037818872691E-14,138.181255476121,
-10.5687024728991));
#285583=CARTESIAN_POINT('Ctrl Pts',(-3.10606372471864,138.33125547612,-9.55948119098353));
#285584=CARTESIAN_POINT('Ctrl Pts',(-6.21212744943719,138.48125547612,-8.55025990906793));
#285585=CARTESIAN_POINT('Ctrl Pts',(-8.13178040253636,138.631255476119,
-5.90808429084315));
#285586=CARTESIAN_POINT('Ctrl Pts',(-10.0514333556355,138.781255476118,
-3.26590867261836));
#285587=CARTESIAN_POINT('Ctrl Pts',(-10.0514333556355,138.931255476118,
2.46189113716437E-15));
#285588=CARTESIAN_POINT('Ctrl Pts',(-10.0514333556355,139.081255476117,
3.26590867261837));
#285589=CARTESIAN_POINT('Ctrl Pts',(-8.13178040253636,139.231255476117,
5.90808429084315));
#285590=CARTESIAN_POINT('Ctrl Pts',(-6.21212744943719,139.381255476116,
8.55025990906793));
#285591=CARTESIAN_POINT('Ctrl Pts',(-3.10606372471864,139.531255476115,
9.55948119098353));
#285592=CARTESIAN_POINT('Ctrl Pts',(-9.09790509921847E-14,139.681255476115,
10.5687024728991));
#285593=CARTESIAN_POINT('Ctrl Pts',(3.10606372471846,139.831255476114,9.55948119098353));
#285594=CARTESIAN_POINT('Ctrl Pts',(6.21212744943701,139.981255476114,8.55025990906793));
#285595=CARTESIAN_POINT('Ctrl Pts',(8.13178040253617,140.131255476113,5.90808429084315));
#285596=CARTESIAN_POINT('Ctrl Pts',(10.0514333556353,140.281255476112,3.26590867261836));
#285597=CARTESIAN_POINT('Ctrl Pts',(10.0514333556353,140.431255476112,-1.23094556858219E-15));
#285598=CARTESIAN_POINT('Ctrl Pts',(10.0514333556353,140.581255476111,-3.26590867261837));
#285599=CARTESIAN_POINT('Ctrl Pts',(8.13178040253617,140.731255476111,-5.90808429084315));
#285600=CARTESIAN_POINT('Ctrl Pts',(6.21212744943701,140.88125547611,-8.55025990906793));
#285601=CARTESIAN_POINT('Ctrl Pts',(3.10606372471846,141.031255476109,-9.55948119098353));
#285602=CARTESIAN_POINT('Ctrl Pts',(-9.4431491158931E-14,141.181255476109,
-10.5687024728991));
#285603=CARTESIAN_POINT('Ctrl Pts',(-3.10606372471864,141.331255476108,
-9.55948119098353));
#285604=CARTESIAN_POINT('Ctrl Pts',(-6.2121274494372,141.481255476108,-8.55025990906793));
#285605=CARTESIAN_POINT('Ctrl Pts',(-8.13178040253636,141.631255476107,
-5.90808429084315));
#285606=CARTESIAN_POINT('Ctrl Pts',(-10.0514333556355,141.781255476106,
-3.26590867261836));
#285607=CARTESIAN_POINT('Ctrl Pts',(-10.0514333556355,141.931255476106,
2.46189113716437E-15));
#285608=CARTESIAN_POINT('Ctrl Pts',(-10.0514333556355,142.081255476105,
3.26590867261837));
#285609=CARTESIAN_POINT('Ctrl Pts',(-8.13178040253636,142.231255476105,
5.90808429084315));
#285610=CARTESIAN_POINT('Ctrl Pts',(-6.21212744943719,142.381255476104,
8.55025990906793));
#285611=CARTESIAN_POINT('Ctrl Pts',(-3.10606372471864,142.531255476103,
9.55948119098353));
#285612=CARTESIAN_POINT('Ctrl Pts',(-9.27067602638466E-14,142.681255476103,
10.5687024728991));
#285613=CARTESIAN_POINT('Ctrl Pts',(3.10606372471846,142.831255476102,9.55948119098353));
#285614=CARTESIAN_POINT('Ctrl Pts',(6.21212744943701,142.981255476102,8.55025990906793));
#285615=CARTESIAN_POINT('Ctrl Pts',(8.13178040253617,143.131255476101,5.90808429084315));
#285616=CARTESIAN_POINT('Ctrl Pts',(10.0514333556353,143.2812554761,3.26590867261836));
#285617=CARTESIAN_POINT('Ctrl Pts',(10.0514333556353,143.4312554761,-1.23094556858219E-15));
#285618=CARTESIAN_POINT('Ctrl Pts',(10.0514333556353,143.581255476099,-3.26590867261837));
#285619=CARTESIAN_POINT('Ctrl Pts',(8.13178040253617,143.731255476099,-5.90808429084315));
#285620=CARTESIAN_POINT('Ctrl Pts',(6.21212744943701,143.881255476098,-8.55025990906793));
#285621=CARTESIAN_POINT('Ctrl Pts',(3.10606372471845,144.031255476097,-9.55948119098353));
#285622=CARTESIAN_POINT('Ctrl Pts',(-9.61592004305929E-14,144.181255476097,
-10.5687024728991));
#285623=CARTESIAN_POINT('Ctrl Pts',(-3.10606372471865,144.331255476096,
-9.55948119098353));
#285624=CARTESIAN_POINT('Ctrl Pts',(-6.2121274494372,144.481255476096,-8.55025990906793));
#285625=CARTESIAN_POINT('Ctrl Pts',(-8.13178040253636,144.631255476095,
-5.90808429084315));
#285626=CARTESIAN_POINT('Ctrl Pts',(-10.0514333556355,144.781255476094,
-3.26590867261836));
#285627=CARTESIAN_POINT('Ctrl Pts',(-10.0514333556355,144.931255476094,
2.46189113716437E-15));
#285628=CARTESIAN_POINT('Ctrl Pts',(-10.0514333556355,145.081255476093,
3.26590867261837));
#285629=CARTESIAN_POINT('Ctrl Pts',(-8.13178040253636,145.231255476093,
5.90808429084315));
#285630=CARTESIAN_POINT('Ctrl Pts',(-6.2121274494372,145.381255476092,8.55025990906793));
#285631=CARTESIAN_POINT('Ctrl Pts',(-3.10606372471864,145.531255476091,
9.55948119098353));
#285632=CARTESIAN_POINT('Ctrl Pts',(-9.44344695355084E-14,145.681255476091,
10.5687024728991));
#285633=CARTESIAN_POINT('Ctrl Pts',(3.10606372471846,145.83125547609,9.55948119098353));
#285634=CARTESIAN_POINT('Ctrl Pts',(6.21212744943701,145.98125547609,8.55025990906793));
#285635=CARTESIAN_POINT('Ctrl Pts',(8.13178040253617,146.131255476089,5.90808429084315));
#285636=CARTESIAN_POINT('Ctrl Pts',(10.0514333556353,146.281255476088,3.26590867261836));
#285637=CARTESIAN_POINT('Ctrl Pts',(10.0514333556353,146.431255476088,-1.23094556858219E-15));
#285638=CARTESIAN_POINT('Ctrl Pts',(10.0514333556353,146.581255476087,-3.26590867261837));
#285639=CARTESIAN_POINT('Ctrl Pts',(8.13178040253617,146.731255476087,-5.90808429084315));
#285640=CARTESIAN_POINT('Ctrl Pts',(6.212127449437,146.881255476086,-8.55025990906793));
#285641=CARTESIAN_POINT('Ctrl Pts',(3.10606372471845,147.031255476085,-9.55948119098353));
#285642=CARTESIAN_POINT('Ctrl Pts',(-9.78869097022547E-14,147.181255476085,
-10.5687024728991));
#285643=CARTESIAN_POINT('Ctrl Pts',(-3.10606372471865,147.331255476084,
-9.55948119098353));
#285644=CARTESIAN_POINT('Ctrl Pts',(-6.2121274494372,147.481255476084,-8.55025990906793));
#285645=CARTESIAN_POINT('Ctrl Pts',(-8.13178040253636,147.631255476083,
-5.90808429084315));
#285646=CARTESIAN_POINT('Ctrl Pts',(-10.0514333556355,147.781255476082,
-3.26590867261836));
#285647=CARTESIAN_POINT('Ctrl Pts',(-10.0514333556355,147.931255476082,
2.46189113716437E-15));
#285648=CARTESIAN_POINT('Ctrl Pts',(-10.0514333556355,148.081255476081,
3.26590867261837));
#285649=CARTESIAN_POINT('Ctrl Pts',(-8.13178040253636,148.231255476081,
5.90808429084315));
#285650=CARTESIAN_POINT('Ctrl Pts',(-6.2121274494372,148.38125547608,8.55025990906793));
#285651=CARTESIAN_POINT('Ctrl Pts',(-3.10606372471865,148.531255476079,
9.55948119098353));
#285652=CARTESIAN_POINT('Ctrl Pts',(-9.61621788071703E-14,148.681255476079,
10.5687024728991));
#285653=CARTESIAN_POINT('Ctrl Pts',(3.10606372471845,148.831255476078,9.55948119098353));
#285654=CARTESIAN_POINT('Ctrl Pts',(6.21212744943701,148.981255476078,8.55025990906793));
#285655=CARTESIAN_POINT('Ctrl Pts',(8.13178040253617,149.131255476077,5.90808429084315));
#285656=CARTESIAN_POINT('Ctrl Pts',(10.0514333556353,149.281255476076,3.26590867261836));
#285657=CARTESIAN_POINT('Ctrl Pts',(10.0514333556353,149.431255476076,-1.23094556858219E-15));
#285658=CARTESIAN_POINT('Ctrl Pts',(10.0514333556353,149.581255476075,-3.26590867261837));
#285659=CARTESIAN_POINT('Ctrl Pts',(8.13178040253617,149.731255476075,-5.90808429084315));
#285660=CARTESIAN_POINT('Ctrl Pts',(6.212127449437,149.881255476074,-8.55025990906793));
#285661=CARTESIAN_POINT('Ctrl Pts',(3.10606372471845,150.031255476073,-9.55948119098353));
#285662=CARTESIAN_POINT('Ctrl Pts',(-9.96146189739165E-14,150.181255476073,
-10.5687024728991));
#285663=CARTESIAN_POINT('Ctrl Pts',(-3.10606372471865,150.331255476072,
-9.55948119098353));
#285664=CARTESIAN_POINT('Ctrl Pts',(-6.2121274494372,150.481255476072,-8.55025990906793));
#285665=CARTESIAN_POINT('Ctrl Pts',(-8.13178040253636,150.631255476071,
-5.90808429084315));
#285666=CARTESIAN_POINT('Ctrl Pts',(-10.0514333556355,150.78125547607,-3.26590867261836));
#285667=CARTESIAN_POINT('Ctrl Pts',(-10.0514333556355,150.93125547607,2.46189113716437E-15));
#285668=CARTESIAN_POINT('Ctrl Pts',(-10.0514333556355,151.081255476069,
3.26590867261837));
#285669=CARTESIAN_POINT('Ctrl Pts',(-8.13178040253636,151.231255476069,
5.90808429084315));
#285670=CARTESIAN_POINT('Ctrl Pts',(-6.2121274494372,151.381255476068,8.55025990906793));
#285671=CARTESIAN_POINT('Ctrl Pts',(-3.10606372471865,151.531255476067,
9.55948119098353));
#285672=CARTESIAN_POINT('Ctrl Pts',(-9.78898880788321E-14,151.681255476067,
10.5687024728991));
#285673=CARTESIAN_POINT('Ctrl Pts',(3.10606372471845,151.831255476066,9.55948119098353));
#285674=CARTESIAN_POINT('Ctrl Pts',(6.212127449437,151.981255476066,8.55025990906793));
#285675=CARTESIAN_POINT('Ctrl Pts',(8.13178040253616,152.131255476065,5.90808429084315));
#285676=CARTESIAN_POINT('Ctrl Pts',(10.0514333556353,152.281255476064,3.26590867261836));
#285677=CARTESIAN_POINT('Ctrl Pts',(10.0514333556353,152.431255476064,-1.23094556858219E-15));
#285678=CARTESIAN_POINT('Ctrl Pts',(10.0514333556353,152.581255476063,-3.26590867261837));
#285679=CARTESIAN_POINT('Ctrl Pts',(8.13178040253616,152.731255476063,-5.90808429084315));
#285680=CARTESIAN_POINT('Ctrl Pts',(6.212127449437,152.881255476062,-8.55025990906793));
#285681=CARTESIAN_POINT('Ctrl Pts',(3.10606372471845,153.031255476061,-9.55948119098353));
#285682=CARTESIAN_POINT('Ctrl Pts',(-1.01342328245578E-13,153.181255476061,
-10.5687024728991));
#285683=CARTESIAN_POINT('Ctrl Pts',(-3.10606372471865,153.33125547606,-9.55948119098353));
#285684=CARTESIAN_POINT('Ctrl Pts',(10.0514428414942,2.43125000000076,-1.23094673026484E-15));
#285685=CARTESIAN_POINT('Ctrl Pts',(10.0514428414941,2.58125000000016,-3.26591175476071));
#285686=CARTESIAN_POINT('Ctrl Pts',(8.13178807675718,2.73124999999956,-5.90808986649102));
#285687=CARTESIAN_POINT('Ctrl Pts',(6.2121333120202,2.88124999999896,-8.55026797822134));
#285688=CARTESIAN_POINT('Ctrl Pts',(3.10606665601009,3.03124999999835,-9.5594902125713));
#285689=CARTESIAN_POINT('Ctrl Pts',(-1.49568621191919E-14,3.18124999999775,
-10.5687124469213));
#285690=CARTESIAN_POINT('Ctrl Pts',(-3.10606665601012,3.33124999999715,
-9.5594902125713));
#285691=CARTESIAN_POINT('Ctrl Pts',(-6.21213331202023,3.48124999999655,
-8.55026797822134));
#285692=CARTESIAN_POINT('Ctrl Pts',(-8.13178807675721,3.63124999999595,
-5.90808986649102));
#285693=CARTESIAN_POINT('Ctrl Pts',(-10.0514428414942,3.78124999999535,
-3.2659117547607));
#285694=CARTESIAN_POINT('Ctrl Pts',(-10.0514428414942,3.93124999999475,
2.46189346052968E-15));
#285695=CARTESIAN_POINT('Ctrl Pts',(-10.0514428414942,4.08124999999415,
3.26591175476071));
#285696=CARTESIAN_POINT('Ctrl Pts',(-8.13178807675721,4.23124999999355,
5.90808986649102));
#285697=CARTESIAN_POINT('Ctrl Pts',(-6.21213331202023,4.38124999999295,
8.55026797822134));
#285698=CARTESIAN_POINT('Ctrl Pts',(-3.10606665601012,4.53124999999235,
9.5594902125713));
#285699=CARTESIAN_POINT('Ctrl Pts',(-1.32321287811766E-14,4.68124999999175,
10.5687124469213));
#285700=CARTESIAN_POINT('Ctrl Pts',(3.10606665601009,4.83124999999115,9.5594902125713));
#285701=CARTESIAN_POINT('Ctrl Pts',(6.2121333120202,4.98124999999056,8.55026797822134));
#285702=CARTESIAN_POINT('Ctrl Pts',(8.13178807675718,5.13124999998996,5.90808986649102));
#285703=CARTESIAN_POINT('Ctrl Pts',(10.0514428414941,5.28124999998936,3.2659117547607));
#285704=CARTESIAN_POINT('Ctrl Pts',(10.0514428414941,5.43124999998876,-1.23094673026484E-15));
#285705=CARTESIAN_POINT('Origin',(-3.77475828372553E-14,-1.881249999982,
2.68644078414671E-15));
#285706=CARTESIAN_POINT('Origin',(-3.77475828372553E-14,-1.881249999982,
2.68644078414671E-15));
#285707=CARTESIAN_POINT('',(10.0514428414941,74.8062499997113,1.13714546409981E-15));
#285708=CARTESIAN_POINT('',(10.0514428414941,74.4312499997127,1.13870218092026E-15));
#285709=CARTESIAN_POINT('',(10.0514428414941,-1.881249999982,4.14193483802857E-15));
#285710=CARTESIAN_POINT('',(-9.80715114026992,73.2014428414942,-2.20256434814687));
#285711=CARTESIAN_POINT('Ctrl Pts',(-9.80715114026993,73.2014428414942,
-2.20256434814687));
#285712=CARTESIAN_POINT('Ctrl Pts',(-10.0514428414942,73.2550470089109,
-1.11482966369299));
#285713=CARTESIAN_POINT('Ctrl Pts',(-10.0514428414942,73.3062499997172,
2.46189346052968E-15));
#285714=CARTESIAN_POINT('Ctrl Pts',(-10.0514428414942,73.4562499997166,
3.26591175476071));
#285715=CARTESIAN_POINT('Ctrl Pts',(-8.13178807675725,73.606249999716,5.90808986649102));
#285716=CARTESIAN_POINT('Ctrl Pts',(-6.21213331202027,73.7562499997155,
8.55026797822134));
#285717=CARTESIAN_POINT('Ctrl Pts',(-3.10606665601016,73.9062499997148,
9.5594902125713));
#285718=CARTESIAN_POINT('Ctrl Pts',(-5.31854056883567E-14,74.0562499997142,
10.5687124469213));
#285719=CARTESIAN_POINT('Ctrl Pts',(3.10606665601005,74.2062499997136,9.5594902125713));
#285720=CARTESIAN_POINT('Ctrl Pts',(6.21213331202016,74.356249999713,8.55026797822134));
#285721=CARTESIAN_POINT('Ctrl Pts',(8.13178807675713,74.5062499997125,5.90808986649102));
#285722=CARTESIAN_POINT('Ctrl Pts',(10.0514428414941,74.6562499997118,3.2659117547607));
#285723=CARTESIAN_POINT('Ctrl Pts',(10.0514428414941,74.8062499997113,-1.23094673026484E-15));
#285724=CARTESIAN_POINT('',(-8.49270765599395,73.2014428414942,5.37637609042067));
#285725=CARTESIAN_POINT('Origin',(-3.44169137633799E-13,73.2014428414937,
6.99440505513849E-14));
#285726=CARTESIAN_POINT('Ctrl Pts',(-8.49270765599395,73.2014428414942,
5.37637609042067));
#285727=CARTESIAN_POINT('Ctrl Pts',(-8.32075096758918,73.2164846189077,
5.64800475990998));
#285728=CARTESIAN_POINT('Ctrl Pts',(-8.13178807675725,73.2312499997175,
5.90808986649102));
#285729=CARTESIAN_POINT('Ctrl Pts',(-6.21213331202027,73.381249999717,8.55026797822134));
#285730=CARTESIAN_POINT('Ctrl Pts',(-3.10606665601016,73.5312499997164,
9.5594902125713));
#285731=CARTESIAN_POINT('Ctrl Pts',(-5.29694420293989E-14,73.6812499997157,
10.5687124469213));
#285732=CARTESIAN_POINT('Ctrl Pts',(3.10606665601005,73.8312499997151,9.5594902125713));
#285733=CARTESIAN_POINT('Ctrl Pts',(6.21213331202016,73.9812499997146,8.55026797822134));
#285734=CARTESIAN_POINT('Ctrl Pts',(8.13178807675713,74.1312499997139,5.90808986649102));
#285735=CARTESIAN_POINT('Ctrl Pts',(10.0514428414941,74.2812499997134,3.2659117547607));
#285736=CARTESIAN_POINT('Ctrl Pts',(10.0514428414941,74.4312499997127,-1.23094673026484E-15));
#285737=CARTESIAN_POINT('Origin',(-5.57567406742018E-14,75.15,0.));
#285738=CARTESIAN_POINT('',(-9.00737896806879,75.15,7.92887912164091));
#285739=CARTESIAN_POINT('',(10.8311093380487,73.9811093380487,1.23959468221528E-12));
#285740=CARTESIAN_POINT('Ctrl Pts',(-9.00737896806883,75.15,7.92887912164089));
#285741=CARTESIAN_POINT('Ctrl Pts',(-9.69820351182042,75.1230722699582,
7.10333352735252));
#285742=CARTESIAN_POINT('Ctrl Pts',(-10.2770817627655,75.0969971768594,
6.18705949069743));
#285743=CARTESIAN_POINT('Ctrl Pts',(-11.1547474128912,75.0427147698165,
4.2537276641924));
#285744=CARTESIAN_POINT('Ctrl Pts',(-11.458772149512,75.0156043034968,3.25192351069933));
#285745=CARTESIAN_POINT('Ctrl Pts',(-11.8647044188623,74.9511670414305,
0.785797690073358));
#285746=CARTESIAN_POINT('Ctrl Pts',(-11.8535693691975,74.9132994586075,
-0.790228468608902));
#285747=CARTESIAN_POINT('Ctrl Pts',(-11.1272611500066,74.8311653831481,
-3.85248059592555));
#285748=CARTESIAN_POINT('Ctrl Pts',(-10.5113513970943,74.7917269214171,
-5.22009107154959));
#285749=CARTESIAN_POINT('Ctrl Pts',(-8.7026739046729,74.7115308255432,-7.78917298606851));
#285750=CARTESIAN_POINT('Ctrl Pts',(-7.5487369270328,74.6715996731515,-8.81702800061587));
#285751=CARTESIAN_POINT('Ctrl Pts',(-5.10207743581983,74.5943169629155,
-10.3505447400521));
#285752=CARTESIAN_POINT('Ctrl Pts',(-3.69969618597168,74.5565407709911,
-10.8915507233601));
#285753=CARTESIAN_POINT('Ctrl Pts',(-0.794814890740859,74.4783147165169,
-11.3946227024501));
#285754=CARTESIAN_POINT('Ctrl Pts',(0.68139788608677,74.438150792467,-11.3620602603414));
#285755=CARTESIAN_POINT('Ctrl Pts',(3.56236022636539,74.3589289937623,-10.731143902091));
#285756=CARTESIAN_POINT('Ctrl Pts',(4.93923718168667,74.3204915277411,-10.1294577658183));
#285757=CARTESIAN_POINT('Ctrl Pts',(7.40978785039317,74.2370194901842,-8.38810103154457));
#285758=CARTESIAN_POINT('Ctrl Pts',(8.35522120235473,74.1986788538341,-7.33447343383047));
#285759=CARTESIAN_POINT('Ctrl Pts',(9.82758315111317,74.1271233244885,-5.09784210187931));
#285760=CARTESIAN_POINT('Ctrl Pts',(10.3737336163218,74.0865160949434,-3.75031615897431));
#285761=CARTESIAN_POINT('Ctrl Pts',(10.7834985097843,74.0248962589012,-1.59575373885132));
#285762=CARTESIAN_POINT('Ctrl Pts',(10.8530454382111,74.0030454382112,-0.811792966467046));
#285763=CARTESIAN_POINT('Ctrl Pts',(10.8311093380487,73.9811093380488,2.51063073936938E-12));
#285764=CARTESIAN_POINT('',(13.0499999999999,76.2,1.59816407288729E-15));
#285765=CARTESIAN_POINT('',(11.9999999999999,75.15,-1.46957615897682E-15));
#285766=CARTESIAN_POINT('Origin',(-5.57567406742018E-14,76.2,-8.12023357684304E-15));
#285767=CARTESIAN_POINT('Ctrl Pts',(10.8311093380487,73.9811093380487,2.52256548982643E-12));
#285768=CARTESIAN_POINT('Ctrl Pts',(10.8143119258943,73.9643119258943,0.621624670788195));
#285769=CARTESIAN_POINT('Ctrl Pts',(10.7431385725595,73.9465278308509,1.25952363016472));
#285770=CARTESIAN_POINT('Ctrl Pts',(10.3237926143794,73.8885847118865,3.26531548950345));
#285771=CARTESIAN_POINT('Ctrl Pts',(9.77869754599333,73.8484301454163,4.55624067764685));
#285772=CARTESIAN_POINT('Ctrl Pts',(8.61389083368662,73.7901623606025,6.28474801719199));
#285773=CARTESIAN_POINT('Ctrl Pts',(8.16898248558591,73.77113065584,6.82379315457571));
#285774=CARTESIAN_POINT('Ctrl Pts',(6.71221416695348,73.712602997372,8.26680986406343));
#285775=CARTESIAN_POINT('Ctrl Pts',(5.57794501718321,73.6728079061673,9.02448648548346));
#285776=CARTESIAN_POINT('Ctrl Pts',(3.07022473208152,73.5946463655228,10.0763920380405));
#285777=CARTESIAN_POINT('Ctrl Pts',(1.71801133373339,73.5565913691597,10.3549183732943));
#285778=CARTESIAN_POINT('Ctrl Pts',(-0.326019100965161,73.495969531245,
10.3626740067965));
#285779=CARTESIAN_POINT('Ctrl Pts',(-0.997426943464804,73.4759407193955,
10.2996319059488));
#285780=CARTESIAN_POINT('Ctrl Pts',(-2.90140476360216,73.4188140988677,
9.93141432674302));
#285781=CARTESIAN_POINT('Ctrl Pts',(-4.18281817054363,73.3808750952915,
9.44793966102463));
#285782=CARTESIAN_POINT('Ctrl Pts',(-6.01121350243221,73.314726247914,8.23101639980502));
#285783=CARTESIAN_POINT('Ctrl Pts',(-6.5879521784306,73.291939229436,7.7472886059721));
#285784=CARTESIAN_POINT('Ctrl Pts',(-7.63444987216405,73.2463907888306,
6.65109656225167));
#285785=CARTESIAN_POINT('Ctrl Pts',(-8.10174935464808,73.2241898391348,
6.03647401622192));
#285786=CARTESIAN_POINT('Ctrl Pts',(-8.49270765599396,73.2014428414942,
5.37637609042066));
#285787=CARTESIAN_POINT('',(-0.772542478744793,75.15,11.975106601552));
#285788=CARTESIAN_POINT('Ctrl Pts',(-0.772542478745,75.15,11.975106601552));
#285789=CARTESIAN_POINT('Ctrl Pts',(-2.04083064796245,75.0278624546732,
11.7708948887632));
#285790=CARTESIAN_POINT('Ctrl Pts',(-3.28683095100001,74.9079915841135,
11.361657813701));
#285791=CARTESIAN_POINT('Ctrl Pts',(-5.51313922720053,74.667613993203,10.1863677934907));
#285792=CARTESIAN_POINT('Ctrl Pts',(-6.50027462213247,74.544601786977,9.43829777442363));
#285793=CARTESIAN_POINT('Ctrl Pts',(-8.13242682116904,74.3050792679408,
7.7192133645345));
#285794=CARTESIAN_POINT('Ctrl Pts',(-9.05390526764337,74.1607724922424,
6.50436427171037));
#285795=CARTESIAN_POINT('Ctrl Pts',(-10.1033813875356,73.8512496555443,
3.72785548679263));
#285796=CARTESIAN_POINT('Ctrl Pts',(-10.3342684942795,73.7200889598579,
2.52709309126293));
#285797=CARTESIAN_POINT('Ctrl Pts',(-10.3754040919887,73.4810018608485,
0.302332627258651));
#285798=CARTESIAN_POINT('Ctrl Pts',(-10.2570731251301,73.3564895116309,
-0.906797363353994));
#285799=CARTESIAN_POINT('Ctrl Pts',(-9.8071511402699,73.2014428414942,-2.20256434814686));
#285800=CARTESIAN_POINT('Origin',(-5.57567406742018E-14,75.15,0.));
#285801=CARTESIAN_POINT('Origin',(-8.79029313101884E-14,130.96875,0.));
#285802=CARTESIAN_POINT('',(10.158727500065,76.2,-6.38750777529532));
#285803=CARTESIAN_POINT('',(11.7004490057565,76.2,2.66448739229345));
#285804=CARTESIAN_POINT('Origin',(-5.63614389192858E-14,76.2,0.));
#285805=CARTESIAN_POINT('Ctrl Pts',(11.7004490057565,76.2,2.66448739229345));
#285806=CARTESIAN_POINT('Ctrl Pts',(11.1542089550934,76.1008922571332,5.06316785750065));
#285807=CARTESIAN_POINT('Ctrl Pts',(9.70820393249932,76.0062499997072,7.05342302750968));
#285808=CARTESIAN_POINT('Ctrl Pts',(7.41640786499869,75.8562499997078,10.2078097002245));
#285809=CARTESIAN_POINT('Ctrl Pts',(3.70820393249932,75.7062499997084,11.4126781955418));
#285810=CARTESIAN_POINT('Ctrl Pts',(-5.36728955793647E-14,75.556249999709,
12.6175466908592));
#285811=CARTESIAN_POINT('Ctrl Pts',(-3.70820393249942,75.4062499997096,
11.4126781955418));
#285812=CARTESIAN_POINT('Ctrl Pts',(-6.83503484848808,75.2797670322315,
10.3967092441472));
#285813=CARTESIAN_POINT('Ctrl Pts',(-9.00737896806879,75.15,7.9288791216409));
#285814=CARTESIAN_POINT('Ctrl Pts',(10.1587275000636,76.1999999999992,-6.38750777529466));
#285815=CARTESIAN_POINT('Ctrl Pts',(10.7617685920941,76.1555651822736,-5.42842790552554));
#285816=CARTESIAN_POINT('Ctrl Pts',(11.2259449173429,76.1097672665456,-4.38879634680429));
#285817=CARTESIAN_POINT('Ctrl Pts',(11.9626296774665,76.0014610227487,-1.81289318850251));
#285818=CARTESIAN_POINT('Ctrl Pts',(12.0964698979846,75.9423786381454,-0.257928135750359));
#285819=CARTESIAN_POINT('Ctrl Pts',(11.7635714974025,75.8187973732225,2.84622558177574));
#285820=CARTESIAN_POINT('Ctrl Pts',(11.2886361360743,75.7544492469013,4.36454762104216));
#285821=CARTESIAN_POINT('Ctrl Pts',(9.78747214476226,75.6298418638766,7.11578131626414));
#285822=CARTESIAN_POINT('Ctrl Pts',(8.78158044779031,75.570682135926,8.32542804683128));
#285823=CARTESIAN_POINT('Ctrl Pts',(6.41003130511432,75.4472027071465,10.2546288766467));
#285824=CARTESIAN_POINT('Ctrl Pts',(5.08061870783028,75.3867653435368,10.9741776338188));
#285825=CARTESIAN_POINT('Ctrl Pts',(2.2250043460616,75.2712533161347,11.8868781811265));
#285826=CARTESIAN_POINT('Ctrl Pts',(0.723748485605121,75.2105262409342,
12.0716358742328));
#285827=CARTESIAN_POINT('Ctrl Pts',(-0.772542478744996,75.15,11.975106601552));
#285828=CARTESIAN_POINT('Ctrl Pts',(-10.0514428414942,-1.69374999998275,
2.46189346052968E-15));
#285829=CARTESIAN_POINT('Ctrl Pts',(-10.0514428414942,-1.54374999998335,
3.26591175476071));
#285830=CARTESIAN_POINT('Ctrl Pts',(-8.1317880767572,-1.39374999998395,
5.90808986649102));
#285831=CARTESIAN_POINT('Ctrl Pts',(-6.21213331202023,-1.24374999998455,
8.55026797822134));
#285832=CARTESIAN_POINT('Ctrl Pts',(-3.10606665601012,-1.09374999998515,
9.5594902125713));
#285833=CARTESIAN_POINT('Ctrl Pts',(-9.99267389681068E-15,-0.943749999985747,
10.5687124469213));
#285834=CARTESIAN_POINT('Ctrl Pts',(3.1060666560101,-0.793749999986346,
9.5594902125713));
#285835=CARTESIAN_POINT('Ctrl Pts',(6.21213331202021,-0.643749999986944,
8.55026797822134));
#285836=CARTESIAN_POINT('Ctrl Pts',(8.13178807675718,-0.493749999987543,
5.90808986649102));
#285837=CARTESIAN_POINT('Ctrl Pts',(10.0514428414942,-0.343749999988142,
3.2659117547607));
#285838=CARTESIAN_POINT('Ctrl Pts',(10.0514428414942,-0.193749999988742,
-1.23094673026484E-15));
#285839=CARTESIAN_POINT('Ctrl Pts',(10.0514428414942,-0.0437499999893418,
-3.26591175476071));
#285840=CARTESIAN_POINT('Ctrl Pts',(8.13178807675718,0.106250000010057,
-5.90808986649102));
#285841=CARTESIAN_POINT('Ctrl Pts',(6.2121333120202,0.256250000009456,-8.55026797822134));
#285842=CARTESIAN_POINT('Ctrl Pts',(3.10606665601009,0.406250000008854,
-9.5594902125713));
#285843=CARTESIAN_POINT('Ctrl Pts',(-1.34451165064878E-14,0.556250000008252,
-10.5687124469213));
#285844=CARTESIAN_POINT('Ctrl Pts',(-3.10606665601012,0.70625000000765,
-9.5594902125713));
#285845=CARTESIAN_POINT('Ctrl Pts',(-6.21213331202023,0.856250000007049,
-8.55026797822134));
#285846=CARTESIAN_POINT('Ctrl Pts',(-8.1317880767572,1.00625000000645,-5.90808986649102));
#285847=CARTESIAN_POINT('Ctrl Pts',(-10.0514428414942,1.15625000000585,
-3.2659117547607));
#285848=CARTESIAN_POINT('Ctrl Pts',(-10.0514428414942,1.30625000000525,
2.46189346052968E-15));
#285849=CARTESIAN_POINT('Ctrl Pts',(-10.0514428414942,1.45625000000465,
3.26591175476071));
#285850=CARTESIAN_POINT('Ctrl Pts',(-8.1317880767572,1.60625000000405,5.90808986649102));
#285851=CARTESIAN_POINT('Ctrl Pts',(-6.21213331202023,1.75625000000345,
8.55026797822134));
#285852=CARTESIAN_POINT('Ctrl Pts',(-3.10606665601012,1.90625000000285,
9.5594902125713));
#285853=CARTESIAN_POINT('Ctrl Pts',(-1.17203831684725E-14,2.05625000000225,
10.5687124469213));
#285854=CARTESIAN_POINT('Ctrl Pts',(3.1060666560101,2.20625000000165,9.5594902125713));
#285855=CARTESIAN_POINT('Ctrl Pts',(6.2121333120202,2.35625000000106,8.55026797822134));
#285856=CARTESIAN_POINT('Ctrl Pts',(8.13178807675718,2.50625000000046,5.90808986649102));
#285857=CARTESIAN_POINT('Ctrl Pts',(10.0514428414942,2.65624999999986,3.2659117547607));
#285858=CARTESIAN_POINT('Ctrl Pts',(10.0514428414942,2.80624999999926,-1.23094673026484E-15));
#285859=CARTESIAN_POINT('Ctrl Pts',(10.0514428414942,2.95624999999866,-3.26591175476071));
#285860=CARTESIAN_POINT('Ctrl Pts',(8.13178807675718,3.10624999999806,-5.90808986649102));
#285861=CARTESIAN_POINT('Ctrl Pts',(6.2121333120202,3.25624999999746,-8.55026797822134));
#285862=CARTESIAN_POINT('Ctrl Pts',(3.10606665601009,3.40624999999685,-9.5594902125713));
#285863=CARTESIAN_POINT('Ctrl Pts',(-1.51728257781496E-14,3.55624999999625,
-10.5687124469213));
#285864=CARTESIAN_POINT('Ctrl Pts',(-3.10606665601012,3.70624999999565,
-9.5594902125713));
#285865=CARTESIAN_POINT('Ctrl Pts',(-6.21213331202023,3.85624999999505,
-8.55026797822134));
#285866=CARTESIAN_POINT('Ctrl Pts',(-8.13178807675721,4.00624999999445,
-5.90808986649102));
#285867=CARTESIAN_POINT('Ctrl Pts',(-10.0514428414942,4.15624999999385,
-3.2659117547607));
#285868=CARTESIAN_POINT('Ctrl Pts',(-10.0514428414942,4.30624999999325,
2.46189346052968E-15));
#285869=CARTESIAN_POINT('Ctrl Pts',(-10.0514428414942,4.45624999999265,
3.26591175476071));
#285870=CARTESIAN_POINT('Ctrl Pts',(-8.13178807675721,4.60624999999205,
5.90808986649102));
#285871=CARTESIAN_POINT('Ctrl Pts',(-6.21213331202023,4.75624999999145,
8.55026797822134));
#285872=CARTESIAN_POINT('Ctrl Pts',(-3.10606665601012,4.90624999999085,
9.5594902125713));
#285873=CARTESIAN_POINT('Ctrl Pts',(-1.34480924401344E-14,5.05624999999025,
10.5687124469213));
#285874=CARTESIAN_POINT('Ctrl Pts',(3.10606665601009,5.20624999998966,9.5594902125713));
#285875=CARTESIAN_POINT('Ctrl Pts',(6.2121333120202,5.35624999998906,8.55026797822134));
#285876=CARTESIAN_POINT('Ctrl Pts',(8.13178807675718,5.50624999998846,5.90808986649102));
#285877=CARTESIAN_POINT('Ctrl Pts',(10.0514428414942,5.65624999998786,3.2659117547607));
#285878=CARTESIAN_POINT('Ctrl Pts',(10.0514428414941,5.80624999998726,-1.23094673026484E-15));
#285879=CARTESIAN_POINT('Ctrl Pts',(10.0514428414941,5.95624999998666,-3.26591175476071));
#285880=CARTESIAN_POINT('Ctrl Pts',(8.13178807675717,6.10624999998606,-5.90808986649102));
#285881=CARTESIAN_POINT('Ctrl Pts',(6.2121333120202,6.25624999998545,-8.55026797822134));
#285882=CARTESIAN_POINT('Ctrl Pts',(3.10606665601009,6.40624999998485,-9.5594902125713));
#285883=CARTESIAN_POINT('Ctrl Pts',(-1.69005350498115E-14,6.55624999998425,
-10.5687124469213));
#285884=CARTESIAN_POINT('Ctrl Pts',(-3.10606665601013,6.70624999998365,
-9.5594902125713));
#285885=CARTESIAN_POINT('Ctrl Pts',(-6.21213331202023,6.85624999998305,
-8.55026797822134));
#285886=CARTESIAN_POINT('Ctrl Pts',(-8.13178807675721,7.00624999998245,
-5.90808986649102));
#285887=CARTESIAN_POINT('Ctrl Pts',(-10.0514428414942,7.15624999998184,
-3.2659117547607));
#285888=CARTESIAN_POINT('Ctrl Pts',(-10.0514428414942,7.30624999998125,
2.46189346052968E-15));
#285889=CARTESIAN_POINT('Ctrl Pts',(-10.0514428414942,7.45624999998065,
3.26591175476071));
#285890=CARTESIAN_POINT('Ctrl Pts',(-8.13178807675721,7.60624999998005,
5.90808986649102));
#285891=CARTESIAN_POINT('Ctrl Pts',(-6.21213331202023,7.75624999997945,
8.55026797822134));
#285892=CARTESIAN_POINT('Ctrl Pts',(-3.10606665601012,7.90624999997885,
9.5594902125713));
#285893=CARTESIAN_POINT('Ctrl Pts',(-1.51758017117962E-14,8.05624999997825,
10.5687124469213));
#285894=CARTESIAN_POINT('Ctrl Pts',(3.10606665601009,8.20624999997765,9.5594902125713));
#285895=CARTESIAN_POINT('Ctrl Pts',(6.2121333120202,8.35624999997706,8.55026797822134));
#285896=CARTESIAN_POINT('Ctrl Pts',(8.13178807675717,8.50624999997646,5.90808986649102));
#285897=CARTESIAN_POINT('Ctrl Pts',(10.0514428414942,8.65624999997586,3.2659117547607));
#285898=CARTESIAN_POINT('Ctrl Pts',(10.0514428414941,8.80624999997526,-1.23094673026484E-15));
#285899=CARTESIAN_POINT('Ctrl Pts',(10.0514428414941,8.95624999997466,-3.26591175476071));
#285900=CARTESIAN_POINT('Ctrl Pts',(8.13178807675717,9.10624999997406,-5.90808986649102));
#285901=CARTESIAN_POINT('Ctrl Pts',(6.2121333120202,9.25624999997346,-8.55026797822134));
#285902=CARTESIAN_POINT('Ctrl Pts',(3.10606665601009,9.40624999997286,-9.5594902125713));
#285903=CARTESIAN_POINT('Ctrl Pts',(-1.86282443214733E-14,9.55624999997225,
-10.5687124469213));
#285904=CARTESIAN_POINT('Ctrl Pts',(-3.10606665601013,9.70624999997165,
-9.5594902125713));
#285905=CARTESIAN_POINT('Ctrl Pts',(-6.21213331202023,9.85624999997105,
-8.55026797822134));
#285906=CARTESIAN_POINT('Ctrl Pts',(-8.13178807675721,10.0062499999704,
-5.90808986649102));
#285907=CARTESIAN_POINT('Ctrl Pts',(-10.0514428414942,10.1562499999698,
-3.2659117547607));
#285908=CARTESIAN_POINT('Ctrl Pts',(-10.0514428414942,10.3062499999692,
2.46189346052968E-15));
#285909=CARTESIAN_POINT('Ctrl Pts',(-10.0514428414942,10.4562499999686,
3.26591175476071));
#285910=CARTESIAN_POINT('Ctrl Pts',(-8.13178807675721,10.606249999968,5.90808986649102));
#285911=CARTESIAN_POINT('Ctrl Pts',(-6.21213331202023,10.7562499999674,
8.55026797822134));
#285912=CARTESIAN_POINT('Ctrl Pts',(-3.10606665601013,10.9062499999668,
9.5594902125713));
#285913=CARTESIAN_POINT('Ctrl Pts',(-1.6903510983458E-14,11.0562499999663,
10.5687124469213));
#285914=CARTESIAN_POINT('Ctrl Pts',(3.10606665601009,11.2062499999657,9.5594902125713));
#285915=CARTESIAN_POINT('Ctrl Pts',(6.2121333120202,11.3562499999651,8.55026797822134));
#285916=CARTESIAN_POINT('Ctrl Pts',(8.13178807675717,11.5062499999645,5.90808986649102));
#285917=CARTESIAN_POINT('Ctrl Pts',(10.0514428414941,11.6562499999639,3.2659117547607));
#285918=CARTESIAN_POINT('Ctrl Pts',(10.0514428414941,11.8062499999633,-1.23094673026484E-15));
#285919=CARTESIAN_POINT('Ctrl Pts',(10.0514428414941,11.9562499999627,-3.26591175476071));
#285920=CARTESIAN_POINT('Ctrl Pts',(8.13178807675717,12.1062499999621,-5.90808986649102));
#285921=CARTESIAN_POINT('Ctrl Pts',(6.2121333120202,12.2562499999615,-8.55026797822134));
#285922=CARTESIAN_POINT('Ctrl Pts',(3.10606665601009,12.4062499999609,-9.5594902125713));
#285923=CARTESIAN_POINT('Ctrl Pts',(-2.03559535931351E-14,12.5562499999603,
-10.5687124469213));
#285924=CARTESIAN_POINT('Ctrl Pts',(-3.10606665601013,12.7062499999597,
-9.5594902125713));
#285925=CARTESIAN_POINT('Ctrl Pts',(-6.21213331202024,12.856249999959,-8.55026797822134));
#285926=CARTESIAN_POINT('Ctrl Pts',(-8.13178807675721,13.0062499999584,
-5.90808986649102));
#285927=CARTESIAN_POINT('Ctrl Pts',(-10.0514428414942,13.1562499999578,
-3.2659117547607));
#285928=CARTESIAN_POINT('Ctrl Pts',(-10.0514428414942,13.3062499999572,
2.46189346052968E-15));
#285929=CARTESIAN_POINT('Ctrl Pts',(-10.0514428414942,13.4562499999566,
3.26591175476071));
#285930=CARTESIAN_POINT('Ctrl Pts',(-8.13178807675721,13.606249999956,5.90808986649102));
#285931=CARTESIAN_POINT('Ctrl Pts',(-6.21213331202023,13.7562499999554,
8.55026797822134));
#285932=CARTESIAN_POINT('Ctrl Pts',(-3.10606665601013,13.9062499999549,
9.5594902125713));
#285933=CARTESIAN_POINT('Ctrl Pts',(-1.86312202551199E-14,14.0562499999543,
10.5687124469213));
#285934=CARTESIAN_POINT('Ctrl Pts',(3.10606665601009,14.2062499999537,9.5594902125713));
#285935=CARTESIAN_POINT('Ctrl Pts',(6.2121333120202,14.3562499999531,8.55026797822134));
#285936=CARTESIAN_POINT('Ctrl Pts',(8.13178807675717,14.5062499999525,5.90808986649102));
#285937=CARTESIAN_POINT('Ctrl Pts',(10.0514428414941,14.6562499999519,3.2659117547607));
#285938=CARTESIAN_POINT('Ctrl Pts',(10.0514428414941,14.8062499999513,-1.23094673026484E-15));
#285939=CARTESIAN_POINT('Ctrl Pts',(10.0514428414941,14.9562499999507,-3.26591175476071));
#285940=CARTESIAN_POINT('Ctrl Pts',(8.13178807675717,15.1062499999501,-5.90808986649102));
#285941=CARTESIAN_POINT('Ctrl Pts',(6.21213331202019,15.2562499999495,-8.55026797822134));
#285942=CARTESIAN_POINT('Ctrl Pts',(3.10606665601009,15.4062499999489,-9.5594902125713));
#285943=CARTESIAN_POINT('Ctrl Pts',(-2.2083662864797E-14,15.5562499999482,
-10.5687124469213));
#285944=CARTESIAN_POINT('Ctrl Pts',(-3.10606665601013,15.7062499999477,
-9.5594902125713));
#285945=CARTESIAN_POINT('Ctrl Pts',(-6.21213331202024,15.856249999947,-8.55026797822134));
#285946=CARTESIAN_POINT('Ctrl Pts',(-8.13178807675721,16.0062499999464,
-5.90808986649102));
#285947=CARTESIAN_POINT('Ctrl Pts',(-10.0514428414942,16.1562499999458,
-3.2659117547607));
#285948=CARTESIAN_POINT('Ctrl Pts',(-10.0514428414942,16.3062499999452,
2.46189346052968E-15));
#285949=CARTESIAN_POINT('Ctrl Pts',(-10.0514428414942,16.4562499999446,
3.26591175476071));
#285950=CARTESIAN_POINT('Ctrl Pts',(-8.13178807675721,16.606249999944,5.90808986649102));
#285951=CARTESIAN_POINT('Ctrl Pts',(-6.21213331202024,16.7562499999434,
8.55026797822134));
#285952=CARTESIAN_POINT('Ctrl Pts',(-3.10606665601013,16.9062499999428,
9.5594902125713));
#285953=CARTESIAN_POINT('Ctrl Pts',(-2.03589295267817E-14,17.0562499999422,
10.5687124469213));
#285954=CARTESIAN_POINT('Ctrl Pts',(3.10606665601009,17.2062499999417,9.5594902125713));
#285955=CARTESIAN_POINT('Ctrl Pts',(6.21213331202019,17.3562499999411,8.55026797822134));
#285956=CARTESIAN_POINT('Ctrl Pts',(8.13178807675717,17.5062499999405,5.90808986649102));
#285957=CARTESIAN_POINT('Ctrl Pts',(10.0514428414941,17.6562499999399,3.2659117547607));
#285958=CARTESIAN_POINT('Ctrl Pts',(10.0514428414941,17.8062499999393,-1.23094673026484E-15));
#285959=CARTESIAN_POINT('Ctrl Pts',(10.0514428414941,17.9562499999387,-3.26591175476071));
#285960=CARTESIAN_POINT('Ctrl Pts',(8.13178807675717,18.1062499999381,-5.90808986649102));
#285961=CARTESIAN_POINT('Ctrl Pts',(6.21213331202019,18.2562499999375,-8.55026797822134));
#285962=CARTESIAN_POINT('Ctrl Pts',(3.10606665601008,18.4062499999369,-9.5594902125713));
#285963=CARTESIAN_POINT('Ctrl Pts',(-2.38113721364588E-14,18.5562499999362,
-10.5687124469213));
#285964=CARTESIAN_POINT('Ctrl Pts',(-3.10606665601013,18.7062499999357,
-9.5594902125713));
#285965=CARTESIAN_POINT('Ctrl Pts',(-6.21213331202024,18.856249999935,-8.55026797822134));
#285966=CARTESIAN_POINT('Ctrl Pts',(-8.13178807675721,19.0062499999344,
-5.90808986649102));
#285967=CARTESIAN_POINT('Ctrl Pts',(-10.0514428414942,19.1562499999338,
-3.2659117547607));
#285968=CARTESIAN_POINT('Ctrl Pts',(-10.0514428414942,19.3062499999332,
2.46189346052968E-15));
#285969=CARTESIAN_POINT('Ctrl Pts',(-10.0514428414942,19.4562499999326,
3.26591175476071));
#285970=CARTESIAN_POINT('Ctrl Pts',(-8.13178807675721,19.606249999932,5.90808986649102));
#285971=CARTESIAN_POINT('Ctrl Pts',(-6.21213331202024,19.7562499999314,
8.55026797822134));
#285972=CARTESIAN_POINT('Ctrl Pts',(-3.10606665601013,19.9062499999308,
9.5594902125713));
#285973=CARTESIAN_POINT('Ctrl Pts',(-2.20866387984435E-14,20.0562499999302,
10.5687124469213));
#285974=CARTESIAN_POINT('Ctrl Pts',(3.10606665601009,20.2062499999297,9.5594902125713));
#285975=CARTESIAN_POINT('Ctrl Pts',(6.21213331202019,20.356249999929,8.55026797822134));
#285976=CARTESIAN_POINT('Ctrl Pts',(8.13178807675717,20.5062499999285,5.90808986649102));
#285977=CARTESIAN_POINT('Ctrl Pts',(10.0514428414941,20.6562499999279,3.2659117547607));
#285978=CARTESIAN_POINT('Ctrl Pts',(10.0514428414941,20.8062499999273,-1.23094673026484E-15));
#285979=CARTESIAN_POINT('Ctrl Pts',(10.0514428414941,20.9562499999267,-3.26591175476071));
#285980=CARTESIAN_POINT('Ctrl Pts',(8.13178807675716,21.1062499999261,-5.90808986649102));
#285981=CARTESIAN_POINT('Ctrl Pts',(6.21213331202019,21.2562499999255,-8.55026797822134));
#285982=CARTESIAN_POINT('Ctrl Pts',(3.10606665601008,21.4062499999249,-9.5594902125713));
#285983=CARTESIAN_POINT('Ctrl Pts',(-2.55390814081207E-14,21.5562499999242,
-10.5687124469213));
#285984=CARTESIAN_POINT('Ctrl Pts',(-3.10606665601013,21.7062499999237,
-9.5594902125713));
#285985=CARTESIAN_POINT('Ctrl Pts',(-6.21213331202024,21.856249999923,-8.55026797822134));
#285986=CARTESIAN_POINT('Ctrl Pts',(-8.13178807675722,22.0062499999224,
-5.90808986649102));
#285987=CARTESIAN_POINT('Ctrl Pts',(-10.0514428414942,22.1562499999218,
-3.2659117547607));
#285988=CARTESIAN_POINT('Ctrl Pts',(-10.0514428414942,22.3062499999212,
2.46189346052968E-15));
#285989=CARTESIAN_POINT('Ctrl Pts',(-10.0514428414942,22.4562499999206,
3.26591175476071));
#285990=CARTESIAN_POINT('Ctrl Pts',(-8.13178807675722,22.60624999992,5.90808986649102));
#285991=CARTESIAN_POINT('Ctrl Pts',(-6.21213331202024,22.7562499999194,
8.55026797822134));
#285992=CARTESIAN_POINT('Ctrl Pts',(-3.10606665601013,22.9062499999188,
9.5594902125713));
#285993=CARTESIAN_POINT('Ctrl Pts',(-2.38143480701054E-14,23.0562499999182,
10.5687124469213));
#285994=CARTESIAN_POINT('Ctrl Pts',(3.10606665601008,23.2062499999177,9.5594902125713));
#285995=CARTESIAN_POINT('Ctrl Pts',(6.21213331202019,23.3562499999171,8.55026797822134));
#285996=CARTESIAN_POINT('Ctrl Pts',(8.13178807675716,23.5062499999165,5.90808986649102));
#285997=CARTESIAN_POINT('Ctrl Pts',(10.0514428414941,23.6562499999159,3.2659117547607));
#285998=CARTESIAN_POINT('Ctrl Pts',(10.0514428414941,23.8062499999153,-1.23094673026484E-15));
#285999=CARTESIAN_POINT('Ctrl Pts',(10.0514428414941,23.9562499999147,-3.26591175476071));
#286000=CARTESIAN_POINT('Ctrl Pts',(8.13178807675716,24.1062499999141,-5.90808986649102));
#286001=CARTESIAN_POINT('Ctrl Pts',(6.21213331202019,24.2562499999135,-8.55026797822134));
#286002=CARTESIAN_POINT('Ctrl Pts',(3.10606665601008,24.4062499999129,-9.5594902125713));
#286003=CARTESIAN_POINT('Ctrl Pts',(-2.72667906797825E-14,24.5562499999122,
-10.5687124469213));
#286004=CARTESIAN_POINT('Ctrl Pts',(-3.10606665601014,24.7062499999116,
-9.5594902125713));
#286005=CARTESIAN_POINT('Ctrl Pts',(-6.21213331202024,24.856249999911,-8.55026797822134));
#286006=CARTESIAN_POINT('Ctrl Pts',(-8.13178807675722,25.0062499999104,
-5.90808986649102));
#286007=CARTESIAN_POINT('Ctrl Pts',(-10.0514428414942,25.1562499999098,
-3.2659117547607));
#286008=CARTESIAN_POINT('Ctrl Pts',(-10.0514428414942,25.3062499999092,
2.46189346052968E-15));
#286009=CARTESIAN_POINT('Ctrl Pts',(-10.0514428414942,25.4562499999086,
3.26591175476071));
#286010=CARTESIAN_POINT('Ctrl Pts',(-8.13178807675722,25.6062499999081,
5.90808986649102));
#286011=CARTESIAN_POINT('Ctrl Pts',(-6.21213331202024,25.7562499999074,
8.55026797822134));
#286012=CARTESIAN_POINT('Ctrl Pts',(-3.10606665601013,25.9062499999069,
9.5594902125713));
#286013=CARTESIAN_POINT('Ctrl Pts',(-2.55420573417672E-14,26.0562499999062,
10.5687124469213));
#286014=CARTESIAN_POINT('Ctrl Pts',(3.10606665601008,26.2062499999057,9.5594902125713));
#286015=CARTESIAN_POINT('Ctrl Pts',(6.21213331202019,26.356249999905,8.55026797822134));
#286016=CARTESIAN_POINT('Ctrl Pts',(8.13178807675716,26.5062499999045,5.90808986649102));
#286017=CARTESIAN_POINT('Ctrl Pts',(10.0514428414941,26.6562499999039,3.2659117547607));
#286018=CARTESIAN_POINT('Ctrl Pts',(10.0514428414941,26.8062499999033,-1.23094673026484E-15));
#286019=CARTESIAN_POINT('Ctrl Pts',(10.0514428414941,26.9562499999027,-3.26591175476071));
#286020=CARTESIAN_POINT('Ctrl Pts',(8.13178807675716,27.1062499999021,-5.90808986649102));
#286021=CARTESIAN_POINT('Ctrl Pts',(6.21213331202019,27.2562499999015,-8.55026797822134));
#286022=CARTESIAN_POINT('Ctrl Pts',(3.10606665601008,27.4062499999009,-9.5594902125713));
#286023=CARTESIAN_POINT('Ctrl Pts',(-2.89944999514443E-14,27.5562499999002,
-10.5687124469213));
#286024=CARTESIAN_POINT('Ctrl Pts',(-3.10606665601014,27.7062499998996,
-9.5594902125713));
#286025=CARTESIAN_POINT('Ctrl Pts',(-6.21213331202024,27.856249999899,-8.55026797822134));
#286026=CARTESIAN_POINT('Ctrl Pts',(-8.13178807675722,28.0062499998984,
-5.90808986649102));
#286027=CARTESIAN_POINT('Ctrl Pts',(-10.0514428414942,28.1562499998978,
-3.2659117547607));
#286028=CARTESIAN_POINT('Ctrl Pts',(-10.0514428414942,28.3062499998973,
2.46189346052968E-15));
#286029=CARTESIAN_POINT('Ctrl Pts',(-10.0514428414942,28.4562499998966,
3.26591175476071));
#286030=CARTESIAN_POINT('Ctrl Pts',(-8.13178807675722,28.606249999896,5.90808986649102));
#286031=CARTESIAN_POINT('Ctrl Pts',(-6.21213331202024,28.7562499998954,
8.55026797822134));
#286032=CARTESIAN_POINT('Ctrl Pts',(-3.10606665601014,28.9062499998949,
9.5594902125713));
#286033=CARTESIAN_POINT('Ctrl Pts',(-2.72697666134291E-14,29.0562499998942,
10.5687124469213));
#286034=CARTESIAN_POINT('Ctrl Pts',(3.10606665601008,29.2062499998937,9.5594902125713));
#286035=CARTESIAN_POINT('Ctrl Pts',(6.21213331202019,29.356249999893,8.55026797822134));
#286036=CARTESIAN_POINT('Ctrl Pts',(8.13178807675716,29.5062499998925,5.90808986649102));
#286037=CARTESIAN_POINT('Ctrl Pts',(10.0514428414941,29.6562499998919,3.2659117547607));
#286038=CARTESIAN_POINT('Ctrl Pts',(10.0514428414941,29.8062499998913,-1.23094673026484E-15));
#286039=CARTESIAN_POINT('Ctrl Pts',(10.0514428414941,29.9562499998907,-3.26591175476071));
#286040=CARTESIAN_POINT('Ctrl Pts',(8.13178807675716,30.1062499998901,-5.90808986649102));
#286041=CARTESIAN_POINT('Ctrl Pts',(6.21213331202019,30.2562499998895,-8.55026797822134));
#286042=CARTESIAN_POINT('Ctrl Pts',(3.10606665601008,30.4062499998889,-9.5594902125713));
#286043=CARTESIAN_POINT('Ctrl Pts',(-3.07222092231062E-14,30.5562499998883,
-10.5687124469213));
#286044=CARTESIAN_POINT('Ctrl Pts',(-3.10606665601014,30.7062499998877,
-9.5594902125713));
#286045=CARTESIAN_POINT('Ctrl Pts',(-6.21213331202025,30.8562499998871,
-8.55026797822134));
#286046=CARTESIAN_POINT('Ctrl Pts',(-8.13178807675722,31.0062499998864,
-5.90808986649102));
#286047=CARTESIAN_POINT('Ctrl Pts',(-10.0514428414942,31.1562499998858,
-3.2659117547607));
#286048=CARTESIAN_POINT('Ctrl Pts',(-10.0514428414942,31.3062499998852,
2.46189346052968E-15));
#286049=CARTESIAN_POINT('Ctrl Pts',(-10.0514428414942,31.4562499998847,
3.26591175476071));
#286050=CARTESIAN_POINT('Ctrl Pts',(-8.13178807675722,31.606249999884,5.90808986649102));
#286051=CARTESIAN_POINT('Ctrl Pts',(-6.21213331202024,31.7562499998835,
8.55026797822134));
#286052=CARTESIAN_POINT('Ctrl Pts',(-3.10606665601014,31.9062499998829,
9.5594902125713));
#286053=CARTESIAN_POINT('Ctrl Pts',(-2.89974758850909E-14,32.0562499998822,
10.5687124469213));
#286054=CARTESIAN_POINT('Ctrl Pts',(3.10606665601008,32.2062499998816,9.5594902125713));
#286055=CARTESIAN_POINT('Ctrl Pts',(6.21213331202019,32.3562499998811,8.55026797822134));
#286056=CARTESIAN_POINT('Ctrl Pts',(8.13178807675716,32.5062499998805,5.90808986649102));
#286057=CARTESIAN_POINT('Ctrl Pts',(10.0514428414941,32.6562499998798,3.2659117547607));
#286058=CARTESIAN_POINT('Ctrl Pts',(10.0514428414941,32.8062499998793,-1.23094673026484E-15));
#286059=CARTESIAN_POINT('Ctrl Pts',(10.0514428414941,32.9562499998787,-3.26591175476071));
#286060=CARTESIAN_POINT('Ctrl Pts',(8.13178807675716,33.1062499998781,-5.90808986649102));
#286061=CARTESIAN_POINT('Ctrl Pts',(6.21213331202019,33.2562499998775,-8.55026797822134));
#286062=CARTESIAN_POINT('Ctrl Pts',(3.10606665601008,33.4062499998769,-9.5594902125713));
#286063=CARTESIAN_POINT('Ctrl Pts',(-3.2449918494768E-14,33.5562499998763,
-10.5687124469213));
#286064=CARTESIAN_POINT('Ctrl Pts',(-3.10606665601014,33.7062499998756,
-9.5594902125713));
#286065=CARTESIAN_POINT('Ctrl Pts',(-6.21213331202025,33.8562499998751,
-8.55026797822134));
#286066=CARTESIAN_POINT('Ctrl Pts',(-8.13178807675722,34.0062499998744,
-5.90808986649102));
#286067=CARTESIAN_POINT('Ctrl Pts',(-10.0514428414942,34.1562499998739,
-3.2659117547607));
#286068=CARTESIAN_POINT('Ctrl Pts',(-10.0514428414942,34.3062499998732,
2.46189346052968E-15));
#286069=CARTESIAN_POINT('Ctrl Pts',(-10.0514428414942,34.4562499998727,
3.26591175476071));
#286070=CARTESIAN_POINT('Ctrl Pts',(-8.13178807675722,34.606249999872,5.90808986649102));
#286071=CARTESIAN_POINT('Ctrl Pts',(-6.21213331202024,34.7562499998715,
8.55026797822134));
#286072=CARTESIAN_POINT('Ctrl Pts',(-3.10606665601014,34.9062499998708,
9.5594902125713));
#286073=CARTESIAN_POINT('Ctrl Pts',(-3.07251851567527E-14,35.0562499998703,
10.5687124469213));
#286074=CARTESIAN_POINT('Ctrl Pts',(3.10606665601008,35.2062499998697,9.5594902125713));
#286075=CARTESIAN_POINT('Ctrl Pts',(6.21213331202019,35.3562499998691,8.55026797822134));
#286076=CARTESIAN_POINT('Ctrl Pts',(8.13178807675716,35.5062499998685,5.90808986649102));
#286077=CARTESIAN_POINT('Ctrl Pts',(10.0514428414941,35.6562499998679,3.2659117547607));
#286078=CARTESIAN_POINT('Ctrl Pts',(10.0514428414941,35.8062499998673,-1.23094673026484E-15));
#286079=CARTESIAN_POINT('Ctrl Pts',(10.0514428414941,35.9562499998667,-3.26591175476071));
#286080=CARTESIAN_POINT('Ctrl Pts',(8.13178807675716,36.1062499998661,-5.90808986649102));
#286081=CARTESIAN_POINT('Ctrl Pts',(6.21213331202018,36.2562499998655,-8.55026797822134));
#286082=CARTESIAN_POINT('Ctrl Pts',(3.10606665601007,36.4062499998649,-9.5594902125713));
#286083=CARTESIAN_POINT('Ctrl Pts',(-3.41776277664299E-14,36.5562499998642,
-10.5687124469213));
#286084=CARTESIAN_POINT('Ctrl Pts',(-3.10606665601014,36.7062499998636,
-9.5594902125713));
#286085=CARTESIAN_POINT('Ctrl Pts',(-6.21213331202025,36.856249999863,-8.55026797822134));
#286086=CARTESIAN_POINT('Ctrl Pts',(-8.13178807675722,37.0062499998624,
-5.90808986649102));
#286087=CARTESIAN_POINT('Ctrl Pts',(-10.0514428414942,37.1562499998618,
-3.2659117547607));
#286088=CARTESIAN_POINT('Ctrl Pts',(-10.0514428414942,37.3062499998613,
2.46189346052968E-15));
#286089=CARTESIAN_POINT('Ctrl Pts',(-10.0514428414942,37.4562499998606,
3.26591175476071));
#286090=CARTESIAN_POINT('Ctrl Pts',(-8.13178807675722,37.60624999986,5.90808986649102));
#286091=CARTESIAN_POINT('Ctrl Pts',(-6.21213331202025,37.7562499998594,
8.55026797822134));
#286092=CARTESIAN_POINT('Ctrl Pts',(-3.10606665601014,37.9062499998588,
9.5594902125713));
#286093=CARTESIAN_POINT('Ctrl Pts',(-3.24528944284146E-14,38.0562499998583,
10.5687124469213));
#286094=CARTESIAN_POINT('Ctrl Pts',(3.10606665601007,38.2062499998577,9.5594902125713));
#286095=CARTESIAN_POINT('Ctrl Pts',(6.21213331202018,38.3562499998571,8.55026797822134));
#286096=CARTESIAN_POINT('Ctrl Pts',(8.13178807675716,38.5062499998565,5.90808986649102));
#286097=CARTESIAN_POINT('Ctrl Pts',(10.0514428414941,38.6562499998559,3.2659117547607));
#286098=CARTESIAN_POINT('Ctrl Pts',(10.0514428414941,38.8062499998553,-1.23094673026484E-15));
#286099=CARTESIAN_POINT('Ctrl Pts',(10.0514428414941,38.9562499998547,-3.26591175476071));
#286100=CARTESIAN_POINT('Ctrl Pts',(8.13178807675715,39.1062499998541,-5.90808986649102));
#286101=CARTESIAN_POINT('Ctrl Pts',(6.21213331202018,39.2562499998535,-8.55026797822134));
#286102=CARTESIAN_POINT('Ctrl Pts',(3.10606665601007,39.4062499998529,-9.5594902125713));
#286103=CARTESIAN_POINT('Ctrl Pts',(-3.59053370380917E-14,39.5562499998523,
-10.5687124469213));
#286104=CARTESIAN_POINT('Ctrl Pts',(-3.10606665601014,39.7062499998516,
-9.5594902125713));
#286105=CARTESIAN_POINT('Ctrl Pts',(-6.21213331202025,39.856249999851,-8.55026797822134));
#286106=CARTESIAN_POINT('Ctrl Pts',(-8.13178807675723,40.0062499998505,
-5.90808986649102));
#286107=CARTESIAN_POINT('Ctrl Pts',(-10.0514428414942,40.1562499998499,
-3.2659117547607));
#286108=CARTESIAN_POINT('Ctrl Pts',(-10.0514428414942,40.3062499998493,
2.46189346052968E-15));
#286109=CARTESIAN_POINT('Ctrl Pts',(-10.0514428414942,40.4562499998487,
3.26591175476071));
#286110=CARTESIAN_POINT('Ctrl Pts',(-8.13178807675723,40.606249999848,5.90808986649102));
#286111=CARTESIAN_POINT('Ctrl Pts',(-6.21213331202025,40.7562499998475,
8.55026797822134));
#286112=CARTESIAN_POINT('Ctrl Pts',(-3.10606665601014,40.9062499998468,
9.5594902125713));
#286113=CARTESIAN_POINT('Ctrl Pts',(-3.41806037000764E-14,41.0562499998463,
10.5687124469213));
#286114=CARTESIAN_POINT('Ctrl Pts',(3.10606665601007,41.2062499998457,9.5594902125713));
#286115=CARTESIAN_POINT('Ctrl Pts',(6.21213331202018,41.3562499998451,8.55026797822134));
#286116=CARTESIAN_POINT('Ctrl Pts',(8.13178807675715,41.5062499998444,5.90808986649102));
#286117=CARTESIAN_POINT('Ctrl Pts',(10.0514428414941,41.6562499998439,3.2659117547607));
#286118=CARTESIAN_POINT('Ctrl Pts',(10.0514428414941,41.8062499998433,-1.23094673026484E-15));
#286119=CARTESIAN_POINT('Ctrl Pts',(10.0514428414941,41.9562499998427,-3.26591175476071));
#286120=CARTESIAN_POINT('Ctrl Pts',(8.13178807675715,42.1062499998421,-5.90808986649102));
#286121=CARTESIAN_POINT('Ctrl Pts',(6.21213331202018,42.2562499998414,-8.55026797822134));
#286122=CARTESIAN_POINT('Ctrl Pts',(3.10606665601007,42.4062499998408,-9.5594902125713));
#286123=CARTESIAN_POINT('Ctrl Pts',(-3.76330463097535E-14,42.5562499998402,
-10.5687124469213));
#286124=CARTESIAN_POINT('Ctrl Pts',(-3.10606665601015,42.7062499998396,
-9.5594902125713));
#286125=CARTESIAN_POINT('Ctrl Pts',(-6.21213331202025,42.8562499998391,
-8.55026797822134));
#286126=CARTESIAN_POINT('Ctrl Pts',(-8.13178807675723,43.0062499998385,
-5.90808986649102));
#286127=CARTESIAN_POINT('Ctrl Pts',(-10.0514428414942,43.1562499998379,
-3.2659117547607));
#286128=CARTESIAN_POINT('Ctrl Pts',(-10.0514428414942,43.3062499998373,
2.46189346052968E-15));
#286129=CARTESIAN_POINT('Ctrl Pts',(-10.0514428414942,43.4562499998366,
3.26591175476071));
#286130=CARTESIAN_POINT('Ctrl Pts',(-8.13178807675723,43.6062499998361,
5.90808986649102));
#286131=CARTESIAN_POINT('Ctrl Pts',(-6.21213331202025,43.7562499998354,
8.55026797822134));
#286132=CARTESIAN_POINT('Ctrl Pts',(-3.10606665601014,43.9062499998348,
9.5594902125713));
#286133=CARTESIAN_POINT('Ctrl Pts',(-3.59083129717383E-14,44.0562499998343,
10.5687124469213));
#286134=CARTESIAN_POINT('Ctrl Pts',(3.10606665601007,44.2062499998337,9.5594902125713));
#286135=CARTESIAN_POINT('Ctrl Pts',(6.21213331202018,44.3562499998331,8.55026797822134));
#286136=CARTESIAN_POINT('Ctrl Pts',(8.13178807675715,44.5062499998324,5.90808986649102));
#286137=CARTESIAN_POINT('Ctrl Pts',(10.0514428414941,44.6562499998319,3.2659117547607));
#286138=CARTESIAN_POINT('Ctrl Pts',(10.0514428414941,44.8062499998313,-1.23094673026484E-15));
#286139=CARTESIAN_POINT('Ctrl Pts',(10.0514428414941,44.9562499998307,-3.26591175476071));
#286140=CARTESIAN_POINT('Ctrl Pts',(8.13178807675715,45.1062499998301,-5.90808986649102));
#286141=CARTESIAN_POINT('Ctrl Pts',(6.21213331202018,45.2562499998295,-8.55026797822134));
#286142=CARTESIAN_POINT('Ctrl Pts',(3.10606665601007,45.4062499998289,-9.5594902125713));
#286143=CARTESIAN_POINT('Ctrl Pts',(-3.93607555814154E-14,45.5562499998283,
-10.5687124469213));
#286144=CARTESIAN_POINT('Ctrl Pts',(-3.10606665601015,45.7062499998276,
-9.5594902125713));
#286145=CARTESIAN_POINT('Ctrl Pts',(-6.21213331202026,45.856249999827,-8.55026797822134));
#286146=CARTESIAN_POINT('Ctrl Pts',(-8.13178807675723,46.0062499998265,
-5.90808986649102));
#286147=CARTESIAN_POINT('Ctrl Pts',(-10.0514428414942,46.1562499998259,
-3.2659117547607));
#286148=CARTESIAN_POINT('Ctrl Pts',(-10.0514428414942,46.3062499998252,
2.46189346052968E-15));
#286149=CARTESIAN_POINT('Ctrl Pts',(-10.0514428414942,46.4562499998247,
3.26591175476071));
#286150=CARTESIAN_POINT('Ctrl Pts',(-8.13178807675723,46.606249999824,5.90808986649102));
#286151=CARTESIAN_POINT('Ctrl Pts',(-6.21213331202025,46.7562499998235,
8.55026797822134));
#286152=CARTESIAN_POINT('Ctrl Pts',(-3.10606665601015,46.9062499998228,
9.5594902125713));
#286153=CARTESIAN_POINT('Ctrl Pts',(-3.76360222434001E-14,47.0562499998223,
10.5687124469213));
#286154=CARTESIAN_POINT('Ctrl Pts',(3.10606665601007,47.2062499998217,9.5594902125713));
#286155=CARTESIAN_POINT('Ctrl Pts',(6.21213331202018,47.3562499998211,8.55026797822134));
#286156=CARTESIAN_POINT('Ctrl Pts',(8.13178807675715,47.5062499998204,5.90808986649102));
#286157=CARTESIAN_POINT('Ctrl Pts',(10.0514428414941,47.6562499998198,3.2659117547607));
#286158=CARTESIAN_POINT('Ctrl Pts',(10.0514428414941,47.8062499998193,-1.23094673026484E-15));
#286159=CARTESIAN_POINT('Ctrl Pts',(10.0514428414941,47.9562499998186,-3.26591175476071));
#286160=CARTESIAN_POINT('Ctrl Pts',(8.13178807675715,48.1062499998181,-5.90808986649102));
#286161=CARTESIAN_POINT('Ctrl Pts',(6.21213331202017,48.2562499998174,-8.55026797822134));
#286162=CARTESIAN_POINT('Ctrl Pts',(3.10606665601007,48.4062499998169,-9.5594902125713));
#286163=CARTESIAN_POINT('Ctrl Pts',(-4.10884648530772E-14,48.5562499998163,
-10.5687124469213));
#286164=CARTESIAN_POINT('Ctrl Pts',(-3.10606665601015,48.7062499998157,
-9.5594902125713));
#286165=CARTESIAN_POINT('Ctrl Pts',(-6.21213331202026,48.8562499998151,
-8.55026797822134));
#286166=CARTESIAN_POINT('Ctrl Pts',(-8.13178807675723,49.0062499998145,
-5.90808986649102));
#286167=CARTESIAN_POINT('Ctrl Pts',(-10.0514428414942,49.1562499998138,
-3.2659117547607));
#286168=CARTESIAN_POINT('Ctrl Pts',(-10.0514428414942,49.3062499998132,
2.46189346052968E-15));
#286169=CARTESIAN_POINT('Ctrl Pts',(-10.0514428414942,49.4562499998126,
3.26591175476071));
#286170=CARTESIAN_POINT('Ctrl Pts',(-8.13178807675723,49.6062499998121,
5.90808986649102));
#286171=CARTESIAN_POINT('Ctrl Pts',(-6.21213331202026,49.7562499998114,
8.55026797822134));
#286172=CARTESIAN_POINT('Ctrl Pts',(-3.10606665601015,49.9062499998109,
9.5594902125713));
#286173=CARTESIAN_POINT('Ctrl Pts',(-3.9363731515062E-14,50.0562499998103,
10.5687124469213));
#286174=CARTESIAN_POINT('Ctrl Pts',(3.10606665601007,50.2062499998097,9.5594902125713));
#286175=CARTESIAN_POINT('Ctrl Pts',(6.21213331202017,50.3562499998091,8.55026797822134));
#286176=CARTESIAN_POINT('Ctrl Pts',(8.13178807675715,50.5062499998085,5.90808986649102));
#286177=CARTESIAN_POINT('Ctrl Pts',(10.0514428414941,50.6562499998078,3.2659117547607));
#286178=CARTESIAN_POINT('Ctrl Pts',(10.0514428414941,50.8062499998072,-1.23094673026484E-15));
#286179=CARTESIAN_POINT('Ctrl Pts',(10.0514428414941,50.9562499998067,-3.26591175476071));
#286180=CARTESIAN_POINT('Ctrl Pts',(8.13178807675715,51.1062499998061,-5.90808986649102));
#286181=CARTESIAN_POINT('Ctrl Pts',(6.21213331202017,51.2562499998055,-8.55026797822134));
#286182=CARTESIAN_POINT('Ctrl Pts',(3.10606665601006,51.4062499998048,-9.5594902125713));
#286183=CARTESIAN_POINT('Ctrl Pts',(-4.2816174124739E-14,51.5562499998043,
-10.5687124469213));
#286184=CARTESIAN_POINT('Ctrl Pts',(-3.10606665601015,51.7062499998037,
-9.5594902125713));
#286185=CARTESIAN_POINT('Ctrl Pts',(-6.21213331202026,51.856249999803,-8.55026797822134));
#286186=CARTESIAN_POINT('Ctrl Pts',(-8.13178807675723,52.0062499998025,
-5.90808986649102));
#286187=CARTESIAN_POINT('Ctrl Pts',(-10.0514428414942,52.1562499998019,
-3.2659117547607));
#286188=CARTESIAN_POINT('Ctrl Pts',(-10.0514428414942,52.3062499998012,
2.46189346052968E-15));
#286189=CARTESIAN_POINT('Ctrl Pts',(-10.0514428414942,52.4562499998006,
3.26591175476071));
#286190=CARTESIAN_POINT('Ctrl Pts',(-8.13178807675723,52.6062499998,5.90808986649102));
#286191=CARTESIAN_POINT('Ctrl Pts',(-6.21213331202026,52.7562499997994,
8.55026797822134));
#286192=CARTESIAN_POINT('Ctrl Pts',(-3.10606665601015,52.9062499997988,
9.5594902125713));
#286193=CARTESIAN_POINT('Ctrl Pts',(-4.10914407867238E-14,53.0562499997983,
10.5687124469213));
#286194=CARTESIAN_POINT('Ctrl Pts',(3.10606665601007,53.2062499997976,9.5594902125713));
#286195=CARTESIAN_POINT('Ctrl Pts',(6.21213331202017,53.3562499997971,8.55026797822134));
#286196=CARTESIAN_POINT('Ctrl Pts',(8.13178807675715,53.5062499997965,5.90808986649102));
#286197=CARTESIAN_POINT('Ctrl Pts',(10.0514428414941,53.6562499997959,3.2659117547607));
#286198=CARTESIAN_POINT('Ctrl Pts',(10.0514428414941,53.8062499997953,-1.23094673026484E-15));
#286199=CARTESIAN_POINT('Ctrl Pts',(10.0514428414941,53.9562499997946,-3.26591175476071));
#286200=CARTESIAN_POINT('Ctrl Pts',(8.13178807675714,54.106249999794,-5.90808986649102));
#286201=CARTESIAN_POINT('Ctrl Pts',(6.21213331202017,54.2562499997934,-8.55026797822134));
#286202=CARTESIAN_POINT('Ctrl Pts',(3.10606665601006,54.4062499997928,-9.5594902125713));
#286203=CARTESIAN_POINT('Ctrl Pts',(-4.45438833964009E-14,54.5562499997923,
-10.5687124469213));
#286204=CARTESIAN_POINT('Ctrl Pts',(-3.10606665601015,54.7062499997917,
-9.5594902125713));
#286205=CARTESIAN_POINT('Ctrl Pts',(-6.21213331202026,54.856249999791,-8.55026797822134));
#286206=CARTESIAN_POINT('Ctrl Pts',(-8.13178807675724,55.0062499997905,
-5.90808986649102));
#286207=CARTESIAN_POINT('Ctrl Pts',(-10.0514428414942,55.1562499997898,
-3.2659117547607));
#286208=CARTESIAN_POINT('Ctrl Pts',(-10.0514428414942,55.3062499997893,
2.46189346052968E-15));
#286209=CARTESIAN_POINT('Ctrl Pts',(-10.0514428414942,55.4562499997886,
3.26591175476071));
#286210=CARTESIAN_POINT('Ctrl Pts',(-8.13178807675724,55.606249999788,5.90808986649102));
#286211=CARTESIAN_POINT('Ctrl Pts',(-6.21213331202026,55.7562499997874,
8.55026797822134));
#286212=CARTESIAN_POINT('Ctrl Pts',(-3.10606665601015,55.9062499997869,
9.5594902125713));
#286213=CARTESIAN_POINT('Ctrl Pts',(-4.28191500583856E-14,56.0562499997862,
10.5687124469213));
#286214=CARTESIAN_POINT('Ctrl Pts',(3.10606665601006,56.2062499997857,9.5594902125713));
#286215=CARTESIAN_POINT('Ctrl Pts',(6.21213331202017,56.356249999785,8.55026797822134));
#286216=CARTESIAN_POINT('Ctrl Pts',(8.13178807675714,56.5062499997845,5.90808986649102));
#286217=CARTESIAN_POINT('Ctrl Pts',(10.0514428414941,56.6562499997839,3.2659117547607));
#286218=CARTESIAN_POINT('Ctrl Pts',(10.0514428414941,56.8062499997833,-1.23094673026484E-15));
#286219=CARTESIAN_POINT('Ctrl Pts',(10.0514428414941,56.9562499997827,-3.26591175476071));
#286220=CARTESIAN_POINT('Ctrl Pts',(8.13178807675714,57.1062499997821,-5.90808986649102));
#286221=CARTESIAN_POINT('Ctrl Pts',(6.21213331202017,57.2562499997814,-8.55026797822134));
#286222=CARTESIAN_POINT('Ctrl Pts',(3.10606665601006,57.4062499997808,-9.5594902125713));
#286223=CARTESIAN_POINT('Ctrl Pts',(-4.62715926680627E-14,57.5562499997802,
-10.5687124469213));
#286224=CARTESIAN_POINT('Ctrl Pts',(-3.10606665601015,57.7062499997797,
-9.5594902125713));
#286225=CARTESIAN_POINT('Ctrl Pts',(-6.21213331202026,57.856249999779,-8.55026797822134));
#286226=CARTESIAN_POINT('Ctrl Pts',(-8.13178807675724,58.0062499997784,
-5.90808986649102));
#286227=CARTESIAN_POINT('Ctrl Pts',(-10.0514428414942,58.1562499997778,
-3.2659117547607));
#286228=CARTESIAN_POINT('Ctrl Pts',(-10.0514428414942,58.3062499997773,
2.46189346052968E-15));
#286229=CARTESIAN_POINT('Ctrl Pts',(-10.0514428414942,58.4562499997766,
3.26591175476071));
#286230=CARTESIAN_POINT('Ctrl Pts',(-8.13178807675724,58.6062499997761,
5.90808986649102));
#286231=CARTESIAN_POINT('Ctrl Pts',(-6.21213331202026,58.7562499997754,
8.55026797822134));
#286232=CARTESIAN_POINT('Ctrl Pts',(-3.10606665601015,58.9062499997749,
9.5594902125713));
#286233=CARTESIAN_POINT('Ctrl Pts',(-4.45468593300475E-14,59.0562499997743,
10.5687124469213));
#286234=CARTESIAN_POINT('Ctrl Pts',(3.10606665601006,59.2062499997736,9.5594902125713));
#286235=CARTESIAN_POINT('Ctrl Pts',(6.21213331202017,59.356249999773,8.55026797822134));
#286236=CARTESIAN_POINT('Ctrl Pts',(8.13178807675714,59.5062499997725,5.90808986649102));
#286237=CARTESIAN_POINT('Ctrl Pts',(10.0514428414941,59.6562499997718,3.2659117547607));
#286238=CARTESIAN_POINT('Ctrl Pts',(10.0514428414941,59.8062499997713,-1.23094673026484E-15));
#286239=CARTESIAN_POINT('Ctrl Pts',(10.0514428414941,59.9562499997706,-3.26591175476071));
#286240=CARTESIAN_POINT('Ctrl Pts',(8.13178807675714,60.10624999977,-5.90808986649102));
#286241=CARTESIAN_POINT('Ctrl Pts',(6.21213331202017,60.2562499997694,-8.55026797822134));
#286242=CARTESIAN_POINT('Ctrl Pts',(3.10606665601006,60.4062499997689,-9.5594902125713));
#286243=CARTESIAN_POINT('Ctrl Pts',(-4.79993019397246E-14,60.5562499997682,
-10.5687124469213));
#286244=CARTESIAN_POINT('Ctrl Pts',(-3.10606665601016,60.7062499997676,
-9.5594902125713));
#286245=CARTESIAN_POINT('Ctrl Pts',(-6.21213331202026,60.856249999767,-8.55026797822134));
#286246=CARTESIAN_POINT('Ctrl Pts',(-8.13178807675724,61.0062499997664,
-5.90808986649102));
#286247=CARTESIAN_POINT('Ctrl Pts',(-10.0514428414942,61.1562499997658,
-3.2659117547607));
#286248=CARTESIAN_POINT('Ctrl Pts',(-10.0514428414942,61.3062499997652,
2.46189346052968E-15));
#286249=CARTESIAN_POINT('Ctrl Pts',(-10.0514428414942,61.4562499997646,
3.26591175476071));
#286250=CARTESIAN_POINT('Ctrl Pts',(-8.13178807675724,61.6062499997641,
5.90808986649102));
#286251=CARTESIAN_POINT('Ctrl Pts',(-6.21213331202026,61.7562499997634,
8.55026797822134));
#286252=CARTESIAN_POINT('Ctrl Pts',(-3.10606665601015,61.9062499997628,
9.5594902125713));
#286253=CARTESIAN_POINT('Ctrl Pts',(-4.62745686017093E-14,62.0562499997622,
10.5687124469213));
#286254=CARTESIAN_POINT('Ctrl Pts',(3.10606665601006,62.2062499997617,9.5594902125713));
#286255=CARTESIAN_POINT('Ctrl Pts',(6.21213331202017,62.356249999761,8.55026797822134));
#286256=CARTESIAN_POINT('Ctrl Pts',(8.13178807675714,62.5062499997605,5.90808986649102));
#286257=CARTESIAN_POINT('Ctrl Pts',(10.0514428414941,62.6562499997599,3.2659117547607));
#286258=CARTESIAN_POINT('Ctrl Pts',(10.0514428414941,62.8062499997593,-1.23094673026484E-15));
#286259=CARTESIAN_POINT('Ctrl Pts',(10.0514428414941,62.9562499997587,-3.26591175476071));
#286260=CARTESIAN_POINT('Ctrl Pts',(8.13178807675714,63.1062499997581,-5.90808986649102));
#286261=CARTESIAN_POINT('Ctrl Pts',(6.21213331202017,63.2562499997575,-8.55026797822134));
#286262=CARTESIAN_POINT('Ctrl Pts',(3.10606665601006,63.4062499997568,-9.5594902125713));
#286263=CARTESIAN_POINT('Ctrl Pts',(-4.97270112113864E-14,63.5562499997562,
-10.5687124469213));
#286264=CARTESIAN_POINT('Ctrl Pts',(-3.10606665601016,63.7062499997556,
-9.5594902125713));
#286265=CARTESIAN_POINT('Ctrl Pts',(-6.21213331202027,63.8562499997551,
-8.55026797822134));
#286266=CARTESIAN_POINT('Ctrl Pts',(-8.13178807675724,64.0062499997544,
-5.90808986649102));
#286267=CARTESIAN_POINT('Ctrl Pts',(-10.0514428414942,64.1562499997538,
-3.2659117547607));
#286268=CARTESIAN_POINT('Ctrl Pts',(-10.0514428414942,64.3062499997532,
2.46189346052968E-15));
#286269=CARTESIAN_POINT('Ctrl Pts',(-10.0514428414942,64.4562499997526,
3.26591175476071));
#286270=CARTESIAN_POINT('Ctrl Pts',(-8.13178807675724,64.606249999752,5.90808986649102));
#286271=CARTESIAN_POINT('Ctrl Pts',(-6.21213331202026,64.7562499997514,
8.55026797822134));
#286272=CARTESIAN_POINT('Ctrl Pts',(-3.10606665601016,64.9062499997509,
9.5594902125713));
#286273=CARTESIAN_POINT('Ctrl Pts',(-4.80022778733711E-14,65.0562499997502,
10.5687124469213));
#286274=CARTESIAN_POINT('Ctrl Pts',(3.10606665601006,65.2062499997497,9.5594902125713));
#286275=CARTESIAN_POINT('Ctrl Pts',(6.21213331202017,65.3562499997491,8.55026797822134));
#286276=CARTESIAN_POINT('Ctrl Pts',(8.13178807675714,65.5062499997484,5.90808986649102));
#286277=CARTESIAN_POINT('Ctrl Pts',(10.0514428414941,65.6562499997479,3.2659117547607));
#286278=CARTESIAN_POINT('Ctrl Pts',(10.0514428414941,65.8062499997473,-1.23094673026484E-15));
#286279=CARTESIAN_POINT('Ctrl Pts',(10.0514428414941,65.9562499997467,-3.26591175476071));
#286280=CARTESIAN_POINT('Ctrl Pts',(8.13178807675714,66.1062499997461,-5.90808986649102));
#286281=CARTESIAN_POINT('Ctrl Pts',(6.21213331202016,66.2562499997454,-8.55026797822134));
#286282=CARTESIAN_POINT('Ctrl Pts',(3.10606665601006,66.4062499997449,-9.5594902125713));
#286283=CARTESIAN_POINT('Ctrl Pts',(-5.14547204830482E-14,66.5562499997443,
-10.5687124469213));
#286284=CARTESIAN_POINT('Ctrl Pts',(-3.10606665601016,66.7062499997436,
-9.5594902125713));
#286285=CARTESIAN_POINT('Ctrl Pts',(-6.21213331202027,66.8562499997431,
-8.55026797822134));
#286286=CARTESIAN_POINT('Ctrl Pts',(-8.13178807675724,67.0062499997424,
-5.90808986649102));
#286287=CARTESIAN_POINT('Ctrl Pts',(-10.0514428414942,67.1562499997418,
-3.2659117547607));
#286288=CARTESIAN_POINT('Ctrl Pts',(-10.0514428414942,67.3062499997412,
2.46189346052968E-15));
#286289=CARTESIAN_POINT('Ctrl Pts',(-10.0514428414942,67.4562499997406,
3.26591175476071));
#286290=CARTESIAN_POINT('Ctrl Pts',(-8.13178807675724,67.60624999974,5.90808986649102));
#286291=CARTESIAN_POINT('Ctrl Pts',(-6.21213331202027,67.7562499997395,
8.55026797822134));
#286292=CARTESIAN_POINT('Ctrl Pts',(-3.10606665601016,67.9062499997388,
9.5594902125713));
#286293=CARTESIAN_POINT('Ctrl Pts',(-4.9729987145033E-14,68.0562499997382,
10.5687124469213));
#286294=CARTESIAN_POINT('Ctrl Pts',(3.10606665601006,68.2062499997377,9.5594902125713));
#286295=CARTESIAN_POINT('Ctrl Pts',(6.21213331202017,68.356249999737,8.55026797822134));
#286296=CARTESIAN_POINT('Ctrl Pts',(8.13178807675714,68.5062499997365,5.90808986649102));
#286297=CARTESIAN_POINT('Ctrl Pts',(10.0514428414941,68.6562499997358,3.2659117547607));
#286298=CARTESIAN_POINT('Ctrl Pts',(10.0514428414941,68.8062499997353,-1.23094673026484E-15));
#286299=CARTESIAN_POINT('Ctrl Pts',(10.0514428414941,68.9562499997347,-3.26591175476071));
#286300=CARTESIAN_POINT('Ctrl Pts',(8.13178807675714,69.1062499997341,-5.90808986649102));
#286301=CARTESIAN_POINT('Ctrl Pts',(6.21213331202016,69.2562499997335,-8.55026797822134));
#286302=CARTESIAN_POINT('Ctrl Pts',(3.10606665601005,69.4062499997329,-9.5594902125713));
#286303=CARTESIAN_POINT('Ctrl Pts',(-5.31824297547101E-14,69.5562499997323,
-10.5687124469213));
#286304=CARTESIAN_POINT('Ctrl Pts',(-3.10606665601016,69.7062499997317,
-9.5594902125713));
#286305=CARTESIAN_POINT('Ctrl Pts',(-6.21213331202027,69.856249999731,-8.55026797822134));
#286306=CARTESIAN_POINT('Ctrl Pts',(-8.13178807675724,70.0062499997304,
-5.90808986649102));
#286307=CARTESIAN_POINT('Ctrl Pts',(-10.0514428414942,70.1562499997298,
-3.2659117547607));
#286308=CARTESIAN_POINT('Ctrl Pts',(-10.0514428414942,70.3062499997292,
2.46189346052968E-15));
#286309=CARTESIAN_POINT('Ctrl Pts',(-10.0514428414942,70.4562499997286,
3.26591175476071));
#286310=CARTESIAN_POINT('Ctrl Pts',(-8.13178807675724,70.606249999728,5.90808986649102));
#286311=CARTESIAN_POINT('Ctrl Pts',(-6.21213331202027,70.7562499997274,
8.55026797822134));
#286312=CARTESIAN_POINT('Ctrl Pts',(-3.10606665601016,70.9062499997269,
9.5594902125713));
#286313=CARTESIAN_POINT('Ctrl Pts',(-5.14576964166948E-14,71.0562499997262,
10.5687124469213));
#286314=CARTESIAN_POINT('Ctrl Pts',(3.10606665601006,71.2062499997256,9.5594902125713));
#286315=CARTESIAN_POINT('Ctrl Pts',(6.21213331202016,71.3562499997251,8.55026797822134));
#286316=CARTESIAN_POINT('Ctrl Pts',(8.13178807675714,71.5062499997244,5.90808986649102));
#286317=CARTESIAN_POINT('Ctrl Pts',(10.0514428414941,71.6562499997239,3.2659117547607));
#286318=CARTESIAN_POINT('Ctrl Pts',(10.0514428414941,71.8062499997232,-1.23094673026484E-15));
#286319=CARTESIAN_POINT('Ctrl Pts',(10.0514428414941,71.9562499997227,-3.26591175476071));
#286320=CARTESIAN_POINT('Ctrl Pts',(8.13178807675713,72.1062499997221,-5.90808986649102));
#286321=CARTESIAN_POINT('Ctrl Pts',(6.21213331202016,72.2562499997215,-8.55026797822134));
#286322=CARTESIAN_POINT('Ctrl Pts',(3.10606665601005,72.4062499997209,-9.5594902125713));
#286323=CARTESIAN_POINT('Ctrl Pts',(-5.49101390263719E-14,72.5562499997203,
-10.5687124469213));
#286324=CARTESIAN_POINT('Ctrl Pts',(-3.10606665601016,72.7062499997197,
-9.5594902125713));
#286325=CARTESIAN_POINT('Ctrl Pts',(-6.21213331202027,72.8562499997191,
-8.55026797822134));
#286326=CARTESIAN_POINT('Ctrl Pts',(-8.13178807675725,73.0062499997184,
-5.90808986649102));
#286327=CARTESIAN_POINT('Ctrl Pts',(-10.0514428414942,73.1562499997178,
-3.2659117547607));
#286328=CARTESIAN_POINT('Ctrl Pts',(-10.0514428414942,73.3062499997172,
2.46189346052968E-15));
#286329=CARTESIAN_POINT('Ctrl Pts',(-10.0514428414942,73.4562499997166,
3.26591175476071));
#286330=CARTESIAN_POINT('Ctrl Pts',(-8.13178807675725,73.606249999716,5.90808986649102));
#286331=CARTESIAN_POINT('Ctrl Pts',(-6.21213331202027,73.7562499997155,
8.55026797822134));
#286332=CARTESIAN_POINT('Ctrl Pts',(-3.10606665601016,73.9062499997148,
9.5594902125713));
#286333=CARTESIAN_POINT('Ctrl Pts',(-5.31854056883567E-14,74.0562499997143,
10.5687124469213));
#286334=CARTESIAN_POINT('Ctrl Pts',(3.10606665601005,74.2062499997136,9.5594902125713));
#286335=CARTESIAN_POINT('Ctrl Pts',(6.21213331202016,74.3562499997131,8.55026797822134));
#286336=CARTESIAN_POINT('Ctrl Pts',(8.13178807675713,74.5062499997125,5.90808986649102));
#286337=CARTESIAN_POINT('Ctrl Pts',(10.0514428414941,74.6562499997118,3.2659117547607));
#286338=CARTESIAN_POINT('Ctrl Pts',(10.0514428414941,74.8062499997113,-1.23094673026484E-15));
#286339=CARTESIAN_POINT('Ctrl Pts',(10.0514428414941,74.9562499997106,-3.26591175476071));
#286340=CARTESIAN_POINT('Ctrl Pts',(8.13178807675713,75.10624999971,-5.90808986649102));
#286341=CARTESIAN_POINT('Ctrl Pts',(6.21213331202016,75.2562499997094,-8.55026797822134));
#286342=CARTESIAN_POINT('Ctrl Pts',(3.10606665601005,75.4062499997088,-9.5594902125713));
#286343=CARTESIAN_POINT('Ctrl Pts',(-5.66378482980338E-14,75.5562499997083,
-10.5687124469213));
#286344=CARTESIAN_POINT('Ctrl Pts',(-3.10606665601016,75.7062499997077,
-9.5594902125713));
#286345=CARTESIAN_POINT('Ctrl Pts',(-6.21213331202027,75.856249999707,-8.55026797822134));
#286346=CARTESIAN_POINT('Ctrl Pts',(-8.13178807675725,76.0062499997065,
-5.90808986649102));
#286347=CARTESIAN_POINT('Ctrl Pts',(-10.0514428414942,76.1562499997058,
-3.2659117547607));
#286348=CARTESIAN_POINT('Ctrl Pts',(-10.0514428414942,76.3062499997052,
2.46189346052968E-15));
#286349=CARTESIAN_POINT('Ctrl Pts',(-10.0514428414942,76.4562499997046,
3.26591175476071));
#286350=CARTESIAN_POINT('Ctrl Pts',(-8.13178807675725,76.606249999704,5.90808986649102));
#286351=CARTESIAN_POINT('Ctrl Pts',(-6.21213331202027,76.7562499997035,
8.55026797822134));
#286352=CARTESIAN_POINT('Ctrl Pts',(-3.10606665601016,76.9062499997029,
9.5594902125713));
#286353=CARTESIAN_POINT('Ctrl Pts',(-5.49131149600185E-14,77.0562499997022,
10.5687124469213));
#286354=CARTESIAN_POINT('Ctrl Pts',(3.10606665601005,77.2062499997016,9.5594902125713));
#286355=CARTESIAN_POINT('Ctrl Pts',(6.21213331202016,77.356249999701,8.55026797822134));
#286356=CARTESIAN_POINT('Ctrl Pts',(8.13178807675713,77.5062499997004,5.90808986649102));
#286357=CARTESIAN_POINT('Ctrl Pts',(10.0514428414941,77.6562499996998,3.2659117547607));
#286358=CARTESIAN_POINT('Ctrl Pts',(10.0514428414941,77.8062499996992,-1.23094673026484E-15));
#286359=CARTESIAN_POINT('Ctrl Pts',(10.0514428414941,77.9562499996987,-3.26591175476071));
#286360=CARTESIAN_POINT('Ctrl Pts',(8.13178807675713,78.1062499996981,-5.90808986649102));
#286361=CARTESIAN_POINT('Ctrl Pts',(6.21213331202016,78.2562499996974,-8.55026797822134));
#286362=CARTESIAN_POINT('Ctrl Pts',(3.10606665601005,78.4062499996969,-9.5594902125713));
#286363=CARTESIAN_POINT('Ctrl Pts',(-5.83655575696956E-14,78.5562499996963,
-10.5687124469213));
#286364=CARTESIAN_POINT('Ctrl Pts',(-3.10606665601017,78.7062499996957,
-9.5594902125713));
#286365=CARTESIAN_POINT('Ctrl Pts',(-6.21213331202028,78.8562499996951,
-8.55026797822134));
#286366=CARTESIAN_POINT('Ctrl Pts',(-8.13178807675725,79.0062499996944,
-5.90808986649102));
#286367=CARTESIAN_POINT('Ctrl Pts',(-10.0514428414942,79.1562499996939,
-3.2659117547607));
#286368=CARTESIAN_POINT('Ctrl Pts',(-10.0514428414942,79.3062499996932,
2.46189346052968E-15));
#286369=CARTESIAN_POINT('Ctrl Pts',(-10.0514428414942,79.4562499996926,
3.26591175476071));
#286370=CARTESIAN_POINT('Ctrl Pts',(-8.13178807675725,79.606249999692,5.90808986649102));
#286371=CARTESIAN_POINT('Ctrl Pts',(-6.21213331202027,79.7562499996915,
8.55026797822134));
#286372=CARTESIAN_POINT('Ctrl Pts',(-3.10606665601016,79.9062499996908,
9.5594902125713));
#286373=CARTESIAN_POINT('Ctrl Pts',(-5.66408242316803E-14,80.0562499996902,
10.5687124469213));
#286374=CARTESIAN_POINT('Ctrl Pts',(3.10606665601005,80.2062499996896,9.5594902125713));
#286375=CARTESIAN_POINT('Ctrl Pts',(6.21213331202016,80.356249999689,8.55026797822134));
#286376=CARTESIAN_POINT('Ctrl Pts',(8.13178807675713,80.5062499996884,5.90808986649102));
#286377=CARTESIAN_POINT('Ctrl Pts',(10.0514428414941,80.6562499996878,3.2659117547607));
#286378=CARTESIAN_POINT('Ctrl Pts',(10.0514428414941,80.8062499996873,-1.23094673026484E-15));
#286379=CARTESIAN_POINT('Ctrl Pts',(10.0514428414941,80.9562499996866,-3.26591175476071));
#286380=CARTESIAN_POINT('Ctrl Pts',(8.13178807675713,81.1062499996861,-5.90808986649102));
#286381=CARTESIAN_POINT('Ctrl Pts',(6.21213331202016,81.2562499996854,-8.55026797822134));
#286382=CARTESIAN_POINT('Ctrl Pts',(3.10606665601005,81.4062499996849,-9.5594902125713));
#286383=CARTESIAN_POINT('Ctrl Pts',(-6.00932668413574E-14,81.5562499996843,
-10.5687124469213));
#286384=CARTESIAN_POINT('Ctrl Pts',(-3.10606665601017,81.7062499996837,
-9.5594902125713));
#286385=CARTESIAN_POINT('Ctrl Pts',(-6.21213331202028,81.856249999683,-8.55026797822134));
#286386=CARTESIAN_POINT('Ctrl Pts',(-8.13178807675725,82.0062499996824,
-5.90808986649102));
#286387=CARTESIAN_POINT('Ctrl Pts',(-10.0514428414942,82.1562499996818,
-3.2659117547607));
#286388=CARTESIAN_POINT('Ctrl Pts',(-10.0514428414942,82.3062499996813,
2.46189346052968E-15));
#286389=CARTESIAN_POINT('Ctrl Pts',(-10.0514428414942,82.4562499996806,
3.26591175476071));
#286390=CARTESIAN_POINT('Ctrl Pts',(-8.13178807675725,82.60624999968,5.90808986649102));
#286391=CARTESIAN_POINT('Ctrl Pts',(-6.21213331202028,82.7562499996795,
8.55026797822134));
#286392=CARTESIAN_POINT('Ctrl Pts',(-3.10606665601017,82.9062499996789,
9.5594902125713));
#286393=CARTESIAN_POINT('Ctrl Pts',(-5.83685335033422E-14,83.0562499996782,
10.5687124469213));
#286394=CARTESIAN_POINT('Ctrl Pts',(3.10606665601005,83.2062499996776,9.5594902125713));
#286395=CARTESIAN_POINT('Ctrl Pts',(6.21213331202016,83.356249999677,8.55026797822134));
#286396=CARTESIAN_POINT('Ctrl Pts',(8.13178807675713,83.5062499996764,5.90808986649102));
#286397=CARTESIAN_POINT('Ctrl Pts',(10.0514428414941,83.6562499996759,3.2659117547607));
#286398=CARTESIAN_POINT('Ctrl Pts',(10.0514428414941,83.8062499996752,-1.23094673026484E-15));
#286399=CARTESIAN_POINT('Ctrl Pts',(10.0514428414941,83.9562499996747,-3.26591175476071));
#286400=CARTESIAN_POINT('Ctrl Pts',(8.13178807675713,84.106249999674,-5.90808986649102));
#286401=CARTESIAN_POINT('Ctrl Pts',(6.21213331202016,84.2562499996734,-8.55026797822134));
#286402=CARTESIAN_POINT('Ctrl Pts',(3.10606665601005,84.4062499996729,-9.5594902125713));
#286403=CARTESIAN_POINT('Ctrl Pts',(-6.18209761130193E-14,84.5562499996723,
-10.5687124469213));
#286404=CARTESIAN_POINT('Ctrl Pts',(-3.10606665601017,84.7062499996717,
-9.5594902125713));
#286405=CARTESIAN_POINT('Ctrl Pts',(-6.21213331202028,84.856249999671,-8.55026797822134));
#286406=CARTESIAN_POINT('Ctrl Pts',(-8.13178807675725,85.0062499996704,
-5.90808986649102));
#286407=CARTESIAN_POINT('Ctrl Pts',(-10.0514428414942,85.1562499996699,
-3.2659117547607));
#286408=CARTESIAN_POINT('Ctrl Pts',(-10.0514428414942,85.3062499996692,
2.46189346052968E-15));
#286409=CARTESIAN_POINT('Ctrl Pts',(-10.0514428414942,85.4562499996686,
3.26591175476071));
#286410=CARTESIAN_POINT('Ctrl Pts',(-8.13178807675725,85.606249999668,5.90808986649102));
#286411=CARTESIAN_POINT('Ctrl Pts',(-6.21213331202028,85.7562499996675,
8.55026797822134));
#286412=CARTESIAN_POINT('Ctrl Pts',(-3.10606665601017,85.9062499996669,
9.5594902125713));
#286413=CARTESIAN_POINT('Ctrl Pts',(-6.0096242775004E-14,86.0562499996662,
10.5687124469213));
#286414=CARTESIAN_POINT('Ctrl Pts',(3.10606665601005,86.2062499996657,9.5594902125713));
#286415=CARTESIAN_POINT('Ctrl Pts',(6.21213331202016,86.3562499996651,8.55026797822134));
#286416=CARTESIAN_POINT('Ctrl Pts',(8.13178807675713,86.5062499996644,5.90808986649102));
#286417=CARTESIAN_POINT('Ctrl Pts',(10.0514428414941,86.6562499996638,3.2659117547607));
#286418=CARTESIAN_POINT('Ctrl Pts',(10.0514428414941,86.8062499996633,-1.23094673026484E-15));
#286419=CARTESIAN_POINT('Ctrl Pts',(10.0514428414941,86.9562499996626,-3.26591175476071));
#286420=CARTESIAN_POINT('Ctrl Pts',(8.13178807675713,87.1062499996621,-5.90808986649102));
#286421=CARTESIAN_POINT('Ctrl Pts',(6.21213331202015,87.2562499996614,-8.55026797822134));
#286422=CARTESIAN_POINT('Ctrl Pts',(3.10606665601004,87.4062499996609,-9.5594902125713));
#286423=CARTESIAN_POINT('Ctrl Pts',(-6.35486853846811E-14,87.5562499996603,
-10.5687124469213));
#286424=CARTESIAN_POINT('Ctrl Pts',(-3.10606665601017,87.7062499996597,
-9.5594902125713));
#286425=CARTESIAN_POINT('Ctrl Pts',(-6.21213331202028,87.856249999659,-8.55026797822134));
#286426=CARTESIAN_POINT('Ctrl Pts',(-8.13178807675726,88.0062499996585,
-5.90808986649102));
#286427=CARTESIAN_POINT('Ctrl Pts',(-10.0514428414942,88.1562499996578,
-3.2659117547607));
#286428=CARTESIAN_POINT('Ctrl Pts',(-10.0514428414942,88.3062499996572,
2.46189346052968E-15));
#286429=CARTESIAN_POINT('Ctrl Pts',(-10.0514428414942,88.4562499996566,
3.26591175476071));
#286430=CARTESIAN_POINT('Ctrl Pts',(-8.13178807675726,88.6062499996561,
5.90808986649102));
#286431=CARTESIAN_POINT('Ctrl Pts',(-6.21213331202028,88.7562499996555,
8.55026797822134));
#286432=CARTESIAN_POINT('Ctrl Pts',(-3.10606665601017,88.9062499996548,
9.5594902125713));
#286433=CARTESIAN_POINT('Ctrl Pts',(-6.18239520466659E-14,89.0562499996542,
10.5687124469213));
#286434=CARTESIAN_POINT('Ctrl Pts',(3.10606665601005,89.2062499996537,9.5594902125713));
#286435=CARTESIAN_POINT('Ctrl Pts',(6.21213331202016,89.3562499996531,8.55026797822134));
#286436=CARTESIAN_POINT('Ctrl Pts',(8.13178807675713,89.5062499996525,5.90808986649102));
#286437=CARTESIAN_POINT('Ctrl Pts',(10.0514428414941,89.6562499996518,3.2659117547607));
#286438=CARTESIAN_POINT('Ctrl Pts',(10.0514428414941,89.8062499996512,-1.23094673026484E-15));
#286439=CARTESIAN_POINT('Ctrl Pts',(10.0514428414941,89.9562499996507,-3.26591175476071));
#286440=CARTESIAN_POINT('Ctrl Pts',(8.13178807675713,90.10624999965,-5.90808986649102));
#286441=CARTESIAN_POINT('Ctrl Pts',(6.21213331202015,90.2562499996494,-8.55026797822134));
#286442=CARTESIAN_POINT('Ctrl Pts',(3.10606665601004,90.4062499996488,-9.5594902125713));
#286443=CARTESIAN_POINT('Ctrl Pts',(-6.52763946563429E-14,90.5562499996483,
-10.5687124469213));
#286444=CARTESIAN_POINT('Ctrl Pts',(-3.10606665601017,90.7062499996476,
-9.5594902125713));
#286445=CARTESIAN_POINT('Ctrl Pts',(-6.21213331202028,90.856249999647,-8.55026797822134));
#286446=CARTESIAN_POINT('Ctrl Pts',(-8.13178807675726,91.0062499996464,
-5.90808986649102));
#286447=CARTESIAN_POINT('Ctrl Pts',(-10.0514428414942,91.1562499996458,
-3.2659117547607));
#286448=CARTESIAN_POINT('Ctrl Pts',(-10.0514428414942,91.3062499996452,
2.46189346052968E-15));
#286449=CARTESIAN_POINT('Ctrl Pts',(-10.0514428414942,91.4562499996446,
3.26591175476071));
#286450=CARTESIAN_POINT('Ctrl Pts',(-8.13178807675726,91.606249999644,5.90808986649102));
#286451=CARTESIAN_POINT('Ctrl Pts',(-6.21213331202028,91.7562499996434,
8.55026797822134));
#286452=CARTESIAN_POINT('Ctrl Pts',(-3.10606665601017,91.9062499996429,
9.5594902125713));
#286453=CARTESIAN_POINT('Ctrl Pts',(-6.35516613183277E-14,92.0562499996422,
10.5687124469213));
#286454=CARTESIAN_POINT('Ctrl Pts',(3.10606665601004,92.2062499996417,9.5594902125713));
#286455=CARTESIAN_POINT('Ctrl Pts',(6.21213331202015,92.3562499996411,8.55026797822134));
#286456=CARTESIAN_POINT('Ctrl Pts',(8.13178807675712,92.5062499996404,5.90808986649102));
#286457=CARTESIAN_POINT('Ctrl Pts',(10.0514428414941,92.6562499996398,3.2659117547607));
#286458=CARTESIAN_POINT('Ctrl Pts',(10.0514428414941,92.8062499996392,-1.23094673026484E-15));
#286459=CARTESIAN_POINT('Ctrl Pts',(10.0514428414941,92.9562499996387,-3.26591175476071));
#286460=CARTESIAN_POINT('Ctrl Pts',(8.13178807675712,93.1062499996381,-5.90808986649102));
#286461=CARTESIAN_POINT('Ctrl Pts',(6.21213331202015,93.2562499996374,-8.55026797822134));
#286462=CARTESIAN_POINT('Ctrl Pts',(3.10606665601004,93.4062499996369,-9.5594902125713));
#286463=CARTESIAN_POINT('Ctrl Pts',(-6.70041039280048E-14,93.5562499996362,
-10.5687124469213));
#286464=CARTESIAN_POINT('Ctrl Pts',(-3.10606665601018,93.7062499996357,
-9.5594902125713));
#286465=CARTESIAN_POINT('Ctrl Pts',(-6.21213331202028,93.856249999635,-8.55026797822134));
#286466=CARTESIAN_POINT('Ctrl Pts',(-8.13178807675726,94.0062499996344,
-5.90808986649102));
#286467=CARTESIAN_POINT('Ctrl Pts',(-10.0514428414942,94.1562499996338,
-3.2659117547607));
#286468=CARTESIAN_POINT('Ctrl Pts',(-10.0514428414942,94.3062499996333,
2.46189346052968E-15));
#286469=CARTESIAN_POINT('Ctrl Pts',(-10.0514428414942,94.4562499996326,
3.26591175476071));
#286470=CARTESIAN_POINT('Ctrl Pts',(-8.13178807675726,94.606249999632,5.90808986649102));
#286471=CARTESIAN_POINT('Ctrl Pts',(-6.21213331202028,94.7562499996315,
8.55026797822134));
#286472=CARTESIAN_POINT('Ctrl Pts',(-3.10606665601017,94.9062499996309,
9.5594902125713));
#286473=CARTESIAN_POINT('Ctrl Pts',(-6.52793705899895E-14,95.0562499996302,
10.5687124469213));
#286474=CARTESIAN_POINT('Ctrl Pts',(3.10606665601004,95.2062499996296,9.5594902125713));
#286475=CARTESIAN_POINT('Ctrl Pts',(6.21213331202015,95.3562499996291,8.55026797822134));
#286476=CARTESIAN_POINT('Ctrl Pts',(8.13178807675712,95.5062499996285,5.90808986649102));
#286477=CARTESIAN_POINT('Ctrl Pts',(10.0514428414941,95.6562499996278,3.2659117547607));
#286478=CARTESIAN_POINT('Ctrl Pts',(10.0514428414941,95.8062499996273,-1.23094673026484E-15));
#286479=CARTESIAN_POINT('Ctrl Pts',(10.0514428414941,95.9562499996266,-3.26591175476071));
#286480=CARTESIAN_POINT('Ctrl Pts',(8.13178807675712,96.1062499996261,-5.90808986649102));
#286481=CARTESIAN_POINT('Ctrl Pts',(6.21213331202015,96.2562499996255,-8.55026797822134));
#286482=CARTESIAN_POINT('Ctrl Pts',(3.10606665601004,96.4062499996248,-9.5594902125713));
#286483=CARTESIAN_POINT('Ctrl Pts',(-6.87318131996666E-14,96.5562499996243,
-10.5687124469213));
#286484=CARTESIAN_POINT('Ctrl Pts',(-3.10606665601018,96.7062499996236,
-9.5594902125713));
#286485=CARTESIAN_POINT('Ctrl Pts',(-6.21213331202028,96.856249999623,-8.55026797822134));
#286486=CARTESIAN_POINT('Ctrl Pts',(-8.13178807675726,97.0062499996224,
-5.90808986649102));
#286487=CARTESIAN_POINT('Ctrl Pts',(-10.0514428414942,97.1562499996218,
-3.2659117547607));
#286488=CARTESIAN_POINT('Ctrl Pts',(-10.0514428414942,97.3062499996212,
2.46189346052968E-15));
#286489=CARTESIAN_POINT('Ctrl Pts',(-10.0514428414942,97.4562499996206,
3.26591175476071));
#286490=CARTESIAN_POINT('Ctrl Pts',(-8.13178807675726,97.60624999962,5.90808986649102));
#286491=CARTESIAN_POINT('Ctrl Pts',(-6.21213331202028,97.7562499996195,
8.55026797822134));
#286492=CARTESIAN_POINT('Ctrl Pts',(-3.10606665601018,97.9062499996189,
9.5594902125713));
#286493=CARTESIAN_POINT('Ctrl Pts',(-6.70070798616514E-14,98.0562499996182,
10.5687124469213));
#286494=CARTESIAN_POINT('Ctrl Pts',(3.10606665601004,98.2062499996177,9.5594902125713));
#286495=CARTESIAN_POINT('Ctrl Pts',(6.21213331202015,98.3562499996171,8.55026797822134));
#286496=CARTESIAN_POINT('Ctrl Pts',(8.13178807675712,98.5062499996165,5.90808986649102));
#286497=CARTESIAN_POINT('Ctrl Pts',(10.0514428414941,98.6562499996158,3.2659117547607));
#286498=CARTESIAN_POINT('Ctrl Pts',(10.0514428414941,98.8062499996153,-1.23094673026484E-15));
#286499=CARTESIAN_POINT('Ctrl Pts',(10.0514428414941,98.9562499996147,-3.26591175476071));
#286500=CARTESIAN_POINT('Ctrl Pts',(8.13178807675712,99.1062499996141,-5.90808986649102));
#286501=CARTESIAN_POINT('Ctrl Pts',(6.21213331202015,99.2562499996134,-8.55026797822134));
#286502=CARTESIAN_POINT('Ctrl Pts',(3.10606665601004,99.4062499996129,-9.5594902125713));
#286503=CARTESIAN_POINT('Ctrl Pts',(-7.04595224713284E-14,99.5562499996123,
-10.5687124469213));
#286504=CARTESIAN_POINT('Ctrl Pts',(-3.10606665601018,99.7062499996117,
-9.5594902125713));
#286505=CARTESIAN_POINT('Ctrl Pts',(-6.21213331202028,99.856249999611,-8.55026797822134));
#286506=CARTESIAN_POINT('Ctrl Pts',(-8.13178807675726,100.00624999961,-5.90808986649102));
#286507=CARTESIAN_POINT('Ctrl Pts',(-10.0514428414942,100.15624999961,-3.2659117547607));
#286508=CARTESIAN_POINT('Ctrl Pts',(-10.0514428414942,100.306249999609,
2.46189346052968E-15));
#286509=CARTESIAN_POINT('Ctrl Pts',(-10.0514428414942,100.456249999609,
3.26591175476071));
#286510=CARTESIAN_POINT('Ctrl Pts',(-8.13178807675726,100.606249999608,
5.90808986649102));
#286511=CARTESIAN_POINT('Ctrl Pts',(-6.21213331202028,100.756249999607,
8.55026797822134));
#286512=CARTESIAN_POINT('Ctrl Pts',(-3.10606665601018,100.906249999607,
9.5594902125713));
#286513=CARTESIAN_POINT('Ctrl Pts',(-6.87347891333132E-14,101.056249999606,
10.5687124469213));
#286514=CARTESIAN_POINT('Ctrl Pts',(3.10606665601004,101.206249999606,9.5594902125713));
#286515=CARTESIAN_POINT('Ctrl Pts',(6.21213331202015,101.356249999605,8.55026797822134));
#286516=CARTESIAN_POINT('Ctrl Pts',(8.13178807675712,101.506249999604,5.90808986649102));
#286517=CARTESIAN_POINT('Ctrl Pts',(10.0514428414941,101.656249999604,3.2659117547607));
#286518=CARTESIAN_POINT('Ctrl Pts',(10.0514428414941,101.806249999603,-1.23094673026484E-15));
#286519=CARTESIAN_POINT('Ctrl Pts',(10.0514428414941,101.956249999603,-3.26591175476071));
#286520=CARTESIAN_POINT('Ctrl Pts',(8.13178807675712,102.106249999602,-5.90808986649102));
#286521=CARTESIAN_POINT('Ctrl Pts',(6.21213331202014,102.256249999601,-8.55026797822134));
#286522=CARTESIAN_POINT('Ctrl Pts',(3.10606665601004,102.406249999601,-9.5594902125713));
#286523=CARTESIAN_POINT('Ctrl Pts',(-7.21872317429903E-14,102.5562499996,
-10.5687124469213));
#286524=CARTESIAN_POINT('Ctrl Pts',(-3.10606665601018,102.7062499996,-9.5594902125713));
#286525=CARTESIAN_POINT('Ctrl Pts',(-6.21213331202029,102.856249999599,
-8.55026797822134));
#286526=CARTESIAN_POINT('Ctrl Pts',(-8.13178807675726,103.006249999598,
-5.90808986649102));
#286527=CARTESIAN_POINT('Ctrl Pts',(-10.0514428414942,103.156249999598,
-3.2659117547607));
#286528=CARTESIAN_POINT('Ctrl Pts',(-10.0514428414942,103.306249999597,
2.46189346052968E-15));
#286529=CARTESIAN_POINT('Ctrl Pts',(-10.0514428414942,103.456249999597,
3.26591175476071));
#286530=CARTESIAN_POINT('Ctrl Pts',(-8.13178807675726,103.606249999596,
5.90808986649102));
#286531=CARTESIAN_POINT('Ctrl Pts',(-6.21213331202028,103.756249999595,
8.55026797822134));
#286532=CARTESIAN_POINT('Ctrl Pts',(-3.10606665601018,103.906249999595,
9.5594902125713));
#286533=CARTESIAN_POINT('Ctrl Pts',(-7.04624984049751E-14,104.056249999594,
10.5687124469213));
#286534=CARTESIAN_POINT('Ctrl Pts',(3.10606665601004,104.206249999594,9.5594902125713));
#286535=CARTESIAN_POINT('Ctrl Pts',(6.21213331202015,104.356249999593,8.55026797822134));
#286536=CARTESIAN_POINT('Ctrl Pts',(8.13178807675712,104.506249999592,5.90808986649102));
#286537=CARTESIAN_POINT('Ctrl Pts',(10.0514428414941,104.656249999592,3.2659117547607));
#286538=CARTESIAN_POINT('Ctrl Pts',(10.0514428414941,104.806249999591,-1.23094673026484E-15));
#286539=CARTESIAN_POINT('Ctrl Pts',(10.0514428414941,104.956249999591,-3.26591175476071));
#286540=CARTESIAN_POINT('Ctrl Pts',(8.13178807675712,105.10624999959,-5.90808986649102));
#286541=CARTESIAN_POINT('Ctrl Pts',(6.21213331202014,105.256249999589,-8.55026797822134));
#286542=CARTESIAN_POINT('Ctrl Pts',(3.10606665601003,105.406249999589,-9.5594902125713));
#286543=CARTESIAN_POINT('Ctrl Pts',(-7.39149410146522E-14,105.556249999588,
-10.5687124469213));
#286544=CARTESIAN_POINT('Ctrl Pts',(-3.10606665601018,105.706249999588,
-9.5594902125713));
#286545=CARTESIAN_POINT('Ctrl Pts',(-6.21213331202029,105.856249999587,
-8.55026797822134));
#286546=CARTESIAN_POINT('Ctrl Pts',(-8.13178807675726,106.006249999586,
-5.90808986649102));
#286547=CARTESIAN_POINT('Ctrl Pts',(-10.0514428414942,106.156249999586,
-3.2659117547607));
#286548=CARTESIAN_POINT('Ctrl Pts',(-10.0514428414942,106.306249999585,
2.46189346052968E-15));
#286549=CARTESIAN_POINT('Ctrl Pts',(-10.0514428414942,106.456249999585,
3.26591175476071));
#286550=CARTESIAN_POINT('Ctrl Pts',(-8.13178807675726,106.606249999584,
5.90808986649102));
#286551=CARTESIAN_POINT('Ctrl Pts',(-6.21213331202029,106.756249999583,
8.55026797822134));
#286552=CARTESIAN_POINT('Ctrl Pts',(-3.10606665601018,106.906249999583,
9.5594902125713));
#286553=CARTESIAN_POINT('Ctrl Pts',(-7.21902076766369E-14,107.056249999582,
10.5687124469213));
#286554=CARTESIAN_POINT('Ctrl Pts',(3.10606665601003,107.206249999582,9.5594902125713));
#286555=CARTESIAN_POINT('Ctrl Pts',(6.21213331202014,107.356249999581,8.55026797822134));
#286556=CARTESIAN_POINT('Ctrl Pts',(8.13178807675711,107.50624999958,5.90808986649102));
#286557=CARTESIAN_POINT('Ctrl Pts',(10.0514428414941,107.65624999958,3.2659117547607));
#286558=CARTESIAN_POINT('Ctrl Pts',(10.0514428414941,107.806249999579,-1.23094673026484E-15));
#286559=CARTESIAN_POINT('Ctrl Pts',(10.0514428414941,107.956249999579,-3.26591175476071));
#286560=CARTESIAN_POINT('Ctrl Pts',(8.13178807675711,108.106249999578,-5.90808986649102));
#286561=CARTESIAN_POINT('Ctrl Pts',(6.21213331202014,108.256249999577,-8.55026797822134));
#286562=CARTESIAN_POINT('Ctrl Pts',(3.10606665601003,108.406249999577,-9.5594902125713));
#286563=CARTESIAN_POINT('Ctrl Pts',(-7.5642650286314E-14,108.556249999576,
-10.5687124469213));
#286564=CARTESIAN_POINT('Ctrl Pts',(-3.10606665601018,108.706249999576,
-9.5594902125713));
#286565=CARTESIAN_POINT('Ctrl Pts',(-6.21213331202029,108.856249999575,
-8.55026797822134));
#286566=CARTESIAN_POINT('Ctrl Pts',(-8.13178807675727,109.006249999574,
-5.90808986649102));
#286567=CARTESIAN_POINT('Ctrl Pts',(-10.0514428414942,109.156249999574,
-3.2659117547607));
#286568=CARTESIAN_POINT('Ctrl Pts',(-10.0514428414942,109.306249999573,
2.46189346052968E-15));
#286569=CARTESIAN_POINT('Ctrl Pts',(-10.0514428414942,109.456249999573,
3.26591175476071));
#286570=CARTESIAN_POINT('Ctrl Pts',(-8.13178807675727,109.606249999572,
5.90808986649102));
#286571=CARTESIAN_POINT('Ctrl Pts',(-6.21213331202029,109.756249999571,
8.55026797822134));
#286572=CARTESIAN_POINT('Ctrl Pts',(-3.10606665601018,109.906249999571,
9.5594902125713));
#286573=CARTESIAN_POINT('Ctrl Pts',(-7.39179169482987E-14,110.05624999957,
10.5687124469213));
#286574=CARTESIAN_POINT('Ctrl Pts',(3.10606665601003,110.20624999957,9.5594902125713));
#286575=CARTESIAN_POINT('Ctrl Pts',(6.21213331202014,110.356249999569,8.55026797822134));
#286576=CARTESIAN_POINT('Ctrl Pts',(8.13178807675711,110.506249999568,5.90808986649102));
#286577=CARTESIAN_POINT('Ctrl Pts',(10.0514428414941,110.656249999568,3.2659117547607));
#286578=CARTESIAN_POINT('Ctrl Pts',(10.0514428414941,110.806249999567,-1.23094673026484E-15));
#286579=CARTESIAN_POINT('Ctrl Pts',(10.0514428414941,110.956249999567,-3.26591175476071));
#286580=CARTESIAN_POINT('Ctrl Pts',(8.13178807675711,111.106249999566,-5.90808986649102));
#286581=CARTESIAN_POINT('Ctrl Pts',(6.21213331202014,111.256249999565,-8.55026797822134));
#286582=CARTESIAN_POINT('Ctrl Pts',(3.10606665601003,111.406249999565,-9.5594902125713));
#286583=CARTESIAN_POINT('Ctrl Pts',(-7.73703595579758E-14,111.556249999564,
-10.5687124469213));
#286584=CARTESIAN_POINT('Ctrl Pts',(-3.10606665601019,111.706249999564,
-9.5594902125713));
#286585=CARTESIAN_POINT('Ctrl Pts',(-6.21213331202029,111.856249999563,
-8.55026797822134));
#286586=CARTESIAN_POINT('Ctrl Pts',(-8.13178807675727,112.006249999562,
-5.90808986649102));
#286587=CARTESIAN_POINT('Ctrl Pts',(-10.0514428414942,112.156249999562,
-3.2659117547607));
#286588=CARTESIAN_POINT('Ctrl Pts',(-10.0514428414942,112.306249999561,
2.46189346052968E-15));
#286589=CARTESIAN_POINT('Ctrl Pts',(-10.0514428414942,112.456249999561,
3.26591175476071));
#286590=CARTESIAN_POINT('Ctrl Pts',(-8.13178807675727,112.60624999956,5.90808986649102));
#286591=CARTESIAN_POINT('Ctrl Pts',(-6.21213331202029,112.756249999559,
8.55026797822134));
#286592=CARTESIAN_POINT('Ctrl Pts',(-3.10606665601018,112.906249999559,
9.5594902125713));
#286593=CARTESIAN_POINT('Ctrl Pts',(-7.56456262199606E-14,113.056249999558,
10.5687124469213));
#286594=CARTESIAN_POINT('Ctrl Pts',(3.10606665601003,113.206249999558,9.5594902125713));
#286595=CARTESIAN_POINT('Ctrl Pts',(6.21213331202014,113.356249999557,8.55026797822134));
#286596=CARTESIAN_POINT('Ctrl Pts',(8.13178807675711,113.506249999556,5.90808986649102));
#286597=CARTESIAN_POINT('Ctrl Pts',(10.0514428414941,113.656249999556,3.2659117547607));
#286598=CARTESIAN_POINT('Ctrl Pts',(10.0514428414941,113.806249999555,-1.23094673026484E-15));
#286599=CARTESIAN_POINT('Ctrl Pts',(10.0514428414941,113.956249999555,-3.26591175476071));
#286600=CARTESIAN_POINT('Ctrl Pts',(8.13178807675711,114.106249999554,-5.90808986649102));
#286601=CARTESIAN_POINT('Ctrl Pts',(6.21213331202014,114.256249999553,-8.55026797822134));
#286602=CARTESIAN_POINT('Ctrl Pts',(3.10606665601003,114.406249999553,-9.5594902125713));
#286603=CARTESIAN_POINT('Ctrl Pts',(-7.90980688296377E-14,114.556249999552,
-10.5687124469213));
#286604=CARTESIAN_POINT('Ctrl Pts',(-3.10606665601019,114.706249999552,
-9.5594902125713));
#286605=CARTESIAN_POINT('Ctrl Pts',(-6.2121333120203,114.856249999551,-8.55026797822134));
#286606=CARTESIAN_POINT('Ctrl Pts',(-8.13178807675727,115.00624999955,-5.90808986649102));
#286607=CARTESIAN_POINT('Ctrl Pts',(-10.0514428414942,115.15624999955,-3.2659117547607));
#286608=CARTESIAN_POINT('Ctrl Pts',(-10.0514428414942,115.306249999549,
2.46189346052968E-15));
#286609=CARTESIAN_POINT('Ctrl Pts',(-10.0514428414942,115.456249999549,
3.26591175476071));
#286610=CARTESIAN_POINT('Ctrl Pts',(-8.13178807675727,115.606249999548,
5.90808986649102));
#286611=CARTESIAN_POINT('Ctrl Pts',(-6.21213331202029,115.756249999547,
8.55026797822134));
#286612=CARTESIAN_POINT('Ctrl Pts',(-3.10606665601019,115.906249999547,
9.5594902125713));
#286613=CARTESIAN_POINT('Ctrl Pts',(-7.73733354916224E-14,116.056249999546,
10.5687124469213));
#286614=CARTESIAN_POINT('Ctrl Pts',(3.10606665601003,116.206249999546,9.5594902125713));
#286615=CARTESIAN_POINT('Ctrl Pts',(6.21213331202014,116.356249999545,8.55026797822134));
#286616=CARTESIAN_POINT('Ctrl Pts',(8.13178807675711,116.506249999544,5.90808986649102));
#286617=CARTESIAN_POINT('Ctrl Pts',(10.0514428414941,116.656249999544,3.2659117547607));
#286618=CARTESIAN_POINT('Ctrl Pts',(10.0514428414941,116.806249999543,-1.23094673026484E-15));
#286619=CARTESIAN_POINT('Ctrl Pts',(10.0514428414941,116.956249999543,-3.26591175476071));
#286620=CARTESIAN_POINT('Ctrl Pts',(8.13178807675711,117.106249999542,-5.90808986649102));
#286621=CARTESIAN_POINT('Ctrl Pts',(6.21213331202014,117.256249999541,-8.55026797822134));
#286622=CARTESIAN_POINT('Ctrl Pts',(3.10606665601003,117.406249999541,-9.5594902125713));
#286623=CARTESIAN_POINT('Ctrl Pts',(-8.08257781012995E-14,117.55624999954,
-10.5687124469213));
#286624=CARTESIAN_POINT('Ctrl Pts',(-3.10606665601019,117.70624999954,-9.5594902125713));
#286625=CARTESIAN_POINT('Ctrl Pts',(-6.2121333120203,117.856249999539,-8.55026797822134));
#286626=CARTESIAN_POINT('Ctrl Pts',(-8.13178807675727,118.006249999538,
-5.90808986649102));
#286627=CARTESIAN_POINT('Ctrl Pts',(-10.0514428414942,118.156249999538,
-3.2659117547607));
#286628=CARTESIAN_POINT('Ctrl Pts',(-10.0514428414942,118.306249999537,
2.46189346052968E-15));
#286629=CARTESIAN_POINT('Ctrl Pts',(-10.0514428414942,118.456249999537,
3.26591175476071));
#286630=CARTESIAN_POINT('Ctrl Pts',(-8.13178807675727,118.606249999536,
5.90808986649102));
#286631=CARTESIAN_POINT('Ctrl Pts',(-6.2121333120203,118.756249999535,8.55026797822134));
#286632=CARTESIAN_POINT('Ctrl Pts',(-3.10606665601019,118.906249999535,
9.5594902125713));
#286633=CARTESIAN_POINT('Ctrl Pts',(-7.91010447632842E-14,119.056249999534,
10.5687124469213));
#286634=CARTESIAN_POINT('Ctrl Pts',(3.10606665601003,119.206249999534,9.5594902125713));
#286635=CARTESIAN_POINT('Ctrl Pts',(6.21213331202014,119.356249999533,8.55026797822134));
#286636=CARTESIAN_POINT('Ctrl Pts',(8.13178807675711,119.506249999532,5.90808986649102));
#286637=CARTESIAN_POINT('Ctrl Pts',(10.0514428414941,119.656249999532,3.2659117547607));
#286638=CARTESIAN_POINT('Ctrl Pts',(10.0514428414941,119.806249999531,-1.23094673026484E-15));
#286639=CARTESIAN_POINT('Ctrl Pts',(10.0514428414941,119.956249999531,-3.26591175476071));
#286640=CARTESIAN_POINT('Ctrl Pts',(8.13178807675711,120.10624999953,-5.90808986649102));
#286641=CARTESIAN_POINT('Ctrl Pts',(6.21213331202013,120.256249999529,-8.55026797822134));
#286642=CARTESIAN_POINT('Ctrl Pts',(3.10606665601003,120.406249999529,-9.5594902125713));
#286643=CARTESIAN_POINT('Ctrl Pts',(-8.25534873729613E-14,120.556249999528,
-10.5687124469213));
#286644=CARTESIAN_POINT('Ctrl Pts',(-3.10606665601019,120.706249999528,
-9.5594902125713));
#286645=CARTESIAN_POINT('Ctrl Pts',(-6.2121333120203,120.856249999527,-8.55026797822134));
#286646=CARTESIAN_POINT('Ctrl Pts',(-8.13178807675727,121.006249999526,
-5.90808986649102));
#286647=CARTESIAN_POINT('Ctrl Pts',(-10.0514428414943,121.156249999526,
-3.2659117547607));
#286648=CARTESIAN_POINT('Ctrl Pts',(-10.0514428414943,121.306249999525,
2.46189346052968E-15));
#286649=CARTESIAN_POINT('Ctrl Pts',(-10.0514428414943,121.456249999525,
3.26591175476071));
#286650=CARTESIAN_POINT('Ctrl Pts',(-8.13178807675727,121.606249999524,
5.90808986649102));
#286651=CARTESIAN_POINT('Ctrl Pts',(-6.2121333120203,121.756249999523,8.55026797822134));
#286652=CARTESIAN_POINT('Ctrl Pts',(-3.10606665601019,121.906249999523,
9.5594902125713));
#286653=CARTESIAN_POINT('Ctrl Pts',(-8.08287540349461E-14,122.056249999522,
10.5687124469213));
#286654=CARTESIAN_POINT('Ctrl Pts',(3.10606665601003,122.206249999522,9.5594902125713));
#286655=CARTESIAN_POINT('Ctrl Pts',(6.21213331202014,122.356249999521,8.55026797822134));
#286656=CARTESIAN_POINT('Ctrl Pts',(8.13178807675711,122.50624999952,5.90808986649102));
#286657=CARTESIAN_POINT('Ctrl Pts',(10.0514428414941,122.65624999952,3.2659117547607));
#286658=CARTESIAN_POINT('Ctrl Pts',(10.0514428414941,122.806249999519,-1.23094673026484E-15));
#286659=CARTESIAN_POINT('Ctrl Pts',(10.0514428414941,122.956249999519,-3.26591175476071));
#286660=CARTESIAN_POINT('Ctrl Pts',(8.13178807675711,123.106249999518,-5.90808986649102));
#286661=CARTESIAN_POINT('Ctrl Pts',(6.21213331202013,123.256249999517,-8.55026797822134));
#286662=CARTESIAN_POINT('Ctrl Pts',(3.10606665601002,123.406249999517,-9.5594902125713));
#286663=CARTESIAN_POINT('Ctrl Pts',(-8.42811966446232E-14,123.556249999516,
-10.5687124469213));
#286664=CARTESIAN_POINT('Ctrl Pts',(-3.10606665601019,123.706249999516,
-9.5594902125713));
#286665=CARTESIAN_POINT('Ctrl Pts',(-6.2121333120203,123.856249999515,-8.55026797822134));
#286666=CARTESIAN_POINT('Ctrl Pts',(-8.13178807675727,124.006249999514,
-5.90808986649102));
#286667=CARTESIAN_POINT('Ctrl Pts',(-10.0514428414943,124.156249999514,
-3.2659117547607));
#286668=CARTESIAN_POINT('Ctrl Pts',(-10.0514428414943,124.306249999513,
2.46189346052968E-15));
#286669=CARTESIAN_POINT('Ctrl Pts',(-10.0514428414943,124.456249999513,
3.26591175476071));
#286670=CARTESIAN_POINT('Ctrl Pts',(-8.13178807675727,124.606249999512,
5.90808986649102));
#286671=CARTESIAN_POINT('Ctrl Pts',(-6.2121333120203,124.756249999511,8.55026797822134));
#286672=CARTESIAN_POINT('Ctrl Pts',(-3.10606665601019,124.906249999511,
9.5594902125713));
#286673=CARTESIAN_POINT('Ctrl Pts',(-8.25564633066079E-14,125.05624999951,
10.5687124469213));
#286674=CARTESIAN_POINT('Ctrl Pts',(3.10606665601002,125.20624999951,9.5594902125713));
#286675=CARTESIAN_POINT('Ctrl Pts',(6.21213331202013,125.356249999509,8.55026797822134));
#286676=CARTESIAN_POINT('Ctrl Pts',(8.13178807675711,125.506249999508,5.90808986649102));
#286677=CARTESIAN_POINT('Ctrl Pts',(10.0514428414941,125.656249999508,3.2659117547607));
#286678=CARTESIAN_POINT('Ctrl Pts',(10.0514428414941,125.806249999507,-1.23094673026484E-15));
#286679=CARTESIAN_POINT('Ctrl Pts',(10.0514428414941,125.956249999507,-3.26591175476071));
#286680=CARTESIAN_POINT('Ctrl Pts',(8.13178807675711,126.106249999506,-5.90808986649102));
#286681=CARTESIAN_POINT('Ctrl Pts',(6.21213331202013,126.256249999505,-8.55026797822134));
#286682=CARTESIAN_POINT('Ctrl Pts',(3.10606665601002,126.406249999505,-9.5594902125713));
#286683=CARTESIAN_POINT('Ctrl Pts',(-8.6008905916285E-14,126.556249999504,
-10.5687124469213));
#286684=CARTESIAN_POINT('Ctrl Pts',(-3.10606665601019,126.706249999504,
-9.5594902125713));
#286685=CARTESIAN_POINT('Ctrl Pts',(-6.2121333120203,126.856249999503,-8.55026797822134));
#286686=CARTESIAN_POINT('Ctrl Pts',(-8.13178807675728,127.006249999502,
-5.90808986649102));
#286687=CARTESIAN_POINT('Ctrl Pts',(-10.0514428414943,127.156249999502,
-3.2659117547607));
#286688=CARTESIAN_POINT('Ctrl Pts',(-10.0514428414943,127.306249999501,
2.46189346052968E-15));
#286689=CARTESIAN_POINT('Ctrl Pts',(-10.0514428414943,127.456249999501,
3.26591175476071));
#286690=CARTESIAN_POINT('Ctrl Pts',(-8.13178807675728,127.6062499995,5.90808986649102));
#286691=CARTESIAN_POINT('Ctrl Pts',(-6.2121333120203,127.756249999499,8.55026797822134));
#286692=CARTESIAN_POINT('Ctrl Pts',(-3.10606665601019,127.906249999499,
9.5594902125713));
#286693=CARTESIAN_POINT('Ctrl Pts',(-8.42841725782698E-14,128.056249999498,
10.5687124469213));
#286694=CARTESIAN_POINT('Ctrl Pts',(3.10606665601002,128.206249999498,9.5594902125713));
#286695=CARTESIAN_POINT('Ctrl Pts',(6.21213331202013,128.356249999497,8.55026797822134));
#286696=CARTESIAN_POINT('Ctrl Pts',(8.1317880767571,128.506249999496,5.90808986649102));
#286697=CARTESIAN_POINT('Ctrl Pts',(10.0514428414941,128.656249999496,3.2659117547607));
#286698=CARTESIAN_POINT('Ctrl Pts',(10.0514428414941,128.806249999495,-1.23094673026484E-15));
#286699=CARTESIAN_POINT('Ctrl Pts',(10.0514428414941,128.956249999495,-3.26591175476071));
#286700=CARTESIAN_POINT('Ctrl Pts',(8.1317880767571,129.106249999494,-5.90808986649102));
#286701=CARTESIAN_POINT('Ctrl Pts',(6.21213331202013,129.256249999493,-8.55026797822134));
#286702=CARTESIAN_POINT('Ctrl Pts',(3.10606665601002,129.406249999493,-9.5594902125713));
#286703=CARTESIAN_POINT('Ctrl Pts',(-8.77366151879469E-14,129.556249999492,
-10.5687124469213));
#286704=CARTESIAN_POINT('Ctrl Pts',(-3.1060666560102,129.706249999492,-9.5594902125713));
#286705=CARTESIAN_POINT('Ctrl Pts',(-6.2121333120203,129.856249999491,-8.55026797822134));
#286706=CARTESIAN_POINT('Ctrl Pts',(-8.13178807675728,130.00624999949,-5.90808986649102));
#286707=CARTESIAN_POINT('Ctrl Pts',(-10.0514428414943,130.15624999949,-3.2659117547607));
#286708=CARTESIAN_POINT('Ctrl Pts',(-10.0514428414943,130.306249999489,
2.46189346052968E-15));
#286709=CARTESIAN_POINT('Ctrl Pts',(-10.0514428414943,130.456249999489,
3.26591175476071));
#286710=CARTESIAN_POINT('Ctrl Pts',(-8.13178807675728,130.606249999488,
5.90808986649102));
#286711=CARTESIAN_POINT('Ctrl Pts',(-6.2121333120203,130.756249999487,8.55026797822134));
#286712=CARTESIAN_POINT('Ctrl Pts',(-3.10606665601019,130.906249999487,
9.5594902125713));
#286713=CARTESIAN_POINT('Ctrl Pts',(-8.60118818499316E-14,131.056249999486,
10.5687124469213));
#286714=CARTESIAN_POINT('Ctrl Pts',(3.10606665601002,131.206249999486,9.5594902125713));
#286715=CARTESIAN_POINT('Ctrl Pts',(6.21213331202013,131.356249999485,8.55026797822134));
#286716=CARTESIAN_POINT('Ctrl Pts',(8.1317880767571,131.506249999484,5.90808986649102));
#286717=CARTESIAN_POINT('Ctrl Pts',(10.0514428414941,131.656249999484,3.2659117547607));
#286718=CARTESIAN_POINT('Ctrl Pts',(10.0514428414941,131.806249999483,-1.23094673026484E-15));
#286719=CARTESIAN_POINT('Ctrl Pts',(10.0514428414941,131.956249999483,-3.26591175476071));
#286720=CARTESIAN_POINT('Ctrl Pts',(8.1317880767571,132.106249999482,-5.90808986649102));
#286721=CARTESIAN_POINT('Ctrl Pts',(6.21213331202012,132.256249999481,-8.55026797822134));
#286722=CARTESIAN_POINT('Ctrl Pts',(3.10606665601002,132.406249999481,-9.5594902125713));
#286723=CARTESIAN_POINT('Ctrl Pts',(-8.94643244596087E-14,132.55624999948,
-10.5687124469213));
#286724=CARTESIAN_POINT('Ctrl Pts',(-3.1060666560102,132.70624999948,-9.5594902125713));
#286725=CARTESIAN_POINT('Ctrl Pts',(-6.2121333120203,132.856249999479,-8.55026797822134));
#286726=CARTESIAN_POINT('Ctrl Pts',(-8.13178807675728,133.006249999478,
-5.90808986649102));
#286727=CARTESIAN_POINT('Ctrl Pts',(-10.0514428414943,133.156249999478,
-3.2659117547607));
#286728=CARTESIAN_POINT('Ctrl Pts',(-10.0514428414943,133.306249999477,
2.46189346052968E-15));
#286729=CARTESIAN_POINT('Ctrl Pts',(-10.0514428414943,133.456249999477,
3.26591175476071));
#286730=CARTESIAN_POINT('Ctrl Pts',(-8.13178807675728,133.606249999476,
5.90808986649102));
#286731=CARTESIAN_POINT('Ctrl Pts',(-6.2121333120203,133.756249999475,8.55026797822134));
#286732=CARTESIAN_POINT('Ctrl Pts',(-3.1060666560102,133.906249999475,9.5594902125713));
#286733=CARTESIAN_POINT('Ctrl Pts',(-8.77395911215934E-14,134.056249999474,
10.5687124469213));
#286734=CARTESIAN_POINT('Ctrl Pts',(3.10606665601002,134.206249999474,9.5594902125713));
#286735=CARTESIAN_POINT('Ctrl Pts',(6.21213331202013,134.356249999473,8.55026797822134));
#286736=CARTESIAN_POINT('Ctrl Pts',(8.1317880767571,134.506249999472,5.90808986649102));
#286737=CARTESIAN_POINT('Ctrl Pts',(10.0514428414941,134.656249999472,3.2659117547607));
#286738=CARTESIAN_POINT('Ctrl Pts',(10.0514428414941,134.806249999471,-1.23094673026484E-15));
#286739=CARTESIAN_POINT('Ctrl Pts',(10.0514428414941,134.956249999471,-3.26591175476071));
#286740=CARTESIAN_POINT('Ctrl Pts',(8.1317880767571,135.10624999947,-5.90808986649102));
#286741=CARTESIAN_POINT('Ctrl Pts',(6.21213331202012,135.256249999469,-8.55026797822134));
#286742=CARTESIAN_POINT('Ctrl Pts',(3.10606665601002,135.406249999469,-9.5594902125713));
#286743=CARTESIAN_POINT('Ctrl Pts',(-9.11920337312706E-14,135.556249999468,
-10.5687124469213));
#286744=CARTESIAN_POINT('Ctrl Pts',(-3.1060666560102,135.706249999468,-9.5594902125713));
#286745=CARTESIAN_POINT('Ctrl Pts',(-6.21213331202031,135.856249999467,
-8.55026797822134));
#286746=CARTESIAN_POINT('Ctrl Pts',(-8.13178807675728,136.006249999466,
-5.90808986649102));
#286747=CARTESIAN_POINT('Ctrl Pts',(-10.0514428414943,136.156249999466,
-3.2659117547607));
#286748=CARTESIAN_POINT('Ctrl Pts',(-10.0514428414943,136.306249999465,
2.46189346052968E-15));
#286749=CARTESIAN_POINT('Ctrl Pts',(-10.0514428414943,136.456249999465,
3.26591175476071));
#286750=CARTESIAN_POINT('Ctrl Pts',(-8.13178807675728,136.606249999464,
5.90808986649102));
#286751=CARTESIAN_POINT('Ctrl Pts',(-6.2121333120203,136.756249999463,8.55026797822134));
#286752=CARTESIAN_POINT('Ctrl Pts',(-3.1060666560102,136.906249999463,9.5594902125713));
#286753=CARTESIAN_POINT('Ctrl Pts',(-8.94673003932553E-14,137.056249999462,
10.5687124469213));
#286754=CARTESIAN_POINT('Ctrl Pts',(3.10606665601002,137.206249999462,9.5594902125713));
#286755=CARTESIAN_POINT('Ctrl Pts',(6.21213331202012,137.356249999461,8.55026797822134));
#286756=CARTESIAN_POINT('Ctrl Pts',(8.1317880767571,137.50624999946,5.90808986649102));
#286757=CARTESIAN_POINT('Ctrl Pts',(10.0514428414941,137.65624999946,3.2659117547607));
#286758=CARTESIAN_POINT('Ctrl Pts',(10.0514428414941,137.806249999459,-1.23094673026484E-15));
#286759=CARTESIAN_POINT('Ctrl Pts',(10.0514428414941,137.956249999459,-3.26591175476071));
#286760=CARTESIAN_POINT('Ctrl Pts',(8.1317880767571,138.106249999458,-5.90808986649102));
#286761=CARTESIAN_POINT('Ctrl Pts',(6.21213331202012,138.256249999457,-8.55026797822134));
#286762=CARTESIAN_POINT('Ctrl Pts',(3.10606665601001,138.406249999457,-9.5594902125713));
#286763=CARTESIAN_POINT('Ctrl Pts',(-9.29197430029324E-14,138.556249999456,
-10.5687124469213));
#286764=CARTESIAN_POINT('Ctrl Pts',(-3.1060666560102,138.706249999456,-9.5594902125713));
#286765=CARTESIAN_POINT('Ctrl Pts',(-6.21213331202031,138.856249999455,
-8.55026797822134));
#286766=CARTESIAN_POINT('Ctrl Pts',(-8.13178807675728,139.006249999454,
-5.90808986649102));
#286767=CARTESIAN_POINT('Ctrl Pts',(-10.0514428414943,139.156249999454,
-3.2659117547607));
#286768=CARTESIAN_POINT('Ctrl Pts',(-10.0514428414943,139.306249999453,
2.46189346052968E-15));
#286769=CARTESIAN_POINT('Ctrl Pts',(-10.0514428414943,139.456249999453,
3.26591175476071));
#286770=CARTESIAN_POINT('Ctrl Pts',(-8.13178807675728,139.606249999452,
5.90808986649102));
#286771=CARTESIAN_POINT('Ctrl Pts',(-6.21213331202031,139.756249999451,
8.55026797822134));
#286772=CARTESIAN_POINT('Ctrl Pts',(-3.1060666560102,139.906249999451,9.5594902125713));
#286773=CARTESIAN_POINT('Ctrl Pts',(-9.11950096649171E-14,140.05624999945,
10.5687124469213));
#286774=CARTESIAN_POINT('Ctrl Pts',(3.10606665601002,140.20624999945,9.5594902125713));
#286775=CARTESIAN_POINT('Ctrl Pts',(6.21213331202012,140.356249999449,8.55026797822134));
#286776=CARTESIAN_POINT('Ctrl Pts',(8.1317880767571,140.506249999448,5.90808986649102));
#286777=CARTESIAN_POINT('Ctrl Pts',(10.0514428414941,140.656249999448,3.2659117547607));
#286778=CARTESIAN_POINT('Ctrl Pts',(10.0514428414941,140.806249999447,-1.23094673026484E-15));
#286779=CARTESIAN_POINT('Ctrl Pts',(10.0514428414941,140.956249999447,-3.26591175476071));
#286780=CARTESIAN_POINT('Ctrl Pts',(8.1317880767571,141.106249999446,-5.90808986649102));
#286781=CARTESIAN_POINT('Ctrl Pts',(6.21213331202012,141.256249999445,-8.55026797822134));
#286782=CARTESIAN_POINT('Ctrl Pts',(3.10606665601001,141.406249999445,-9.5594902125713));
#286783=CARTESIAN_POINT('Ctrl Pts',(-9.46474522745942E-14,141.556249999444,
-10.5687124469213));
#286784=CARTESIAN_POINT('Ctrl Pts',(-3.1060666560102,141.706249999444,-9.5594902125713));
#286785=CARTESIAN_POINT('Ctrl Pts',(-6.21213331202031,141.856249999443,
-8.55026797822134));
#286786=CARTESIAN_POINT('Ctrl Pts',(-8.13178807675729,142.006249999442,
-5.90808986649102));
#286787=CARTESIAN_POINT('Ctrl Pts',(-10.0514428414943,142.156249999442,
-3.2659117547607));
#286788=CARTESIAN_POINT('Ctrl Pts',(-10.0514428414943,142.306249999441,
2.46189346052968E-15));
#286789=CARTESIAN_POINT('Ctrl Pts',(-10.0514428414943,142.456249999441,
3.26591175476071));
#286790=CARTESIAN_POINT('Ctrl Pts',(-8.13178807675729,142.60624999944,5.90808986649102));
#286791=CARTESIAN_POINT('Ctrl Pts',(-6.21213331202031,142.756249999439,
8.55026797822134));
#286792=CARTESIAN_POINT('Ctrl Pts',(-3.1060666560102,142.906249999439,9.5594902125713));
#286793=CARTESIAN_POINT('Ctrl Pts',(-9.29227189365789E-14,143.056249999438,
10.5687124469213));
#286794=CARTESIAN_POINT('Ctrl Pts',(3.10606665601001,143.206249999438,9.5594902125713));
#286795=CARTESIAN_POINT('Ctrl Pts',(6.21213331202012,143.356249999437,8.55026797822134));
#286796=CARTESIAN_POINT('Ctrl Pts',(8.1317880767571,143.506249999436,5.90808986649102));
#286797=CARTESIAN_POINT('Ctrl Pts',(10.0514428414941,143.656249999436,3.2659117547607));
#286798=CARTESIAN_POINT('Ctrl Pts',(10.0514428414941,143.806249999435,-1.23094673026484E-15));
#286799=CARTESIAN_POINT('Ctrl Pts',(10.0514428414941,143.956249999435,-3.26591175476071));
#286800=CARTESIAN_POINT('Ctrl Pts',(8.1317880767571,144.106249999434,-5.90808986649102));
#286801=CARTESIAN_POINT('Ctrl Pts',(6.21213331202012,144.256249999433,-8.55026797822134));
#286802=CARTESIAN_POINT('Ctrl Pts',(3.10606665601001,144.406249999433,-9.5594902125713));
#286803=CARTESIAN_POINT('Ctrl Pts',(-9.63751615462561E-14,144.556249999432,
-10.5687124469213));
#286804=CARTESIAN_POINT('Ctrl Pts',(-3.1060666560102,144.706249999432,-9.5594902125713));
#286805=CARTESIAN_POINT('Ctrl Pts',(-6.21213331202031,144.856249999431,
-8.55026797822134));
#286806=CARTESIAN_POINT('Ctrl Pts',(-8.13178807675729,145.00624999943,-5.90808986649102));
#286807=CARTESIAN_POINT('Ctrl Pts',(-10.0514428414943,145.15624999943,-3.2659117547607));
#286808=CARTESIAN_POINT('Ctrl Pts',(-10.0514428414943,145.306249999429,
2.46189346052968E-15));
#286809=CARTESIAN_POINT('Ctrl Pts',(-10.0514428414943,145.456249999429,
3.26591175476071));
#286810=CARTESIAN_POINT('Ctrl Pts',(-8.13178807675729,145.606249999428,
5.90808986649102));
#286811=CARTESIAN_POINT('Ctrl Pts',(-6.21213331202031,145.756249999427,
8.55026797822134));
#286812=CARTESIAN_POINT('Ctrl Pts',(-3.1060666560102,145.906249999427,9.5594902125713));
#286813=CARTESIAN_POINT('Ctrl Pts',(-9.46504282082408E-14,146.056249999426,
10.5687124469213));
#286814=CARTESIAN_POINT('Ctrl Pts',(3.10606665601001,146.206249999426,9.5594902125713));
#286815=CARTESIAN_POINT('Ctrl Pts',(6.21213331202012,146.356249999425,8.55026797822134));
#286816=CARTESIAN_POINT('Ctrl Pts',(8.13178807675709,146.506249999424,5.90808986649102));
#286817=CARTESIAN_POINT('Ctrl Pts',(10.0514428414941,146.656249999424,3.2659117547607));
#286818=CARTESIAN_POINT('Ctrl Pts',(10.0514428414941,146.806249999423,-1.23094673026484E-15));
#286819=CARTESIAN_POINT('Ctrl Pts',(10.0514428414941,146.956249999423,-3.26591175476071));
#286820=CARTESIAN_POINT('Ctrl Pts',(8.13178807675709,147.106249999422,-5.90808986649102));
#286821=CARTESIAN_POINT('Ctrl Pts',(6.21213331202012,147.256249999421,-8.55026797822134));
#286822=CARTESIAN_POINT('Ctrl Pts',(3.10606665601001,147.406249999421,-9.5594902125713));
#286823=CARTESIAN_POINT('Ctrl Pts',(-9.81028708179179E-14,147.55624999942,
-10.5687124469213));
#286824=CARTESIAN_POINT('Ctrl Pts',(-3.10606665601021,147.70624999942,-9.5594902125713));
#286825=CARTESIAN_POINT('Ctrl Pts',(-6.21213331202032,147.856249999419,
-8.55026797822134));
#286826=CARTESIAN_POINT('Ctrl Pts',(-8.13178807675729,148.006249999418,
-5.90808986649102));
#286827=CARTESIAN_POINT('Ctrl Pts',(-10.0514428414943,148.156249999418,
-3.2659117547607));
#286828=CARTESIAN_POINT('Ctrl Pts',(-10.0514428414943,148.306249999417,
2.46189346052968E-15));
#286829=CARTESIAN_POINT('Ctrl Pts',(-10.0514428414943,148.456249999417,
3.26591175476071));
#286830=CARTESIAN_POINT('Ctrl Pts',(-8.13178807675729,148.606249999416,
5.90808986649102));
#286831=CARTESIAN_POINT('Ctrl Pts',(-6.21213331202031,148.756249999415,
8.55026797822134));
#286832=CARTESIAN_POINT('Ctrl Pts',(-3.1060666560102,148.906249999415,9.5594902125713));
#286833=CARTESIAN_POINT('Ctrl Pts',(-9.63781374799026E-14,149.056249999414,
10.5687124469213));
#286834=CARTESIAN_POINT('Ctrl Pts',(3.10606665601001,149.206249999414,9.5594902125713));
#286835=CARTESIAN_POINT('Ctrl Pts',(6.21213331202012,149.356249999413,8.55026797822134));
#286836=CARTESIAN_POINT('Ctrl Pts',(8.13178807675709,149.506249999412,5.90808986649102));
#286837=CARTESIAN_POINT('Ctrl Pts',(10.0514428414941,149.656249999412,3.2659117547607));
#286838=CARTESIAN_POINT('Ctrl Pts',(10.0514428414941,149.806249999411,-1.23094673026484E-15));
#286839=CARTESIAN_POINT('Ctrl Pts',(10.0514428414941,149.956249999411,-3.26591175476071));
#286840=CARTESIAN_POINT('Ctrl Pts',(8.13178807675709,150.10624999941,-5.90808986649102));
#286841=CARTESIAN_POINT('Ctrl Pts',(6.21213331202012,150.256249999409,-8.55026797822134));
#286842=CARTESIAN_POINT('Ctrl Pts',(3.10606665601001,150.406249999409,-9.5594902125713));
#286843=CARTESIAN_POINT('Ctrl Pts',(-9.98305800895797E-14,150.556249999408,
-10.5687124469213));
#286844=CARTESIAN_POINT('Ctrl Pts',(-3.10606665601021,150.706249999408,
-9.5594902125713));
#286845=CARTESIAN_POINT('Ctrl Pts',(-6.21213331202032,150.856249999407,
-8.55026797822134));
#286846=CARTESIAN_POINT('Ctrl Pts',(-8.13178807675729,151.006249999406,
-5.90808986649102));
#286847=CARTESIAN_POINT('Ctrl Pts',(-10.0514428414943,151.156249999406,
-3.2659117547607));
#286848=CARTESIAN_POINT('Ctrl Pts',(-10.0514428414943,151.306249999405,
2.46189346052968E-15));
#286849=CARTESIAN_POINT('Ctrl Pts',(-10.0514428414943,151.456249999405,
3.26591175476071));
#286850=CARTESIAN_POINT('Ctrl Pts',(-8.13178807675729,151.606249999404,
5.90808986649102));
#286851=CARTESIAN_POINT('Ctrl Pts',(-6.21213331202032,151.756249999403,
8.55026797822134));
#286852=CARTESIAN_POINT('Ctrl Pts',(-3.10606665601021,151.906249999403,
9.5594902125713));
#286853=CARTESIAN_POINT('Ctrl Pts',(-9.81058467515645E-14,152.056249999402,
10.5687124469213));
#286854=CARTESIAN_POINT('Ctrl Pts',(3.10606665601001,152.206249999402,9.5594902125713));
#286855=CARTESIAN_POINT('Ctrl Pts',(6.21213331202012,152.356249999401,8.55026797822134));
#286856=CARTESIAN_POINT('Ctrl Pts',(8.13178807675709,152.5062499994,5.90808986649102));
#286857=CARTESIAN_POINT('Ctrl Pts',(10.0514428414941,152.6562499994,3.2659117547607));
#286858=CARTESIAN_POINT('Ctrl Pts',(10.0514428414941,152.806249999399,-1.23094673026484E-15));
#286859=CARTESIAN_POINT('Ctrl Pts',(10.0514428414941,152.956249999399,-3.26591175476071));
#286860=CARTESIAN_POINT('Ctrl Pts',(8.13178807675709,153.106249999398,-5.90808986649102));
#286861=CARTESIAN_POINT('Ctrl Pts',(6.21213331202012,153.256249999397,-8.55026797822134));
#286862=CARTESIAN_POINT('Ctrl Pts',(3.10606665601001,153.406249999397,-9.5594902125713));
#286863=CARTESIAN_POINT('Ctrl Pts',(-1.01558289361242E-13,153.556249999396,
-10.5687124469213));
#286864=CARTESIAN_POINT('Ctrl Pts',(-3.10606665601021,153.706249999396,
-9.5594902125713));
#286865=CARTESIAN_POINT('Ctrl Pts',(-12.1623797632097,-0.474999999988005,
2.97892388940585E-15));
#286866=CARTESIAN_POINT('Ctrl Pts',(-12.1623797632096,-0.324999999988605,
3.95179673813133));
#286867=CARTESIAN_POINT('Ctrl Pts',(-9.83957192047856,-0.174999999989203,
7.14886745759505));
#286868=CARTESIAN_POINT('Ctrl Pts',(-7.51676407774747,-0.0249999999898023,
10.3459381770588));
#286869=CARTESIAN_POINT('Ctrl Pts',(-3.75838203887374,0.1250000000096,11.5671105274568));
#286870=CARTESIAN_POINT('Ctrl Pts',(-1.02868273148643E-14,0.275000000009002,
12.7882828778549));
#286871=CARTESIAN_POINT('Ctrl Pts',(3.75838203887372,0.425000000008404,
11.5671105274568));
#286872=CARTESIAN_POINT('Ctrl Pts',(7.51676407774745,0.575000000007806,
10.3459381770588));
#286873=CARTESIAN_POINT('Ctrl Pts',(9.83957192047854,0.725000000007208,
7.14886745759505));
#286874=CARTESIAN_POINT('Ctrl Pts',(12.1623797632096,0.875000000006609,
3.95179673813132));
#286875=CARTESIAN_POINT('Ctrl Pts',(12.1623797632096,1.02500000000601,-1.48946194470292E-15));
#286876=CARTESIAN_POINT('Ctrl Pts',(12.1623797632096,1.17500000000541,-3.95179673813132));
#286877=CARTESIAN_POINT('Ctrl Pts',(9.83957192047853,1.32500000000481,-7.14886745759505));
#286878=CARTESIAN_POINT('Ctrl Pts',(7.51676407774744,1.47500000000421,-10.3459381770588));
#286879=CARTESIAN_POINT('Ctrl Pts',(3.75838203887371,1.6250000000036,-11.5671105274568));
#286880=CARTESIAN_POINT('Ctrl Pts',(-1.42829078892864E-14,1.775000000003,
-12.7882828778549));
#286881=CARTESIAN_POINT('Ctrl Pts',(-3.75838203887374,1.9250000000024,-11.5671105274568));
#286882=CARTESIAN_POINT('Ctrl Pts',(-7.51676407774747,2.0750000000018,-10.3459381770588));
#286883=CARTESIAN_POINT('Ctrl Pts',(-9.83957192047856,2.2250000000012,-7.14886745759505));
#286884=CARTESIAN_POINT('Ctrl Pts',(-12.1623797632097,2.37500000000059,
-3.95179673813132));
#286885=CARTESIAN_POINT('Ctrl Pts',(-12.1623797632097,2.525,2.97892388940585E-15));
#286886=CARTESIAN_POINT('Ctrl Pts',(-12.1623797632097,2.6749999999994,3.95179673813133));
#286887=CARTESIAN_POINT('Ctrl Pts',(-9.83957192047856,2.8249999999988,7.14886745759505));
#286888=CARTESIAN_POINT('Ctrl Pts',(-7.51676407774747,2.9749999999982,10.3459381770588));
#286889=CARTESIAN_POINT('Ctrl Pts',(-3.75838203887374,3.1249999999976,11.5671105274568));
#286890=CARTESIAN_POINT('Ctrl Pts',(-1.20145365865262E-14,3.274999999997,
12.7882828778549));
#286891=CARTESIAN_POINT('Ctrl Pts',(3.75838203887372,3.4249999999964,11.5671105274568));
#286892=CARTESIAN_POINT('Ctrl Pts',(7.51676407774744,3.57499999999581,10.3459381770588));
#286893=CARTESIAN_POINT('Ctrl Pts',(9.83957192047853,3.72499999999521,7.14886745759505));
#286894=CARTESIAN_POINT('Ctrl Pts',(12.1623797632096,3.87499999999461,3.95179673813132));
#286895=CARTESIAN_POINT('Ctrl Pts',(12.1623797632096,4.02499999999401,-1.48946194470292E-15));
#286896=CARTESIAN_POINT('Ctrl Pts',(12.1623797632096,4.17499999999341,-3.95179673813132));
#286897=CARTESIAN_POINT('Ctrl Pts',(9.83957192047853,4.32499999999281,-7.14886745759505));
#286898=CARTESIAN_POINT('Ctrl Pts',(7.51676407774744,4.47499999999221,-10.3459381770588));
#286899=CARTESIAN_POINT('Ctrl Pts',(3.75838203887371,4.6249999999916,-11.5671105274568));
#286900=CARTESIAN_POINT('Ctrl Pts',(-1.60106171609483E-14,4.774999999991,
-12.7882828778549));
#286901=CARTESIAN_POINT('Ctrl Pts',(-3.75838203887374,4.9249999999904,-11.5671105274568));
#286902=CARTESIAN_POINT('Ctrl Pts',(-7.51676407774747,5.0749999999898,-10.3459381770588));
#286903=CARTESIAN_POINT('Ctrl Pts',(-9.83957192047857,5.2249999999892,-7.14886745759505));
#286904=CARTESIAN_POINT('Ctrl Pts',(-12.1623797632097,5.3749999999886,-3.95179673813132));
#286905=CARTESIAN_POINT('Ctrl Pts',(-12.1623797632097,5.52499999998799,
2.97892388940585E-15));
#286906=CARTESIAN_POINT('Ctrl Pts',(-12.1623797632097,5.6749999999874,3.95179673813133));
#286907=CARTESIAN_POINT('Ctrl Pts',(-9.83957192047857,5.8249999999868,7.14886745759505));
#286908=CARTESIAN_POINT('Ctrl Pts',(-7.51676407774747,5.9749999999862,10.3459381770588));
#286909=CARTESIAN_POINT('Ctrl Pts',(-3.75838203887374,6.1249999999856,11.5671105274568));
#286910=CARTESIAN_POINT('Ctrl Pts',(-1.3742245858188E-14,6.274999999985,
12.7882828778549));
#286911=CARTESIAN_POINT('Ctrl Pts',(3.75838203887371,6.4249999999844,11.5671105274568));
#286912=CARTESIAN_POINT('Ctrl Pts',(7.51676407774744,6.57499999998381,10.3459381770588));
#286913=CARTESIAN_POINT('Ctrl Pts',(9.83957192047853,6.72499999998321,7.14886745759505));
#286914=CARTESIAN_POINT('Ctrl Pts',(12.1623797632096,6.87499999998261,3.95179673813132));
#286915=CARTESIAN_POINT('Ctrl Pts',(12.1623797632096,7.02499999998201,-1.48946194470292E-15));
#286916=CARTESIAN_POINT('Ctrl Pts',(12.1623797632096,7.17499999998141,-3.95179673813132));
#286917=CARTESIAN_POINT('Ctrl Pts',(9.83957192047853,7.32499999998081,-7.14886745759505));
#286918=CARTESIAN_POINT('Ctrl Pts',(7.51676407774744,7.47499999998021,-10.3459381770588));
#286919=CARTESIAN_POINT('Ctrl Pts',(3.75838203887371,7.6249999999796,-11.5671105274568));
#286920=CARTESIAN_POINT('Ctrl Pts',(-1.77383264326101E-14,7.774999999979,
-12.7882828778549));
#286921=CARTESIAN_POINT('Ctrl Pts',(-3.75838203887375,7.9249999999784,-11.5671105274568));
#286922=CARTESIAN_POINT('Ctrl Pts',(-7.51676407774747,8.0749999999778,-10.3459381770588));
#286923=CARTESIAN_POINT('Ctrl Pts',(-9.83957192047857,8.2249999999772,-7.14886745759505));
#286924=CARTESIAN_POINT('Ctrl Pts',(-12.1623797632097,8.3749999999766,-3.95179673813132));
#286925=CARTESIAN_POINT('Ctrl Pts',(-12.1623797632097,8.52499999997599,
2.97892388940585E-15));
#286926=CARTESIAN_POINT('Ctrl Pts',(-12.1623797632097,8.6749999999754,3.95179673813133));
#286927=CARTESIAN_POINT('Ctrl Pts',(-9.83957192047857,8.8249999999748,7.14886745759505));
#286928=CARTESIAN_POINT('Ctrl Pts',(-7.51676407774747,8.9749999999742,10.3459381770588));
#286929=CARTESIAN_POINT('Ctrl Pts',(-3.75838203887374,9.1249999999736,11.5671105274568));
#286930=CARTESIAN_POINT('Ctrl Pts',(-1.54699551298498E-14,9.274999999973,
12.7882828778549));
#286931=CARTESIAN_POINT('Ctrl Pts',(3.75838203887371,9.4249999999724,11.5671105274568));
#286932=CARTESIAN_POINT('Ctrl Pts',(7.51676407774744,9.57499999997181,10.3459381770588));
#286933=CARTESIAN_POINT('Ctrl Pts',(9.83957192047853,9.72499999997121,7.14886745759505));
#286934=CARTESIAN_POINT('Ctrl Pts',(12.1623797632096,9.87499999997061,3.95179673813132));
#286935=CARTESIAN_POINT('Ctrl Pts',(12.1623797632096,10.02499999997,-1.48946194470292E-15));
#286936=CARTESIAN_POINT('Ctrl Pts',(12.1623797632096,10.1749999999694,-3.95179673813132));
#286937=CARTESIAN_POINT('Ctrl Pts',(9.83957192047853,10.3249999999688,-7.14886745759505));
#286938=CARTESIAN_POINT('Ctrl Pts',(7.51676407774744,10.4749999999682,-10.3459381770588));
#286939=CARTESIAN_POINT('Ctrl Pts',(3.75838203887371,10.6249999999676,-11.5671105274568));
#286940=CARTESIAN_POINT('Ctrl Pts',(-1.9466035704272E-14,10.774999999967,
-12.7882828778549));
#286941=CARTESIAN_POINT('Ctrl Pts',(-3.75838203887375,10.9249999999664,
-11.5671105274568));
#286942=CARTESIAN_POINT('Ctrl Pts',(-7.51676407774748,11.0749999999658,
-10.3459381770588));
#286943=CARTESIAN_POINT('Ctrl Pts',(-9.83957192047857,11.2249999999652,
-7.14886745759505));
#286944=CARTESIAN_POINT('Ctrl Pts',(-12.1623797632097,11.3749999999646,
-3.95179673813132));
#286945=CARTESIAN_POINT('Ctrl Pts',(-12.1623797632097,11.524999999964,2.97892388940585E-15));
#286946=CARTESIAN_POINT('Ctrl Pts',(-12.1623797632097,11.6749999999634,
3.95179673813133));
#286947=CARTESIAN_POINT('Ctrl Pts',(-9.83957192047857,11.8249999999628,
7.14886745759505));
#286948=CARTESIAN_POINT('Ctrl Pts',(-7.51676407774747,11.9749999999622,
10.3459381770588));
#286949=CARTESIAN_POINT('Ctrl Pts',(-3.75838203887375,12.1249999999616,
11.5671105274568));
#286950=CARTESIAN_POINT('Ctrl Pts',(-1.71976644015117E-14,12.274999999961,
12.7882828778549));
#286951=CARTESIAN_POINT('Ctrl Pts',(3.75838203887371,12.4249999999604,11.5671105274568));
#286952=CARTESIAN_POINT('Ctrl Pts',(7.51676407774744,12.5749999999598,10.3459381770588));
#286953=CARTESIAN_POINT('Ctrl Pts',(9.83957192047853,12.7249999999592,7.14886745759505));
#286954=CARTESIAN_POINT('Ctrl Pts',(12.1623797632096,12.8749999999586,3.95179673813132));
#286955=CARTESIAN_POINT('Ctrl Pts',(12.1623797632096,13.024999999958,-1.48946194470292E-15));
#286956=CARTESIAN_POINT('Ctrl Pts',(12.1623797632096,13.1749999999574,-3.95179673813132));
#286957=CARTESIAN_POINT('Ctrl Pts',(9.83957192047853,13.3249999999568,-7.14886745759505));
#286958=CARTESIAN_POINT('Ctrl Pts',(7.51676407774743,13.4749999999562,-10.3459381770588));
#286959=CARTESIAN_POINT('Ctrl Pts',(3.75838203887371,13.6249999999556,-11.5671105274568));
#286960=CARTESIAN_POINT('Ctrl Pts',(-2.11937449759338E-14,13.774999999955,
-12.7882828778549));
#286961=CARTESIAN_POINT('Ctrl Pts',(-3.75838203887375,13.9249999999544,
-11.5671105274568));
#286962=CARTESIAN_POINT('Ctrl Pts',(-7.51676407774748,14.0749999999538,
-10.3459381770588));
#286963=CARTESIAN_POINT('Ctrl Pts',(-9.83957192047857,14.2249999999532,
-7.14886745759505));
#286964=CARTESIAN_POINT('Ctrl Pts',(-12.1623797632097,14.3749999999526,
-3.95179673813132));
#286965=CARTESIAN_POINT('Ctrl Pts',(-12.1623797632097,14.524999999952,2.97892388940585E-15));
#286966=CARTESIAN_POINT('Ctrl Pts',(-12.1623797632097,14.6749999999514,
3.95179673813133));
#286967=CARTESIAN_POINT('Ctrl Pts',(-9.83957192047857,14.8249999999508,
7.14886745759505));
#286968=CARTESIAN_POINT('Ctrl Pts',(-7.51676407774747,14.9749999999502,
10.3459381770588));
#286969=CARTESIAN_POINT('Ctrl Pts',(-3.75838203887375,15.1249999999496,
11.5671105274568));
#286970=CARTESIAN_POINT('Ctrl Pts',(-1.89253736731735E-14,15.274999999949,
12.7882828778549));
#286971=CARTESIAN_POINT('Ctrl Pts',(3.75838203887371,15.4249999999484,11.5671105274568));
#286972=CARTESIAN_POINT('Ctrl Pts',(7.51676407774744,15.5749999999478,10.3459381770588));
#286973=CARTESIAN_POINT('Ctrl Pts',(9.83957192047853,15.7249999999472,7.14886745759505));
#286974=CARTESIAN_POINT('Ctrl Pts',(12.1623797632096,15.8749999999466,3.95179673813132));
#286975=CARTESIAN_POINT('Ctrl Pts',(12.1623797632096,16.024999999946,-1.48946194470292E-15));
#286976=CARTESIAN_POINT('Ctrl Pts',(12.1623797632096,16.1749999999454,-3.95179673813132));
#286977=CARTESIAN_POINT('Ctrl Pts',(9.83957192047852,16.3249999999448,-7.14886745759505));
#286978=CARTESIAN_POINT('Ctrl Pts',(7.51676407774743,16.4749999999442,-10.3459381770588));
#286979=CARTESIAN_POINT('Ctrl Pts',(3.7583820388737,16.6249999999436,-11.5671105274568));
#286980=CARTESIAN_POINT('Ctrl Pts',(-2.29214542475956E-14,16.774999999943,
-12.7882828778549));
#286981=CARTESIAN_POINT('Ctrl Pts',(-3.75838203887375,16.9249999999424,
-11.5671105274568));
#286982=CARTESIAN_POINT('Ctrl Pts',(-7.51676407774748,17.0749999999418,
-10.3459381770588));
#286983=CARTESIAN_POINT('Ctrl Pts',(-9.83957192047857,17.2249999999412,
-7.14886745759505));
#286984=CARTESIAN_POINT('Ctrl Pts',(-12.1623797632097,17.3749999999406,
-3.95179673813132));
#286985=CARTESIAN_POINT('Ctrl Pts',(-12.1623797632097,17.52499999994,2.97892388940585E-15));
#286986=CARTESIAN_POINT('Ctrl Pts',(-12.1623797632097,17.6749999999394,
3.95179673813133));
#286987=CARTESIAN_POINT('Ctrl Pts',(-9.83957192047857,17.8249999999388,
7.14886745759505));
#286988=CARTESIAN_POINT('Ctrl Pts',(-7.51676407774748,17.9749999999382,
10.3459381770588));
#286989=CARTESIAN_POINT('Ctrl Pts',(-3.75838203887375,18.1249999999376,
11.5671105274568));
#286990=CARTESIAN_POINT('Ctrl Pts',(-2.06530829448354E-14,18.274999999937,
12.7882828778549));
#286991=CARTESIAN_POINT('Ctrl Pts',(3.75838203887371,18.4249999999364,11.5671105274568));
#286992=CARTESIAN_POINT('Ctrl Pts',(7.51676407774743,18.5749999999358,10.3459381770588));
#286993=CARTESIAN_POINT('Ctrl Pts',(9.83957192047852,18.7249999999352,7.14886745759505));
#286994=CARTESIAN_POINT('Ctrl Pts',(12.1623797632096,18.8749999999346,3.95179673813132));
#286995=CARTESIAN_POINT('Ctrl Pts',(12.1623797632096,19.024999999934,-1.48946194470292E-15));
#286996=CARTESIAN_POINT('Ctrl Pts',(12.1623797632096,19.1749999999334,-3.95179673813132));
#286997=CARTESIAN_POINT('Ctrl Pts',(9.83957192047852,19.3249999999328,-7.14886745759505));
#286998=CARTESIAN_POINT('Ctrl Pts',(7.51676407774743,19.4749999999322,-10.3459381770588));
#286999=CARTESIAN_POINT('Ctrl Pts',(3.7583820388737,19.6249999999316,-11.5671105274568));
#287000=CARTESIAN_POINT('Ctrl Pts',(-2.46491635192575E-14,19.774999999931,
-12.7882828778549));
#287001=CARTESIAN_POINT('Ctrl Pts',(-3.75838203887375,19.9249999999304,
-11.5671105274568));
#287002=CARTESIAN_POINT('Ctrl Pts',(-7.51676407774748,20.0749999999298,
-10.3459381770588));
#287003=CARTESIAN_POINT('Ctrl Pts',(-9.83957192047857,20.2249999999292,
-7.14886745759505));
#287004=CARTESIAN_POINT('Ctrl Pts',(-12.1623797632097,20.3749999999286,
-3.95179673813132));
#287005=CARTESIAN_POINT('Ctrl Pts',(-12.1623797632097,20.524999999928,2.97892388940585E-15));
#287006=CARTESIAN_POINT('Ctrl Pts',(-12.1623797632097,20.6749999999274,
3.95179673813133));
#287007=CARTESIAN_POINT('Ctrl Pts',(-9.83957192047857,20.8249999999268,
7.14886745759505));
#287008=CARTESIAN_POINT('Ctrl Pts',(-7.51676407774748,20.9749999999262,
10.3459381770588));
#287009=CARTESIAN_POINT('Ctrl Pts',(-3.75838203887375,21.1249999999256,
11.5671105274568));
#287010=CARTESIAN_POINT('Ctrl Pts',(-2.23807922164972E-14,21.274999999925,
12.7882828778549));
#287011=CARTESIAN_POINT('Ctrl Pts',(3.7583820388737,21.4249999999244,11.5671105274568));
#287012=CARTESIAN_POINT('Ctrl Pts',(7.51676407774743,21.5749999999238,10.3459381770588));
#287013=CARTESIAN_POINT('Ctrl Pts',(9.83957192047852,21.7249999999232,7.14886745759505));
#287014=CARTESIAN_POINT('Ctrl Pts',(12.1623797632096,21.8749999999226,3.95179673813132));
#287015=CARTESIAN_POINT('Ctrl Pts',(12.1623797632096,22.024999999922,-1.48946194470292E-15));
#287016=CARTESIAN_POINT('Ctrl Pts',(12.1623797632096,22.1749999999214,-3.95179673813132));
#287017=CARTESIAN_POINT('Ctrl Pts',(9.83957192047852,22.3249999999208,-7.14886745759505));
#287018=CARTESIAN_POINT('Ctrl Pts',(7.51676407774743,22.4749999999202,-10.3459381770588));
#287019=CARTESIAN_POINT('Ctrl Pts',(3.7583820388737,22.6249999999196,-11.5671105274568));
#287020=CARTESIAN_POINT('Ctrl Pts',(-2.63768727909193E-14,22.774999999919,
-12.7882828778549));
#287021=CARTESIAN_POINT('Ctrl Pts',(-3.75838203887375,22.9249999999184,
-11.5671105274568));
#287022=CARTESIAN_POINT('Ctrl Pts',(-7.51676407774748,23.0749999999178,
-10.3459381770588));
#287023=CARTESIAN_POINT('Ctrl Pts',(-9.83957192047857,23.2249999999172,
-7.14886745759505));
#287024=CARTESIAN_POINT('Ctrl Pts',(-12.1623797632097,23.3749999999166,
-3.95179673813132));
#287025=CARTESIAN_POINT('Ctrl Pts',(-12.1623797632097,23.524999999916,2.97892388940585E-15));
#287026=CARTESIAN_POINT('Ctrl Pts',(-12.1623797632097,23.6749999999154,
3.95179673813133));
#287027=CARTESIAN_POINT('Ctrl Pts',(-9.83957192047857,23.8249999999148,
7.14886745759505));
#287028=CARTESIAN_POINT('Ctrl Pts',(-7.51676407774748,23.9749999999142,
10.3459381770588));
#287029=CARTESIAN_POINT('Ctrl Pts',(-3.75838203887375,24.1249999999136,
11.5671105274568));
#287030=CARTESIAN_POINT('Ctrl Pts',(-2.4108501488159E-14,24.274999999913,
12.7882828778549));
#287031=CARTESIAN_POINT('Ctrl Pts',(3.7583820388737,24.4249999999124,11.5671105274568));
#287032=CARTESIAN_POINT('Ctrl Pts',(7.51676407774743,24.5749999999118,10.3459381770588));
#287033=CARTESIAN_POINT('Ctrl Pts',(9.83957192047852,24.7249999999112,7.14886745759505));
#287034=CARTESIAN_POINT('Ctrl Pts',(12.1623797632096,24.8749999999106,3.95179673813132));
#287035=CARTESIAN_POINT('Ctrl Pts',(12.1623797632096,25.02499999991,-1.48946194470292E-15));
#287036=CARTESIAN_POINT('Ctrl Pts',(12.1623797632096,25.1749999999094,-3.95179673813132));
#287037=CARTESIAN_POINT('Ctrl Pts',(9.83957192047852,25.3249999999088,-7.14886745759505));
#287038=CARTESIAN_POINT('Ctrl Pts',(7.51676407774743,25.4749999999082,-10.3459381770588));
#287039=CARTESIAN_POINT('Ctrl Pts',(3.7583820388737,25.6249999999076,-11.5671105274568));
#287040=CARTESIAN_POINT('Ctrl Pts',(-2.81045820625811E-14,25.774999999907,
-12.7882828778549));
#287041=CARTESIAN_POINT('Ctrl Pts',(-3.75838203887376,25.9249999999064,
-11.5671105274568));
#287042=CARTESIAN_POINT('Ctrl Pts',(-7.51676407774749,26.0749999999058,
-10.3459381770588));
#287043=CARTESIAN_POINT('Ctrl Pts',(-9.83957192047857,26.2249999999052,
-7.14886745759505));
#287044=CARTESIAN_POINT('Ctrl Pts',(-12.1623797632097,26.3749999999046,
-3.95179673813132));
#287045=CARTESIAN_POINT('Ctrl Pts',(-12.1623797632097,26.524999999904,2.97892388940585E-15));
#287046=CARTESIAN_POINT('Ctrl Pts',(-12.1623797632097,26.6749999999034,
3.95179673813133));
#287047=CARTESIAN_POINT('Ctrl Pts',(-9.83957192047857,26.8249999999028,
7.14886745759505));
#287048=CARTESIAN_POINT('Ctrl Pts',(-7.51676407774748,26.9749999999022,
10.3459381770588));
#287049=CARTESIAN_POINT('Ctrl Pts',(-3.75838203887375,27.1249999999016,
11.5671105274568));
#287050=CARTESIAN_POINT('Ctrl Pts',(-2.58362107598209E-14,27.274999999901,
12.7882828778549));
#287051=CARTESIAN_POINT('Ctrl Pts',(3.7583820388737,27.4249999999004,11.5671105274568));
#287052=CARTESIAN_POINT('Ctrl Pts',(7.51676407774743,27.5749999998998,10.3459381770588));
#287053=CARTESIAN_POINT('Ctrl Pts',(9.83957192047852,27.7249999998992,7.14886745759505));
#287054=CARTESIAN_POINT('Ctrl Pts',(12.1623797632096,27.8749999998986,3.95179673813132));
#287055=CARTESIAN_POINT('Ctrl Pts',(12.1623797632096,28.024999999898,-1.48946194470292E-15));
#287056=CARTESIAN_POINT('Ctrl Pts',(12.1623797632096,28.1749999998974,-3.95179673813132));
#287057=CARTESIAN_POINT('Ctrl Pts',(9.83957192047852,28.3249999998968,-7.14886745759505));
#287058=CARTESIAN_POINT('Ctrl Pts',(7.51676407774743,28.4749999998962,-10.3459381770588));
#287059=CARTESIAN_POINT('Ctrl Pts',(3.7583820388737,28.6249999998956,-11.5671105274568));
#287060=CARTESIAN_POINT('Ctrl Pts',(-2.9832291334243E-14,28.774999999895,
-12.7882828778549));
#287061=CARTESIAN_POINT('Ctrl Pts',(-3.75838203887376,28.9249999998944,
-11.5671105274568));
#287062=CARTESIAN_POINT('Ctrl Pts',(-7.51676407774749,29.0749999998938,
-10.3459381770588));
#287063=CARTESIAN_POINT('Ctrl Pts',(-9.83957192047858,29.2249999998932,
-7.14886745759505));
#287064=CARTESIAN_POINT('Ctrl Pts',(-12.1623797632097,29.3749999998926,
-3.95179673813132));
#287065=CARTESIAN_POINT('Ctrl Pts',(-12.1623797632097,29.524999999892,2.97892388940585E-15));
#287066=CARTESIAN_POINT('Ctrl Pts',(-12.1623797632097,29.6749999998914,
3.95179673813133));
#287067=CARTESIAN_POINT('Ctrl Pts',(-9.83957192047858,29.8249999998908,
7.14886745759505));
#287068=CARTESIAN_POINT('Ctrl Pts',(-7.51676407774748,29.9749999998902,
10.3459381770588));
#287069=CARTESIAN_POINT('Ctrl Pts',(-3.75838203887376,30.1249999998896,
11.5671105274568));
#287070=CARTESIAN_POINT('Ctrl Pts',(-2.75639200314827E-14,30.274999999889,
12.7882828778549));
#287071=CARTESIAN_POINT('Ctrl Pts',(3.7583820388737,30.4249999998884,11.5671105274568));
#287072=CARTESIAN_POINT('Ctrl Pts',(7.51676407774743,30.5749999998878,10.3459381770588));
#287073=CARTESIAN_POINT('Ctrl Pts',(9.83957192047852,30.7249999998872,7.14886745759505));
#287074=CARTESIAN_POINT('Ctrl Pts',(12.1623797632096,30.8749999998866,3.95179673813132));
#287075=CARTESIAN_POINT('Ctrl Pts',(12.1623797632096,31.024999999886,-1.48946194470292E-15));
#287076=CARTESIAN_POINT('Ctrl Pts',(12.1623797632096,31.1749999998854,-3.95179673813132));
#287077=CARTESIAN_POINT('Ctrl Pts',(9.83957192047852,31.3249999998848,-7.14886745759505));
#287078=CARTESIAN_POINT('Ctrl Pts',(7.51676407774742,31.4749999998842,-10.3459381770588));
#287079=CARTESIAN_POINT('Ctrl Pts',(3.7583820388737,31.6249999998836,-11.5671105274568));
#287080=CARTESIAN_POINT('Ctrl Pts',(-3.15600006059048E-14,31.774999999883,
-12.7882828778549));
#287081=CARTESIAN_POINT('Ctrl Pts',(-3.75838203887376,31.9249999998824,
-11.5671105274568));
#287082=CARTESIAN_POINT('Ctrl Pts',(-7.51676407774749,32.0749999998818,
-10.3459381770588));
#287083=CARTESIAN_POINT('Ctrl Pts',(-9.83957192047858,32.2249999998812,
-7.14886745759505));
#287084=CARTESIAN_POINT('Ctrl Pts',(-12.1623797632097,32.3749999998806,
-3.95179673813132));
#287085=CARTESIAN_POINT('Ctrl Pts',(-12.1623797632097,32.52499999988,2.97892388940585E-15));
#287086=CARTESIAN_POINT('Ctrl Pts',(-12.1623797632097,32.6749999998794,
3.95179673813133));
#287087=CARTESIAN_POINT('Ctrl Pts',(-9.83957192047858,32.8249999998788,
7.14886745759505));
#287088=CARTESIAN_POINT('Ctrl Pts',(-7.51676407774749,32.9749999998782,
10.3459381770588));
#287089=CARTESIAN_POINT('Ctrl Pts',(-3.75838203887376,33.1249999998776,
11.5671105274568));
#287090=CARTESIAN_POINT('Ctrl Pts',(-2.92916293031446E-14,33.274999999877,
12.7882828778549));
#287091=CARTESIAN_POINT('Ctrl Pts',(3.7583820388737,33.4249999998764,11.5671105274568));
#287092=CARTESIAN_POINT('Ctrl Pts',(7.51676407774743,33.5749999998758,10.3459381770588));
#287093=CARTESIAN_POINT('Ctrl Pts',(9.83957192047852,33.7249999998752,7.14886745759505));
#287094=CARTESIAN_POINT('Ctrl Pts',(12.1623797632096,33.8749999998746,3.95179673813132));
#287095=CARTESIAN_POINT('Ctrl Pts',(12.1623797632096,34.024999999874,-1.48946194470292E-15));
#287096=CARTESIAN_POINT('Ctrl Pts',(12.1623797632096,34.1749999998734,-3.95179673813132));
#287097=CARTESIAN_POINT('Ctrl Pts',(9.83957192047851,34.3249999998728,-7.14886745759505));
#287098=CARTESIAN_POINT('Ctrl Pts',(7.51676407774742,34.4749999998722,-10.3459381770588));
#287099=CARTESIAN_POINT('Ctrl Pts',(3.7583820388737,34.6249999998716,-11.5671105274568));
#287100=CARTESIAN_POINT('Ctrl Pts',(-3.32877098775667E-14,34.774999999871,
-12.7882828778549));
#287101=CARTESIAN_POINT('Ctrl Pts',(-3.75838203887376,34.9249999998704,
-11.5671105274568));
#287102=CARTESIAN_POINT('Ctrl Pts',(-7.51676407774749,35.0749999998698,
-10.3459381770588));
#287103=CARTESIAN_POINT('Ctrl Pts',(-9.83957192047858,35.2249999998692,
-7.14886745759505));
#287104=CARTESIAN_POINT('Ctrl Pts',(-12.1623797632097,35.3749999998686,
-3.95179673813132));
#287105=CARTESIAN_POINT('Ctrl Pts',(-12.1623797632097,35.524999999868,2.97892388940585E-15));
#287106=CARTESIAN_POINT('Ctrl Pts',(-12.1623797632097,35.6749999998674,
3.95179673813133));
#287107=CARTESIAN_POINT('Ctrl Pts',(-9.83957192047858,35.8249999998668,
7.14886745759505));
#287108=CARTESIAN_POINT('Ctrl Pts',(-7.51676407774749,35.9749999998662,
10.3459381770588));
#287109=CARTESIAN_POINT('Ctrl Pts',(-3.75838203887376,36.1249999998656,
11.5671105274568));
#287110=CARTESIAN_POINT('Ctrl Pts',(-3.10193385748064E-14,36.274999999865,
12.7882828778549));
#287111=CARTESIAN_POINT('Ctrl Pts',(3.7583820388737,36.4249999998644,11.5671105274568));
#287112=CARTESIAN_POINT('Ctrl Pts',(7.51676407774742,36.5749999998638,10.3459381770588));
#287113=CARTESIAN_POINT('Ctrl Pts',(9.83957192047851,36.7249999998632,7.14886745759505));
#287114=CARTESIAN_POINT('Ctrl Pts',(12.1623797632096,36.8749999998626,3.95179673813132));
#287115=CARTESIAN_POINT('Ctrl Pts',(12.1623797632096,37.024999999862,-1.48946194470292E-15));
#287116=CARTESIAN_POINT('Ctrl Pts',(12.1623797632096,37.1749999998614,-3.95179673813132));
#287117=CARTESIAN_POINT('Ctrl Pts',(9.83957192047851,37.3249999998608,-7.14886745759505));
#287118=CARTESIAN_POINT('Ctrl Pts',(7.51676407774742,37.4749999998602,-10.3459381770588));
#287119=CARTESIAN_POINT('Ctrl Pts',(3.75838203887369,37.6249999998596,-11.5671105274568));
#287120=CARTESIAN_POINT('Ctrl Pts',(-3.50154191492285E-14,37.774999999859,
-12.7882828778549));
#287121=CARTESIAN_POINT('Ctrl Pts',(-3.75838203887376,37.9249999998584,
-11.5671105274568));
#287122=CARTESIAN_POINT('Ctrl Pts',(-7.51676407774749,38.0749999998578,
-10.3459381770588));
#287123=CARTESIAN_POINT('Ctrl Pts',(-9.83957192047858,38.2249999998572,
-7.14886745759505));
#287124=CARTESIAN_POINT('Ctrl Pts',(-12.1623797632097,38.3749999998566,
-3.95179673813132));
#287125=CARTESIAN_POINT('Ctrl Pts',(-12.1623797632097,38.524999999856,2.97892388940585E-15));
#287126=CARTESIAN_POINT('Ctrl Pts',(-12.1623797632097,38.6749999998554,
3.95179673813133));
#287127=CARTESIAN_POINT('Ctrl Pts',(-9.83957192047858,38.8249999998548,
7.14886745759505));
#287128=CARTESIAN_POINT('Ctrl Pts',(-7.51676407774749,38.9749999998542,
10.3459381770588));
#287129=CARTESIAN_POINT('Ctrl Pts',(-3.75838203887376,39.1249999998536,
11.5671105274568));
#287130=CARTESIAN_POINT('Ctrl Pts',(-3.27470478464682E-14,39.274999999853,
12.7882828778549));
#287131=CARTESIAN_POINT('Ctrl Pts',(3.7583820388737,39.4249999998524,11.5671105274568));
#287132=CARTESIAN_POINT('Ctrl Pts',(7.51676407774742,39.5749999998518,10.3459381770588));
#287133=CARTESIAN_POINT('Ctrl Pts',(9.83957192047851,39.7249999998512,7.14886745759505));
#287134=CARTESIAN_POINT('Ctrl Pts',(12.1623797632096,39.8749999998506,3.95179673813132));
#287135=CARTESIAN_POINT('Ctrl Pts',(12.1623797632096,40.02499999985,-1.48946194470292E-15));
#287136=CARTESIAN_POINT('Ctrl Pts',(12.1623797632096,40.1749999998494,-3.95179673813132));
#287137=CARTESIAN_POINT('Ctrl Pts',(9.83957192047851,40.3249999998488,-7.14886745759505));
#287138=CARTESIAN_POINT('Ctrl Pts',(7.51676407774742,40.4749999998482,-10.3459381770588));
#287139=CARTESIAN_POINT('Ctrl Pts',(3.75838203887369,40.6249999998476,-11.5671105274568));
#287140=CARTESIAN_POINT('Ctrl Pts',(-3.67431284208903E-14,40.774999999847,
-12.7882828778549));
#287141=CARTESIAN_POINT('Ctrl Pts',(-3.75838203887376,40.9249999998464,
-11.5671105274568));
#287142=CARTESIAN_POINT('Ctrl Pts',(-7.51676407774749,41.0749999998458,
-10.3459381770588));
#287143=CARTESIAN_POINT('Ctrl Pts',(-9.83957192047858,41.2249999998452,
-7.14886745759505));
#287144=CARTESIAN_POINT('Ctrl Pts',(-12.1623797632097,41.3749999998446,
-3.95179673813132));
#287145=CARTESIAN_POINT('Ctrl Pts',(-12.1623797632097,41.524999999844,2.97892388940585E-15));
#287146=CARTESIAN_POINT('Ctrl Pts',(-12.1623797632097,41.6749999998434,
3.95179673813133));
#287147=CARTESIAN_POINT('Ctrl Pts',(-9.83957192047858,41.8249999998428,
7.14886745759505));
#287148=CARTESIAN_POINT('Ctrl Pts',(-7.51676407774749,41.9749999998422,
10.3459381770588));
#287149=CARTESIAN_POINT('Ctrl Pts',(-3.75838203887376,42.1249999998416,
11.5671105274568));
#287150=CARTESIAN_POINT('Ctrl Pts',(-3.44747571181301E-14,42.274999999841,
12.7882828778549));
#287151=CARTESIAN_POINT('Ctrl Pts',(3.75838203887369,42.4249999998404,11.5671105274568));
#287152=CARTESIAN_POINT('Ctrl Pts',(7.51676407774742,42.5749999998398,10.3459381770588));
#287153=CARTESIAN_POINT('Ctrl Pts',(9.83957192047851,42.7249999998392,7.14886745759505));
#287154=CARTESIAN_POINT('Ctrl Pts',(12.1623797632096,42.8749999998386,3.95179673813132));
#287155=CARTESIAN_POINT('Ctrl Pts',(12.1623797632096,43.024999999838,-1.48946194470292E-15));
#287156=CARTESIAN_POINT('Ctrl Pts',(12.1623797632096,43.1749999998374,-3.95179673813132));
#287157=CARTESIAN_POINT('Ctrl Pts',(9.83957192047851,43.3249999998368,-7.14886745759505));
#287158=CARTESIAN_POINT('Ctrl Pts',(7.51676407774742,43.4749999998362,-10.3459381770588));
#287159=CARTESIAN_POINT('Ctrl Pts',(3.75838203887369,43.6249999998356,-11.5671105274568));
#287160=CARTESIAN_POINT('Ctrl Pts',(-3.84708376925522E-14,43.774999999835,
-12.7882828778549));
#287161=CARTESIAN_POINT('Ctrl Pts',(-3.75838203887377,43.9249999998344,
-11.5671105274568));
#287162=CARTESIAN_POINT('Ctrl Pts',(-7.51676407774749,44.0749999998338,
-10.3459381770588));
#287163=CARTESIAN_POINT('Ctrl Pts',(-9.83957192047859,44.2249999998332,
-7.14886745759505));
#287164=CARTESIAN_POINT('Ctrl Pts',(-12.1623797632097,44.3749999998326,
-3.95179673813132));
#287165=CARTESIAN_POINT('Ctrl Pts',(-12.1623797632097,44.524999999832,2.97892388940585E-15));
#287166=CARTESIAN_POINT('Ctrl Pts',(-12.1623797632097,44.6749999998314,
3.95179673813133));
#287167=CARTESIAN_POINT('Ctrl Pts',(-9.83957192047859,44.8249999998308,
7.14886745759505));
#287168=CARTESIAN_POINT('Ctrl Pts',(-7.51676407774749,44.9749999998302,
10.3459381770588));
#287169=CARTESIAN_POINT('Ctrl Pts',(-3.75838203887376,45.1249999998296,
11.5671105274568));
#287170=CARTESIAN_POINT('Ctrl Pts',(-3.62024663897919E-14,45.274999999829,
12.7882828778549));
#287171=CARTESIAN_POINT('Ctrl Pts',(3.75838203887369,45.4249999998284,11.5671105274568));
#287172=CARTESIAN_POINT('Ctrl Pts',(7.51676407774742,45.5749999998278,10.3459381770588));
#287173=CARTESIAN_POINT('Ctrl Pts',(9.83957192047851,45.7249999998272,7.14886745759505));
#287174=CARTESIAN_POINT('Ctrl Pts',(12.1623797632096,45.8749999998266,3.95179673813132));
#287175=CARTESIAN_POINT('Ctrl Pts',(12.1623797632096,46.024999999826,-1.48946194470292E-15));
#287176=CARTESIAN_POINT('Ctrl Pts',(12.1623797632096,46.1749999998254,-3.95179673813132));
#287177=CARTESIAN_POINT('Ctrl Pts',(9.83957192047851,46.3249999998248,-7.14886745759505));
#287178=CARTESIAN_POINT('Ctrl Pts',(7.51676407774742,46.4749999998242,-10.3459381770588));
#287179=CARTESIAN_POINT('Ctrl Pts',(3.75838203887369,46.6249999998236,-11.5671105274568));
#287180=CARTESIAN_POINT('Ctrl Pts',(-4.0198546964214E-14,46.774999999823,
-12.7882828778549));
#287181=CARTESIAN_POINT('Ctrl Pts',(-3.75838203887377,46.9249999998224,
-11.5671105274568));
#287182=CARTESIAN_POINT('Ctrl Pts',(-7.5167640777475,47.0749999998218,-10.3459381770588));
#287183=CARTESIAN_POINT('Ctrl Pts',(-9.83957192047859,47.2249999998212,
-7.14886745759505));
#287184=CARTESIAN_POINT('Ctrl Pts',(-12.1623797632097,47.3749999998206,
-3.95179673813132));
#287185=CARTESIAN_POINT('Ctrl Pts',(-12.1623797632097,47.52499999982,2.97892388940585E-15));
#287186=CARTESIAN_POINT('Ctrl Pts',(-12.1623797632097,47.6749999998194,
3.95179673813133));
#287187=CARTESIAN_POINT('Ctrl Pts',(-9.83957192047859,47.8249999998188,
7.14886745759505));
#287188=CARTESIAN_POINT('Ctrl Pts',(-7.51676407774749,47.9749999998182,
10.3459381770588));
#287189=CARTESIAN_POINT('Ctrl Pts',(-3.75838203887377,48.1249999998176,
11.5671105274568));
#287190=CARTESIAN_POINT('Ctrl Pts',(-3.79301756614538E-14,48.274999999817,
12.7882828778549));
#287191=CARTESIAN_POINT('Ctrl Pts',(3.75838203887369,48.4249999998164,11.5671105274568));
#287192=CARTESIAN_POINT('Ctrl Pts',(7.51676407774742,48.5749999998158,10.3459381770588));
#287193=CARTESIAN_POINT('Ctrl Pts',(9.83957192047851,48.7249999998152,7.14886745759505));
#287194=CARTESIAN_POINT('Ctrl Pts',(12.1623797632096,48.8749999998146,3.95179673813132));
#287195=CARTESIAN_POINT('Ctrl Pts',(12.1623797632096,49.024999999814,-1.48946194470292E-15));
#287196=CARTESIAN_POINT('Ctrl Pts',(12.1623797632096,49.1749999998134,-3.95179673813132));
#287197=CARTESIAN_POINT('Ctrl Pts',(9.83957192047851,49.3249999998128,-7.14886745759505));
#287198=CARTESIAN_POINT('Ctrl Pts',(7.51676407774741,49.4749999998122,-10.3459381770588));
#287199=CARTESIAN_POINT('Ctrl Pts',(3.75838203887369,49.6249999998116,-11.5671105274568));
#287200=CARTESIAN_POINT('Ctrl Pts',(-4.19262562358759E-14,49.774999999811,
-12.7882828778549));
#287201=CARTESIAN_POINT('Ctrl Pts',(-3.75838203887377,49.9249999998104,
-11.5671105274568));
#287202=CARTESIAN_POINT('Ctrl Pts',(-7.5167640777475,50.0749999998098,-10.3459381770588));
#287203=CARTESIAN_POINT('Ctrl Pts',(-9.83957192047859,50.2249999998092,
-7.14886745759505));
#287204=CARTESIAN_POINT('Ctrl Pts',(-12.1623797632097,50.3749999998086,
-3.95179673813132));
#287205=CARTESIAN_POINT('Ctrl Pts',(-12.1623797632097,50.524999999808,2.97892388940585E-15));
#287206=CARTESIAN_POINT('Ctrl Pts',(-12.1623797632097,50.6749999998074,
3.95179673813133));
#287207=CARTESIAN_POINT('Ctrl Pts',(-9.83957192047859,50.8249999998068,
7.14886745759505));
#287208=CARTESIAN_POINT('Ctrl Pts',(-7.51676407774749,50.9749999998062,
10.3459381770588));
#287209=CARTESIAN_POINT('Ctrl Pts',(-3.75838203887377,51.1249999998056,
11.5671105274568));
#287210=CARTESIAN_POINT('Ctrl Pts',(-3.96578849331156E-14,51.274999999805,
12.7882828778549));
#287211=CARTESIAN_POINT('Ctrl Pts',(3.75838203887369,51.4249999998044,11.5671105274568));
#287212=CARTESIAN_POINT('Ctrl Pts',(7.51676407774742,51.5749999998038,10.3459381770588));
#287213=CARTESIAN_POINT('Ctrl Pts',(9.83957192047851,51.7249999998032,7.14886745759505));
#287214=CARTESIAN_POINT('Ctrl Pts',(12.1623797632096,51.8749999998026,3.95179673813132));
#287215=CARTESIAN_POINT('Ctrl Pts',(12.1623797632096,52.024999999802,-1.48946194470292E-15));
#287216=CARTESIAN_POINT('Ctrl Pts',(12.1623797632096,52.1749999998014,-3.95179673813132));
#287217=CARTESIAN_POINT('Ctrl Pts',(9.8395719204785,52.3249999998008,-7.14886745759505));
#287218=CARTESIAN_POINT('Ctrl Pts',(7.51676407774741,52.4749999998002,-10.3459381770588));
#287219=CARTESIAN_POINT('Ctrl Pts',(3.75838203887368,52.6249999997996,-11.5671105274568));
#287220=CARTESIAN_POINT('Ctrl Pts',(-4.36539655075377E-14,52.774999999799,
-12.7882828778549));
#287221=CARTESIAN_POINT('Ctrl Pts',(-3.75838203887377,52.9249999997984,
-11.5671105274568));
#287222=CARTESIAN_POINT('Ctrl Pts',(-7.5167640777475,53.0749999997978,-10.3459381770588));
#287223=CARTESIAN_POINT('Ctrl Pts',(-9.83957192047859,53.2249999997972,
-7.14886745759505));
#287224=CARTESIAN_POINT('Ctrl Pts',(-12.1623797632097,53.3749999997966,
-3.95179673813132));
#287225=CARTESIAN_POINT('Ctrl Pts',(-12.1623797632097,53.524999999796,2.97892388940585E-15));
#287226=CARTESIAN_POINT('Ctrl Pts',(-12.1623797632097,53.6749999997954,
3.95179673813133));
#287227=CARTESIAN_POINT('Ctrl Pts',(-9.83957192047859,53.8249999997948,
7.14886745759505));
#287228=CARTESIAN_POINT('Ctrl Pts',(-7.5167640777475,53.9749999997942,10.3459381770588));
#287229=CARTESIAN_POINT('Ctrl Pts',(-3.75838203887377,54.1249999997936,
11.5671105274568));
#287230=CARTESIAN_POINT('Ctrl Pts',(-4.13855942047774E-14,54.274999999793,
12.7882828778549));
#287231=CARTESIAN_POINT('Ctrl Pts',(3.75838203887369,54.4249999997924,11.5671105274568));
#287232=CARTESIAN_POINT('Ctrl Pts',(7.51676407774741,54.5749999997918,10.3459381770588));
#287233=CARTESIAN_POINT('Ctrl Pts',(9.8395719204785,54.7249999997912,7.14886745759505));
#287234=CARTESIAN_POINT('Ctrl Pts',(12.1623797632096,54.8749999997906,3.95179673813132));
#287235=CARTESIAN_POINT('Ctrl Pts',(12.1623797632096,55.02499999979,-1.48946194470292E-15));
#287236=CARTESIAN_POINT('Ctrl Pts',(12.1623797632096,55.1749999997894,-3.95179673813132));
#287237=CARTESIAN_POINT('Ctrl Pts',(9.8395719204785,55.3249999997888,-7.14886745759505));
#287238=CARTESIAN_POINT('Ctrl Pts',(7.51676407774741,55.4749999997882,-10.3459381770588));
#287239=CARTESIAN_POINT('Ctrl Pts',(3.75838203887368,55.6249999997876,-11.5671105274568));
#287240=CARTESIAN_POINT('Ctrl Pts',(-4.53816747791995E-14,55.774999999787,
-12.7882828778549));
#287241=CARTESIAN_POINT('Ctrl Pts',(-3.75838203887377,55.9249999997864,
-11.5671105274568));
#287242=CARTESIAN_POINT('Ctrl Pts',(-7.5167640777475,56.0749999997858,-10.3459381770588));
#287243=CARTESIAN_POINT('Ctrl Pts',(-9.83957192047859,56.2249999997852,
-7.14886745759505));
#287244=CARTESIAN_POINT('Ctrl Pts',(-12.1623797632097,56.3749999997846,
-3.95179673813132));
#287245=CARTESIAN_POINT('Ctrl Pts',(-12.1623797632097,56.524999999784,2.97892388940585E-15));
#287246=CARTESIAN_POINT('Ctrl Pts',(-12.1623797632097,56.6749999997834,
3.95179673813133));
#287247=CARTESIAN_POINT('Ctrl Pts',(-9.83957192047859,56.8249999997828,
7.14886745759505));
#287248=CARTESIAN_POINT('Ctrl Pts',(-7.5167640777475,56.9749999997822,10.3459381770588));
#287249=CARTESIAN_POINT('Ctrl Pts',(-3.75838203887377,57.1249999997816,
11.5671105274568));
#287250=CARTESIAN_POINT('Ctrl Pts',(-4.31133034764393E-14,57.274999999781,
12.7882828778549));
#287251=CARTESIAN_POINT('Ctrl Pts',(3.75838203887368,57.4249999997804,11.5671105274568));
#287252=CARTESIAN_POINT('Ctrl Pts',(7.51676407774741,57.5749999997798,10.3459381770588));
#287253=CARTESIAN_POINT('Ctrl Pts',(9.8395719204785,57.7249999997792,7.14886745759505));
#287254=CARTESIAN_POINT('Ctrl Pts',(12.1623797632096,57.8749999997786,3.95179673813132));
#287255=CARTESIAN_POINT('Ctrl Pts',(12.1623797632096,58.024999999778,-1.48946194470292E-15));
#287256=CARTESIAN_POINT('Ctrl Pts',(12.1623797632096,58.1749999997774,-3.95179673813132));
#287257=CARTESIAN_POINT('Ctrl Pts',(9.8395719204785,58.3249999997768,-7.14886745759505));
#287258=CARTESIAN_POINT('Ctrl Pts',(7.51676407774741,58.4749999997762,-10.3459381770588));
#287259=CARTESIAN_POINT('Ctrl Pts',(3.75838203887368,58.6249999997756,-11.5671105274568));
#287260=CARTESIAN_POINT('Ctrl Pts',(-4.71093840508614E-14,58.774999999775,
-12.7882828778549));
#287261=CARTESIAN_POINT('Ctrl Pts',(-3.75838203887377,58.9249999997744,
-11.5671105274568));
#287262=CARTESIAN_POINT('Ctrl Pts',(-7.5167640777475,59.0749999997738,-10.3459381770588));
#287263=CARTESIAN_POINT('Ctrl Pts',(-9.83957192047859,59.2249999997732,
-7.14886745759505));
#287264=CARTESIAN_POINT('Ctrl Pts',(-12.1623797632097,59.3749999997726,
-3.95179673813132));
#287265=CARTESIAN_POINT('Ctrl Pts',(-12.1623797632097,59.524999999772,2.97892388940585E-15));
#287266=CARTESIAN_POINT('Ctrl Pts',(-12.1623797632097,59.6749999997714,
3.95179673813133));
#287267=CARTESIAN_POINT('Ctrl Pts',(-9.83957192047859,59.8249999997708,
7.14886745759505));
#287268=CARTESIAN_POINT('Ctrl Pts',(-7.5167640777475,59.9749999997702,10.3459381770588));
#287269=CARTESIAN_POINT('Ctrl Pts',(-3.75838203887377,60.1249999997696,
11.5671105274568));
#287270=CARTESIAN_POINT('Ctrl Pts',(-4.48410127481011E-14,60.274999999769,
12.7882828778549));
#287271=CARTESIAN_POINT('Ctrl Pts',(3.75838203887368,60.4249999997684,11.5671105274568));
#287272=CARTESIAN_POINT('Ctrl Pts',(7.51676407774741,60.5749999997678,10.3459381770588));
#287273=CARTESIAN_POINT('Ctrl Pts',(9.8395719204785,60.7249999997672,7.14886745759505));
#287274=CARTESIAN_POINT('Ctrl Pts',(12.1623797632096,60.8749999997666,3.95179673813132));
#287275=CARTESIAN_POINT('Ctrl Pts',(12.1623797632096,61.024999999766,-1.48946194470292E-15));
#287276=CARTESIAN_POINT('Ctrl Pts',(12.1623797632096,61.1749999997654,-3.95179673813132));
#287277=CARTESIAN_POINT('Ctrl Pts',(9.8395719204785,61.3249999997648,-7.14886745759505));
#287278=CARTESIAN_POINT('Ctrl Pts',(7.51676407774741,61.4749999997642,-10.3459381770588));
#287279=CARTESIAN_POINT('Ctrl Pts',(3.75838203887368,61.6249999997636,-11.5671105274568));
#287280=CARTESIAN_POINT('Ctrl Pts',(-4.88370933225232E-14,61.774999999763,
-12.7882828778549));
#287281=CARTESIAN_POINT('Ctrl Pts',(-3.75838203887378,61.9249999997624,
-11.5671105274568));
#287282=CARTESIAN_POINT('Ctrl Pts',(-7.5167640777475,62.0749999997618,-10.3459381770588));
#287283=CARTESIAN_POINT('Ctrl Pts',(-9.8395719204786,62.2249999997612,-7.14886745759505));
#287284=CARTESIAN_POINT('Ctrl Pts',(-12.1623797632097,62.3749999997606,
-3.95179673813132));
#287285=CARTESIAN_POINT('Ctrl Pts',(-12.1623797632097,62.52499999976,2.97892388940585E-15));
#287286=CARTESIAN_POINT('Ctrl Pts',(-12.1623797632097,62.6749999997594,
3.95179673813133));
#287287=CARTESIAN_POINT('Ctrl Pts',(-9.8395719204786,62.8249999997588,7.14886745759505));
#287288=CARTESIAN_POINT('Ctrl Pts',(-7.5167640777475,62.9749999997582,10.3459381770588));
#287289=CARTESIAN_POINT('Ctrl Pts',(-3.75838203887377,63.1249999997576,
11.5671105274568));
#287290=CARTESIAN_POINT('Ctrl Pts',(-4.6568722019763E-14,63.274999999757,
12.7882828778549));
#287291=CARTESIAN_POINT('Ctrl Pts',(3.75838203887368,63.4249999997564,11.5671105274568));
#287292=CARTESIAN_POINT('Ctrl Pts',(7.51676407774741,63.5749999997558,10.3459381770588));
#287293=CARTESIAN_POINT('Ctrl Pts',(9.8395719204785,63.7249999997552,7.14886745759505));
#287294=CARTESIAN_POINT('Ctrl Pts',(12.1623797632096,63.8749999997546,3.95179673813132));
#287295=CARTESIAN_POINT('Ctrl Pts',(12.1623797632096,64.024999999754,-1.48946194470292E-15));
#287296=CARTESIAN_POINT('Ctrl Pts',(12.1623797632096,64.1749999997534,-3.95179673813132));
#287297=CARTESIAN_POINT('Ctrl Pts',(9.8395719204785,64.3249999997528,-7.14886745759505));
#287298=CARTESIAN_POINT('Ctrl Pts',(7.5167640777474,64.4749999997522,-10.3459381770588));
#287299=CARTESIAN_POINT('Ctrl Pts',(3.75838203887368,64.6249999997516,-11.5671105274568));
#287300=CARTESIAN_POINT('Ctrl Pts',(-5.05648025941851E-14,64.774999999751,
-12.7882828778549));
#287301=CARTESIAN_POINT('Ctrl Pts',(-3.75838203887378,64.9249999997504,
-11.5671105274568));
#287302=CARTESIAN_POINT('Ctrl Pts',(-7.51676407774751,65.0749999997498,
-10.3459381770588));
#287303=CARTESIAN_POINT('Ctrl Pts',(-9.8395719204786,65.2249999997492,-7.14886745759505));
#287304=CARTESIAN_POINT('Ctrl Pts',(-12.1623797632097,65.3749999997486,
-3.95179673813132));
#287305=CARTESIAN_POINT('Ctrl Pts',(-12.1623797632097,65.524999999748,2.97892388940585E-15));
#287306=CARTESIAN_POINT('Ctrl Pts',(-12.1623797632097,65.6749999997474,
3.95179673813133));
#287307=CARTESIAN_POINT('Ctrl Pts',(-9.8395719204786,65.8249999997468,7.14886745759505));
#287308=CARTESIAN_POINT('Ctrl Pts',(-7.5167640777475,65.9749999997462,10.3459381770588));
#287309=CARTESIAN_POINT('Ctrl Pts',(-3.75838203887378,66.1249999997456,
11.5671105274568));
#287310=CARTESIAN_POINT('Ctrl Pts',(-4.82964312914248E-14,66.274999999745,
12.7882828778549));
#287311=CARTESIAN_POINT('Ctrl Pts',(3.75838203887368,66.4249999997444,11.5671105274568));
#287312=CARTESIAN_POINT('Ctrl Pts',(7.51676407774741,66.5749999997438,10.3459381770588));
#287313=CARTESIAN_POINT('Ctrl Pts',(9.8395719204785,66.7249999997432,7.14886745759505));
#287314=CARTESIAN_POINT('Ctrl Pts',(12.1623797632096,66.8749999997426,3.95179673813132));
#287315=CARTESIAN_POINT('Ctrl Pts',(12.1623797632096,67.024999999742,-1.48946194470292E-15));
#287316=CARTESIAN_POINT('Ctrl Pts',(12.1623797632096,67.1749999997414,-3.95179673813132));
#287317=CARTESIAN_POINT('Ctrl Pts',(9.8395719204785,67.3249999997408,-7.14886745759505));
#287318=CARTESIAN_POINT('Ctrl Pts',(7.5167640777474,67.4749999997402,-10.3459381770588));
#287319=CARTESIAN_POINT('Ctrl Pts',(3.75838203887368,67.6249999997396,-11.5671105274568));
#287320=CARTESIAN_POINT('Ctrl Pts',(-5.22925118658469E-14,67.774999999739,
-12.7882828778549));
#287321=CARTESIAN_POINT('Ctrl Pts',(-3.75838203887378,67.9249999997384,
-11.5671105274568));
#287322=CARTESIAN_POINT('Ctrl Pts',(-7.51676407774751,68.0749999997378,
-10.3459381770588));
#287323=CARTESIAN_POINT('Ctrl Pts',(-9.8395719204786,68.2249999997372,-7.14886745759505));
#287324=CARTESIAN_POINT('Ctrl Pts',(-12.1623797632097,68.3749999997366,
-3.95179673813132));
#287325=CARTESIAN_POINT('Ctrl Pts',(-12.1623797632097,68.524999999736,2.97892388940585E-15));
#287326=CARTESIAN_POINT('Ctrl Pts',(-12.1623797632097,68.6749999997354,
3.95179673813133));
#287327=CARTESIAN_POINT('Ctrl Pts',(-9.8395719204786,68.8249999997348,7.14886745759505));
#287328=CARTESIAN_POINT('Ctrl Pts',(-7.51676407774751,68.9749999997342,
10.3459381770588));
#287329=CARTESIAN_POINT('Ctrl Pts',(-3.75838203887378,69.1249999997336,
11.5671105274568));
#287330=CARTESIAN_POINT('Ctrl Pts',(-5.00241405630866E-14,69.274999999733,
12.7882828778549));
#287331=CARTESIAN_POINT('Ctrl Pts',(3.75838203887368,69.4249999997324,11.5671105274568));
#287332=CARTESIAN_POINT('Ctrl Pts',(7.5167640777474,69.5749999997318,10.3459381770588));
#287333=CARTESIAN_POINT('Ctrl Pts',(9.8395719204785,69.7249999997312,7.14886745759505));
#287334=CARTESIAN_POINT('Ctrl Pts',(12.1623797632096,69.8749999997306,3.95179673813132));
#287335=CARTESIAN_POINT('Ctrl Pts',(12.1623797632096,70.02499999973,-1.48946194470292E-15));
#287336=CARTESIAN_POINT('Ctrl Pts',(12.1623797632096,70.1749999997294,-3.95179673813132));
#287337=CARTESIAN_POINT('Ctrl Pts',(9.83957192047849,70.3249999997288,-7.14886745759505));
#287338=CARTESIAN_POINT('Ctrl Pts',(7.5167640777474,70.4749999997282,-10.3459381770588));
#287339=CARTESIAN_POINT('Ctrl Pts',(3.75838203887367,70.6249999997276,-11.5671105274568));
#287340=CARTESIAN_POINT('Ctrl Pts',(-5.40202211375087E-14,70.774999999727,
-12.7882828778549));
#287341=CARTESIAN_POINT('Ctrl Pts',(-3.75838203887378,70.9249999997264,
-11.5671105274568));
#287342=CARTESIAN_POINT('Ctrl Pts',(-7.51676407774751,71.0749999997258,
-10.3459381770588));
#287343=CARTESIAN_POINT('Ctrl Pts',(-9.8395719204786,71.2249999997252,-7.14886745759505));
#287344=CARTESIAN_POINT('Ctrl Pts',(-12.1623797632097,71.3749999997246,
-3.95179673813132));
#287345=CARTESIAN_POINT('Ctrl Pts',(-12.1623797632097,71.524999999724,2.97892388940585E-15));
#287346=CARTESIAN_POINT('Ctrl Pts',(-12.1623797632097,71.6749999997234,
3.95179673813133));
#287347=CARTESIAN_POINT('Ctrl Pts',(-9.8395719204786,71.8249999997228,7.14886745759505));
#287348=CARTESIAN_POINT('Ctrl Pts',(-7.51676407774751,71.9749999997222,
10.3459381770588));
#287349=CARTESIAN_POINT('Ctrl Pts',(-3.75838203887378,72.1249999997216,
11.5671105274568));
#287350=CARTESIAN_POINT('Ctrl Pts',(-5.17518498347485E-14,72.274999999721,
12.7882828778549));
#287351=CARTESIAN_POINT('Ctrl Pts',(3.75838203887368,72.4249999997204,11.5671105274568));
#287352=CARTESIAN_POINT('Ctrl Pts',(7.5167640777474,72.5749999997198,10.3459381770588));
#287353=CARTESIAN_POINT('Ctrl Pts',(9.83957192047849,72.7249999997192,7.14886745759505));
#287354=CARTESIAN_POINT('Ctrl Pts',(12.1623797632096,72.8749999997186,3.95179673813132));
#287355=CARTESIAN_POINT('Ctrl Pts',(12.1623797632096,73.024999999718,-1.48946194470292E-15));
#287356=CARTESIAN_POINT('Ctrl Pts',(12.1623797632096,73.1749999997174,-3.95179673813132));
#287357=CARTESIAN_POINT('Ctrl Pts',(9.83957192047849,73.3249999997168,-7.14886745759505));
#287358=CARTESIAN_POINT('Ctrl Pts',(7.5167640777474,73.4749999997162,-10.3459381770588));
#287359=CARTESIAN_POINT('Ctrl Pts',(3.75838203887367,73.6249999997156,-11.5671105274568));
#287360=CARTESIAN_POINT('Ctrl Pts',(-5.57479304091706E-14,73.774999999715,
-12.7882828778549));
#287361=CARTESIAN_POINT('Ctrl Pts',(-3.75838203887378,73.9249999997144,
-11.5671105274568));
#287362=CARTESIAN_POINT('Ctrl Pts',(-7.51676407774751,74.0749999997138,
-10.3459381770588));
#287363=CARTESIAN_POINT('Ctrl Pts',(-9.8395719204786,74.2249999997132,-7.14886745759505));
#287364=CARTESIAN_POINT('Ctrl Pts',(-12.1623797632097,74.3749999997126,
-3.95179673813132));
#287365=CARTESIAN_POINT('Ctrl Pts',(-12.1623797632097,74.524999999712,2.97892388940585E-15));
#287366=CARTESIAN_POINT('Ctrl Pts',(-12.1623797632097,74.6749999997114,
3.95179673813133));
#287367=CARTESIAN_POINT('Ctrl Pts',(-9.8395719204786,74.8249999997108,7.14886745759505));
#287368=CARTESIAN_POINT('Ctrl Pts',(-7.51676407774751,74.9749999997102,
10.3459381770588));
#287369=CARTESIAN_POINT('Ctrl Pts',(-3.75838203887378,75.1249999997096,
11.5671105274568));
#287370=CARTESIAN_POINT('Ctrl Pts',(-5.34795591064103E-14,75.274999999709,
12.7882828778549));
#287371=CARTESIAN_POINT('Ctrl Pts',(3.75838203887367,75.4249999997084,11.5671105274568));
#287372=CARTESIAN_POINT('Ctrl Pts',(7.5167640777474,75.5749999997078,10.3459381770588));
#287373=CARTESIAN_POINT('Ctrl Pts',(9.83957192047849,75.7249999997072,7.14886745759505));
#287374=CARTESIAN_POINT('Ctrl Pts',(12.1623797632096,75.8749999997066,3.95179673813132));
#287375=CARTESIAN_POINT('Ctrl Pts',(12.1623797632096,76.024999999706,-1.48946194470292E-15));
#287376=CARTESIAN_POINT('Ctrl Pts',(12.1623797632096,76.1749999997054,-3.95179673813132));
#287377=CARTESIAN_POINT('Ctrl Pts',(9.83957192047849,76.3249999997048,-7.14886745759505));
#287378=CARTESIAN_POINT('Ctrl Pts',(7.5167640777474,76.4749999997042,-10.3459381770588));
#287379=CARTESIAN_POINT('Ctrl Pts',(3.75838203887367,76.6249999997036,-11.5671105274568));
#287380=CARTESIAN_POINT('Ctrl Pts',(-5.74756396808324E-14,76.774999999703,
-12.7882828778549));
#287381=CARTESIAN_POINT('Ctrl Pts',(-3.75838203887379,76.9249999997024,
-11.5671105274568));
#287382=CARTESIAN_POINT('Ctrl Pts',(-7.51676407774751,77.0749999997018,
-10.3459381770588));
#287383=CARTESIAN_POINT('Ctrl Pts',(-9.8395719204786,77.2249999997012,-7.14886745759505));
#287384=CARTESIAN_POINT('Ctrl Pts',(-12.1623797632097,77.3749999997006,
-3.95179673813132));
#287385=CARTESIAN_POINT('Ctrl Pts',(-12.1623797632097,77.5249999997,2.97892388940585E-15));
#287386=CARTESIAN_POINT('Ctrl Pts',(-12.1623797632097,77.6749999996994,
3.95179673813133));
#287387=CARTESIAN_POINT('Ctrl Pts',(-9.8395719204786,77.8249999996988,7.14886745759505));
#287388=CARTESIAN_POINT('Ctrl Pts',(-7.51676407774751,77.9749999996982,
10.3459381770588));
#287389=CARTESIAN_POINT('Ctrl Pts',(-3.75838203887378,78.1249999996976,
11.5671105274568));
#287390=CARTESIAN_POINT('Ctrl Pts',(-5.52072683780721E-14,78.274999999697,
12.7882828778549));
#287391=CARTESIAN_POINT('Ctrl Pts',(3.75838203887367,78.4249999996964,11.5671105274568));
#287392=CARTESIAN_POINT('Ctrl Pts',(7.5167640777474,78.5749999996958,10.3459381770588));
#287393=CARTESIAN_POINT('Ctrl Pts',(9.83957192047849,78.7249999996952,7.14886745759505));
#287394=CARTESIAN_POINT('Ctrl Pts',(12.1623797632096,78.8749999996946,3.95179673813132));
#287395=CARTESIAN_POINT('Ctrl Pts',(12.1623797632096,79.024999999694,-1.48946194470292E-15));
#287396=CARTESIAN_POINT('Ctrl Pts',(12.1623797632096,79.1749999996934,-3.95179673813132));
#287397=CARTESIAN_POINT('Ctrl Pts',(9.83957192047849,79.3249999996928,-7.14886745759505));
#287398=CARTESIAN_POINT('Ctrl Pts',(7.5167640777474,79.4749999996922,-10.3459381770588));
#287399=CARTESIAN_POINT('Ctrl Pts',(3.75838203887367,79.6249999996916,-11.5671105274568));
#287400=CARTESIAN_POINT('Ctrl Pts',(-5.92033489524943E-14,79.774999999691,
-12.7882828778549));
#287401=CARTESIAN_POINT('Ctrl Pts',(-3.75838203887379,79.9249999996904,
-11.5671105274568));
#287402=CARTESIAN_POINT('Ctrl Pts',(-7.51676407774751,80.0749999996898,
-10.3459381770588));
#287403=CARTESIAN_POINT('Ctrl Pts',(-9.83957192047861,80.2249999996892,
-7.14886745759505));
#287404=CARTESIAN_POINT('Ctrl Pts',(-12.1623797632097,80.3749999996886,
-3.95179673813132));
#287405=CARTESIAN_POINT('Ctrl Pts',(-12.1623797632097,80.524999999688,2.97892388940585E-15));
#287406=CARTESIAN_POINT('Ctrl Pts',(-12.1623797632097,80.6749999996874,
3.95179673813133));
#287407=CARTESIAN_POINT('Ctrl Pts',(-9.83957192047861,80.8249999996868,
7.14886745759505));
#287408=CARTESIAN_POINT('Ctrl Pts',(-7.51676407774751,80.9749999996862,
10.3459381770588));
#287409=CARTESIAN_POINT('Ctrl Pts',(-3.75838203887378,81.1249999996856,
11.5671105274568));
#287410=CARTESIAN_POINT('Ctrl Pts',(-5.6934977649734E-14,81.274999999685,
12.7882828778549));
#287411=CARTESIAN_POINT('Ctrl Pts',(3.75838203887367,81.4249999996844,11.5671105274568));
#287412=CARTESIAN_POINT('Ctrl Pts',(7.5167640777474,81.5749999996838,10.3459381770588));
#287413=CARTESIAN_POINT('Ctrl Pts',(9.83957192047849,81.7249999996832,7.14886745759505));
#287414=CARTESIAN_POINT('Ctrl Pts',(12.1623797632096,81.8749999996826,3.95179673813132));
#287415=CARTESIAN_POINT('Ctrl Pts',(12.1623797632096,82.024999999682,-1.48946194470292E-15));
#287416=CARTESIAN_POINT('Ctrl Pts',(12.1623797632096,82.1749999996814,-3.95179673813132));
#287417=CARTESIAN_POINT('Ctrl Pts',(9.83957192047849,82.3249999996808,-7.14886745759505));
#287418=CARTESIAN_POINT('Ctrl Pts',(7.5167640777474,82.4749999996802,-10.3459381770588));
#287419=CARTESIAN_POINT('Ctrl Pts',(3.75838203887367,82.6249999996796,-11.5671105274568));
#287420=CARTESIAN_POINT('Ctrl Pts',(-6.09310582241561E-14,82.774999999679,
-12.7882828778549));
#287421=CARTESIAN_POINT('Ctrl Pts',(-3.75838203887379,82.9249999996784,
-11.5671105274568));
#287422=CARTESIAN_POINT('Ctrl Pts',(-7.51676407774752,83.0749999996778,
-10.3459381770588));
#287423=CARTESIAN_POINT('Ctrl Pts',(-9.83957192047861,83.2249999996772,
-7.14886745759505));
#287424=CARTESIAN_POINT('Ctrl Pts',(-12.1623797632097,83.3749999996766,
-3.95179673813132));
#287425=CARTESIAN_POINT('Ctrl Pts',(-12.1623797632097,83.524999999676,2.97892388940585E-15));
#287426=CARTESIAN_POINT('Ctrl Pts',(-12.1623797632097,83.6749999996754,
3.95179673813133));
#287427=CARTESIAN_POINT('Ctrl Pts',(-9.83957192047861,83.8249999996748,
7.14886745759505));
#287428=CARTESIAN_POINT('Ctrl Pts',(-7.51676407774751,83.9749999996742,
10.3459381770588));
#287429=CARTESIAN_POINT('Ctrl Pts',(-3.75838203887379,84.1249999996736,
11.5671105274568));
#287430=CARTESIAN_POINT('Ctrl Pts',(-5.86626869213958E-14,84.274999999673,
12.7882828778549));
#287431=CARTESIAN_POINT('Ctrl Pts',(3.75838203887367,84.4249999996724,11.5671105274568));
#287432=CARTESIAN_POINT('Ctrl Pts',(7.5167640777474,84.5749999996718,10.3459381770588));
#287433=CARTESIAN_POINT('Ctrl Pts',(9.83957192047849,84.7249999996712,7.14886745759505));
#287434=CARTESIAN_POINT('Ctrl Pts',(12.1623797632096,84.8749999996706,3.95179673813132));
#287435=CARTESIAN_POINT('Ctrl Pts',(12.1623797632096,85.02499999967,-1.48946194470292E-15));
#287436=CARTESIAN_POINT('Ctrl Pts',(12.1623797632096,85.1749999996694,-3.95179673813132));
#287437=CARTESIAN_POINT('Ctrl Pts',(9.83957192047849,85.3249999996688,-7.14886745759505));
#287438=CARTESIAN_POINT('Ctrl Pts',(7.51676407774739,85.4749999996682,-10.3459381770588));
#287439=CARTESIAN_POINT('Ctrl Pts',(3.75838203887367,85.6249999996676,-11.5671105274568));
#287440=CARTESIAN_POINT('Ctrl Pts',(-6.26587674958179E-14,85.774999999667,
-12.7882828778549));
#287441=CARTESIAN_POINT('Ctrl Pts',(-3.75838203887379,85.9249999996664,
-11.5671105274568));
#287442=CARTESIAN_POINT('Ctrl Pts',(-7.51676407774752,86.0749999996658,
-10.3459381770588));
#287443=CARTESIAN_POINT('Ctrl Pts',(-9.83957192047861,86.2249999996652,
-7.14886745759505));
#287444=CARTESIAN_POINT('Ctrl Pts',(-12.1623797632097,86.3749999996646,
-3.95179673813132));
#287445=CARTESIAN_POINT('Ctrl Pts',(-12.1623797632097,86.524999999664,2.97892388940585E-15));
#287446=CARTESIAN_POINT('Ctrl Pts',(-12.1623797632097,86.6749999996634,
3.95179673813133));
#287447=CARTESIAN_POINT('Ctrl Pts',(-9.83957192047861,86.8249999996628,
7.14886745759505));
#287448=CARTESIAN_POINT('Ctrl Pts',(-7.51676407774752,86.9749999996622,
10.3459381770588));
#287449=CARTESIAN_POINT('Ctrl Pts',(-3.75838203887379,87.1249999996616,
11.5671105274568));
#287450=CARTESIAN_POINT('Ctrl Pts',(-6.03903961930577E-14,87.274999999661,
12.7882828778549));
#287451=CARTESIAN_POINT('Ctrl Pts',(3.75838203887367,87.4249999996604,11.5671105274568));
#287452=CARTESIAN_POINT('Ctrl Pts',(7.5167640777474,87.5749999996598,10.3459381770588));
#287453=CARTESIAN_POINT('Ctrl Pts',(9.83957192047849,87.7249999996592,7.14886745759505));
#287454=CARTESIAN_POINT('Ctrl Pts',(12.1623797632096,87.8749999996586,3.95179673813132));
#287455=CARTESIAN_POINT('Ctrl Pts',(12.1623797632096,88.024999999658,-1.48946194470292E-15));
#287456=CARTESIAN_POINT('Ctrl Pts',(12.1623797632096,88.1749999996574,-3.95179673813132));
#287457=CARTESIAN_POINT('Ctrl Pts',(9.83957192047849,88.3249999996568,-7.14886745759505));
#287458=CARTESIAN_POINT('Ctrl Pts',(7.51676407774739,88.4749999996562,-10.3459381770588));
#287459=CARTESIAN_POINT('Ctrl Pts',(3.75838203887366,88.6249999996556,-11.5671105274568));
#287460=CARTESIAN_POINT('Ctrl Pts',(-6.43864767674798E-14,88.774999999655,
-12.7882828778549));
#287461=CARTESIAN_POINT('Ctrl Pts',(-3.75838203887379,88.9249999996544,
-11.5671105274568));
#287462=CARTESIAN_POINT('Ctrl Pts',(-7.51676407774752,89.0749999996538,
-10.3459381770588));
#287463=CARTESIAN_POINT('Ctrl Pts',(-9.83957192047861,89.2249999996532,
-7.14886745759505));
#287464=CARTESIAN_POINT('Ctrl Pts',(-12.1623797632097,89.3749999996526,
-3.95179673813132));
#287465=CARTESIAN_POINT('Ctrl Pts',(-12.1623797632097,89.524999999652,2.97892388940585E-15));
#287466=CARTESIAN_POINT('Ctrl Pts',(-12.1623797632097,89.6749999996514,
3.95179673813133));
#287467=CARTESIAN_POINT('Ctrl Pts',(-9.83957192047861,89.8249999996508,
7.14886745759505));
#287468=CARTESIAN_POINT('Ctrl Pts',(-7.51676407774752,89.9749999996502,
10.3459381770588));
#287469=CARTESIAN_POINT('Ctrl Pts',(-3.75838203887379,90.1249999996496,
11.5671105274568));
#287470=CARTESIAN_POINT('Ctrl Pts',(-6.21181054647195E-14,90.274999999649,
12.7882828778549));
#287471=CARTESIAN_POINT('Ctrl Pts',(3.75838203887366,90.4249999996484,11.5671105274568));
#287472=CARTESIAN_POINT('Ctrl Pts',(7.51676407774739,90.5749999996478,10.3459381770588));
#287473=CARTESIAN_POINT('Ctrl Pts',(9.83957192047848,90.7249999996472,7.14886745759505));
#287474=CARTESIAN_POINT('Ctrl Pts',(12.1623797632096,90.8749999996466,3.95179673813132));
#287475=CARTESIAN_POINT('Ctrl Pts',(12.1623797632096,91.024999999646,-1.48946194470292E-15));
#287476=CARTESIAN_POINT('Ctrl Pts',(12.1623797632096,91.1749999996454,-3.95179673813132));
#287477=CARTESIAN_POINT('Ctrl Pts',(9.83957192047848,91.3249999996448,-7.14886745759505));
#287478=CARTESIAN_POINT('Ctrl Pts',(7.51676407774739,91.4749999996442,-10.3459381770588));
#287479=CARTESIAN_POINT('Ctrl Pts',(3.75838203887366,91.6249999996436,-11.5671105274568));
#287480=CARTESIAN_POINT('Ctrl Pts',(-6.61141860391416E-14,91.774999999643,
-12.7882828778549));
#287481=CARTESIAN_POINT('Ctrl Pts',(-3.75838203887379,91.9249999996424,
-11.5671105274568));
#287482=CARTESIAN_POINT('Ctrl Pts',(-7.51676407774752,92.0749999996418,
-10.3459381770588));
#287483=CARTESIAN_POINT('Ctrl Pts',(-9.83957192047861,92.2249999996412,
-7.14886745759505));
#287484=CARTESIAN_POINT('Ctrl Pts',(-12.1623797632097,92.3749999996406,
-3.95179673813132));
#287485=CARTESIAN_POINT('Ctrl Pts',(-12.1623797632097,92.52499999964,2.97892388940585E-15));
#287486=CARTESIAN_POINT('Ctrl Pts',(-12.1623797632097,92.6749999996394,
3.95179673813133));
#287487=CARTESIAN_POINT('Ctrl Pts',(-9.83957192047861,92.8249999996388,
7.14886745759505));
#287488=CARTESIAN_POINT('Ctrl Pts',(-7.51676407774752,92.9749999996382,
10.3459381770588));
#287489=CARTESIAN_POINT('Ctrl Pts',(-3.75838203887379,93.1249999996376,
11.5671105274568));
#287490=CARTESIAN_POINT('Ctrl Pts',(-6.38458147363813E-14,93.274999999637,
12.7882828778549));
#287491=CARTESIAN_POINT('Ctrl Pts',(3.75838203887366,93.4249999996364,11.5671105274568));
#287492=CARTESIAN_POINT('Ctrl Pts',(7.51676407774739,93.5749999996358,10.3459381770588));
#287493=CARTESIAN_POINT('Ctrl Pts',(9.83957192047848,93.7249999996352,7.14886745759505));
#287494=CARTESIAN_POINT('Ctrl Pts',(12.1623797632096,93.8749999996346,3.95179673813132));
#287495=CARTESIAN_POINT('Ctrl Pts',(12.1623797632096,94.024999999634,-1.48946194470292E-15));
#287496=CARTESIAN_POINT('Ctrl Pts',(12.1623797632096,94.1749999996334,-3.95179673813132));
#287497=CARTESIAN_POINT('Ctrl Pts',(9.83957192047848,94.3249999996328,-7.14886745759505));
#287498=CARTESIAN_POINT('Ctrl Pts',(7.51676407774739,94.4749999996322,-10.3459381770588));
#287499=CARTESIAN_POINT('Ctrl Pts',(3.75838203887366,94.6249999996316,-11.5671105274568));
#287500=CARTESIAN_POINT('Ctrl Pts',(-6.78418953108034E-14,94.774999999631,
-12.7882828778549));
#287501=CARTESIAN_POINT('Ctrl Pts',(-3.7583820388738,94.9249999996304,-11.5671105274568));
#287502=CARTESIAN_POINT('Ctrl Pts',(-7.51676407774752,95.0749999996298,
-10.3459381770588));
#287503=CARTESIAN_POINT('Ctrl Pts',(-9.83957192047862,95.2249999996292,
-7.14886745759505));
#287504=CARTESIAN_POINT('Ctrl Pts',(-12.1623797632097,95.3749999996286,
-3.95179673813132));
#287505=CARTESIAN_POINT('Ctrl Pts',(-12.1623797632097,95.524999999628,2.97892388940585E-15));
#287506=CARTESIAN_POINT('Ctrl Pts',(-12.1623797632097,95.6749999996274,
3.95179673813133));
#287507=CARTESIAN_POINT('Ctrl Pts',(-9.83957192047862,95.8249999996268,
7.14886745759505));
#287508=CARTESIAN_POINT('Ctrl Pts',(-7.51676407774752,95.9749999996262,
10.3459381770588));
#287509=CARTESIAN_POINT('Ctrl Pts',(-3.75838203887379,96.1249999996256,
11.5671105274568));
#287510=CARTESIAN_POINT('Ctrl Pts',(-6.55735240080432E-14,96.274999999625,
12.7882828778549));
#287511=CARTESIAN_POINT('Ctrl Pts',(3.75838203887366,96.4249999996244,11.5671105274568));
#287512=CARTESIAN_POINT('Ctrl Pts',(7.51676407774739,96.5749999996238,10.3459381770588));
#287513=CARTESIAN_POINT('Ctrl Pts',(9.83957192047848,96.7249999996232,7.14886745759505));
#287514=CARTESIAN_POINT('Ctrl Pts',(12.1623797632096,96.8749999996226,3.95179673813132));
#287515=CARTESIAN_POINT('Ctrl Pts',(12.1623797632096,97.024999999622,-1.48946194470292E-15));
#287516=CARTESIAN_POINT('Ctrl Pts',(12.1623797632096,97.1749999996214,-3.95179673813132));
#287517=CARTESIAN_POINT('Ctrl Pts',(9.83957192047848,97.3249999996208,-7.14886745759505));
#287518=CARTESIAN_POINT('Ctrl Pts',(7.51676407774739,97.4749999996202,-10.3459381770588));
#287519=CARTESIAN_POINT('Ctrl Pts',(3.75838203887366,97.6249999996196,-11.5671105274568));
#287520=CARTESIAN_POINT('Ctrl Pts',(-6.95696045824653E-14,97.774999999619,
-12.7882828778549));
#287521=CARTESIAN_POINT('Ctrl Pts',(-3.7583820388738,97.9249999996184,-11.5671105274568));
#287522=CARTESIAN_POINT('Ctrl Pts',(-7.51676407774752,98.0749999996178,
-10.3459381770588));
#287523=CARTESIAN_POINT('Ctrl Pts',(-9.83957192047862,98.2249999996172,
-7.14886745759505));
#287524=CARTESIAN_POINT('Ctrl Pts',(-12.1623797632097,98.3749999996166,
-3.95179673813132));
#287525=CARTESIAN_POINT('Ctrl Pts',(-12.1623797632097,98.524999999616,2.97892388940585E-15));
#287526=CARTESIAN_POINT('Ctrl Pts',(-12.1623797632097,98.6749999996154,
3.95179673813133));
#287527=CARTESIAN_POINT('Ctrl Pts',(-9.83957192047862,98.8249999996148,
7.14886745759505));
#287528=CARTESIAN_POINT('Ctrl Pts',(-7.51676407774752,98.9749999996142,
10.3459381770588));
#287529=CARTESIAN_POINT('Ctrl Pts',(-3.7583820388738,99.1249999996136,11.5671105274568));
#287530=CARTESIAN_POINT('Ctrl Pts',(-6.7301233279705E-14,99.274999999613,
12.7882828778549));
#287531=CARTESIAN_POINT('Ctrl Pts',(3.75838203887366,99.4249999996124,11.5671105274568));
#287532=CARTESIAN_POINT('Ctrl Pts',(7.51676407774739,99.5749999996118,10.3459381770588));
#287533=CARTESIAN_POINT('Ctrl Pts',(9.83957192047848,99.7249999996112,7.14886745759505));
#287534=CARTESIAN_POINT('Ctrl Pts',(12.1623797632096,99.8749999996106,3.95179673813132));
#287535=CARTESIAN_POINT('Ctrl Pts',(12.1623797632096,100.02499999961,-1.48946194470292E-15));
#287536=CARTESIAN_POINT('Ctrl Pts',(12.1623797632096,100.174999999609,-3.95179673813132));
#287537=CARTESIAN_POINT('Ctrl Pts',(9.83957192047848,100.324999999609,-7.14886745759505));
#287538=CARTESIAN_POINT('Ctrl Pts',(7.51676407774738,100.474999999608,-10.3459381770588));
#287539=CARTESIAN_POINT('Ctrl Pts',(3.75838203887366,100.624999999608,-11.5671105274568));
#287540=CARTESIAN_POINT('Ctrl Pts',(-7.12973138541271E-14,100.774999999607,
-12.7882828778549));
#287541=CARTESIAN_POINT('Ctrl Pts',(-3.7583820388738,100.924999999606,-11.5671105274568));
#287542=CARTESIAN_POINT('Ctrl Pts',(-7.51676407774753,101.074999999606,
-10.3459381770588));
#287543=CARTESIAN_POINT('Ctrl Pts',(-9.83957192047862,101.224999999605,
-7.14886745759505));
#287544=CARTESIAN_POINT('Ctrl Pts',(-12.1623797632097,101.374999999605,
-3.95179673813132));
#287545=CARTESIAN_POINT('Ctrl Pts',(-12.1623797632097,101.524999999604,
2.97892388940585E-15));
#287546=CARTESIAN_POINT('Ctrl Pts',(-12.1623797632097,101.674999999603,
3.95179673813133));
#287547=CARTESIAN_POINT('Ctrl Pts',(-9.83957192047862,101.824999999603,
7.14886745759505));
#287548=CARTESIAN_POINT('Ctrl Pts',(-7.51676407774752,101.974999999602,
10.3459381770588));
#287549=CARTESIAN_POINT('Ctrl Pts',(-3.7583820388738,102.124999999602,11.5671105274568));
#287550=CARTESIAN_POINT('Ctrl Pts',(-6.90289425513669E-14,102.274999999601,
12.7882828778549));
#287551=CARTESIAN_POINT('Ctrl Pts',(3.75838203887366,102.4249999996,11.5671105274568));
#287552=CARTESIAN_POINT('Ctrl Pts',(7.51676407774739,102.5749999996,10.3459381770588));
#287553=CARTESIAN_POINT('Ctrl Pts',(9.83957192047848,102.724999999599,7.14886745759505));
#287554=CARTESIAN_POINT('Ctrl Pts',(12.1623797632096,102.874999999599,3.95179673813132));
#287555=CARTESIAN_POINT('Ctrl Pts',(12.1623797632096,103.024999999598,-1.48946194470292E-15));
#287556=CARTESIAN_POINT('Ctrl Pts',(12.1623797632096,103.174999999597,-3.95179673813132));
#287557=CARTESIAN_POINT('Ctrl Pts',(9.83957192047848,103.324999999597,-7.14886745759505));
#287558=CARTESIAN_POINT('Ctrl Pts',(7.51676407774738,103.474999999596,-10.3459381770588));
#287559=CARTESIAN_POINT('Ctrl Pts',(3.75838203887366,103.624999999596,-11.5671105274568));
#287560=CARTESIAN_POINT('Ctrl Pts',(-7.3025023125789E-14,103.774999999595,
-12.7882828778549));
#287561=CARTESIAN_POINT('Ctrl Pts',(-3.7583820388738,103.924999999594,-11.5671105274568));
#287562=CARTESIAN_POINT('Ctrl Pts',(-7.51676407774753,104.074999999594,
-10.3459381770588));
#287563=CARTESIAN_POINT('Ctrl Pts',(-9.83957192047862,104.224999999593,
-7.14886745759505));
#287564=CARTESIAN_POINT('Ctrl Pts',(-12.1623797632097,104.374999999593,
-3.95179673813132));
#287565=CARTESIAN_POINT('Ctrl Pts',(-12.1623797632097,104.524999999592,
2.97892388940585E-15));
#287566=CARTESIAN_POINT('Ctrl Pts',(-12.1623797632097,104.674999999591,
3.95179673813133));
#287567=CARTESIAN_POINT('Ctrl Pts',(-9.83957192047862,104.824999999591,
7.14886745759505));
#287568=CARTESIAN_POINT('Ctrl Pts',(-7.51676407774753,104.97499999959,10.3459381770588));
#287569=CARTESIAN_POINT('Ctrl Pts',(-3.7583820388738,105.12499999959,11.5671105274568));
#287570=CARTESIAN_POINT('Ctrl Pts',(-7.07566518230287E-14,105.274999999589,
12.7882828778549));
#287571=CARTESIAN_POINT('Ctrl Pts',(3.75838203887366,105.424999999588,11.5671105274568));
#287572=CARTESIAN_POINT('Ctrl Pts',(7.51676407774738,105.574999999588,10.3459381770588));
#287573=CARTESIAN_POINT('Ctrl Pts',(9.83957192047848,105.724999999587,7.14886745759505));
#287574=CARTESIAN_POINT('Ctrl Pts',(12.1623797632096,105.874999999587,3.95179673813132));
#287575=CARTESIAN_POINT('Ctrl Pts',(12.1623797632096,106.024999999586,-1.48946194470292E-15));
#287576=CARTESIAN_POINT('Ctrl Pts',(12.1623797632096,106.174999999585,-3.95179673813132));
#287577=CARTESIAN_POINT('Ctrl Pts',(9.83957192047848,106.324999999585,-7.14886745759505));
#287578=CARTESIAN_POINT('Ctrl Pts',(7.51676407774738,106.474999999584,-10.3459381770588));
#287579=CARTESIAN_POINT('Ctrl Pts',(3.75838203887365,106.624999999584,-11.5671105274568));
#287580=CARTESIAN_POINT('Ctrl Pts',(-7.47527323974508E-14,106.774999999583,
-12.7882828778549));
#287581=CARTESIAN_POINT('Ctrl Pts',(-3.7583820388738,106.924999999582,-11.5671105274568));
#287582=CARTESIAN_POINT('Ctrl Pts',(-7.51676407774753,107.074999999582,
-10.3459381770588));
#287583=CARTESIAN_POINT('Ctrl Pts',(-9.83957192047862,107.224999999581,
-7.14886745759505));
#287584=CARTESIAN_POINT('Ctrl Pts',(-12.1623797632097,107.374999999581,
-3.95179673813132));
#287585=CARTESIAN_POINT('Ctrl Pts',(-12.1623797632097,107.52499999958,2.97892388940585E-15));
#287586=CARTESIAN_POINT('Ctrl Pts',(-12.1623797632097,107.674999999579,
3.95179673813133));
#287587=CARTESIAN_POINT('Ctrl Pts',(-9.83957192047862,107.824999999579,
7.14886745759505));
#287588=CARTESIAN_POINT('Ctrl Pts',(-7.51676407774753,107.974999999578,
10.3459381770588));
#287589=CARTESIAN_POINT('Ctrl Pts',(-3.7583820388738,108.124999999578,11.5671105274568));
#287590=CARTESIAN_POINT('Ctrl Pts',(-7.24843610946905E-14,108.274999999577,
12.7882828778549));
#287591=CARTESIAN_POINT('Ctrl Pts',(3.75838203887366,108.424999999576,11.5671105274568));
#287592=CARTESIAN_POINT('Ctrl Pts',(7.51676407774738,108.574999999576,10.3459381770588));
#287593=CARTESIAN_POINT('Ctrl Pts',(9.83957192047847,108.724999999575,7.14886745759505));
#287594=CARTESIAN_POINT('Ctrl Pts',(12.1623797632096,108.874999999575,3.95179673813132));
#287595=CARTESIAN_POINT('Ctrl Pts',(12.1623797632096,109.024999999574,-1.48946194470292E-15));
#287596=CARTESIAN_POINT('Ctrl Pts',(12.1623797632096,109.174999999573,-3.95179673813132));
#287597=CARTESIAN_POINT('Ctrl Pts',(9.83957192047847,109.324999999573,-7.14886745759505));
#287598=CARTESIAN_POINT('Ctrl Pts',(7.51676407774738,109.474999999572,-10.3459381770588));
#287599=CARTESIAN_POINT('Ctrl Pts',(3.75838203887365,109.624999999572,-11.5671105274568));
#287600=CARTESIAN_POINT('Ctrl Pts',(-7.64804416691126E-14,109.774999999571,
-12.7882828778549));
#287601=CARTESIAN_POINT('Ctrl Pts',(-3.7583820388738,109.92499999957,-11.5671105274568));
#287602=CARTESIAN_POINT('Ctrl Pts',(-7.51676407774753,110.07499999957,-10.3459381770588));
#287603=CARTESIAN_POINT('Ctrl Pts',(-9.83957192047862,110.224999999569,
-7.14886745759505));
#287604=CARTESIAN_POINT('Ctrl Pts',(-12.1623797632097,110.374999999569,
-3.95179673813132));
#287605=CARTESIAN_POINT('Ctrl Pts',(-12.1623797632097,110.524999999568,
2.97892388940585E-15));
#287606=CARTESIAN_POINT('Ctrl Pts',(-12.1623797632097,110.674999999567,
3.95179673813133));
#287607=CARTESIAN_POINT('Ctrl Pts',(-9.83957192047862,110.824999999567,
7.14886745759505));
#287608=CARTESIAN_POINT('Ctrl Pts',(-7.51676407774753,110.974999999566,
10.3459381770588));
#287609=CARTESIAN_POINT('Ctrl Pts',(-3.7583820388738,111.124999999566,11.5671105274568));
#287610=CARTESIAN_POINT('Ctrl Pts',(-7.42120703663524E-14,111.274999999565,
12.7882828778549));
#287611=CARTESIAN_POINT('Ctrl Pts',(3.75838203887365,111.424999999564,11.5671105274568));
#287612=CARTESIAN_POINT('Ctrl Pts',(7.51676407774738,111.574999999564,10.3459381770588));
#287613=CARTESIAN_POINT('Ctrl Pts',(9.83957192047847,111.724999999563,7.14886745759505));
#287614=CARTESIAN_POINT('Ctrl Pts',(12.1623797632096,111.874999999563,3.95179673813132));
#287615=CARTESIAN_POINT('Ctrl Pts',(12.1623797632096,112.024999999562,-1.48946194470292E-15));
#287616=CARTESIAN_POINT('Ctrl Pts',(12.1623797632096,112.174999999561,-3.95179673813132));
#287617=CARTESIAN_POINT('Ctrl Pts',(9.83957192047847,112.324999999561,-7.14886745759505));
#287618=CARTESIAN_POINT('Ctrl Pts',(7.51676407774738,112.47499999956,-10.3459381770588));
#287619=CARTESIAN_POINT('Ctrl Pts',(3.75838203887365,112.62499999956,-11.5671105274568));
#287620=CARTESIAN_POINT('Ctrl Pts',(-7.82081509407745E-14,112.774999999559,
-12.7882828778549));
#287621=CARTESIAN_POINT('Ctrl Pts',(-3.75838203887381,112.924999999558,
-11.5671105274568));
#287622=CARTESIAN_POINT('Ctrl Pts',(-7.51676407774753,113.074999999558,
-10.3459381770588));
#287623=CARTESIAN_POINT('Ctrl Pts',(-9.83957192047863,113.224999999557,
-7.14886745759505));
#287624=CARTESIAN_POINT('Ctrl Pts',(-12.1623797632097,113.374999999557,
-3.95179673813132));
#287625=CARTESIAN_POINT('Ctrl Pts',(-12.1623797632097,113.524999999556,
2.97892388940585E-15));
#287626=CARTESIAN_POINT('Ctrl Pts',(-12.1623797632097,113.674999999555,
3.95179673813133));
#287627=CARTESIAN_POINT('Ctrl Pts',(-9.83957192047863,113.824999999555,
7.14886745759505));
#287628=CARTESIAN_POINT('Ctrl Pts',(-7.51676407774753,113.974999999554,
10.3459381770588));
#287629=CARTESIAN_POINT('Ctrl Pts',(-3.7583820388738,114.124999999554,11.5671105274568));
#287630=CARTESIAN_POINT('Ctrl Pts',(-7.59397796380142E-14,114.274999999553,
12.7882828778549));
#287631=CARTESIAN_POINT('Ctrl Pts',(3.75838203887365,114.424999999552,11.5671105274568));
#287632=CARTESIAN_POINT('Ctrl Pts',(7.51676407774738,114.574999999552,10.3459381770588));
#287633=CARTESIAN_POINT('Ctrl Pts',(9.83957192047847,114.724999999551,7.14886745759505));
#287634=CARTESIAN_POINT('Ctrl Pts',(12.1623797632096,114.874999999551,3.95179673813132));
#287635=CARTESIAN_POINT('Ctrl Pts',(12.1623797632096,115.02499999955,-1.48946194470292E-15));
#287636=CARTESIAN_POINT('Ctrl Pts',(12.1623797632096,115.174999999549,-3.95179673813132));
#287637=CARTESIAN_POINT('Ctrl Pts',(9.83957192047847,115.324999999549,-7.14886745759505));
#287638=CARTESIAN_POINT('Ctrl Pts',(7.51676407774738,115.474999999548,-10.3459381770588));
#287639=CARTESIAN_POINT('Ctrl Pts',(3.75838203887365,115.624999999548,-11.5671105274568));
#287640=CARTESIAN_POINT('Ctrl Pts',(-7.99358602124363E-14,115.774999999547,
-12.7882828778549));
#287641=CARTESIAN_POINT('Ctrl Pts',(-3.75838203887381,115.924999999546,
-11.5671105274568));
#287642=CARTESIAN_POINT('Ctrl Pts',(-7.51676407774754,116.074999999546,
-10.3459381770588));
#287643=CARTESIAN_POINT('Ctrl Pts',(-9.83957192047863,116.224999999545,
-7.14886745759505));
#287644=CARTESIAN_POINT('Ctrl Pts',(-12.1623797632097,116.374999999545,
-3.95179673813132));
#287645=CARTESIAN_POINT('Ctrl Pts',(-12.1623797632097,116.524999999544,
2.97892388940585E-15));
#287646=CARTESIAN_POINT('Ctrl Pts',(-12.1623797632097,116.674999999543,
3.95179673813133));
#287647=CARTESIAN_POINT('Ctrl Pts',(-9.83957192047863,116.824999999543,
7.14886745759505));
#287648=CARTESIAN_POINT('Ctrl Pts',(-7.51676407774753,116.974999999542,
10.3459381770588));
#287649=CARTESIAN_POINT('Ctrl Pts',(-3.75838203887381,117.124999999542,
11.5671105274568));
#287650=CARTESIAN_POINT('Ctrl Pts',(-7.76674889096761E-14,117.274999999541,
12.7882828778549));
#287651=CARTESIAN_POINT('Ctrl Pts',(3.75838203887365,117.42499999954,11.5671105274568));
#287652=CARTESIAN_POINT('Ctrl Pts',(7.51676407774738,117.57499999954,10.3459381770588));
#287653=CARTESIAN_POINT('Ctrl Pts',(9.83957192047847,117.724999999539,7.14886745759505));
#287654=CARTESIAN_POINT('Ctrl Pts',(12.1623797632096,117.874999999539,3.95179673813132));
#287655=CARTESIAN_POINT('Ctrl Pts',(12.1623797632096,118.024999999538,-1.48946194470292E-15));
#287656=CARTESIAN_POINT('Ctrl Pts',(12.1623797632096,118.174999999537,-3.95179673813132));
#287657=CARTESIAN_POINT('Ctrl Pts',(9.83957192047847,118.324999999537,-7.14886745759505));
#287658=CARTESIAN_POINT('Ctrl Pts',(7.51676407774737,118.474999999536,-10.3459381770588));
#287659=CARTESIAN_POINT('Ctrl Pts',(3.75838203887365,118.624999999536,-11.5671105274568));
#287660=CARTESIAN_POINT('Ctrl Pts',(-8.16635694840981E-14,118.774999999535,
-12.7882828778549));
#287661=CARTESIAN_POINT('Ctrl Pts',(-3.75838203887381,118.924999999534,
-11.5671105274568));
#287662=CARTESIAN_POINT('Ctrl Pts',(-7.51676407774754,119.074999999534,
-10.3459381770588));
#287663=CARTESIAN_POINT('Ctrl Pts',(-9.83957192047863,119.224999999533,
-7.14886745759505));
#287664=CARTESIAN_POINT('Ctrl Pts',(-12.1623797632097,119.374999999533,
-3.95179673813132));
#287665=CARTESIAN_POINT('Ctrl Pts',(-12.1623797632097,119.524999999532,
2.97892388940585E-15));
#287666=CARTESIAN_POINT('Ctrl Pts',(-12.1623797632097,119.674999999531,
3.95179673813133));
#287667=CARTESIAN_POINT('Ctrl Pts',(-9.83957192047863,119.824999999531,
7.14886745759505));
#287668=CARTESIAN_POINT('Ctrl Pts',(-7.51676407774754,119.97499999953,10.3459381770588));
#287669=CARTESIAN_POINT('Ctrl Pts',(-3.75838203887381,120.12499999953,11.5671105274568));
#287670=CARTESIAN_POINT('Ctrl Pts',(-7.93951981813379E-14,120.274999999529,
12.7882828778549));
#287671=CARTESIAN_POINT('Ctrl Pts',(3.75838203887365,120.424999999528,11.5671105274568));
#287672=CARTESIAN_POINT('Ctrl Pts',(7.51676407774738,120.574999999528,10.3459381770588));
#287673=CARTESIAN_POINT('Ctrl Pts',(9.83957192047847,120.724999999527,7.14886745759505));
#287674=CARTESIAN_POINT('Ctrl Pts',(12.1623797632096,120.874999999527,3.95179673813132));
#287675=CARTESIAN_POINT('Ctrl Pts',(12.1623797632096,121.024999999526,-1.48946194470292E-15));
#287676=CARTESIAN_POINT('Ctrl Pts',(12.1623797632096,121.174999999525,-3.95179673813132));
#287677=CARTESIAN_POINT('Ctrl Pts',(9.83957192047847,121.324999999525,-7.14886745759505));
#287678=CARTESIAN_POINT('Ctrl Pts',(7.51676407774737,121.474999999524,-10.3459381770588));
#287679=CARTESIAN_POINT('Ctrl Pts',(3.75838203887364,121.624999999524,-11.5671105274568));
#287680=CARTESIAN_POINT('Ctrl Pts',(-8.339127875576E-14,121.774999999523,
-12.7882828778549));
#287681=CARTESIAN_POINT('Ctrl Pts',(-3.75838203887381,121.924999999522,
-11.5671105274568));
#287682=CARTESIAN_POINT('Ctrl Pts',(-7.51676407774754,122.074999999522,
-10.3459381770588));
#287683=CARTESIAN_POINT('Ctrl Pts',(-9.83957192047863,122.224999999521,
-7.14886745759505));
#287684=CARTESIAN_POINT('Ctrl Pts',(-12.1623797632097,122.374999999521,
-3.95179673813132));
#287685=CARTESIAN_POINT('Ctrl Pts',(-12.1623797632097,122.52499999952,2.97892388940585E-15));
#287686=CARTESIAN_POINT('Ctrl Pts',(-12.1623797632097,122.674999999519,
3.95179673813133));
#287687=CARTESIAN_POINT('Ctrl Pts',(-9.83957192047863,122.824999999519,
7.14886745759505));
#287688=CARTESIAN_POINT('Ctrl Pts',(-7.51676407774754,122.974999999518,
10.3459381770588));
#287689=CARTESIAN_POINT('Ctrl Pts',(-3.75838203887381,123.124999999518,
11.5671105274568));
#287690=CARTESIAN_POINT('Ctrl Pts',(-8.11229074529997E-14,123.274999999517,
12.7882828778549));
#287691=CARTESIAN_POINT('Ctrl Pts',(3.75838203887365,123.424999999516,11.5671105274568));
#287692=CARTESIAN_POINT('Ctrl Pts',(7.51676407774737,123.574999999516,10.3459381770588));
#287693=CARTESIAN_POINT('Ctrl Pts',(9.83957192047846,123.724999999515,7.14886745759505));
#287694=CARTESIAN_POINT('Ctrl Pts',(12.1623797632096,123.874999999515,3.95179673813132));
#287695=CARTESIAN_POINT('Ctrl Pts',(12.1623797632096,124.024999999514,-1.48946194470292E-15));
#287696=CARTESIAN_POINT('Ctrl Pts',(12.1623797632096,124.174999999513,-3.95179673813132));
#287697=CARTESIAN_POINT('Ctrl Pts',(9.83957192047846,124.324999999513,-7.14886745759505));
#287698=CARTESIAN_POINT('Ctrl Pts',(7.51676407774737,124.474999999512,-10.3459381770588));
#287699=CARTESIAN_POINT('Ctrl Pts',(3.75838203887364,124.624999999512,-11.5671105274568));
#287700=CARTESIAN_POINT('Ctrl Pts',(-8.51189880274219E-14,124.774999999511,
-12.7882828778549));
#287701=CARTESIAN_POINT('Ctrl Pts',(-3.75838203887381,124.92499999951,-11.5671105274568));
#287702=CARTESIAN_POINT('Ctrl Pts',(-7.51676407774754,125.07499999951,-10.3459381770588));
#287703=CARTESIAN_POINT('Ctrl Pts',(-9.83957192047863,125.224999999509,
-7.14886745759505));
#287704=CARTESIAN_POINT('Ctrl Pts',(-12.1623797632097,125.374999999509,
-3.95179673813132));
#287705=CARTESIAN_POINT('Ctrl Pts',(-12.1623797632097,125.524999999508,
2.97892388940585E-15));
#287706=CARTESIAN_POINT('Ctrl Pts',(-12.1623797632097,125.674999999507,
3.95179673813133));
#287707=CARTESIAN_POINT('Ctrl Pts',(-9.83957192047863,125.824999999507,
7.14886745759505));
#287708=CARTESIAN_POINT('Ctrl Pts',(-7.51676407774754,125.974999999506,
10.3459381770588));
#287709=CARTESIAN_POINT('Ctrl Pts',(-3.75838203887381,126.124999999506,
11.5671105274568));
#287710=CARTESIAN_POINT('Ctrl Pts',(-8.28506167246616E-14,126.274999999505,
12.7882828778549));
#287711=CARTESIAN_POINT('Ctrl Pts',(3.75838203887364,126.424999999504,11.5671105274568));
#287712=CARTESIAN_POINT('Ctrl Pts',(7.51676407774737,126.574999999504,10.3459381770588));
#287713=CARTESIAN_POINT('Ctrl Pts',(9.83957192047846,126.724999999503,7.14886745759505));
#287714=CARTESIAN_POINT('Ctrl Pts',(12.1623797632096,126.874999999503,3.95179673813132));
#287715=CARTESIAN_POINT('Ctrl Pts',(12.1623797632096,127.024999999502,-1.48946194470292E-15));
#287716=CARTESIAN_POINT('Ctrl Pts',(12.1623797632096,127.174999999501,-3.95179673813132));
#287717=CARTESIAN_POINT('Ctrl Pts',(9.83957192047846,127.324999999501,-7.14886745759505));
#287718=CARTESIAN_POINT('Ctrl Pts',(7.51676407774737,127.4749999995,-10.3459381770588));
#287719=CARTESIAN_POINT('Ctrl Pts',(3.75838203887364,127.6249999995,-11.5671105274568));
#287720=CARTESIAN_POINT('Ctrl Pts',(-8.68466972990837E-14,127.774999999499,
-12.7882828778549));
#287721=CARTESIAN_POINT('Ctrl Pts',(-3.75838203887381,127.924999999498,
-11.5671105274568));
#287722=CARTESIAN_POINT('Ctrl Pts',(-7.51676407774754,128.074999999498,
-10.3459381770588));
#287723=CARTESIAN_POINT('Ctrl Pts',(-9.83957192047864,128.224999999497,
-7.14886745759505));
#287724=CARTESIAN_POINT('Ctrl Pts',(-12.1623797632097,128.374999999497,
-3.95179673813132));
#287725=CARTESIAN_POINT('Ctrl Pts',(-12.1623797632097,128.524999999496,
2.97892388940585E-15));
#287726=CARTESIAN_POINT('Ctrl Pts',(-12.1623797632097,128.674999999495,
3.95179673813133));
#287727=CARTESIAN_POINT('Ctrl Pts',(-9.83957192047864,128.824999999495,
7.14886745759505));
#287728=CARTESIAN_POINT('Ctrl Pts',(-7.51676407774754,128.974999999494,
10.3459381770588));
#287729=CARTESIAN_POINT('Ctrl Pts',(-3.75838203887381,129.124999999494,
11.5671105274568));
#287730=CARTESIAN_POINT('Ctrl Pts',(-8.45783259963234E-14,129.274999999493,
12.7882828778549));
#287731=CARTESIAN_POINT('Ctrl Pts',(3.75838203887364,129.424999999492,11.5671105274568));
#287732=CARTESIAN_POINT('Ctrl Pts',(7.51676407774737,129.574999999492,10.3459381770588));
#287733=CARTESIAN_POINT('Ctrl Pts',(9.83957192047846,129.724999999491,7.14886745759505));
#287734=CARTESIAN_POINT('Ctrl Pts',(12.1623797632096,129.874999999491,3.95179673813132));
#287735=CARTESIAN_POINT('Ctrl Pts',(12.1623797632096,130.02499999949,-1.48946194470292E-15));
#287736=CARTESIAN_POINT('Ctrl Pts',(12.1623797632096,130.174999999489,-3.95179673813132));
#287737=CARTESIAN_POINT('Ctrl Pts',(9.83957192047846,130.324999999489,-7.14886745759505));
#287738=CARTESIAN_POINT('Ctrl Pts',(7.51676407774737,130.474999999488,-10.3459381770588));
#287739=CARTESIAN_POINT('Ctrl Pts',(3.75838203887364,130.624999999488,-11.5671105274568));
#287740=CARTESIAN_POINT('Ctrl Pts',(-8.85744065707455E-14,130.774999999487,
-12.7882828778549));
#287741=CARTESIAN_POINT('Ctrl Pts',(-3.75838203887382,130.924999999486,
-11.5671105274568));
#287742=CARTESIAN_POINT('Ctrl Pts',(-7.51676407774754,131.074999999486,
-10.3459381770588));
#287743=CARTESIAN_POINT('Ctrl Pts',(-9.83957192047864,131.224999999485,
-7.14886745759505));
#287744=CARTESIAN_POINT('Ctrl Pts',(-12.1623797632097,131.374999999485,
-3.95179673813132));
#287745=CARTESIAN_POINT('Ctrl Pts',(-12.1623797632097,131.524999999484,
2.97892388940585E-15));
#287746=CARTESIAN_POINT('Ctrl Pts',(-12.1623797632097,131.674999999483,
3.95179673813133));
#287747=CARTESIAN_POINT('Ctrl Pts',(-9.83957192047864,131.824999999483,
7.14886745759505));
#287748=CARTESIAN_POINT('Ctrl Pts',(-7.51676407774754,131.974999999482,
10.3459381770588));
#287749=CARTESIAN_POINT('Ctrl Pts',(-3.75838203887381,132.124999999482,
11.5671105274568));
#287750=CARTESIAN_POINT('Ctrl Pts',(-8.63060352679853E-14,132.274999999481,
12.7882828778549));
#287751=CARTESIAN_POINT('Ctrl Pts',(3.75838203887364,132.42499999948,11.5671105274568));
#287752=CARTESIAN_POINT('Ctrl Pts',(7.51676407774737,132.57499999948,10.3459381770588));
#287753=CARTESIAN_POINT('Ctrl Pts',(9.83957192047846,132.724999999479,7.14886745759505));
#287754=CARTESIAN_POINT('Ctrl Pts',(12.1623797632096,132.874999999479,3.95179673813132));
#287755=CARTESIAN_POINT('Ctrl Pts',(12.1623797632096,133.024999999478,-1.48946194470292E-15));
#287756=CARTESIAN_POINT('Ctrl Pts',(12.1623797632096,133.174999999477,-3.95179673813132));
#287757=CARTESIAN_POINT('Ctrl Pts',(9.83957192047846,133.324999999477,-7.14886745759505));
#287758=CARTESIAN_POINT('Ctrl Pts',(7.51676407774736,133.474999999476,-10.3459381770588));
#287759=CARTESIAN_POINT('Ctrl Pts',(3.75838203887364,133.624999999476,-11.5671105274568));
#287760=CARTESIAN_POINT('Ctrl Pts',(-9.03021158424074E-14,133.774999999475,
-12.7882828778549));
#287761=CARTESIAN_POINT('Ctrl Pts',(-3.75838203887382,133.924999999474,
-11.5671105274568));
#287762=CARTESIAN_POINT('Ctrl Pts',(-7.51676407774755,134.074999999474,
-10.3459381770588));
#287763=CARTESIAN_POINT('Ctrl Pts',(-9.83957192047864,134.224999999473,
-7.14886745759505));
#287764=CARTESIAN_POINT('Ctrl Pts',(-12.1623797632097,134.374999999473,
-3.95179673813132));
#287765=CARTESIAN_POINT('Ctrl Pts',(-12.1623797632097,134.524999999472,
2.97892388940585E-15));
#287766=CARTESIAN_POINT('Ctrl Pts',(-12.1623797632097,134.674999999471,
3.95179673813133));
#287767=CARTESIAN_POINT('Ctrl Pts',(-9.83957192047864,134.824999999471,
7.14886745759505));
#287768=CARTESIAN_POINT('Ctrl Pts',(-7.51676407774754,134.97499999947,10.3459381770588));
#287769=CARTESIAN_POINT('Ctrl Pts',(-3.75838203887382,135.12499999947,11.5671105274568));
#287770=CARTESIAN_POINT('Ctrl Pts',(-8.80337445396471E-14,135.274999999469,
12.7882828778549));
#287771=CARTESIAN_POINT('Ctrl Pts',(3.75838203887364,135.424999999468,11.5671105274568));
#287772=CARTESIAN_POINT('Ctrl Pts',(7.51676407774737,135.574999999468,10.3459381770588));
#287773=CARTESIAN_POINT('Ctrl Pts',(9.83957192047846,135.724999999467,7.14886745759505));
#287774=CARTESIAN_POINT('Ctrl Pts',(12.1623797632096,135.874999999467,3.95179673813132));
#287775=CARTESIAN_POINT('Ctrl Pts',(12.1623797632096,136.024999999466,-1.48946194470292E-15));
#287776=CARTESIAN_POINT('Ctrl Pts',(12.1623797632095,136.174999999465,-3.95179673813132));
#287777=CARTESIAN_POINT('Ctrl Pts',(9.83957192047846,136.324999999465,-7.14886745759505));
#287778=CARTESIAN_POINT('Ctrl Pts',(7.51676407774736,136.474999999464,-10.3459381770588));
#287779=CARTESIAN_POINT('Ctrl Pts',(3.75838203887364,136.624999999464,-11.5671105274568));
#287780=CARTESIAN_POINT('Ctrl Pts',(-9.20298251140692E-14,136.774999999463,
-12.7882828778549));
#287781=CARTESIAN_POINT('Ctrl Pts',(-3.75838203887382,136.924999999462,
-11.5671105274568));
#287782=CARTESIAN_POINT('Ctrl Pts',(-7.51676407774755,137.074999999462,
-10.3459381770588));
#287783=CARTESIAN_POINT('Ctrl Pts',(-9.83957192047864,137.224999999461,
-7.14886745759505));
#287784=CARTESIAN_POINT('Ctrl Pts',(-12.1623797632097,137.374999999461,
-3.95179673813132));
#287785=CARTESIAN_POINT('Ctrl Pts',(-12.1623797632097,137.52499999946,2.97892388940585E-15));
#287786=CARTESIAN_POINT('Ctrl Pts',(-12.1623797632097,137.674999999459,
3.95179673813133));
#287787=CARTESIAN_POINT('Ctrl Pts',(-9.83957192047864,137.824999999459,
7.14886745759505));
#287788=CARTESIAN_POINT('Ctrl Pts',(-7.51676407774755,137.974999999458,
10.3459381770588));
#287789=CARTESIAN_POINT('Ctrl Pts',(-3.75838203887382,138.124999999458,
11.5671105274568));
#287790=CARTESIAN_POINT('Ctrl Pts',(-8.97614538113089E-14,138.274999999457,
12.7882828778549));
#287791=CARTESIAN_POINT('Ctrl Pts',(3.75838203887364,138.424999999456,11.5671105274568));
#287792=CARTESIAN_POINT('Ctrl Pts',(7.51676407774736,138.574999999456,10.3459381770588));
#287793=CARTESIAN_POINT('Ctrl Pts',(9.83957192047846,138.724999999455,7.14886745759505));
#287794=CARTESIAN_POINT('Ctrl Pts',(12.1623797632096,138.874999999455,3.95179673813132));
#287795=CARTESIAN_POINT('Ctrl Pts',(12.1623797632096,139.024999999454,-1.48946194470292E-15));
#287796=CARTESIAN_POINT('Ctrl Pts',(12.1623797632095,139.174999999453,-3.95179673813132));
#287797=CARTESIAN_POINT('Ctrl Pts',(9.83957192047846,139.324999999453,-7.14886745759505));
#287798=CARTESIAN_POINT('Ctrl Pts',(7.51676407774736,139.474999999452,-10.3459381770588));
#287799=CARTESIAN_POINT('Ctrl Pts',(3.75838203887363,139.624999999452,-11.5671105274568));
#287800=CARTESIAN_POINT('Ctrl Pts',(-9.3757534385731E-14,139.774999999451,
-12.7882828778549));
#287801=CARTESIAN_POINT('Ctrl Pts',(-3.75838203887382,139.92499999945,-11.5671105274568));
#287802=CARTESIAN_POINT('Ctrl Pts',(-7.51676407774755,140.07499999945,-10.3459381770588));
#287803=CARTESIAN_POINT('Ctrl Pts',(-9.83957192047864,140.224999999449,
-7.14886745759505));
#287804=CARTESIAN_POINT('Ctrl Pts',(-12.1623797632097,140.374999999449,
-3.95179673813132));
#287805=CARTESIAN_POINT('Ctrl Pts',(-12.1623797632097,140.524999999448,
2.97892388940585E-15));
#287806=CARTESIAN_POINT('Ctrl Pts',(-12.1623797632097,140.674999999447,
3.95179673813133));
#287807=CARTESIAN_POINT('Ctrl Pts',(-9.83957192047864,140.824999999447,
7.14886745759505));
#287808=CARTESIAN_POINT('Ctrl Pts',(-7.51676407774755,140.974999999446,
10.3459381770588));
#287809=CARTESIAN_POINT('Ctrl Pts',(-3.75838203887382,141.124999999446,
11.5671105274568));
#287810=CARTESIAN_POINT('Ctrl Pts',(-9.14891630829708E-14,141.274999999445,
12.7882828778549));
#287811=CARTESIAN_POINT('Ctrl Pts',(3.75838203887364,141.424999999444,11.5671105274568));
#287812=CARTESIAN_POINT('Ctrl Pts',(7.51676407774736,141.574999999444,10.3459381770588));
#287813=CARTESIAN_POINT('Ctrl Pts',(9.83957192047845,141.724999999443,7.14886745759505));
#287814=CARTESIAN_POINT('Ctrl Pts',(12.1623797632095,141.874999999443,3.95179673813132));
#287815=CARTESIAN_POINT('Ctrl Pts',(12.1623797632095,142.024999999442,-1.48946194470292E-15));
#287816=CARTESIAN_POINT('Ctrl Pts',(12.1623797632095,142.174999999441,-3.95179673813132));
#287817=CARTESIAN_POINT('Ctrl Pts',(9.83957192047845,142.324999999441,-7.14886745759505));
#287818=CARTESIAN_POINT('Ctrl Pts',(7.51676407774736,142.47499999944,-10.3459381770588));
#287819=CARTESIAN_POINT('Ctrl Pts',(3.75838203887363,142.62499999944,-11.5671105274568));
#287820=CARTESIAN_POINT('Ctrl Pts',(-9.54852436573929E-14,142.774999999439,
-12.7882828778549));
#287821=CARTESIAN_POINT('Ctrl Pts',(-3.75838203887382,142.924999999438,
-11.5671105274568));
#287822=CARTESIAN_POINT('Ctrl Pts',(-7.51676407774755,143.074999999438,
-10.3459381770588));
#287823=CARTESIAN_POINT('Ctrl Pts',(-9.83957192047864,143.224999999437,
-7.14886745759505));
#287824=CARTESIAN_POINT('Ctrl Pts',(-12.1623797632097,143.374999999437,
-3.95179673813132));
#287825=CARTESIAN_POINT('Ctrl Pts',(-12.1623797632097,143.524999999436,
2.97892388940585E-15));
#287826=CARTESIAN_POINT('Ctrl Pts',(-12.1623797632097,143.674999999435,
3.95179673813133));
#287827=CARTESIAN_POINT('Ctrl Pts',(-9.83957192047864,143.824999999435,
7.14886745759505));
#287828=CARTESIAN_POINT('Ctrl Pts',(-7.51676407774755,143.974999999434,
10.3459381770588));
#287829=CARTESIAN_POINT('Ctrl Pts',(-3.75838203887382,144.124999999434,
11.5671105274568));
#287830=CARTESIAN_POINT('Ctrl Pts',(-9.32168723546326E-14,144.274999999433,
12.7882828778549));
#287831=CARTESIAN_POINT('Ctrl Pts',(3.75838203887363,144.424999999432,11.5671105274568));
#287832=CARTESIAN_POINT('Ctrl Pts',(7.51676407774736,144.574999999432,10.3459381770588));
#287833=CARTESIAN_POINT('Ctrl Pts',(9.83957192047845,144.724999999431,7.14886745759505));
#287834=CARTESIAN_POINT('Ctrl Pts',(12.1623797632095,144.874999999431,3.95179673813132));
#287835=CARTESIAN_POINT('Ctrl Pts',(12.1623797632095,145.02499999943,-1.48946194470292E-15));
#287836=CARTESIAN_POINT('Ctrl Pts',(12.1623797632095,145.174999999429,-3.95179673813132));
#287837=CARTESIAN_POINT('Ctrl Pts',(9.83957192047845,145.324999999429,-7.14886745759505));
#287838=CARTESIAN_POINT('Ctrl Pts',(7.51676407774736,145.474999999428,-10.3459381770588));
#287839=CARTESIAN_POINT('Ctrl Pts',(3.75838203887363,145.624999999428,-11.5671105274568));
#287840=CARTESIAN_POINT('Ctrl Pts',(-9.72129529290547E-14,145.774999999427,
-12.7882828778549));
#287841=CARTESIAN_POINT('Ctrl Pts',(-3.75838203887382,145.924999999426,
-11.5671105274568));
#287842=CARTESIAN_POINT('Ctrl Pts',(-7.51676407774755,146.074999999426,
-10.3459381770588));
#287843=CARTESIAN_POINT('Ctrl Pts',(-9.83957192047865,146.224999999425,
-7.14886745759505));
#287844=CARTESIAN_POINT('Ctrl Pts',(-12.1623797632097,146.374999999425,
-3.95179673813132));
#287845=CARTESIAN_POINT('Ctrl Pts',(-12.1623797632097,146.524999999424,
2.97892388940585E-15));
#287846=CARTESIAN_POINT('Ctrl Pts',(-12.1623797632097,146.674999999423,
3.95179673813133));
#287847=CARTESIAN_POINT('Ctrl Pts',(-9.83957192047865,146.824999999423,
7.14886745759505));
#287848=CARTESIAN_POINT('Ctrl Pts',(-7.51676407774755,146.974999999422,
10.3459381770588));
#287849=CARTESIAN_POINT('Ctrl Pts',(-3.75838203887382,147.124999999422,
11.5671105274568));
#287850=CARTESIAN_POINT('Ctrl Pts',(-9.49445816262944E-14,147.274999999421,
12.7882828778549));
#287851=CARTESIAN_POINT('Ctrl Pts',(3.75838203887363,147.42499999942,11.5671105274568));
#287852=CARTESIAN_POINT('Ctrl Pts',(7.51676407774736,147.57499999942,10.3459381770588));
#287853=CARTESIAN_POINT('Ctrl Pts',(9.83957192047845,147.724999999419,7.14886745759505));
#287854=CARTESIAN_POINT('Ctrl Pts',(12.1623797632095,147.874999999419,3.95179673813132));
#287855=CARTESIAN_POINT('Ctrl Pts',(12.1623797632095,148.024999999418,-1.48946194470292E-15));
#287856=CARTESIAN_POINT('Ctrl Pts',(12.1623797632095,148.174999999417,-3.95179673813132));
#287857=CARTESIAN_POINT('Ctrl Pts',(9.83957192047845,148.324999999417,-7.14886745759505));
#287858=CARTESIAN_POINT('Ctrl Pts',(7.51676407774736,148.474999999416,-10.3459381770588));
#287859=CARTESIAN_POINT('Ctrl Pts',(3.75838203887363,148.624999999416,-11.5671105274568));
#287860=CARTESIAN_POINT('Ctrl Pts',(-9.89406622007166E-14,148.774999999415,
-12.7882828778549));
#287861=CARTESIAN_POINT('Ctrl Pts',(-3.75838203887383,148.924999999414,
-11.5671105274568));
#287862=CARTESIAN_POINT('Ctrl Pts',(-7.51676407774756,149.074999999414,
-10.3459381770588));
#287863=CARTESIAN_POINT('Ctrl Pts',(-9.83957192047865,149.224999999413,
-7.14886745759505));
#287864=CARTESIAN_POINT('Ctrl Pts',(-12.1623797632097,149.374999999413,
-3.95179673813132));
#287865=CARTESIAN_POINT('Ctrl Pts',(-12.1623797632097,149.524999999412,
2.97892388940585E-15));
#287866=CARTESIAN_POINT('Ctrl Pts',(-12.1623797632097,149.674999999411,
3.95179673813133));
#287867=CARTESIAN_POINT('Ctrl Pts',(-9.83957192047865,149.824999999411,
7.14886745759505));
#287868=CARTESIAN_POINT('Ctrl Pts',(-7.51676407774755,149.97499999941,10.3459381770588));
#287869=CARTESIAN_POINT('Ctrl Pts',(-3.75838203887382,150.12499999941,11.5671105274568));
#287870=CARTESIAN_POINT('Ctrl Pts',(-9.66722908979563E-14,150.274999999409,
12.7882828778549));
#287871=CARTESIAN_POINT('Ctrl Pts',(3.75838203887363,150.424999999408,11.5671105274568));
#287872=CARTESIAN_POINT('Ctrl Pts',(7.51676407774736,150.574999999408,10.3459381770588));
#287873=CARTESIAN_POINT('Ctrl Pts',(9.83957192047845,150.724999999407,7.14886745759505));
#287874=CARTESIAN_POINT('Ctrl Pts',(12.1623797632095,150.874999999407,3.95179673813132));
#287875=CARTESIAN_POINT('Ctrl Pts',(12.1623797632095,151.024999999406,-1.48946194470292E-15));
#287876=CARTESIAN_POINT('Ctrl Pts',(12.1623797632095,151.174999999405,-3.95179673813132));
#287877=CARTESIAN_POINT('Ctrl Pts',(9.83957192047845,151.324999999405,-7.14886745759505));
#287878=CARTESIAN_POINT('Ctrl Pts',(7.51676407774736,151.474999999404,-10.3459381770588));
#287879=CARTESIAN_POINT('Ctrl Pts',(3.75838203887363,151.624999999404,-11.5671105274568));
#287880=CARTESIAN_POINT('Ctrl Pts',(-1.00668371472378E-13,151.774999999403,
-12.7882828778549));
#287881=CARTESIAN_POINT('Ctrl Pts',(-3.75838203887383,151.924999999402,
-11.5671105274568));
#287882=CARTESIAN_POINT('Ctrl Pts',(-7.51676407774756,152.074999999402,
-10.3459381770588));
#287883=CARTESIAN_POINT('Ctrl Pts',(-9.83957192047865,152.224999999401,
-7.14886745759505));
#287884=CARTESIAN_POINT('Ctrl Pts',(-12.1623797632097,152.374999999401,
-3.95179673813132));
#287885=CARTESIAN_POINT('Ctrl Pts',(-12.1623797632097,152.5249999994,2.97892388940585E-15));
#287886=CARTESIAN_POINT('Ctrl Pts',(-12.1623797632097,152.674999999399,
3.95179673813133));
#287887=CARTESIAN_POINT('Ctrl Pts',(-9.83957192047865,152.824999999399,
7.14886745759505));
#287888=CARTESIAN_POINT('Ctrl Pts',(-7.51676407774756,152.974999999398,
10.3459381770588));
#287889=CARTESIAN_POINT('Ctrl Pts',(-3.75838203887383,153.124999999398,
11.5671105274568));
#287890=CARTESIAN_POINT('Ctrl Pts',(-9.84000001696181E-14,153.274999999397,
12.7882828778549));
#287891=CARTESIAN_POINT('Ctrl Pts',(3.75838203887363,153.424999999396,11.5671105274568));
#287892=CARTESIAN_POINT('Ctrl Pts',(7.51676407774736,153.574999999396,10.3459381770588));
#287893=CARTESIAN_POINT('Ctrl Pts',(9.83957192047845,153.724999999395,7.14886745759505));
#287894=CARTESIAN_POINT('Ctrl Pts',(12.1623797632095,153.874999999395,3.95179673813132));
#287895=CARTESIAN_POINT('Ctrl Pts',(12.1623797632095,154.024999999394,-1.48946194470292E-15));
#287896=CARTESIAN_POINT('Ctrl Pts',(12.1623797632095,154.174999999393,-3.95179673813132));
#287897=CARTESIAN_POINT('Ctrl Pts',(9.83957192047845,154.324999999393,-7.14886745759505));
#287898=CARTESIAN_POINT('Ctrl Pts',(7.51676407774735,154.474999999392,-10.3459381770588));
#287899=CARTESIAN_POINT('Ctrl Pts',(3.75838203887363,154.624999999392,-11.5671105274568));
#287900=CARTESIAN_POINT('Ctrl Pts',(-1.0239608074404E-13,154.774999999391,
-12.7882828778549));
#287901=CARTESIAN_POINT('Ctrl Pts',(-3.75838203887383,154.92499999939,-11.5671105274568));
#287902=CARTESIAN_POINT('',(-9.80053286676861,76.2,-2.23182856044403));
#287903=CARTESIAN_POINT('Ctrl Pts',(10.0514428414941,74.8062499997113,-1.23094673026484E-15));
#287904=CARTESIAN_POINT('Ctrl Pts',(10.0514428414941,74.9562499997106,-3.26591175476071));
#287905=CARTESIAN_POINT('Ctrl Pts',(8.13178807675713,75.10624999971,-5.90808986649102));
#287906=CARTESIAN_POINT('Ctrl Pts',(6.21213331202016,75.2562499997095,-8.55026797822134));
#287907=CARTESIAN_POINT('Ctrl Pts',(3.10606665601005,75.4062499997088,-9.5594902125713));
#287908=CARTESIAN_POINT('Ctrl Pts',(-5.66378482980338E-14,75.5562499997083,
-10.5687124469213));
#287909=CARTESIAN_POINT('Ctrl Pts',(-3.10606665601016,75.7062499997077,
-9.5594902125713));
#287910=CARTESIAN_POINT('Ctrl Pts',(-6.21213331202027,75.8562499997071,
-8.55026797822134));
#287911=CARTESIAN_POINT('Ctrl Pts',(-8.13178807675725,76.0062499997065,
-5.90808986649102));
#287912=CARTESIAN_POINT('Ctrl Pts',(-9.34299114618875,76.1008922571328,
-4.2410118597063));
#287913=CARTESIAN_POINT('Ctrl Pts',(-9.80053286676861,76.2,-2.23182856044403));
#287914=CARTESIAN_POINT('Ctrl Pts',(-9.80053286676861,76.2,-2.23182856044404));
#287915=CARTESIAN_POINT('Ctrl Pts',(-9.6944232497338,76.2,-2.98049389998223));
#287916=CARTESIAN_POINT('Ctrl Pts',(-9.50451644375251,76.2,-3.71482315444662));
#287917=CARTESIAN_POINT('Ctrl Pts',(-8.9507720992266,76.2,-5.16268983688915));
#287918=CARTESIAN_POINT('Ctrl Pts',(-8.58384186538138,76.2,-5.86027015767421));
#287919=CARTESIAN_POINT('Ctrl Pts',(-7.36855104616312,76.2,-7.64541067699849));
#287920=CARTESIAN_POINT('Ctrl Pts',(-6.39031235163314,76.1999999999999,
-8.61475197019007));
#287921=CARTESIAN_POINT('Ctrl Pts',(-3.72933845937247,76.1999999999999,
-10.3909605175236));
#287922=CARTESIAN_POINT('Ctrl Pts',(-2.26196014736257,76.2,-10.8035407208194));
#287923=CARTESIAN_POINT('Ctrl Pts',(0.153337835077095,76.2,-11.2744264553899));
#287924=CARTESIAN_POINT('Ctrl Pts',(1.64295619773128,76.2,-11.2661126066267));
#287925=CARTESIAN_POINT('Ctrl Pts',(4.28244648061358,76.2,-10.7213720931628));
#287926=CARTESIAN_POINT('Ctrl Pts',(5.67769351012328,76.2,-10.229155280931));
#287927=CARTESIAN_POINT('Ctrl Pts',(7.64416788707506,76.2,-8.9539354014207));
#287928=CARTESIAN_POINT('Ctrl Pts',(8.19850424462796,76.2000000003225,-8.51856537485932));
#287929=CARTESIAN_POINT('Ctrl Pts',(9.24635223087657,76.2000000003225,-7.53021049871108));
#287930=CARTESIAN_POINT('Ctrl Pts',(9.73034607334846,76.2,-6.97611193267191));
#287931=CARTESIAN_POINT('Ctrl Pts',(10.1587275000649,76.2,-6.38750777529538));
#287932=CARTESIAN_POINT('Ctrl Pts',(-12.1623797632103,-3.28749999997638,
2.97892388940601E-15));
#287933=CARTESIAN_POINT('Ctrl Pts',(-12.1623797632103,-3.13749999997698,
3.95179673813154));
#287934=CARTESIAN_POINT('Ctrl Pts',(-9.83957192047908,-2.98749999997758,
7.14886745759543));
#287935=CARTESIAN_POINT('Ctrl Pts',(-7.51676407774787,-2.83749999997817,
10.3459381770593));
#287936=CARTESIAN_POINT('Ctrl Pts',(-3.75838203887394,-2.68749999997877,
11.5671105274575));
#287937=CARTESIAN_POINT('Ctrl Pts',(-8.66709987268145E-15,-2.53749999997937,
12.7882828778556));
#287938=CARTESIAN_POINT('Ctrl Pts',(3.75838203887392,-2.38749999997997,
11.5671105274575));
#287939=CARTESIAN_POINT('Ctrl Pts',(7.51676407774785,-2.23749999998057,
10.3459381770593));
#287940=CARTESIAN_POINT('Ctrl Pts',(9.83957192047906,-2.08749999998117,
7.14886745759543));
#287941=CARTESIAN_POINT('Ctrl Pts',(12.1623797632103,-1.93749999998176,
3.95179673813153));
#287942=CARTESIAN_POINT('Ctrl Pts',(12.1623797632103,-1.78749999998236,
-1.489461944703E-15));
#287943=CARTESIAN_POINT('Ctrl Pts',(12.1623797632103,-1.63749999998296,
-3.95179673813154));
#287944=CARTESIAN_POINT('Ctrl Pts',(9.83957192047906,-1.48749999998357,
-7.14886745759543));
#287945=CARTESIAN_POINT('Ctrl Pts',(7.51676407774784,-1.33749999998417,
-10.3459381770593));
#287946=CARTESIAN_POINT('Ctrl Pts',(3.75838203887392,-1.18749999998477,
-11.5671105274575));
#287947=CARTESIAN_POINT('Ctrl Pts',(-1.26631804471037E-14,-1.03749999998537,
-12.7882828778556));
#287948=CARTESIAN_POINT('Ctrl Pts',(-3.75838203887394,-0.887499999985973,
-11.5671105274575));
#287949=CARTESIAN_POINT('Ctrl Pts',(-7.51676407774787,-0.737499999986575,
-10.3459381770593));
#287950=CARTESIAN_POINT('Ctrl Pts',(-9.83957192047909,-0.587499999987176,
-7.14886745759543));
#287951=CARTESIAN_POINT('Ctrl Pts',(-12.1623797632103,-0.437499999987778,
-3.95179673813153));
#287952=CARTESIAN_POINT('Ctrl Pts',(-12.1623797632103,-0.287499999988378,
2.97892388940601E-15));
#287953=CARTESIAN_POINT('Ctrl Pts',(-12.1623797632103,-0.137499999988978,
3.95179673813154));
#287954=CARTESIAN_POINT('Ctrl Pts',(-9.83957192047909,0.0125000000104236,
7.14886745759543));
#287955=CARTESIAN_POINT('Ctrl Pts',(-7.51676407774787,0.162500000009825,
10.3459381770593));
#287956=CARTESIAN_POINT('Ctrl Pts',(-3.75838203887394,0.312500000009227,
11.5671105274575));
#287957=CARTESIAN_POINT('Ctrl Pts',(-1.03948091443433E-14,0.462500000008629,
12.7882828778556));
#287958=CARTESIAN_POINT('Ctrl Pts',(3.75838203887392,0.612500000008031,
11.5671105274575));
#287959=CARTESIAN_POINT('Ctrl Pts',(7.51676407774785,0.762500000007433,
10.3459381770593));
#287960=CARTESIAN_POINT('Ctrl Pts',(9.83957192047906,0.912500000006835,
7.14886745759543));
#287961=CARTESIAN_POINT('Ctrl Pts',(12.1623797632103,1.06250000000624,3.95179673813153));
#287962=CARTESIAN_POINT('Ctrl Pts',(12.1623797632103,1.21250000000564,-1.489461944703E-15));
#287963=CARTESIAN_POINT('Ctrl Pts',(12.1623797632103,1.36250000000504,-3.95179673813154));
#287964=CARTESIAN_POINT('Ctrl Pts',(9.83957192047906,1.51250000000444,-7.14886745759543));
#287965=CARTESIAN_POINT('Ctrl Pts',(7.51676407774784,1.66250000000383,-10.3459381770593));
#287966=CARTESIAN_POINT('Ctrl Pts',(3.75838203887391,1.81250000000323,-11.5671105274575));
#287967=CARTESIAN_POINT('Ctrl Pts',(-1.43908897187656E-14,1.96250000000263,
-12.7882828778556));
#287968=CARTESIAN_POINT('Ctrl Pts',(-3.75838203887394,2.11250000000203,
-11.5671105274575));
#287969=CARTESIAN_POINT('Ctrl Pts',(-7.51676407774787,2.26250000000143,
-10.3459381770593));
#287970=CARTESIAN_POINT('Ctrl Pts',(-9.83957192047909,2.41250000000082,
-7.14886745759543));
#287971=CARTESIAN_POINT('Ctrl Pts',(-12.1623797632103,2.56250000000022,
-3.95179673813153));
#287972=CARTESIAN_POINT('Ctrl Pts',(-12.1623797632103,2.71249999999962,
2.97892388940601E-15));
#287973=CARTESIAN_POINT('Ctrl Pts',(-12.1623797632103,2.86249999999902,
3.95179673813154));
#287974=CARTESIAN_POINT('Ctrl Pts',(-9.83957192047909,3.01249999999842,
7.14886745759543));
#287975=CARTESIAN_POINT('Ctrl Pts',(-7.51676407774787,3.16249999999782,
10.3459381770593));
#287976=CARTESIAN_POINT('Ctrl Pts',(-3.75838203887394,3.31249999999723,
11.5671105274575));
#287977=CARTESIAN_POINT('Ctrl Pts',(-1.21225184160051E-14,3.46249999999663,
12.7882828778556));
#287978=CARTESIAN_POINT('Ctrl Pts',(3.75838203887392,3.61249999999603,11.5671105274575));
#287979=CARTESIAN_POINT('Ctrl Pts',(7.51676407774784,3.76249999999543,10.3459381770593));
#287980=CARTESIAN_POINT('Ctrl Pts',(9.83957192047906,3.91249999999483,7.14886745759543));
#287981=CARTESIAN_POINT('Ctrl Pts',(12.1623797632103,4.06249999999424,3.95179673813153));
#287982=CARTESIAN_POINT('Ctrl Pts',(12.1623797632103,4.21249999999364,-1.489461944703E-15));
#287983=CARTESIAN_POINT('Ctrl Pts',(12.1623797632103,4.36249999999303,-3.95179673813154));
#287984=CARTESIAN_POINT('Ctrl Pts',(9.83957192047906,4.51249999999243,-7.14886745759543));
#287985=CARTESIAN_POINT('Ctrl Pts',(7.51676407774784,4.66249999999183,-10.3459381770593));
#287986=CARTESIAN_POINT('Ctrl Pts',(3.75838203887391,4.81249999999123,-11.5671105274575));
#287987=CARTESIAN_POINT('Ctrl Pts',(-1.61185989904274E-14,4.96249999999063,
-12.7882828778556));
#287988=CARTESIAN_POINT('Ctrl Pts',(-3.75838203887394,5.11249999999003,
-11.5671105274575));
#287989=CARTESIAN_POINT('Ctrl Pts',(-7.51676407774788,5.26249999998942,
-10.3459381770593));
#287990=CARTESIAN_POINT('Ctrl Pts',(-9.83957192047909,5.41249999998882,
-7.14886745759543));
#287991=CARTESIAN_POINT('Ctrl Pts',(-12.1623797632103,5.56249999998822,
-3.95179673813153));
#287992=CARTESIAN_POINT('Ctrl Pts',(-12.1623797632103,5.71249999998762,
2.97892388940601E-15));
#287993=CARTESIAN_POINT('Ctrl Pts',(-12.1623797632103,5.86249999998702,
3.95179673813154));
#287994=CARTESIAN_POINT('Ctrl Pts',(-9.83957192047909,6.01249999998642,
7.14886745759543));
#287995=CARTESIAN_POINT('Ctrl Pts',(-7.51676407774787,6.16249999998582,
10.3459381770593));
#287996=CARTESIAN_POINT('Ctrl Pts',(-3.75838203887394,6.31249999998523,
11.5671105274575));
#287997=CARTESIAN_POINT('Ctrl Pts',(-1.3850227687667E-14,6.46249999998463,
12.7882828778556));
#287998=CARTESIAN_POINT('Ctrl Pts',(3.75838203887392,6.61249999998403,11.5671105274575));
#287999=CARTESIAN_POINT('Ctrl Pts',(7.51676407774784,6.76249999998343,10.3459381770593));
#288000=CARTESIAN_POINT('Ctrl Pts',(9.83957192047906,6.91249999998283,7.14886745759543));
#288001=CARTESIAN_POINT('Ctrl Pts',(12.1623797632103,7.06249999998224,3.95179673813153));
#288002=CARTESIAN_POINT('Ctrl Pts',(12.1623797632103,7.21249999998164,-1.489461944703E-15));
#288003=CARTESIAN_POINT('Ctrl Pts',(12.1623797632103,7.36249999998104,-3.95179673813154));
#288004=CARTESIAN_POINT('Ctrl Pts',(9.83957192047906,7.51249999998044,-7.14886745759543));
#288005=CARTESIAN_POINT('Ctrl Pts',(7.51676407774784,7.66249999997983,-10.3459381770593));
#288006=CARTESIAN_POINT('Ctrl Pts',(3.75838203887391,7.81249999997923,-11.5671105274575));
#288007=CARTESIAN_POINT('Ctrl Pts',(-1.78463082620892E-14,7.96249999997863,
-12.7882828778556));
#288008=CARTESIAN_POINT('Ctrl Pts',(-3.75838203887395,8.11249999997803,
-11.5671105274575));
#288009=CARTESIAN_POINT('Ctrl Pts',(-7.51676407774788,8.26249999997743,
-10.3459381770593));
#288010=CARTESIAN_POINT('Ctrl Pts',(-9.83957192047909,8.41249999997682,
-7.14886745759543));
#288011=CARTESIAN_POINT('Ctrl Pts',(-12.1623797632103,8.56249999997622,
-3.95179673813153));
#288012=CARTESIAN_POINT('Ctrl Pts',(-12.1623797632103,8.71249999997562,
2.97892388940601E-15));
#288013=CARTESIAN_POINT('Ctrl Pts',(-12.1623797632103,8.86249999997502,
3.95179673813154));
#288014=CARTESIAN_POINT('Ctrl Pts',(-9.83957192047909,9.01249999997442,
7.14886745759543));
#288015=CARTESIAN_POINT('Ctrl Pts',(-7.51676407774787,9.16249999997382,
10.3459381770593));
#288016=CARTESIAN_POINT('Ctrl Pts',(-3.75838203887394,9.31249999997323,
11.5671105274575));
#288017=CARTESIAN_POINT('Ctrl Pts',(-1.55779369593288E-14,9.46249999997263,
12.7882828778556));
#288018=CARTESIAN_POINT('Ctrl Pts',(3.75838203887391,9.61249999997203,11.5671105274575));
#288019=CARTESIAN_POINT('Ctrl Pts',(7.51676407774784,9.76249999997144,10.3459381770593));
#288020=CARTESIAN_POINT('Ctrl Pts',(9.83957192047906,9.91249999997084,7.14886745759543));
#288021=CARTESIAN_POINT('Ctrl Pts',(12.1623797632103,10.0624999999702,3.95179673813153));
#288022=CARTESIAN_POINT('Ctrl Pts',(12.1623797632103,10.2124999999696,-1.489461944703E-15));
#288023=CARTESIAN_POINT('Ctrl Pts',(12.1623797632103,10.362499999969,-3.95179673813154));
#288024=CARTESIAN_POINT('Ctrl Pts',(9.83957192047905,10.5124999999684,-7.14886745759543));
#288025=CARTESIAN_POINT('Ctrl Pts',(7.51676407774784,10.6624999999678,-10.3459381770593));
#288026=CARTESIAN_POINT('Ctrl Pts',(3.75838203887391,10.8124999999672,-11.5671105274575));
#288027=CARTESIAN_POINT('Ctrl Pts',(-1.95740175337511E-14,10.9624999999666,
-12.7882828778556));
#288028=CARTESIAN_POINT('Ctrl Pts',(-3.75838203887395,11.112499999966,-11.5671105274575));
#288029=CARTESIAN_POINT('Ctrl Pts',(-7.51676407774788,11.2624999999654,
-10.3459381770593));
#288030=CARTESIAN_POINT('Ctrl Pts',(-9.83957192047909,11.4124999999648,
-7.14886745759543));
#288031=CARTESIAN_POINT('Ctrl Pts',(-12.1623797632103,11.5624999999642,
-3.95179673813153));
#288032=CARTESIAN_POINT('Ctrl Pts',(-12.1623797632103,11.7124999999636,
2.97892388940601E-15));
#288033=CARTESIAN_POINT('Ctrl Pts',(-12.1623797632103,11.862499999963,3.95179673813154));
#288034=CARTESIAN_POINT('Ctrl Pts',(-9.83957192047909,12.0124999999624,
7.14886745759543));
#288035=CARTESIAN_POINT('Ctrl Pts',(-7.51676407774788,12.1624999999618,
10.3459381770593));
#288036=CARTESIAN_POINT('Ctrl Pts',(-3.75838203887395,12.3124999999612,
11.5671105274575));
#288037=CARTESIAN_POINT('Ctrl Pts',(-1.73056462309906E-14,12.4624999999606,
12.7882828778556));
#288038=CARTESIAN_POINT('Ctrl Pts',(3.75838203887391,12.61249999996,11.5671105274575));
#288039=CARTESIAN_POINT('Ctrl Pts',(7.51676407774784,12.7624999999594,10.3459381770593));
#288040=CARTESIAN_POINT('Ctrl Pts',(9.83957192047906,12.9124999999588,7.14886745759543));
#288041=CARTESIAN_POINT('Ctrl Pts',(12.1623797632103,13.0624999999582,3.95179673813153));
#288042=CARTESIAN_POINT('Ctrl Pts',(12.1623797632103,13.2124999999576,-1.489461944703E-15));
#288043=CARTESIAN_POINT('Ctrl Pts',(12.1623797632103,13.362499999957,-3.95179673813154));
#288044=CARTESIAN_POINT('Ctrl Pts',(9.83957192047905,13.5124999999564,-7.14886745759543));
#288045=CARTESIAN_POINT('Ctrl Pts',(7.51676407774784,13.6624999999558,-10.3459381770593));
#288046=CARTESIAN_POINT('Ctrl Pts',(3.75838203887391,13.8124999999552,-11.5671105274575));
#288047=CARTESIAN_POINT('Ctrl Pts',(-2.13017268054129E-14,13.9624999999546,
-12.7882828778556));
#288048=CARTESIAN_POINT('Ctrl Pts',(-3.75838203887395,14.112499999954,-11.5671105274575));
#288049=CARTESIAN_POINT('Ctrl Pts',(-7.51676407774788,14.2624999999534,
-10.3459381770593));
#288050=CARTESIAN_POINT('Ctrl Pts',(-9.8395719204791,14.4124999999528,-7.14886745759543));
#288051=CARTESIAN_POINT('Ctrl Pts',(-12.1623797632103,14.5624999999522,
-3.95179673813153));
#288052=CARTESIAN_POINT('Ctrl Pts',(-12.1623797632103,14.7124999999516,
2.97892388940601E-15));
#288053=CARTESIAN_POINT('Ctrl Pts',(-12.1623797632103,14.862499999951,3.95179673813154));
#288054=CARTESIAN_POINT('Ctrl Pts',(-9.83957192047909,15.0124999999504,
7.14886745759543));
#288055=CARTESIAN_POINT('Ctrl Pts',(-7.51676407774788,15.1624999999498,
10.3459381770593));
#288056=CARTESIAN_POINT('Ctrl Pts',(-3.75838203887395,15.3124999999492,
11.5671105274575));
#288057=CARTESIAN_POINT('Ctrl Pts',(-1.90333555026525E-14,15.4624999999486,
12.7882828778556));
#288058=CARTESIAN_POINT('Ctrl Pts',(3.75838203887391,15.612499999948,11.5671105274575));
#288059=CARTESIAN_POINT('Ctrl Pts',(7.51676407774784,15.7624999999474,10.3459381770593));
#288060=CARTESIAN_POINT('Ctrl Pts',(9.83957192047905,15.9124999999468,7.14886745759543));
#288061=CARTESIAN_POINT('Ctrl Pts',(12.1623797632103,16.0624999999462,3.95179673813153));
#288062=CARTESIAN_POINT('Ctrl Pts',(12.1623797632103,16.2124999999456,-1.489461944703E-15));
#288063=CARTESIAN_POINT('Ctrl Pts',(12.1623797632103,16.362499999945,-3.95179673813154));
#288064=CARTESIAN_POINT('Ctrl Pts',(9.83957192047905,16.5124999999444,-7.14886745759543));
#288065=CARTESIAN_POINT('Ctrl Pts',(7.51676407774784,16.6624999999438,-10.3459381770593));
#288066=CARTESIAN_POINT('Ctrl Pts',(3.75838203887391,16.8124999999432,-11.5671105274575));
#288067=CARTESIAN_POINT('Ctrl Pts',(-2.30294360770748E-14,16.9624999999426,
-12.7882828778556));
#288068=CARTESIAN_POINT('Ctrl Pts',(-3.75838203887395,17.112499999942,-11.5671105274575));
#288069=CARTESIAN_POINT('Ctrl Pts',(-7.51676407774788,17.2624999999414,
-10.3459381770593));
#288070=CARTESIAN_POINT('Ctrl Pts',(-9.8395719204791,17.4124999999408,-7.14886745759543));
#288071=CARTESIAN_POINT('Ctrl Pts',(-12.1623797632103,17.5624999999402,
-3.95179673813153));
#288072=CARTESIAN_POINT('Ctrl Pts',(-12.1623797632103,17.7124999999396,
2.97892388940601E-15));
#288073=CARTESIAN_POINT('Ctrl Pts',(-12.1623797632103,17.862499999939,3.95179673813154));
#288074=CARTESIAN_POINT('Ctrl Pts',(-9.8395719204791,18.0124999999384,7.14886745759543));
#288075=CARTESIAN_POINT('Ctrl Pts',(-7.51676407774788,18.1624999999378,
10.3459381770593));
#288076=CARTESIAN_POINT('Ctrl Pts',(-3.75838203887395,18.3124999999372,
11.5671105274575));
#288077=CARTESIAN_POINT('Ctrl Pts',(-2.07610647743143E-14,18.4624999999366,
12.7882828778556));
#288078=CARTESIAN_POINT('Ctrl Pts',(3.75838203887391,18.612499999936,11.5671105274575));
#288079=CARTESIAN_POINT('Ctrl Pts',(7.51676407774784,18.7624999999354,10.3459381770593));
#288080=CARTESIAN_POINT('Ctrl Pts',(9.83957192047905,18.9124999999348,7.14886745759543));
#288081=CARTESIAN_POINT('Ctrl Pts',(12.1623797632103,19.0624999999342,3.95179673813153));
#288082=CARTESIAN_POINT('Ctrl Pts',(12.1623797632103,19.2124999999336,-1.489461944703E-15));
#288083=CARTESIAN_POINT('Ctrl Pts',(12.1623797632103,19.362499999933,-3.95179673813154));
#288084=CARTESIAN_POINT('Ctrl Pts',(9.83957192047905,19.5124999999324,-7.14886745759543));
#288085=CARTESIAN_POINT('Ctrl Pts',(7.51676407774784,19.6624999999318,-10.3459381770593));
#288086=CARTESIAN_POINT('Ctrl Pts',(3.7583820388739,19.8124999999312,-11.5671105274575));
#288087=CARTESIAN_POINT('Ctrl Pts',(-2.47571453487366E-14,19.9624999999306,
-12.7882828778556));
#288088=CARTESIAN_POINT('Ctrl Pts',(-3.75838203887395,20.11249999993,-11.5671105274575));
#288089=CARTESIAN_POINT('Ctrl Pts',(-7.51676407774788,20.2624999999294,
-10.3459381770593));
#288090=CARTESIAN_POINT('Ctrl Pts',(-9.8395719204791,20.4124999999288,-7.14886745759543));
#288091=CARTESIAN_POINT('Ctrl Pts',(-12.1623797632103,20.5624999999282,
-3.95179673813153));
#288092=CARTESIAN_POINT('Ctrl Pts',(-12.1623797632103,20.7124999999276,
2.97892388940601E-15));
#288093=CARTESIAN_POINT('Ctrl Pts',(-12.1623797632103,20.862499999927,3.95179673813154));
#288094=CARTESIAN_POINT('Ctrl Pts',(-9.8395719204791,21.0124999999264,7.14886745759543));
#288095=CARTESIAN_POINT('Ctrl Pts',(-7.51676407774788,21.1624999999258,
10.3459381770593));
#288096=CARTESIAN_POINT('Ctrl Pts',(-3.75838203887395,21.3124999999252,
11.5671105274575));
#288097=CARTESIAN_POINT('Ctrl Pts',(-2.24887740459762E-14,21.4624999999246,
12.7882828778556));
#288098=CARTESIAN_POINT('Ctrl Pts',(3.75838203887391,21.612499999924,11.5671105274575));
#288099=CARTESIAN_POINT('Ctrl Pts',(7.51676407774784,21.7624999999234,10.3459381770593));
#288100=CARTESIAN_POINT('Ctrl Pts',(9.83957192047905,21.9124999999228,7.14886745759543));
#288101=CARTESIAN_POINT('Ctrl Pts',(12.1623797632103,22.0624999999222,3.95179673813153));
#288102=CARTESIAN_POINT('Ctrl Pts',(12.1623797632103,22.2124999999216,-1.489461944703E-15));
#288103=CARTESIAN_POINT('Ctrl Pts',(12.1623797632103,22.362499999921,-3.95179673813154));
#288104=CARTESIAN_POINT('Ctrl Pts',(9.83957192047905,22.5124999999204,-7.14886745759543));
#288105=CARTESIAN_POINT('Ctrl Pts',(7.51676407774783,22.6624999999198,-10.3459381770593));
#288106=CARTESIAN_POINT('Ctrl Pts',(3.7583820388739,22.8124999999192,-11.5671105274575));
#288107=CARTESIAN_POINT('Ctrl Pts',(-2.64848546203984E-14,22.9624999999186,
-12.7882828778556));
#288108=CARTESIAN_POINT('Ctrl Pts',(-3.75838203887396,23.112499999918,-11.5671105274575));
#288109=CARTESIAN_POINT('Ctrl Pts',(-7.51676407774788,23.2624999999174,
-10.3459381770593));
#288110=CARTESIAN_POINT('Ctrl Pts',(-9.8395719204791,23.4124999999168,-7.14886745759543));
#288111=CARTESIAN_POINT('Ctrl Pts',(-12.1623797632103,23.5624999999162,
-3.95179673813153));
#288112=CARTESIAN_POINT('Ctrl Pts',(-12.1623797632103,23.7124999999156,
2.97892388940601E-15));
#288113=CARTESIAN_POINT('Ctrl Pts',(-12.1623797632103,23.862499999915,3.95179673813154));
#288114=CARTESIAN_POINT('Ctrl Pts',(-9.8395719204791,24.0124999999144,7.14886745759543));
#288115=CARTESIAN_POINT('Ctrl Pts',(-7.51676407774788,24.1624999999138,
10.3459381770593));
#288116=CARTESIAN_POINT('Ctrl Pts',(-3.75838203887395,24.3124999999132,
11.5671105274575));
#288117=CARTESIAN_POINT('Ctrl Pts',(-2.4216483317638E-14,24.4624999999126,
12.7882828778556));
#288118=CARTESIAN_POINT('Ctrl Pts',(3.7583820388739,24.612499999912,11.5671105274575));
#288119=CARTESIAN_POINT('Ctrl Pts',(7.51676407774783,24.7624999999114,10.3459381770593));
#288120=CARTESIAN_POINT('Ctrl Pts',(9.83957192047905,24.9124999999108,7.14886745759543));
#288121=CARTESIAN_POINT('Ctrl Pts',(12.1623797632103,25.0624999999102,3.95179673813153));
#288122=CARTESIAN_POINT('Ctrl Pts',(12.1623797632103,25.2124999999096,-1.489461944703E-15));
#288123=CARTESIAN_POINT('Ctrl Pts',(12.1623797632103,25.362499999909,-3.95179673813154));
#288124=CARTESIAN_POINT('Ctrl Pts',(9.83957192047905,25.5124999999084,-7.14886745759543));
#288125=CARTESIAN_POINT('Ctrl Pts',(7.51676407774783,25.6624999999078,-10.3459381770593));
#288126=CARTESIAN_POINT('Ctrl Pts',(3.7583820388739,25.8124999999072,-11.5671105274575));
#288127=CARTESIAN_POINT('Ctrl Pts',(-2.82125638920603E-14,25.9624999999066,
-12.7882828778556));
#288128=CARTESIAN_POINT('Ctrl Pts',(-3.75838203887396,26.112499999906,-11.5671105274575));
#288129=CARTESIAN_POINT('Ctrl Pts',(-7.51676407774788,26.2624999999054,
-10.3459381770593));
#288130=CARTESIAN_POINT('Ctrl Pts',(-9.8395719204791,26.4124999999048,-7.14886745759543));
#288131=CARTESIAN_POINT('Ctrl Pts',(-12.1623797632103,26.5624999999042,
-3.95179673813153));
#288132=CARTESIAN_POINT('Ctrl Pts',(-12.1623797632103,26.7124999999036,
2.97892388940601E-15));
#288133=CARTESIAN_POINT('Ctrl Pts',(-12.1623797632103,26.862499999903,3.95179673813154));
#288134=CARTESIAN_POINT('Ctrl Pts',(-9.8395719204791,27.0124999999024,7.14886745759543));
#288135=CARTESIAN_POINT('Ctrl Pts',(-7.51676407774788,27.1624999999018,
10.3459381770593));
#288136=CARTESIAN_POINT('Ctrl Pts',(-3.75838203887396,27.3124999999012,
11.5671105274575));
#288137=CARTESIAN_POINT('Ctrl Pts',(-2.59441925892998E-14,27.4624999999006,
12.7882828778556));
#288138=CARTESIAN_POINT('Ctrl Pts',(3.7583820388739,27.6124999999,11.5671105274575));
#288139=CARTESIAN_POINT('Ctrl Pts',(7.51676407774783,27.7624999998994,10.3459381770593));
#288140=CARTESIAN_POINT('Ctrl Pts',(9.83957192047905,27.9124999998988,7.14886745759543));
#288141=CARTESIAN_POINT('Ctrl Pts',(12.1623797632103,28.0624999998982,3.95179673813153));
#288142=CARTESIAN_POINT('Ctrl Pts',(12.1623797632103,28.2124999998976,-1.489461944703E-15));
#288143=CARTESIAN_POINT('Ctrl Pts',(12.1623797632103,28.362499999897,-3.95179673813154));
#288144=CARTESIAN_POINT('Ctrl Pts',(9.83957192047905,28.5124999998964,-7.14886745759543));
#288145=CARTESIAN_POINT('Ctrl Pts',(7.51676407774783,28.6624999998958,-10.3459381770593));
#288146=CARTESIAN_POINT('Ctrl Pts',(3.7583820388739,28.8124999998952,-11.5671105274575));
#288147=CARTESIAN_POINT('Ctrl Pts',(-2.99402731637221E-14,28.9624999998946,
-12.7882828778556));
#288148=CARTESIAN_POINT('Ctrl Pts',(-3.75838203887396,29.112499999894,-11.5671105274575));
#288149=CARTESIAN_POINT('Ctrl Pts',(-7.51676407774789,29.2624999998934,
-10.3459381770593));
#288150=CARTESIAN_POINT('Ctrl Pts',(-9.8395719204791,29.4124999998928,-7.14886745759543));
#288151=CARTESIAN_POINT('Ctrl Pts',(-12.1623797632103,29.5624999998922,
-3.95179673813153));
#288152=CARTESIAN_POINT('Ctrl Pts',(-12.1623797632103,29.7124999998916,
2.97892388940601E-15));
#288153=CARTESIAN_POINT('Ctrl Pts',(-12.1623797632103,29.862499999891,3.95179673813154));
#288154=CARTESIAN_POINT('Ctrl Pts',(-9.8395719204791,30.0124999998904,7.14886745759543));
#288155=CARTESIAN_POINT('Ctrl Pts',(-7.51676407774788,30.1624999998898,
10.3459381770593));
#288156=CARTESIAN_POINT('Ctrl Pts',(-3.75838203887396,30.3124999998892,
11.5671105274575));
#288157=CARTESIAN_POINT('Ctrl Pts',(-2.76719018609617E-14,30.4624999998886,
12.7882828778556));
#288158=CARTESIAN_POINT('Ctrl Pts',(3.7583820388739,30.612499999888,11.5671105274575));
#288159=CARTESIAN_POINT('Ctrl Pts',(7.51676407774783,30.7624999998874,10.3459381770593));
#288160=CARTESIAN_POINT('Ctrl Pts',(9.83957192047905,30.9124999998868,7.14886745759543));
#288161=CARTESIAN_POINT('Ctrl Pts',(12.1623797632103,31.0624999998862,3.95179673813153));
#288162=CARTESIAN_POINT('Ctrl Pts',(12.1623797632103,31.2124999998856,-1.489461944703E-15));
#288163=CARTESIAN_POINT('Ctrl Pts',(12.1623797632103,31.362499999885,-3.95179673813154));
#288164=CARTESIAN_POINT('Ctrl Pts',(9.83957192047904,31.5124999998844,-7.14886745759543));
#288165=CARTESIAN_POINT('Ctrl Pts',(7.51676407774783,31.6624999998838,-10.3459381770593));
#288166=CARTESIAN_POINT('Ctrl Pts',(3.7583820388739,31.8124999998832,-11.5671105274575));
#288167=CARTESIAN_POINT('Ctrl Pts',(-3.16679824353839E-14,31.9624999998826,
-12.7882828778556));
#288168=CARTESIAN_POINT('Ctrl Pts',(-3.75838203887396,32.112499999882,-11.5671105274575));
#288169=CARTESIAN_POINT('Ctrl Pts',(-7.51676407774789,32.2624999998814,
-10.3459381770593));
#288170=CARTESIAN_POINT('Ctrl Pts',(-9.83957192047911,32.4124999998808,
-7.14886745759543));
#288171=CARTESIAN_POINT('Ctrl Pts',(-12.1623797632103,32.5624999998802,
-3.95179673813153));
#288172=CARTESIAN_POINT('Ctrl Pts',(-12.1623797632103,32.7124999998796,
2.97892388940601E-15));
#288173=CARTESIAN_POINT('Ctrl Pts',(-12.1623797632103,32.862499999879,3.95179673813154));
#288174=CARTESIAN_POINT('Ctrl Pts',(-9.8395719204791,33.0124999998784,7.14886745759543));
#288175=CARTESIAN_POINT('Ctrl Pts',(-7.51676407774789,33.1624999998778,
10.3459381770593));
#288176=CARTESIAN_POINT('Ctrl Pts',(-3.75838203887396,33.3124999998772,
11.5671105274575));
#288177=CARTESIAN_POINT('Ctrl Pts',(-2.93996111326235E-14,33.4624999998766,
12.7882828778556));
#288178=CARTESIAN_POINT('Ctrl Pts',(3.7583820388739,33.612499999876,11.5671105274575));
#288179=CARTESIAN_POINT('Ctrl Pts',(7.51676407774783,33.7624999998754,10.3459381770593));
#288180=CARTESIAN_POINT('Ctrl Pts',(9.83957192047905,33.9124999998748,7.14886745759543));
#288181=CARTESIAN_POINT('Ctrl Pts',(12.1623797632103,34.0624999998742,3.95179673813153));
#288182=CARTESIAN_POINT('Ctrl Pts',(12.1623797632103,34.2124999998736,-1.489461944703E-15));
#288183=CARTESIAN_POINT('Ctrl Pts',(12.1623797632103,34.362499999873,-3.95179673813154));
#288184=CARTESIAN_POINT('Ctrl Pts',(9.83957192047904,34.5124999998724,-7.14886745759543));
#288185=CARTESIAN_POINT('Ctrl Pts',(7.51676407774783,34.6624999998718,-10.3459381770593));
#288186=CARTESIAN_POINT('Ctrl Pts',(3.7583820388739,34.8124999998712,-11.5671105274575));
#288187=CARTESIAN_POINT('Ctrl Pts',(-3.33956917070458E-14,34.9624999998706,
-12.7882828778556));
#288188=CARTESIAN_POINT('Ctrl Pts',(-3.75838203887396,35.11249999987,-11.5671105274575));
#288189=CARTESIAN_POINT('Ctrl Pts',(-7.51676407774789,35.2624999998694,
-10.3459381770593));
#288190=CARTESIAN_POINT('Ctrl Pts',(-9.83957192047911,35.4124999998688,
-7.14886745759543));
#288191=CARTESIAN_POINT('Ctrl Pts',(-12.1623797632103,35.5624999998682,
-3.95179673813153));
#288192=CARTESIAN_POINT('Ctrl Pts',(-12.1623797632103,35.7124999998676,
2.97892388940601E-15));
#288193=CARTESIAN_POINT('Ctrl Pts',(-12.1623797632103,35.862499999867,3.95179673813154));
#288194=CARTESIAN_POINT('Ctrl Pts',(-9.83957192047911,36.0124999998664,
7.14886745759543));
#288195=CARTESIAN_POINT('Ctrl Pts',(-7.51676407774789,36.1624999998658,
10.3459381770593));
#288196=CARTESIAN_POINT('Ctrl Pts',(-3.75838203887396,36.3124999998652,
11.5671105274575));
#288197=CARTESIAN_POINT('Ctrl Pts',(-3.11273204042854E-14,36.4624999998646,
12.7882828778556));
#288198=CARTESIAN_POINT('Ctrl Pts',(3.7583820388739,36.612499999864,11.5671105274575));
#288199=CARTESIAN_POINT('Ctrl Pts',(7.51676407774783,36.7624999998634,10.3459381770593));
#288200=CARTESIAN_POINT('Ctrl Pts',(9.83957192047904,36.9124999998628,7.14886745759543));
#288201=CARTESIAN_POINT('Ctrl Pts',(12.1623797632103,37.0624999998622,3.95179673813153));
#288202=CARTESIAN_POINT('Ctrl Pts',(12.1623797632103,37.2124999998616,-1.489461944703E-15));
#288203=CARTESIAN_POINT('Ctrl Pts',(12.1623797632103,37.362499999861,-3.95179673813154));
#288204=CARTESIAN_POINT('Ctrl Pts',(9.83957192047904,37.5124999998604,-7.14886745759543));
#288205=CARTESIAN_POINT('Ctrl Pts',(7.51676407774782,37.6624999998598,-10.3459381770593));
#288206=CARTESIAN_POINT('Ctrl Pts',(3.75838203887389,37.8124999998592,-11.5671105274575));
#288207=CARTESIAN_POINT('Ctrl Pts',(-3.51234009787076E-14,37.9624999998586,
-12.7882828778556));
#288208=CARTESIAN_POINT('Ctrl Pts',(-3.75838203887396,38.112499999858,-11.5671105274575));
#288209=CARTESIAN_POINT('Ctrl Pts',(-7.51676407774789,38.2624999998574,
-10.3459381770593));
#288210=CARTESIAN_POINT('Ctrl Pts',(-9.83957192047911,38.4124999998568,
-7.14886745759543));
#288211=CARTESIAN_POINT('Ctrl Pts',(-12.1623797632103,38.5624999998562,
-3.95179673813153));
#288212=CARTESIAN_POINT('Ctrl Pts',(-12.1623797632103,38.7124999998556,
2.97892388940601E-15));
#288213=CARTESIAN_POINT('Ctrl Pts',(-12.1623797632103,38.862499999855,3.95179673813154));
#288214=CARTESIAN_POINT('Ctrl Pts',(-9.83957192047911,39.0124999998544,
7.14886745759543));
#288215=CARTESIAN_POINT('Ctrl Pts',(-7.51676407774789,39.1624999998538,
10.3459381770593));
#288216=CARTESIAN_POINT('Ctrl Pts',(-3.75838203887396,39.3124999998532,
11.5671105274575));
#288217=CARTESIAN_POINT('Ctrl Pts',(-3.28550296759472E-14,39.4624999998526,
12.7882828778556));
#288218=CARTESIAN_POINT('Ctrl Pts',(3.7583820388739,39.612499999852,11.5671105274575));
#288219=CARTESIAN_POINT('Ctrl Pts',(7.51676407774782,39.7624999998514,10.3459381770593));
#288220=CARTESIAN_POINT('Ctrl Pts',(9.83957192047904,39.9124999998508,7.14886745759543));
#288221=CARTESIAN_POINT('Ctrl Pts',(12.1623797632103,40.0624999998502,3.95179673813153));
#288222=CARTESIAN_POINT('Ctrl Pts',(12.1623797632103,40.2124999998496,-1.489461944703E-15));
#288223=CARTESIAN_POINT('Ctrl Pts',(12.1623797632103,40.362499999849,-3.95179673813154));
#288224=CARTESIAN_POINT('Ctrl Pts',(9.83957192047904,40.5124999998484,-7.14886745759543));
#288225=CARTESIAN_POINT('Ctrl Pts',(7.51676407774782,40.6624999998478,-10.3459381770593));
#288226=CARTESIAN_POINT('Ctrl Pts',(3.75838203887389,40.8124999998472,-11.5671105274575));
#288227=CARTESIAN_POINT('Ctrl Pts',(-3.68511102503695E-14,40.9624999998466,
-12.7882828778556));
#288228=CARTESIAN_POINT('Ctrl Pts',(-3.75838203887397,41.112499999846,-11.5671105274575));
#288229=CARTESIAN_POINT('Ctrl Pts',(-7.51676407774789,41.2624999998454,
-10.3459381770593));
#288230=CARTESIAN_POINT('Ctrl Pts',(-9.83957192047911,41.4124999998448,
-7.14886745759543));
#288231=CARTESIAN_POINT('Ctrl Pts',(-12.1623797632103,41.5624999998442,
-3.95179673813153));
#288232=CARTESIAN_POINT('Ctrl Pts',(-12.1623797632103,41.7124999998436,
2.97892388940601E-15));
#288233=CARTESIAN_POINT('Ctrl Pts',(-12.1623797632103,41.862499999843,3.95179673813154));
#288234=CARTESIAN_POINT('Ctrl Pts',(-9.83957192047911,42.0124999998424,
7.14886745759543));
#288235=CARTESIAN_POINT('Ctrl Pts',(-7.51676407774789,42.1624999998418,
10.3459381770593));
#288236=CARTESIAN_POINT('Ctrl Pts',(-3.75838203887396,42.3124999998412,
11.5671105274575));
#288237=CARTESIAN_POINT('Ctrl Pts',(-3.4582738947609E-14,42.4624999998406,
12.7882828778556));
#288238=CARTESIAN_POINT('Ctrl Pts',(3.75838203887389,42.61249999984,11.5671105274575));
#288239=CARTESIAN_POINT('Ctrl Pts',(7.51676407774782,42.7624999998394,10.3459381770593));
#288240=CARTESIAN_POINT('Ctrl Pts',(9.83957192047904,42.9124999998388,7.14886745759543));
#288241=CARTESIAN_POINT('Ctrl Pts',(12.1623797632103,43.0624999998382,3.95179673813153));
#288242=CARTESIAN_POINT('Ctrl Pts',(12.1623797632103,43.2124999998376,-1.489461944703E-15));
#288243=CARTESIAN_POINT('Ctrl Pts',(12.1623797632103,43.362499999837,-3.95179673813154));
#288244=CARTESIAN_POINT('Ctrl Pts',(9.83957192047903,43.5124999998364,-7.14886745759543));
#288245=CARTESIAN_POINT('Ctrl Pts',(7.51676407774782,43.6624999998358,-10.3459381770593));
#288246=CARTESIAN_POINT('Ctrl Pts',(3.75838203887389,43.8124999998352,-11.5671105274575));
#288247=CARTESIAN_POINT('Ctrl Pts',(-3.85788195220313E-14,43.9624999998346,
-12.7882828778556));
#288248=CARTESIAN_POINT('Ctrl Pts',(-3.75838203887397,44.112499999834,-11.5671105274575));
#288249=CARTESIAN_POINT('Ctrl Pts',(-7.5167640777479,44.2624999998334,-10.3459381770593));
#288250=CARTESIAN_POINT('Ctrl Pts',(-9.83957192047911,44.4124999998328,
-7.14886745759543));
#288251=CARTESIAN_POINT('Ctrl Pts',(-12.1623797632103,44.5624999998322,
-3.95179673813153));
#288252=CARTESIAN_POINT('Ctrl Pts',(-12.1623797632103,44.7124999998316,
2.97892388940601E-15));
#288253=CARTESIAN_POINT('Ctrl Pts',(-12.1623797632103,44.862499999831,3.95179673813154));
#288254=CARTESIAN_POINT('Ctrl Pts',(-9.83957192047911,45.0124999998304,
7.14886745759543));
#288255=CARTESIAN_POINT('Ctrl Pts',(-7.51676407774789,45.1624999998298,
10.3459381770593));
#288256=CARTESIAN_POINT('Ctrl Pts',(-3.75838203887397,45.3124999998292,
11.5671105274575));
#288257=CARTESIAN_POINT('Ctrl Pts',(-3.63104482192709E-14,45.4624999998286,
12.7882828778556));
#288258=CARTESIAN_POINT('Ctrl Pts',(3.75838203887389,45.612499999828,11.5671105274575));
#288259=CARTESIAN_POINT('Ctrl Pts',(7.51676407774782,45.7624999998274,10.3459381770593));
#288260=CARTESIAN_POINT('Ctrl Pts',(9.83957192047904,45.9124999998268,7.14886745759543));
#288261=CARTESIAN_POINT('Ctrl Pts',(12.1623797632103,46.0624999998262,3.95179673813153));
#288262=CARTESIAN_POINT('Ctrl Pts',(12.1623797632103,46.2124999998256,-1.489461944703E-15));
#288263=CARTESIAN_POINT('Ctrl Pts',(12.1623797632103,46.362499999825,-3.95179673813154));
#288264=CARTESIAN_POINT('Ctrl Pts',(9.83957192047903,46.5124999998244,-7.14886745759543));
#288265=CARTESIAN_POINT('Ctrl Pts',(7.51676407774782,46.6624999998238,-10.3459381770593));
#288266=CARTESIAN_POINT('Ctrl Pts',(3.75838203887389,46.8124999998232,-11.5671105274575));
#288267=CARTESIAN_POINT('Ctrl Pts',(-4.03065287936931E-14,46.9624999998226,
-12.7882828778556));
#288268=CARTESIAN_POINT('Ctrl Pts',(-3.75838203887397,47.112499999822,-11.5671105274575));
#288269=CARTESIAN_POINT('Ctrl Pts',(-7.5167640777479,47.2624999998214,-10.3459381770593));
#288270=CARTESIAN_POINT('Ctrl Pts',(-9.83957192047912,47.4124999998208,
-7.14886745759543));
#288271=CARTESIAN_POINT('Ctrl Pts',(-12.1623797632103,47.5624999998202,
-3.95179673813153));
#288272=CARTESIAN_POINT('Ctrl Pts',(-12.1623797632103,47.7124999998196,
2.97892388940601E-15));
#288273=CARTESIAN_POINT('Ctrl Pts',(-12.1623797632103,47.862499999819,3.95179673813154));
#288274=CARTESIAN_POINT('Ctrl Pts',(-9.83957192047911,48.0124999998184,
7.14886745759543));
#288275=CARTESIAN_POINT('Ctrl Pts',(-7.51676407774789,48.1624999998178,
10.3459381770593));
#288276=CARTESIAN_POINT('Ctrl Pts',(-3.75838203887397,48.3124999998172,
11.5671105274575));
#288277=CARTESIAN_POINT('Ctrl Pts',(-3.80381574909327E-14,48.4624999998166,
12.7882828778556));
#288278=CARTESIAN_POINT('Ctrl Pts',(3.75838203887389,48.612499999816,11.5671105274575));
#288279=CARTESIAN_POINT('Ctrl Pts',(7.51676407774782,48.7624999998154,10.3459381770593));
#288280=CARTESIAN_POINT('Ctrl Pts',(9.83957192047903,48.9124999998148,7.14886745759543));
#288281=CARTESIAN_POINT('Ctrl Pts',(12.1623797632103,49.0624999998142,3.95179673813153));
#288282=CARTESIAN_POINT('Ctrl Pts',(12.1623797632103,49.2124999998136,-1.489461944703E-15));
#288283=CARTESIAN_POINT('Ctrl Pts',(12.1623797632103,49.362499999813,-3.95179673813154));
#288284=CARTESIAN_POINT('Ctrl Pts',(9.83957192047903,49.5124999998124,-7.14886745759543));
#288285=CARTESIAN_POINT('Ctrl Pts',(7.51676407774782,49.6624999998118,-10.3459381770593));
#288286=CARTESIAN_POINT('Ctrl Pts',(3.75838203887389,49.8124999998112,-11.5671105274575));
#288287=CARTESIAN_POINT('Ctrl Pts',(-4.2034238065355E-14,49.9624999998106,
-12.7882828778556));
#288288=CARTESIAN_POINT('Ctrl Pts',(-3.75838203887397,50.11249999981,-11.5671105274575));
#288289=CARTESIAN_POINT('Ctrl Pts',(-7.5167640777479,50.2624999998094,-10.3459381770593));
#288290=CARTESIAN_POINT('Ctrl Pts',(-9.83957192047912,50.4124999998088,
-7.14886745759543));
#288291=CARTESIAN_POINT('Ctrl Pts',(-12.1623797632103,50.5624999998082,
-3.95179673813153));
#288292=CARTESIAN_POINT('Ctrl Pts',(-12.1623797632103,50.7124999998076,
2.97892388940601E-15));
#288293=CARTESIAN_POINT('Ctrl Pts',(-12.1623797632103,50.862499999807,3.95179673813154));
#288294=CARTESIAN_POINT('Ctrl Pts',(-9.83957192047912,51.0124999998064,
7.14886745759543));
#288295=CARTESIAN_POINT('Ctrl Pts',(-7.5167640777479,51.1624999998058,10.3459381770593));
#288296=CARTESIAN_POINT('Ctrl Pts',(-3.75838203887397,51.3124999998052,
11.5671105274575));
#288297=CARTESIAN_POINT('Ctrl Pts',(-3.97658667625946E-14,51.4624999998046,
12.7882828778556));
#288298=CARTESIAN_POINT('Ctrl Pts',(3.75838203887389,51.612499999804,11.5671105274575));
#288299=CARTESIAN_POINT('Ctrl Pts',(7.51676407774782,51.7624999998034,10.3459381770593));
#288300=CARTESIAN_POINT('Ctrl Pts',(9.83957192047903,51.9124999998028,7.14886745759543));
#288301=CARTESIAN_POINT('Ctrl Pts',(12.1623797632103,52.0624999998022,3.95179673813153));
#288302=CARTESIAN_POINT('Ctrl Pts',(12.1623797632103,52.2124999998016,-1.489461944703E-15));
#288303=CARTESIAN_POINT('Ctrl Pts',(12.1623797632103,52.362499999801,-3.95179673813154));
#288304=CARTESIAN_POINT('Ctrl Pts',(9.83957192047903,52.5124999998004,-7.14886745759543));
#288305=CARTESIAN_POINT('Ctrl Pts',(7.51676407774781,52.6624999997998,-10.3459381770593));
#288306=CARTESIAN_POINT('Ctrl Pts',(3.75838203887388,52.8124999997992,-11.5671105274575));
#288307=CARTESIAN_POINT('Ctrl Pts',(-4.37619473370168E-14,52.9624999997986,
-12.7882828778556));
#288308=CARTESIAN_POINT('Ctrl Pts',(-3.75838203887397,53.112499999798,-11.5671105274575));
#288309=CARTESIAN_POINT('Ctrl Pts',(-7.5167640777479,53.2624999997974,-10.3459381770593));
#288310=CARTESIAN_POINT('Ctrl Pts',(-9.83957192047912,53.4124999997968,
-7.14886745759543));
#288311=CARTESIAN_POINT('Ctrl Pts',(-12.1623797632103,53.5624999997962,
-3.95179673813153));
#288312=CARTESIAN_POINT('Ctrl Pts',(-12.1623797632103,53.7124999997956,
2.97892388940601E-15));
#288313=CARTESIAN_POINT('Ctrl Pts',(-12.1623797632103,53.862499999795,3.95179673813154));
#288314=CARTESIAN_POINT('Ctrl Pts',(-9.83957192047912,54.0124999997944,
7.14886745759543));
#288315=CARTESIAN_POINT('Ctrl Pts',(-7.5167640777479,54.1624999997938,10.3459381770593));
#288316=CARTESIAN_POINT('Ctrl Pts',(-3.75838203887397,54.3124999997932,
11.5671105274575));
#288317=CARTESIAN_POINT('Ctrl Pts',(-4.14935760342564E-14,54.4624999997926,
12.7882828778556));
#288318=CARTESIAN_POINT('Ctrl Pts',(3.75838203887389,54.612499999792,11.5671105274575));
#288319=CARTESIAN_POINT('Ctrl Pts',(7.51676407774782,54.7624999997914,10.3459381770593));
#288320=CARTESIAN_POINT('Ctrl Pts',(9.83957192047903,54.9124999997908,7.14886745759543));
#288321=CARTESIAN_POINT('Ctrl Pts',(12.1623797632103,55.0624999997902,3.95179673813153));
#288322=CARTESIAN_POINT('Ctrl Pts',(12.1623797632103,55.2124999997896,-1.489461944703E-15));
#288323=CARTESIAN_POINT('Ctrl Pts',(12.1623797632103,55.362499999789,-3.95179673813154));
#288324=CARTESIAN_POINT('Ctrl Pts',(9.83957192047903,55.5124999997884,-7.14886745759543));
#288325=CARTESIAN_POINT('Ctrl Pts',(7.51676407774781,55.6624999997878,-10.3459381770593));
#288326=CARTESIAN_POINT('Ctrl Pts',(3.75838203887388,55.8124999997872,-11.5671105274575));
#288327=CARTESIAN_POINT('Ctrl Pts',(-4.54896566086787E-14,55.9624999997866,
-12.7882828778556));
#288328=CARTESIAN_POINT('Ctrl Pts',(-3.75838203887397,56.112499999786,-11.5671105274575));
#288329=CARTESIAN_POINT('Ctrl Pts',(-7.5167640777479,56.2624999997854,-10.3459381770593));
#288330=CARTESIAN_POINT('Ctrl Pts',(-9.83957192047912,56.4124999997848,
-7.14886745759543));
#288331=CARTESIAN_POINT('Ctrl Pts',(-12.1623797632103,56.5624999997842,
-3.95179673813153));
#288332=CARTESIAN_POINT('Ctrl Pts',(-12.1623797632103,56.7124999997836,
2.97892388940601E-15));
#288333=CARTESIAN_POINT('Ctrl Pts',(-12.1623797632103,56.862499999783,3.95179673813154));
#288334=CARTESIAN_POINT('Ctrl Pts',(-9.83957192047912,57.0124999997824,
7.14886745759543));
#288335=CARTESIAN_POINT('Ctrl Pts',(-7.5167640777479,57.1624999997818,10.3459381770593));
#288336=CARTESIAN_POINT('Ctrl Pts',(-3.75838203887397,57.3124999997812,
11.5671105274575));
#288337=CARTESIAN_POINT('Ctrl Pts',(-4.32212853059182E-14,57.4624999997806,
12.7882828778556));
#288338=CARTESIAN_POINT('Ctrl Pts',(3.75838203887389,57.61249999978,11.5671105274575));
#288339=CARTESIAN_POINT('Ctrl Pts',(7.51676407774781,57.7624999997794,10.3459381770593));
#288340=CARTESIAN_POINT('Ctrl Pts',(9.83957192047903,57.9124999997788,7.14886745759543));
#288341=CARTESIAN_POINT('Ctrl Pts',(12.1623797632103,58.0624999997782,3.95179673813153));
#288342=CARTESIAN_POINT('Ctrl Pts',(12.1623797632102,58.2124999997776,-1.489461944703E-15));
#288343=CARTESIAN_POINT('Ctrl Pts',(12.1623797632102,58.362499999777,-3.95179673813154));
#288344=CARTESIAN_POINT('Ctrl Pts',(9.83957192047903,58.5124999997764,-7.14886745759543));
#288345=CARTESIAN_POINT('Ctrl Pts',(7.51676407774781,58.6624999997758,-10.3459381770593));
#288346=CARTESIAN_POINT('Ctrl Pts',(3.75838203887388,58.8124999997752,-11.5671105274575));
#288347=CARTESIAN_POINT('Ctrl Pts',(-4.72173658803405E-14,58.9624999997746,
-12.7882828778556));
#288348=CARTESIAN_POINT('Ctrl Pts',(-3.75838203887398,59.112499999774,-11.5671105274575));
#288349=CARTESIAN_POINT('Ctrl Pts',(-7.51676407774791,59.2624999997734,
-10.3459381770593));
#288350=CARTESIAN_POINT('Ctrl Pts',(-9.83957192047912,59.4124999997728,
-7.14886745759543));
#288351=CARTESIAN_POINT('Ctrl Pts',(-12.1623797632103,59.5624999997722,
-3.95179673813153));
#288352=CARTESIAN_POINT('Ctrl Pts',(-12.1623797632103,59.7124999997716,
2.97892388940601E-15));
#288353=CARTESIAN_POINT('Ctrl Pts',(-12.1623797632103,59.862499999771,3.95179673813154));
#288354=CARTESIAN_POINT('Ctrl Pts',(-9.83957192047912,60.0124999997704,
7.14886745759543));
#288355=CARTESIAN_POINT('Ctrl Pts',(-7.5167640777479,60.1624999997698,10.3459381770593));
#288356=CARTESIAN_POINT('Ctrl Pts',(-3.75838203887397,60.3124999997692,
11.5671105274575));
#288357=CARTESIAN_POINT('Ctrl Pts',(-4.49489945775801E-14,60.4624999997686,
12.7882828778556));
#288358=CARTESIAN_POINT('Ctrl Pts',(3.75838203887388,60.612499999768,11.5671105274575));
#288359=CARTESIAN_POINT('Ctrl Pts',(7.51676407774781,60.7624999997674,10.3459381770593));
#288360=CARTESIAN_POINT('Ctrl Pts',(9.83957192047903,60.9124999997668,7.14886745759543));
#288361=CARTESIAN_POINT('Ctrl Pts',(12.1623797632103,61.0624999997662,3.95179673813153));
#288362=CARTESIAN_POINT('Ctrl Pts',(12.1623797632102,61.2124999997656,-1.489461944703E-15));
#288363=CARTESIAN_POINT('Ctrl Pts',(12.1623797632102,61.362499999765,-3.95179673813154));
#288364=CARTESIAN_POINT('Ctrl Pts',(9.83957192047902,61.5124999997644,-7.14886745759543));
#288365=CARTESIAN_POINT('Ctrl Pts',(7.51676407774781,61.6624999997638,-10.3459381770593));
#288366=CARTESIAN_POINT('Ctrl Pts',(3.75838203887388,61.8124999997632,-11.5671105274575));
#288367=CARTESIAN_POINT('Ctrl Pts',(-4.89450751520023E-14,61.9624999997626,
-12.7882828778556));
#288368=CARTESIAN_POINT('Ctrl Pts',(-3.75838203887398,62.112499999762,-11.5671105274575));
#288369=CARTESIAN_POINT('Ctrl Pts',(-7.51676407774791,62.2624999997614,
-10.3459381770593));
#288370=CARTESIAN_POINT('Ctrl Pts',(-9.83957192047912,62.4124999997608,
-7.14886745759543));
#288371=CARTESIAN_POINT('Ctrl Pts',(-12.1623797632103,62.5624999997602,
-3.95179673813153));
#288372=CARTESIAN_POINT('Ctrl Pts',(-12.1623797632103,62.7124999997596,
2.97892388940601E-15));
#288373=CARTESIAN_POINT('Ctrl Pts',(-12.1623797632103,62.862499999759,3.95179673813154));
#288374=CARTESIAN_POINT('Ctrl Pts',(-9.83957192047912,63.0124999997584,
7.14886745759543));
#288375=CARTESIAN_POINT('Ctrl Pts',(-7.5167640777479,63.1624999997578,10.3459381770593));
#288376=CARTESIAN_POINT('Ctrl Pts',(-3.75838203887398,63.3124999997572,
11.5671105274575));
#288377=CARTESIAN_POINT('Ctrl Pts',(-4.66767038492419E-14,63.4624999997566,
12.7882828778556));
#288378=CARTESIAN_POINT('Ctrl Pts',(3.75838203887388,63.612499999756,11.5671105274575));
#288379=CARTESIAN_POINT('Ctrl Pts',(7.51676407774781,63.7624999997554,10.3459381770593));
#288380=CARTESIAN_POINT('Ctrl Pts',(9.83957192047903,63.9124999997548,7.14886745759543));
#288381=CARTESIAN_POINT('Ctrl Pts',(12.1623797632102,64.0624999997542,3.95179673813153));
#288382=CARTESIAN_POINT('Ctrl Pts',(12.1623797632102,64.2124999997536,-1.489461944703E-15));
#288383=CARTESIAN_POINT('Ctrl Pts',(12.1623797632102,64.362499999753,-3.95179673813154));
#288384=CARTESIAN_POINT('Ctrl Pts',(9.83957192047902,64.5124999997524,-7.14886745759543));
#288385=CARTESIAN_POINT('Ctrl Pts',(7.51676407774781,64.6624999997518,-10.3459381770593));
#288386=CARTESIAN_POINT('Ctrl Pts',(3.75838203887388,64.8124999997512,-11.5671105274575));
#288387=CARTESIAN_POINT('Ctrl Pts',(-5.06727844236642E-14,64.9624999997506,
-12.7882828778556));
#288388=CARTESIAN_POINT('Ctrl Pts',(-3.75838203887398,65.11249999975,-11.5671105274575));
#288389=CARTESIAN_POINT('Ctrl Pts',(-7.51676407774791,65.2624999997494,
-10.3459381770593));
#288390=CARTESIAN_POINT('Ctrl Pts',(-9.83957192047913,65.4124999997488,
-7.14886745759543));
#288391=CARTESIAN_POINT('Ctrl Pts',(-12.1623797632103,65.5624999997482,
-3.95179673813153));
#288392=CARTESIAN_POINT('Ctrl Pts',(-12.1623797632103,65.7124999997476,
2.97892388940601E-15));
#288393=CARTESIAN_POINT('Ctrl Pts',(-12.1623797632103,65.862499999747,3.95179673813154));
#288394=CARTESIAN_POINT('Ctrl Pts',(-9.83957192047912,66.0124999997464,
7.14886745759543));
#288395=CARTESIAN_POINT('Ctrl Pts',(-7.51676407774791,66.1624999997458,
10.3459381770593));
#288396=CARTESIAN_POINT('Ctrl Pts',(-3.75838203887398,66.3124999997452,
11.5671105274575));
#288397=CARTESIAN_POINT('Ctrl Pts',(-4.84044131209037E-14,66.4624999997446,
12.7882828778556));
#288398=CARTESIAN_POINT('Ctrl Pts',(3.75838203887388,66.612499999744,11.5671105274575));
#288399=CARTESIAN_POINT('Ctrl Pts',(7.51676407774781,66.7624999997434,10.3459381770593));
#288400=CARTESIAN_POINT('Ctrl Pts',(9.83957192047902,66.9124999997428,7.14886745759543));
#288401=CARTESIAN_POINT('Ctrl Pts',(12.1623797632102,67.0624999997422,3.95179673813153));
#288402=CARTESIAN_POINT('Ctrl Pts',(12.1623797632102,67.2124999997416,-1.489461944703E-15));
#288403=CARTESIAN_POINT('Ctrl Pts',(12.1623797632102,67.362499999741,-3.95179673813154));
#288404=CARTESIAN_POINT('Ctrl Pts',(9.83957192047902,67.5124999997404,-7.14886745759543));
#288405=CARTESIAN_POINT('Ctrl Pts',(7.51676407774781,67.6624999997398,-10.3459381770593));
#288406=CARTESIAN_POINT('Ctrl Pts',(3.75838203887388,67.8124999997392,-11.5671105274575));
#288407=CARTESIAN_POINT('Ctrl Pts',(-5.2400493695326E-14,67.9624999997386,
-12.7882828778556));
#288408=CARTESIAN_POINT('Ctrl Pts',(-3.75838203887398,68.112499999738,-11.5671105274575));
#288409=CARTESIAN_POINT('Ctrl Pts',(-7.51676407774791,68.2624999997374,
-10.3459381770593));
#288410=CARTESIAN_POINT('Ctrl Pts',(-9.83957192047913,68.4124999997368,
-7.14886745759543));
#288411=CARTESIAN_POINT('Ctrl Pts',(-12.1623797632103,68.5624999997362,
-3.95179673813153));
#288412=CARTESIAN_POINT('Ctrl Pts',(-12.1623797632103,68.7124999997356,
2.97892388940601E-15));
#288413=CARTESIAN_POINT('Ctrl Pts',(-12.1623797632103,68.862499999735,3.95179673813154));
#288414=CARTESIAN_POINT('Ctrl Pts',(-9.83957192047913,69.0124999997344,
7.14886745759543));
#288415=CARTESIAN_POINT('Ctrl Pts',(-7.51676407774791,69.1624999997338,
10.3459381770593));
#288416=CARTESIAN_POINT('Ctrl Pts',(-3.75838203887398,69.3124999997332,
11.5671105274575));
#288417=CARTESIAN_POINT('Ctrl Pts',(-5.01321223925656E-14,69.4624999997326,
12.7882828778556));
#288418=CARTESIAN_POINT('Ctrl Pts',(3.75838203887388,69.612499999732,11.5671105274575));
#288419=CARTESIAN_POINT('Ctrl Pts',(7.51676407774781,69.7624999997314,10.3459381770593));
#288420=CARTESIAN_POINT('Ctrl Pts',(9.83957192047902,69.9124999997308,7.14886745759543));
#288421=CARTESIAN_POINT('Ctrl Pts',(12.1623797632102,70.0624999997302,3.95179673813153));
#288422=CARTESIAN_POINT('Ctrl Pts',(12.1623797632102,70.2124999997296,-1.489461944703E-15));
#288423=CARTESIAN_POINT('Ctrl Pts',(12.1623797632102,70.362499999729,-3.95179673813154));
#288424=CARTESIAN_POINT('Ctrl Pts',(9.83957192047902,70.5124999997284,-7.14886745759543));
#288425=CARTESIAN_POINT('Ctrl Pts',(7.5167640777478,70.6624999997278,-10.3459381770593));
#288426=CARTESIAN_POINT('Ctrl Pts',(3.75838203887388,70.8124999997272,-11.5671105274575));
#288427=CARTESIAN_POINT('Ctrl Pts',(-5.41282029669879E-14,70.9624999997266,
-12.7882828778556));
#288428=CARTESIAN_POINT('Ctrl Pts',(-3.75838203887398,71.112499999726,-11.5671105274575));
#288429=CARTESIAN_POINT('Ctrl Pts',(-7.51676407774791,71.2624999997254,
-10.3459381770593));
#288430=CARTESIAN_POINT('Ctrl Pts',(-9.83957192047913,71.4124999997248,
-7.14886745759543));
#288431=CARTESIAN_POINT('Ctrl Pts',(-12.1623797632103,71.5624999997242,
-3.95179673813153));
#288432=CARTESIAN_POINT('Ctrl Pts',(-12.1623797632103,71.7124999997236,
2.97892388940601E-15));
#288433=CARTESIAN_POINT('Ctrl Pts',(-12.1623797632103,71.862499999723,3.95179673813154));
#288434=CARTESIAN_POINT('Ctrl Pts',(-9.83957192047913,72.0124999997224,
7.14886745759543));
#288435=CARTESIAN_POINT('Ctrl Pts',(-7.51676407774791,72.1624999997218,
10.3459381770593));
#288436=CARTESIAN_POINT('Ctrl Pts',(-3.75838203887398,72.3124999997212,
11.5671105274575));
#288437=CARTESIAN_POINT('Ctrl Pts',(-5.18598316642274E-14,72.4624999997206,
12.7882828778556));
#288438=CARTESIAN_POINT('Ctrl Pts',(3.75838203887388,72.61249999972,11.5671105274575));
#288439=CARTESIAN_POINT('Ctrl Pts',(7.51676407774781,72.7624999997194,10.3459381770593));
#288440=CARTESIAN_POINT('Ctrl Pts',(9.83957192047902,72.9124999997188,7.14886745759543));
#288441=CARTESIAN_POINT('Ctrl Pts',(12.1623797632102,73.0624999997182,3.95179673813153));
#288442=CARTESIAN_POINT('Ctrl Pts',(12.1623797632102,73.2124999997176,-1.489461944703E-15));
#288443=CARTESIAN_POINT('Ctrl Pts',(12.1623797632102,73.362499999717,-3.95179673813154));
#288444=CARTESIAN_POINT('Ctrl Pts',(9.83957192047902,73.5124999997164,-7.14886745759543));
#288445=CARTESIAN_POINT('Ctrl Pts',(7.5167640777478,73.6624999997158,-10.3459381770593));
#288446=CARTESIAN_POINT('Ctrl Pts',(3.75838203887387,73.8124999997152,-11.5671105274575));
#288447=CARTESIAN_POINT('Ctrl Pts',(-5.58559122386497E-14,73.9624999997146,
-12.7882828778556));
#288448=CARTESIAN_POINT('Ctrl Pts',(-3.75838203887398,74.112499999714,-11.5671105274575));
#288449=CARTESIAN_POINT('Ctrl Pts',(-7.51676407774791,74.2624999997134,
-10.3459381770593));
#288450=CARTESIAN_POINT('Ctrl Pts',(-9.83957192047913,74.4124999997128,
-7.14886745759543));
#288451=CARTESIAN_POINT('Ctrl Pts',(-12.1623797632103,74.5624999997122,
-3.95179673813153));
#288452=CARTESIAN_POINT('Ctrl Pts',(-12.1623797632103,74.7124999997116,
2.97892388940601E-15));
#288453=CARTESIAN_POINT('Ctrl Pts',(-12.1623797632103,74.862499999711,3.95179673813154));
#288454=CARTESIAN_POINT('Ctrl Pts',(-9.83957192047913,75.0124999997104,
7.14886745759543));
#288455=CARTESIAN_POINT('Ctrl Pts',(-7.51676407774791,75.1624999997098,
10.3459381770593));
#288456=CARTESIAN_POINT('Ctrl Pts',(-3.75838203887398,75.3124999997092,
11.5671105274575));
#288457=CARTESIAN_POINT('Ctrl Pts',(-5.35875409358893E-14,75.4624999997086,
12.7882828778556));
#288458=CARTESIAN_POINT('Ctrl Pts',(3.75838203887388,75.612499999708,11.5671105274575));
#288459=CARTESIAN_POINT('Ctrl Pts',(7.5167640777478,75.7624999997074,10.3459381770593));
#288460=CARTESIAN_POINT('Ctrl Pts',(9.83957192047902,75.9124999997068,7.14886745759543));
#288461=CARTESIAN_POINT('Ctrl Pts',(12.1623797632102,76.0624999997062,3.95179673813153));
#288462=CARTESIAN_POINT('Ctrl Pts',(12.1623797632102,76.2124999997056,-1.489461944703E-15));
#288463=CARTESIAN_POINT('Ctrl Pts',(12.1623797632102,76.362499999705,-3.95179673813154));
#288464=CARTESIAN_POINT('Ctrl Pts',(9.83957192047902,76.5124999997044,-7.14886745759543));
#288465=CARTESIAN_POINT('Ctrl Pts',(7.5167640777478,76.6624999997038,-10.3459381770593));
#288466=CARTESIAN_POINT('Ctrl Pts',(3.75838203887387,76.8124999997032,-11.5671105274575));
#288467=CARTESIAN_POINT('Ctrl Pts',(-5.75836215103115E-14,76.9624999997026,
-12.7882828778556));
#288468=CARTESIAN_POINT('Ctrl Pts',(-3.75838203887399,77.112499999702,-11.5671105274575));
#288469=CARTESIAN_POINT('Ctrl Pts',(-7.51676407774791,77.2624999997014,
-10.3459381770593));
#288470=CARTESIAN_POINT('Ctrl Pts',(-9.83957192047913,77.4124999997008,
-7.14886745759543));
#288471=CARTESIAN_POINT('Ctrl Pts',(-12.1623797632103,77.5624999997002,
-3.95179673813153));
#288472=CARTESIAN_POINT('Ctrl Pts',(-12.1623797632103,77.7124999996996,
2.97892388940601E-15));
#288473=CARTESIAN_POINT('Ctrl Pts',(-12.1623797632103,77.862499999699,3.95179673813154));
#288474=CARTESIAN_POINT('Ctrl Pts',(-9.83957192047913,78.0124999996984,
7.14886745759543));
#288475=CARTESIAN_POINT('Ctrl Pts',(-7.51676407774791,78.1624999996978,
10.3459381770593));
#288476=CARTESIAN_POINT('Ctrl Pts',(-3.75838203887398,78.3124999996972,
11.5671105274575));
#288477=CARTESIAN_POINT('Ctrl Pts',(-5.53152502075511E-14,78.4624999996966,
12.7882828778556));
#288478=CARTESIAN_POINT('Ctrl Pts',(3.75838203887387,78.612499999696,11.5671105274575));
#288479=CARTESIAN_POINT('Ctrl Pts',(7.5167640777478,78.7624999996954,10.3459381770593));
#288480=CARTESIAN_POINT('Ctrl Pts',(9.83957192047902,78.9124999996948,7.14886745759543));
#288481=CARTESIAN_POINT('Ctrl Pts',(12.1623797632102,79.0624999996942,3.95179673813153));
#288482=CARTESIAN_POINT('Ctrl Pts',(12.1623797632102,79.2124999996936,-1.489461944703E-15));
#288483=CARTESIAN_POINT('Ctrl Pts',(12.1623797632102,79.362499999693,-3.95179673813154));
#288484=CARTESIAN_POINT('Ctrl Pts',(9.83957192047902,79.5124999996924,-7.14886745759543));
#288485=CARTESIAN_POINT('Ctrl Pts',(7.5167640777478,79.6624999996918,-10.3459381770593));
#288486=CARTESIAN_POINT('Ctrl Pts',(3.75838203887387,79.8124999996912,-11.5671105274575));
#288487=CARTESIAN_POINT('Ctrl Pts',(-5.93113307819734E-14,79.9624999996906,
-12.7882828778556));
#288488=CARTESIAN_POINT('Ctrl Pts',(-3.75838203887399,80.11249999969,-11.5671105274575));
#288489=CARTESIAN_POINT('Ctrl Pts',(-7.51676407774791,80.2624999996894,
-10.3459381770593));
#288490=CARTESIAN_POINT('Ctrl Pts',(-9.83957192047913,80.4124999996888,
-7.14886745759543));
#288491=CARTESIAN_POINT('Ctrl Pts',(-12.1623797632104,80.5624999996882,
-3.95179673813153));
#288492=CARTESIAN_POINT('Ctrl Pts',(-12.1623797632104,80.7124999996876,
2.97892388940601E-15));
#288493=CARTESIAN_POINT('Ctrl Pts',(-12.1623797632104,80.862499999687,3.95179673813154));
#288494=CARTESIAN_POINT('Ctrl Pts',(-9.83957192047913,81.0124999996864,
7.14886745759543));
#288495=CARTESIAN_POINT('Ctrl Pts',(-7.51676407774791,81.1624999996858,
10.3459381770593));
#288496=CARTESIAN_POINT('Ctrl Pts',(-3.75838203887399,81.3124999996852,
11.5671105274575));
#288497=CARTESIAN_POINT('Ctrl Pts',(-5.70429594792129E-14,81.4624999996846,
12.7882828778556));
#288498=CARTESIAN_POINT('Ctrl Pts',(3.75838203887387,81.612499999684,11.5671105274575));
#288499=CARTESIAN_POINT('Ctrl Pts',(7.5167640777478,81.7624999996834,10.3459381770593));
#288500=CARTESIAN_POINT('Ctrl Pts',(9.83957192047902,81.9124999996828,7.14886745759543));
#288501=CARTESIAN_POINT('Ctrl Pts',(12.1623797632102,82.0624999996822,3.95179673813153));
#288502=CARTESIAN_POINT('Ctrl Pts',(12.1623797632102,82.2124999996816,-1.489461944703E-15));
#288503=CARTESIAN_POINT('Ctrl Pts',(12.1623797632102,82.362499999681,-3.95179673813154));
#288504=CARTESIAN_POINT('Ctrl Pts',(9.83957192047902,82.5124999996804,-7.14886745759543));
#288505=CARTESIAN_POINT('Ctrl Pts',(7.5167640777478,82.6624999996798,-10.3459381770593));
#288506=CARTESIAN_POINT('Ctrl Pts',(3.75838203887387,82.8124999996792,-11.5671105274575));
#288507=CARTESIAN_POINT('Ctrl Pts',(-6.10390400536352E-14,82.9624999996786,
-12.7882828778556));
#288508=CARTESIAN_POINT('Ctrl Pts',(-3.75838203887399,83.112499999678,-11.5671105274575));
#288509=CARTESIAN_POINT('Ctrl Pts',(-7.51676407774792,83.2624999996774,
-10.3459381770593));
#288510=CARTESIAN_POINT('Ctrl Pts',(-9.83957192047914,83.4124999996768,
-7.14886745759543));
#288511=CARTESIAN_POINT('Ctrl Pts',(-12.1623797632104,83.5624999996762,
-3.95179673813153));
#288512=CARTESIAN_POINT('Ctrl Pts',(-12.1623797632104,83.7124999996756,
2.97892388940601E-15));
#288513=CARTESIAN_POINT('Ctrl Pts',(-12.1623797632104,83.862499999675,3.95179673813154));
#288514=CARTESIAN_POINT('Ctrl Pts',(-9.83957192047913,84.0124999996744,
7.14886745759543));
#288515=CARTESIAN_POINT('Ctrl Pts',(-7.51676407774791,84.1624999996738,
10.3459381770593));
#288516=CARTESIAN_POINT('Ctrl Pts',(-3.75838203887399,84.3124999996732,
11.5671105274575));
#288517=CARTESIAN_POINT('Ctrl Pts',(-5.87706687508748E-14,84.4624999996726,
12.7882828778556));
#288518=CARTESIAN_POINT('Ctrl Pts',(3.75838203887387,84.6124999996721,11.5671105274575));
#288519=CARTESIAN_POINT('Ctrl Pts',(7.5167640777478,84.7624999996714,10.3459381770593));
#288520=CARTESIAN_POINT('Ctrl Pts',(9.83957192047902,84.9124999996708,7.14886745759543));
#288521=CARTESIAN_POINT('Ctrl Pts',(12.1623797632102,85.0624999996702,3.95179673813153));
#288522=CARTESIAN_POINT('Ctrl Pts',(12.1623797632102,85.2124999996696,-1.489461944703E-15));
#288523=CARTESIAN_POINT('Ctrl Pts',(12.1623797632102,85.362499999669,-3.95179673813154));
#288524=CARTESIAN_POINT('Ctrl Pts',(9.83957192047901,85.5124999996684,-7.14886745759543));
#288525=CARTESIAN_POINT('Ctrl Pts',(7.5167640777478,85.6624999996678,-10.3459381770593));
#288526=CARTESIAN_POINT('Ctrl Pts',(3.75838203887387,85.8124999996672,-11.5671105274575));
#288527=CARTESIAN_POINT('Ctrl Pts',(-6.27667493252971E-14,85.9624999996666,
-12.7882828778556));
#288528=CARTESIAN_POINT('Ctrl Pts',(-3.75838203887399,86.112499999666,-11.5671105274575));
#288529=CARTESIAN_POINT('Ctrl Pts',(-7.51676407774792,86.2624999996654,
-10.3459381770593));
#288530=CARTESIAN_POINT('Ctrl Pts',(-9.83957192047914,86.4124999996648,
-7.14886745759543));
#288531=CARTESIAN_POINT('Ctrl Pts',(-12.1623797632104,86.5624999996642,
-3.95179673813153));
#288532=CARTESIAN_POINT('Ctrl Pts',(-12.1623797632104,86.7124999996636,
2.97892388940601E-15));
#288533=CARTESIAN_POINT('Ctrl Pts',(-12.1623797632104,86.862499999663,3.95179673813154));
#288534=CARTESIAN_POINT('Ctrl Pts',(-9.83957192047914,87.0124999996624,
7.14886745759543));
#288535=CARTESIAN_POINT('Ctrl Pts',(-7.51676407774792,87.1624999996618,
10.3459381770593));
#288536=CARTESIAN_POINT('Ctrl Pts',(-3.75838203887399,87.3124999996612,
11.5671105274575));
#288537=CARTESIAN_POINT('Ctrl Pts',(-6.04983780225366E-14,87.4624999996606,
12.7882828778556));
#288538=CARTESIAN_POINT('Ctrl Pts',(3.75838203887387,87.61249999966,11.5671105274575));
#288539=CARTESIAN_POINT('Ctrl Pts',(7.5167640777478,87.7624999996594,10.3459381770593));
#288540=CARTESIAN_POINT('Ctrl Pts',(9.83957192047901,87.9124999996588,7.14886745759543));
#288541=CARTESIAN_POINT('Ctrl Pts',(12.1623797632102,88.0624999996582,3.95179673813153));
#288542=CARTESIAN_POINT('Ctrl Pts',(12.1623797632102,88.2124999996576,-1.489461944703E-15));
#288543=CARTESIAN_POINT('Ctrl Pts',(12.1623797632102,88.362499999657,-3.95179673813154));
#288544=CARTESIAN_POINT('Ctrl Pts',(9.83957192047901,88.5124999996564,-7.14886745759543));
#288545=CARTESIAN_POINT('Ctrl Pts',(7.51676407774779,88.6624999996558,-10.3459381770593));
#288546=CARTESIAN_POINT('Ctrl Pts',(3.75838203887386,88.8124999996552,-11.5671105274575));
#288547=CARTESIAN_POINT('Ctrl Pts',(-6.44944585969589E-14,88.9624999996546,
-12.7882828778556));
#288548=CARTESIAN_POINT('Ctrl Pts',(-3.75838203887399,89.112499999654,-11.5671105274575));
#288549=CARTESIAN_POINT('Ctrl Pts',(-7.51676407774792,89.2624999996534,
-10.3459381770593));
#288550=CARTESIAN_POINT('Ctrl Pts',(-9.83957192047914,89.4124999996528,
-7.14886745759543));
#288551=CARTESIAN_POINT('Ctrl Pts',(-12.1623797632104,89.5624999996522,
-3.95179673813153));
#288552=CARTESIAN_POINT('Ctrl Pts',(-12.1623797632104,89.7124999996516,
2.97892388940601E-15));
#288553=CARTESIAN_POINT('Ctrl Pts',(-12.1623797632104,89.862499999651,3.95179673813154));
#288554=CARTESIAN_POINT('Ctrl Pts',(-9.83957192047914,90.0124999996504,
7.14886745759543));
#288555=CARTESIAN_POINT('Ctrl Pts',(-7.51676407774792,90.1624999996498,
10.3459381770593));
#288556=CARTESIAN_POINT('Ctrl Pts',(-3.75838203887399,90.3124999996492,
11.5671105274575));
#288557=CARTESIAN_POINT('Ctrl Pts',(-6.22260872941985E-14,90.4624999996486,
12.7882828778556));
#288558=CARTESIAN_POINT('Ctrl Pts',(3.75838203887387,90.612499999648,11.5671105274575));
#288559=CARTESIAN_POINT('Ctrl Pts',(7.5167640777478,90.7624999996474,10.3459381770593));
#288560=CARTESIAN_POINT('Ctrl Pts',(9.83957192047901,90.9124999996468,7.14886745759543));
#288561=CARTESIAN_POINT('Ctrl Pts',(12.1623797632102,91.0624999996462,3.95179673813153));
#288562=CARTESIAN_POINT('Ctrl Pts',(12.1623797632102,91.2124999996456,-1.489461944703E-15));
#288563=CARTESIAN_POINT('Ctrl Pts',(12.1623797632102,91.362499999645,-3.95179673813154));
#288564=CARTESIAN_POINT('Ctrl Pts',(9.83957192047901,91.5124999996444,-7.14886745759543));
#288565=CARTESIAN_POINT('Ctrl Pts',(7.51676407774779,91.6624999996438,-10.3459381770593));
#288566=CARTESIAN_POINT('Ctrl Pts',(3.75838203887386,91.8124999996432,-11.5671105274575));
#288567=CARTESIAN_POINT('Ctrl Pts',(-6.62221678686207E-14,91.9624999996426,
-12.7882828778556));
#288568=CARTESIAN_POINT('Ctrl Pts',(-3.75838203887399,92.112499999642,-11.5671105274575));
#288569=CARTESIAN_POINT('Ctrl Pts',(-7.51676407774792,92.2624999996414,
-10.3459381770593));
#288570=CARTESIAN_POINT('Ctrl Pts',(-9.83957192047914,92.4124999996408,
-7.14886745759543));
#288571=CARTESIAN_POINT('Ctrl Pts',(-12.1623797632104,92.5624999996402,
-3.95179673813153));
#288572=CARTESIAN_POINT('Ctrl Pts',(-12.1623797632104,92.7124999996396,
2.97892388940601E-15));
#288573=CARTESIAN_POINT('Ctrl Pts',(-12.1623797632104,92.862499999639,3.95179673813154));
#288574=CARTESIAN_POINT('Ctrl Pts',(-9.83957192047914,93.0124999996384,
7.14886745759543));
#288575=CARTESIAN_POINT('Ctrl Pts',(-7.51676407774792,93.1624999996378,
10.3459381770593));
#288576=CARTESIAN_POINT('Ctrl Pts',(-3.75838203887399,93.3124999996372,
11.5671105274575));
#288577=CARTESIAN_POINT('Ctrl Pts',(-6.39537965658603E-14,93.4624999996366,
12.7882828778556));
#288578=CARTESIAN_POINT('Ctrl Pts',(3.75838203887386,93.612499999636,11.5671105274575));
#288579=CARTESIAN_POINT('Ctrl Pts',(7.51676407774779,93.7624999996354,10.3459381770593));
#288580=CARTESIAN_POINT('Ctrl Pts',(9.83957192047901,93.9124999996348,7.14886745759543));
#288581=CARTESIAN_POINT('Ctrl Pts',(12.1623797632102,94.0624999996342,3.95179673813153));
#288582=CARTESIAN_POINT('Ctrl Pts',(12.1623797632102,94.2124999996336,-1.489461944703E-15));
#288583=CARTESIAN_POINT('Ctrl Pts',(12.1623797632102,94.362499999633,-3.95179673813154));
#288584=CARTESIAN_POINT('Ctrl Pts',(9.83957192047901,94.5124999996324,-7.14886745759543));
#288585=CARTESIAN_POINT('Ctrl Pts',(7.51676407774779,94.6624999996318,-10.3459381770593));
#288586=CARTESIAN_POINT('Ctrl Pts',(3.75838203887386,94.8124999996312,-11.5671105274575));
#288587=CARTESIAN_POINT('Ctrl Pts',(-6.79498771402825E-14,94.9624999996306,
-12.7882828778556));
#288588=CARTESIAN_POINT('Ctrl Pts',(-3.758382038874,95.11249999963,-11.5671105274575));
#288589=CARTESIAN_POINT('Ctrl Pts',(-7.51676407774792,95.2624999996294,
-10.3459381770593));
#288590=CARTESIAN_POINT('Ctrl Pts',(-9.83957192047914,95.4124999996288,
-7.14886745759543));
#288591=CARTESIAN_POINT('Ctrl Pts',(-12.1623797632104,95.5624999996282,
-3.95179673813153));
#288592=CARTESIAN_POINT('Ctrl Pts',(-12.1623797632104,95.7124999996276,
2.97892388940601E-15));
#288593=CARTESIAN_POINT('Ctrl Pts',(-12.1623797632104,95.862499999627,3.95179673813154));
#288594=CARTESIAN_POINT('Ctrl Pts',(-9.83957192047914,96.0124999996264,
7.14886745759543));
#288595=CARTESIAN_POINT('Ctrl Pts',(-7.51676407774792,96.1624999996258,
10.3459381770593));
#288596=CARTESIAN_POINT('Ctrl Pts',(-3.75838203887399,96.3124999996252,
11.5671105274575));
#288597=CARTESIAN_POINT('Ctrl Pts',(-6.56815058375222E-14,96.4624999996246,
12.7882828778556));
#288598=CARTESIAN_POINT('Ctrl Pts',(3.75838203887386,96.612499999624,11.5671105274575));
#288599=CARTESIAN_POINT('Ctrl Pts',(7.51676407774779,96.7624999996234,10.3459381770593));
#288600=CARTESIAN_POINT('Ctrl Pts',(9.83957192047901,96.9124999996228,7.14886745759543));
#288601=CARTESIAN_POINT('Ctrl Pts',(12.1623797632102,97.0624999996222,3.95179673813153));
#288602=CARTESIAN_POINT('Ctrl Pts',(12.1623797632102,97.2124999996216,-1.489461944703E-15));
#288603=CARTESIAN_POINT('Ctrl Pts',(12.1623797632102,97.3624999996211,-3.95179673813154));
#288604=CARTESIAN_POINT('Ctrl Pts',(9.83957192047901,97.5124999996204,-7.14886745759543));
#288605=CARTESIAN_POINT('Ctrl Pts',(7.51676407774779,97.6624999996198,-10.3459381770593));
#288606=CARTESIAN_POINT('Ctrl Pts',(3.75838203887386,97.8124999996192,-11.5671105274575));
#288607=CARTESIAN_POINT('Ctrl Pts',(-6.96775864119444E-14,97.9624999996187,
-12.7882828778556));
#288608=CARTESIAN_POINT('Ctrl Pts',(-3.758382038874,98.112499999618,-11.5671105274575));
#288609=CARTESIAN_POINT('Ctrl Pts',(-7.51676407774793,98.2624999996174,
-10.3459381770593));
#288610=CARTESIAN_POINT('Ctrl Pts',(-9.83957192047914,98.4124999996168,
-7.14886745759543));
#288611=CARTESIAN_POINT('Ctrl Pts',(-12.1623797632104,98.5624999996162,
-3.95179673813153));
#288612=CARTESIAN_POINT('Ctrl Pts',(-12.1623797632104,98.7124999996156,
2.97892388940601E-15));
#288613=CARTESIAN_POINT('Ctrl Pts',(-12.1623797632104,98.862499999615,3.95179673813154));
#288614=CARTESIAN_POINT('Ctrl Pts',(-9.83957192047914,99.0124999996144,
7.14886745759543));
#288615=CARTESIAN_POINT('Ctrl Pts',(-7.51676407774792,99.1624999996138,
10.3459381770593));
#288616=CARTESIAN_POINT('Ctrl Pts',(-3.758382038874,99.3124999996132,11.5671105274575));
#288617=CARTESIAN_POINT('Ctrl Pts',(-6.7409215109184E-14,99.4624999996126,
12.7882828778556));
#288618=CARTESIAN_POINT('Ctrl Pts',(3.75838203887386,99.612499999612,11.5671105274575));
#288619=CARTESIAN_POINT('Ctrl Pts',(7.51676407774779,99.7624999996114,10.3459381770593));
#288620=CARTESIAN_POINT('Ctrl Pts',(9.83957192047901,99.9124999996108,7.14886745759543));
#288621=CARTESIAN_POINT('Ctrl Pts',(12.1623797632102,100.06249999961,3.95179673813153));
#288622=CARTESIAN_POINT('Ctrl Pts',(12.1623797632102,100.21249999961,-1.489461944703E-15));
#288623=CARTESIAN_POINT('Ctrl Pts',(12.1623797632102,100.362499999609,-3.95179673813154));
#288624=CARTESIAN_POINT('Ctrl Pts',(9.839571920479,100.512499999608,-7.14886745759543));
#288625=CARTESIAN_POINT('Ctrl Pts',(7.51676407774779,100.662499999608,-10.3459381770593));
#288626=CARTESIAN_POINT('Ctrl Pts',(3.75838203887386,100.812499999607,-11.5671105274575));
#288627=CARTESIAN_POINT('Ctrl Pts',(-7.14052956836063E-14,100.962499999607,
-12.7882828778556));
#288628=CARTESIAN_POINT('Ctrl Pts',(-3.758382038874,101.112499999606,-11.5671105274575));
#288629=CARTESIAN_POINT('Ctrl Pts',(-7.51676407774793,101.262499999605,
-10.3459381770593));
#288630=CARTESIAN_POINT('Ctrl Pts',(-9.83957192047915,101.412499999605,
-7.14886745759543));
#288631=CARTESIAN_POINT('Ctrl Pts',(-12.1623797632104,101.562499999604,
-3.95179673813153));
#288632=CARTESIAN_POINT('Ctrl Pts',(-12.1623797632104,101.712499999604,
2.97892388940601E-15));
#288633=CARTESIAN_POINT('Ctrl Pts',(-12.1623797632104,101.862499999603,
3.95179673813154));
#288634=CARTESIAN_POINT('Ctrl Pts',(-9.83957192047914,102.012499999602,
7.14886745759543));
#288635=CARTESIAN_POINT('Ctrl Pts',(-7.51676407774793,102.162499999602,
10.3459381770593));
#288636=CARTESIAN_POINT('Ctrl Pts',(-3.758382038874,102.312499999601,11.5671105274575));
#288637=CARTESIAN_POINT('Ctrl Pts',(-6.91369243808458E-14,102.462499999601,
12.7882828778556));
#288638=CARTESIAN_POINT('Ctrl Pts',(3.75838203887386,102.6124999996,11.5671105274575));
#288639=CARTESIAN_POINT('Ctrl Pts',(7.51676407774779,102.762499999599,10.3459381770593));
#288640=CARTESIAN_POINT('Ctrl Pts',(9.839571920479,102.912499999599,7.14886745759543));
#288641=CARTESIAN_POINT('Ctrl Pts',(12.1623797632102,103.062499999598,3.95179673813153));
#288642=CARTESIAN_POINT('Ctrl Pts',(12.1623797632102,103.212499999598,-1.489461944703E-15));
#288643=CARTESIAN_POINT('Ctrl Pts',(12.1623797632102,103.362499999597,-3.95179673813154));
#288644=CARTESIAN_POINT('Ctrl Pts',(9.839571920479,103.512499999596,-7.14886745759543));
#288645=CARTESIAN_POINT('Ctrl Pts',(7.51676407774779,103.662499999596,-10.3459381770593));
#288646=CARTESIAN_POINT('Ctrl Pts',(3.75838203887386,103.812499999595,-11.5671105274575));
#288647=CARTESIAN_POINT('Ctrl Pts',(-7.31330049552681E-14,103.962499999595,
-12.7882828778556));
#288648=CARTESIAN_POINT('Ctrl Pts',(-3.758382038874,104.112499999594,-11.5671105274575));
#288649=CARTESIAN_POINT('Ctrl Pts',(-7.51676407774793,104.262499999593,
-10.3459381770593));
#288650=CARTESIAN_POINT('Ctrl Pts',(-9.83957192047915,104.412499999593,
-7.14886745759543));
#288651=CARTESIAN_POINT('Ctrl Pts',(-12.1623797632104,104.562499999592,
-3.95179673813153));
#288652=CARTESIAN_POINT('Ctrl Pts',(-12.1623797632104,104.712499999592,
2.97892388940601E-15));
#288653=CARTESIAN_POINT('Ctrl Pts',(-12.1623797632104,104.862499999591,
3.95179673813154));
#288654=CARTESIAN_POINT('Ctrl Pts',(-9.83957192047915,105.01249999959,7.14886745759543));
#288655=CARTESIAN_POINT('Ctrl Pts',(-7.51676407774793,105.16249999959,10.3459381770593));
#288656=CARTESIAN_POINT('Ctrl Pts',(-3.758382038874,105.312499999589,11.5671105274575));
#288657=CARTESIAN_POINT('Ctrl Pts',(-7.08646336525076E-14,105.462499999589,
12.7882828778556));
#288658=CARTESIAN_POINT('Ctrl Pts',(3.75838203887386,105.612499999588,11.5671105274575));
#288659=CARTESIAN_POINT('Ctrl Pts',(7.51676407774779,105.762499999587,10.3459381770593));
#288660=CARTESIAN_POINT('Ctrl Pts',(9.839571920479,105.912499999587,7.14886745759543));
#288661=CARTESIAN_POINT('Ctrl Pts',(12.1623797632102,106.062499999586,3.95179673813153));
#288662=CARTESIAN_POINT('Ctrl Pts',(12.1623797632102,106.212499999586,-1.489461944703E-15));
#288663=CARTESIAN_POINT('Ctrl Pts',(12.1623797632102,106.362499999585,-3.95179673813154));
#288664=CARTESIAN_POINT('Ctrl Pts',(9.839571920479,106.512499999584,-7.14886745759543));
#288665=CARTESIAN_POINT('Ctrl Pts',(7.51676407774778,106.662499999584,-10.3459381770593));
#288666=CARTESIAN_POINT('Ctrl Pts',(3.75838203887385,106.812499999583,-11.5671105274575));
#288667=CARTESIAN_POINT('Ctrl Pts',(-7.48607142269299E-14,106.962499999583,
-12.7882828778556));
#288668=CARTESIAN_POINT('Ctrl Pts',(-3.758382038874,107.112499999582,-11.5671105274575));
#288669=CARTESIAN_POINT('Ctrl Pts',(-7.51676407774793,107.262499999581,
-10.3459381770593));
#288670=CARTESIAN_POINT('Ctrl Pts',(-9.83957192047915,107.412499999581,
-7.14886745759543));
#288671=CARTESIAN_POINT('Ctrl Pts',(-12.1623797632104,107.56249999958,-3.95179673813153));
#288672=CARTESIAN_POINT('Ctrl Pts',(-12.1623797632104,107.71249999958,2.97892388940601E-15));
#288673=CARTESIAN_POINT('Ctrl Pts',(-12.1623797632104,107.862499999579,
3.95179673813154));
#288674=CARTESIAN_POINT('Ctrl Pts',(-9.83957192047915,108.012499999578,
7.14886745759543));
#288675=CARTESIAN_POINT('Ctrl Pts',(-7.51676407774793,108.162499999578,
10.3459381770593));
#288676=CARTESIAN_POINT('Ctrl Pts',(-3.758382038874,108.312499999577,11.5671105274575));
#288677=CARTESIAN_POINT('Ctrl Pts',(-7.25923429241695E-14,108.462499999577,
12.7882828778556));
#288678=CARTESIAN_POINT('Ctrl Pts',(3.75838203887386,108.612499999576,11.5671105274575));
#288679=CARTESIAN_POINT('Ctrl Pts',(7.51676407774779,108.762499999575,10.3459381770593));
#288680=CARTESIAN_POINT('Ctrl Pts',(9.839571920479,108.912499999575,7.14886745759543));
#288681=CARTESIAN_POINT('Ctrl Pts',(12.1623797632102,109.062499999574,3.95179673813153));
#288682=CARTESIAN_POINT('Ctrl Pts',(12.1623797632102,109.212499999574,-1.489461944703E-15));
#288683=CARTESIAN_POINT('Ctrl Pts',(12.1623797632102,109.362499999573,-3.95179673813154));
#288684=CARTESIAN_POINT('Ctrl Pts',(9.839571920479,109.512499999572,-7.14886745759543));
#288685=CARTESIAN_POINT('Ctrl Pts',(7.51676407774778,109.662499999572,-10.3459381770593));
#288686=CARTESIAN_POINT('Ctrl Pts',(3.75838203887385,109.812499999571,-11.5671105274575));
#288687=CARTESIAN_POINT('Ctrl Pts',(-7.65884234985918E-14,109.962499999571,
-12.7882828778556));
#288688=CARTESIAN_POINT('Ctrl Pts',(-3.75838203887401,110.11249999957,-11.5671105274575));
#288689=CARTESIAN_POINT('Ctrl Pts',(-7.51676407774793,110.262499999569,
-10.3459381770593));
#288690=CARTESIAN_POINT('Ctrl Pts',(-9.83957192047915,110.412499999569,
-7.14886745759543));
#288691=CARTESIAN_POINT('Ctrl Pts',(-12.1623797632104,110.562499999568,
-3.95179673813153));
#288692=CARTESIAN_POINT('Ctrl Pts',(-12.1623797632104,110.712499999568,
2.97892388940601E-15));
#288693=CARTESIAN_POINT('Ctrl Pts',(-12.1623797632104,110.862499999567,
3.95179673813154));
#288694=CARTESIAN_POINT('Ctrl Pts',(-9.83957192047915,111.012499999566,
7.14886745759543));
#288695=CARTESIAN_POINT('Ctrl Pts',(-7.51676407774793,111.162499999566,
10.3459381770593));
#288696=CARTESIAN_POINT('Ctrl Pts',(-3.758382038874,111.312499999565,11.5671105274575));
#288697=CARTESIAN_POINT('Ctrl Pts',(-7.43200521958313E-14,111.462499999565,
12.7882828778556));
#288698=CARTESIAN_POINT('Ctrl Pts',(3.75838203887385,111.612499999564,11.5671105274575));
#288699=CARTESIAN_POINT('Ctrl Pts',(7.51676407774778,111.762499999563,10.3459381770593));
#288700=CARTESIAN_POINT('Ctrl Pts',(9.839571920479,111.912499999563,7.14886745759543));
#288701=CARTESIAN_POINT('Ctrl Pts',(12.1623797632102,112.062499999562,3.95179673813153));
#288702=CARTESIAN_POINT('Ctrl Pts',(12.1623797632102,112.212499999562,-1.489461944703E-15));
#288703=CARTESIAN_POINT('Ctrl Pts',(12.1623797632102,112.362499999561,-3.95179673813154));
#288704=CARTESIAN_POINT('Ctrl Pts',(9.839571920479,112.51249999956,-7.14886745759543));
#288705=CARTESIAN_POINT('Ctrl Pts',(7.51676407774778,112.66249999956,-10.3459381770593));
#288706=CARTESIAN_POINT('Ctrl Pts',(3.75838203887385,112.812499999559,-11.5671105274575));
#288707=CARTESIAN_POINT('Ctrl Pts',(-7.83161327702536E-14,112.962499999559,
-12.7882828778556));
#288708=CARTESIAN_POINT('Ctrl Pts',(-3.75838203887401,113.112499999558,
-11.5671105274575));
#288709=CARTESIAN_POINT('Ctrl Pts',(-7.51676407774793,113.262499999557,
-10.3459381770593));
#288710=CARTESIAN_POINT('Ctrl Pts',(-9.83957192047915,113.412499999557,
-7.14886745759543));
#288711=CARTESIAN_POINT('Ctrl Pts',(-12.1623797632104,113.562499999556,
-3.95179673813153));
#288712=CARTESIAN_POINT('Ctrl Pts',(-12.1623797632104,113.712499999556,
2.97892388940601E-15));
#288713=CARTESIAN_POINT('Ctrl Pts',(-12.1623797632104,113.862499999555,
3.95179673813154));
#288714=CARTESIAN_POINT('Ctrl Pts',(-9.83957192047915,114.012499999554,
7.14886745759543));
#288715=CARTESIAN_POINT('Ctrl Pts',(-7.51676407774793,114.162499999554,
10.3459381770593));
#288716=CARTESIAN_POINT('Ctrl Pts',(-3.758382038874,114.312499999553,11.5671105274575));
#288717=CARTESIAN_POINT('Ctrl Pts',(-7.60477614674932E-14,114.462499999553,
12.7882828778556));
#288718=CARTESIAN_POINT('Ctrl Pts',(3.75838203887385,114.612499999552,11.5671105274575));
#288719=CARTESIAN_POINT('Ctrl Pts',(7.51676407774778,114.762499999551,10.3459381770593));
#288720=CARTESIAN_POINT('Ctrl Pts',(9.839571920479,114.912499999551,7.14886745759543));
#288721=CARTESIAN_POINT('Ctrl Pts',(12.1623797632102,115.06249999955,3.95179673813153));
#288722=CARTESIAN_POINT('Ctrl Pts',(12.1623797632102,115.21249999955,-1.489461944703E-15));
#288723=CARTESIAN_POINT('Ctrl Pts',(12.1623797632102,115.362499999549,-3.95179673813154));
#288724=CARTESIAN_POINT('Ctrl Pts',(9.839571920479,115.512499999548,-7.14886745759543));
#288725=CARTESIAN_POINT('Ctrl Pts',(7.51676407774778,115.662499999548,-10.3459381770593));
#288726=CARTESIAN_POINT('Ctrl Pts',(3.75838203887385,115.812499999547,-11.5671105274575));
#288727=CARTESIAN_POINT('Ctrl Pts',(-8.00438420419154E-14,115.962499999547,
-12.7882828778556));
#288728=CARTESIAN_POINT('Ctrl Pts',(-3.75838203887401,116.112499999546,
-11.5671105274575));
#288729=CARTESIAN_POINT('Ctrl Pts',(-7.51676407774794,116.262499999545,
-10.3459381770593));
#288730=CARTESIAN_POINT('Ctrl Pts',(-9.83957192047916,116.412499999545,
-7.14886745759543));
#288731=CARTESIAN_POINT('Ctrl Pts',(-12.1623797632104,116.562499999544,
-3.95179673813153));
#288732=CARTESIAN_POINT('Ctrl Pts',(-12.1623797632104,116.712499999544,
2.97892388940601E-15));
#288733=CARTESIAN_POINT('Ctrl Pts',(-12.1623797632104,116.862499999543,
3.95179673813154));
#288734=CARTESIAN_POINT('Ctrl Pts',(-9.83957192047915,117.012499999542,
7.14886745759543));
#288735=CARTESIAN_POINT('Ctrl Pts',(-7.51676407774793,117.162499999542,
10.3459381770593));
#288736=CARTESIAN_POINT('Ctrl Pts',(-3.75838203887401,117.312499999541,
11.5671105274575));
#288737=CARTESIAN_POINT('Ctrl Pts',(-7.7775470739155E-14,117.462499999541,
12.7882828778556));
#288738=CARTESIAN_POINT('Ctrl Pts',(3.75838203887385,117.61249999954,11.5671105274575));
#288739=CARTESIAN_POINT('Ctrl Pts',(7.51676407774778,117.762499999539,10.3459381770593));
#288740=CARTESIAN_POINT('Ctrl Pts',(9.839571920479,117.912499999539,7.14886745759543));
#288741=CARTESIAN_POINT('Ctrl Pts',(12.1623797632102,118.062499999538,3.95179673813153));
#288742=CARTESIAN_POINT('Ctrl Pts',(12.1623797632102,118.212499999538,-1.489461944703E-15));
#288743=CARTESIAN_POINT('Ctrl Pts',(12.1623797632102,118.362499999537,-3.95179673813154));
#288744=CARTESIAN_POINT('Ctrl Pts',(9.83957192047899,118.512499999536,-7.14886745759543));
#288745=CARTESIAN_POINT('Ctrl Pts',(7.51676407774778,118.662499999536,-10.3459381770593));
#288746=CARTESIAN_POINT('Ctrl Pts',(3.75838203887385,118.812499999535,-11.5671105274575));
#288747=CARTESIAN_POINT('Ctrl Pts',(-8.17715513135773E-14,118.962499999535,
-12.7882828778556));
#288748=CARTESIAN_POINT('Ctrl Pts',(-3.75838203887401,119.112499999534,
-11.5671105274575));
#288749=CARTESIAN_POINT('Ctrl Pts',(-7.51676407774794,119.262499999533,
-10.3459381770593));
#288750=CARTESIAN_POINT('Ctrl Pts',(-9.83957192047916,119.412499999533,
-7.14886745759543));
#288751=CARTESIAN_POINT('Ctrl Pts',(-12.1623797632104,119.562499999532,
-3.95179673813153));
#288752=CARTESIAN_POINT('Ctrl Pts',(-12.1623797632104,119.712499999532,
2.97892388940601E-15));
#288753=CARTESIAN_POINT('Ctrl Pts',(-12.1623797632104,119.862499999531,
3.95179673813154));
#288754=CARTESIAN_POINT('Ctrl Pts',(-9.83957192047916,120.01249999953,7.14886745759543));
#288755=CARTESIAN_POINT('Ctrl Pts',(-7.51676407774794,120.16249999953,10.3459381770593));
#288756=CARTESIAN_POINT('Ctrl Pts',(-3.75838203887401,120.312499999529,
11.5671105274575));
#288757=CARTESIAN_POINT('Ctrl Pts',(-7.95031800108169E-14,120.462499999529,
12.7882828778556));
#288758=CARTESIAN_POINT('Ctrl Pts',(3.75838203887385,120.612499999528,11.5671105274575));
#288759=CARTESIAN_POINT('Ctrl Pts',(7.51676407774778,120.762499999527,10.3459381770593));
#288760=CARTESIAN_POINT('Ctrl Pts',(9.83957192047899,120.912499999527,7.14886745759543));
#288761=CARTESIAN_POINT('Ctrl Pts',(12.1623797632102,121.062499999526,3.95179673813153));
#288762=CARTESIAN_POINT('Ctrl Pts',(12.1623797632102,121.212499999526,-1.489461944703E-15));
#288763=CARTESIAN_POINT('Ctrl Pts',(12.1623797632102,121.362499999525,-3.95179673813154));
#288764=CARTESIAN_POINT('Ctrl Pts',(9.83957192047899,121.512499999524,-7.14886745759543));
#288765=CARTESIAN_POINT('Ctrl Pts',(7.51676407774777,121.662499999524,-10.3459381770593));
#288766=CARTESIAN_POINT('Ctrl Pts',(3.75838203887385,121.812499999523,-11.5671105274575));
#288767=CARTESIAN_POINT('Ctrl Pts',(-8.34992605852391E-14,121.962499999523,
-12.7882828778556));
#288768=CARTESIAN_POINT('Ctrl Pts',(-3.75838203887401,122.112499999522,
-11.5671105274575));
#288769=CARTESIAN_POINT('Ctrl Pts',(-7.51676407774794,122.262499999521,
-10.3459381770593));
#288770=CARTESIAN_POINT('Ctrl Pts',(-9.83957192047916,122.412499999521,
-7.14886745759543));
#288771=CARTESIAN_POINT('Ctrl Pts',(-12.1623797632104,122.56249999952,-3.95179673813153));
#288772=CARTESIAN_POINT('Ctrl Pts',(-12.1623797632104,122.71249999952,2.97892388940601E-15));
#288773=CARTESIAN_POINT('Ctrl Pts',(-12.1623797632104,122.862499999519,
3.95179673813154));
#288774=CARTESIAN_POINT('Ctrl Pts',(-9.83957192047916,123.012499999518,
7.14886745759543));
#288775=CARTESIAN_POINT('Ctrl Pts',(-7.51676407774794,123.162499999518,
10.3459381770593));
#288776=CARTESIAN_POINT('Ctrl Pts',(-3.75838203887401,123.312499999517,
11.5671105274575));
#288777=CARTESIAN_POINT('Ctrl Pts',(-8.12308892824787E-14,123.462499999517,
12.7882828778556));
#288778=CARTESIAN_POINT('Ctrl Pts',(3.75838203887385,123.612499999516,11.5671105274575));
#288779=CARTESIAN_POINT('Ctrl Pts',(7.51676407774778,123.762499999515,10.3459381770593));
#288780=CARTESIAN_POINT('Ctrl Pts',(9.83957192047899,123.912499999515,7.14886745759543));
#288781=CARTESIAN_POINT('Ctrl Pts',(12.1623797632102,124.062499999514,3.95179673813153));
#288782=CARTESIAN_POINT('Ctrl Pts',(12.1623797632102,124.212499999514,-1.489461944703E-15));
#288783=CARTESIAN_POINT('Ctrl Pts',(12.1623797632102,124.362499999513,-3.95179673813154));
#288784=CARTESIAN_POINT('Ctrl Pts',(9.83957192047899,124.512499999512,-7.14886745759543));
#288785=CARTESIAN_POINT('Ctrl Pts',(7.51676407774777,124.662499999512,-10.3459381770593));
#288786=CARTESIAN_POINT('Ctrl Pts',(3.75838203887384,124.812499999511,-11.5671105274575));
#288787=CARTESIAN_POINT('Ctrl Pts',(-8.52269698569009E-14,124.962499999511,
-12.7882828778556));
#288788=CARTESIAN_POINT('Ctrl Pts',(-3.75838203887401,125.11249999951,-11.5671105274575));
#288789=CARTESIAN_POINT('Ctrl Pts',(-7.51676407774794,125.262499999509,
-10.3459381770593));
#288790=CARTESIAN_POINT('Ctrl Pts',(-9.83957192047916,125.412499999509,
-7.14886745759543));
#288791=CARTESIAN_POINT('Ctrl Pts',(-12.1623797632104,125.562499999508,
-3.95179673813153));
#288792=CARTESIAN_POINT('Ctrl Pts',(-12.1623797632104,125.712499999508,
2.97892388940601E-15));
#288793=CARTESIAN_POINT('Ctrl Pts',(-12.1623797632104,125.862499999507,
3.95179673813154));
#288794=CARTESIAN_POINT('Ctrl Pts',(-9.83957192047916,126.012499999506,
7.14886745759543));
#288795=CARTESIAN_POINT('Ctrl Pts',(-7.51676407774794,126.162499999506,
10.3459381770593));
#288796=CARTESIAN_POINT('Ctrl Pts',(-3.75838203887401,126.312499999505,
11.5671105274575));
#288797=CARTESIAN_POINT('Ctrl Pts',(-8.29585985541405E-14,126.462499999505,
12.7882828778556));
#288798=CARTESIAN_POINT('Ctrl Pts',(3.75838203887385,126.612499999504,11.5671105274575));
#288799=CARTESIAN_POINT('Ctrl Pts',(7.51676407774777,126.762499999503,10.3459381770593));
#288800=CARTESIAN_POINT('Ctrl Pts',(9.83957192047899,126.912499999503,7.14886745759543));
#288801=CARTESIAN_POINT('Ctrl Pts',(12.1623797632102,127.062499999502,3.95179673813153));
#288802=CARTESIAN_POINT('Ctrl Pts',(12.1623797632102,127.212499999502,-1.489461944703E-15));
#288803=CARTESIAN_POINT('Ctrl Pts',(12.1623797632102,127.362499999501,-3.95179673813154));
#288804=CARTESIAN_POINT('Ctrl Pts',(9.83957192047899,127.5124999995,-7.14886745759543));
#288805=CARTESIAN_POINT('Ctrl Pts',(7.51676407774777,127.6624999995,-10.3459381770593));
#288806=CARTESIAN_POINT('Ctrl Pts',(3.75838203887384,127.812499999499,-11.5671105274575));
#288807=CARTESIAN_POINT('Ctrl Pts',(-8.69546791285628E-14,127.962499999499,
-12.7882828778556));
#288808=CARTESIAN_POINT('Ctrl Pts',(-3.75838203887402,128.112499999498,
-11.5671105274575));
#288809=CARTESIAN_POINT('Ctrl Pts',(-7.51676407774795,128.262499999497,
-10.3459381770593));
#288810=CARTESIAN_POINT('Ctrl Pts',(-9.83957192047916,128.412499999497,
-7.14886745759543));
#288811=CARTESIAN_POINT('Ctrl Pts',(-12.1623797632104,128.562499999496,
-3.95179673813153));
#288812=CARTESIAN_POINT('Ctrl Pts',(-12.1623797632104,128.712499999496,
2.97892388940601E-15));
#288813=CARTESIAN_POINT('Ctrl Pts',(-12.1623797632104,128.862499999495,
3.95179673813154));
#288814=CARTESIAN_POINT('Ctrl Pts',(-9.83957192047916,129.012499999494,
7.14886745759543));
#288815=CARTESIAN_POINT('Ctrl Pts',(-7.51676407774794,129.162499999494,
10.3459381770593));
#288816=CARTESIAN_POINT('Ctrl Pts',(-3.75838203887401,129.312499999493,
11.5671105274575));
#288817=CARTESIAN_POINT('Ctrl Pts',(-8.46863078258024E-14,129.462499999493,
12.7882828778556));
#288818=CARTESIAN_POINT('Ctrl Pts',(3.75838203887384,129.612499999492,11.5671105274575));
#288819=CARTESIAN_POINT('Ctrl Pts',(7.51676407774777,129.762499999491,10.3459381770593));
#288820=CARTESIAN_POINT('Ctrl Pts',(9.83957192047899,129.912499999491,7.14886745759543));
#288821=CARTESIAN_POINT('Ctrl Pts',(12.1623797632102,130.06249999949,3.95179673813153));
#288822=CARTESIAN_POINT('Ctrl Pts',(12.1623797632102,130.21249999949,-1.489461944703E-15));
#288823=CARTESIAN_POINT('Ctrl Pts',(12.1623797632102,130.362499999489,-3.95179673813154));
#288824=CARTESIAN_POINT('Ctrl Pts',(9.83957192047899,130.512499999488,-7.14886745759543));
#288825=CARTESIAN_POINT('Ctrl Pts',(7.51676407774777,130.662499999488,-10.3459381770593));
#288826=CARTESIAN_POINT('Ctrl Pts',(3.75838203887384,130.812499999487,-11.5671105274575));
#288827=CARTESIAN_POINT('Ctrl Pts',(-8.86823884002247E-14,130.962499999487,
-12.7882828778556));
#288828=CARTESIAN_POINT('Ctrl Pts',(-3.75838203887402,131.112499999486,
-11.5671105274575));
#288829=CARTESIAN_POINT('Ctrl Pts',(-7.51676407774795,131.262499999485,
-10.3459381770593));
#288830=CARTESIAN_POINT('Ctrl Pts',(-9.83957192047916,131.412499999485,
-7.14886745759543));
#288831=CARTESIAN_POINT('Ctrl Pts',(-12.1623797632104,131.562499999484,
-3.95179673813153));
#288832=CARTESIAN_POINT('Ctrl Pts',(-12.1623797632104,131.712499999484,
2.97892388940601E-15));
#288833=CARTESIAN_POINT('Ctrl Pts',(-12.1623797632104,131.862499999483,
3.95179673813154));
#288834=CARTESIAN_POINT('Ctrl Pts',(-9.83957192047916,132.012499999482,
7.14886745759543));
#288835=CARTESIAN_POINT('Ctrl Pts',(-7.51676407774795,132.162499999482,
10.3459381770593));
#288836=CARTESIAN_POINT('Ctrl Pts',(-3.75838203887402,132.312499999481,
11.5671105274575));
#288837=CARTESIAN_POINT('Ctrl Pts',(-8.64140170974642E-14,132.462499999481,
12.7882828778556));
#288838=CARTESIAN_POINT('Ctrl Pts',(3.75838203887384,132.61249999948,11.5671105274575));
#288839=CARTESIAN_POINT('Ctrl Pts',(7.51676407774777,132.762499999479,10.3459381770593));
#288840=CARTESIAN_POINT('Ctrl Pts',(9.83957192047899,132.912499999479,7.14886745759543));
#288841=CARTESIAN_POINT('Ctrl Pts',(12.1623797632102,133.062499999478,3.95179673813153));
#288842=CARTESIAN_POINT('Ctrl Pts',(12.1623797632102,133.212499999478,-1.489461944703E-15));
#288843=CARTESIAN_POINT('Ctrl Pts',(12.1623797632102,133.362499999477,-3.95179673813154));
#288844=CARTESIAN_POINT('Ctrl Pts',(9.83957192047898,133.512499999476,-7.14886745759543));
#288845=CARTESIAN_POINT('Ctrl Pts',(7.51676407774777,133.662499999476,-10.3459381770593));
#288846=CARTESIAN_POINT('Ctrl Pts',(3.75838203887384,133.812499999475,-11.5671105274575));
#288847=CARTESIAN_POINT('Ctrl Pts',(-9.04100976718865E-14,133.962499999475,
-12.7882828778556));
#288848=CARTESIAN_POINT('Ctrl Pts',(-3.75838203887402,134.112499999474,
-11.5671105274575));
#288849=CARTESIAN_POINT('Ctrl Pts',(-7.51676407774795,134.262499999473,
-10.3459381770593));
#288850=CARTESIAN_POINT('Ctrl Pts',(-9.83957192047917,134.412499999473,
-7.14886745759543));
#288851=CARTESIAN_POINT('Ctrl Pts',(-12.1623797632104,134.562499999472,
-3.95179673813153));
#288852=CARTESIAN_POINT('Ctrl Pts',(-12.1623797632104,134.712499999472,
2.97892388940601E-15));
#288853=CARTESIAN_POINT('Ctrl Pts',(-12.1623797632104,134.862499999471,
3.95179673813154));
#288854=CARTESIAN_POINT('Ctrl Pts',(-9.83957192047916,135.01249999947,7.14886745759543));
#288855=CARTESIAN_POINT('Ctrl Pts',(-7.51676407774795,135.16249999947,10.3459381770593));
#288856=CARTESIAN_POINT('Ctrl Pts',(-3.75838203887402,135.312499999469,
11.5671105274575));
#288857=CARTESIAN_POINT('Ctrl Pts',(-8.8141726369126E-14,135.462499999469,
12.7882828778556));
#288858=CARTESIAN_POINT('Ctrl Pts',(3.75838203887384,135.612499999468,11.5671105274575));
#288859=CARTESIAN_POINT('Ctrl Pts',(7.51676407774777,135.762499999467,10.3459381770593));
#288860=CARTESIAN_POINT('Ctrl Pts',(9.83957192047898,135.912499999467,7.14886745759543));
#288861=CARTESIAN_POINT('Ctrl Pts',(12.1623797632102,136.062499999466,3.95179673813153));
#288862=CARTESIAN_POINT('Ctrl Pts',(12.1623797632102,136.212499999466,-1.489461944703E-15));
#288863=CARTESIAN_POINT('Ctrl Pts',(12.1623797632102,136.362499999465,-3.95179673813154));
#288864=CARTESIAN_POINT('Ctrl Pts',(9.83957192047898,136.512499999464,-7.14886745759543));
#288865=CARTESIAN_POINT('Ctrl Pts',(7.51676407774777,136.662499999464,-10.3459381770593));
#288866=CARTESIAN_POINT('Ctrl Pts',(3.75838203887384,136.812499999463,-11.5671105274575));
#288867=CARTESIAN_POINT('Ctrl Pts',(-9.21378069435483E-14,136.962499999463,
-12.7882828778556));
#288868=CARTESIAN_POINT('Ctrl Pts',(-3.75838203887402,137.112499999462,
-11.5671105274575));
#288869=CARTESIAN_POINT('Ctrl Pts',(-7.51676407774795,137.262499999461,
-10.3459381770593));
#288870=CARTESIAN_POINT('Ctrl Pts',(-9.83957192047917,137.412499999461,
-7.14886745759543));
#288871=CARTESIAN_POINT('Ctrl Pts',(-12.1623797632104,137.56249999946,-3.95179673813153));
#288872=CARTESIAN_POINT('Ctrl Pts',(-12.1623797632104,137.71249999946,2.97892388940601E-15));
#288873=CARTESIAN_POINT('Ctrl Pts',(-12.1623797632104,137.862499999459,
3.95179673813154));
#288874=CARTESIAN_POINT('Ctrl Pts',(-9.83957192047917,138.012499999458,
7.14886745759543));
#288875=CARTESIAN_POINT('Ctrl Pts',(-7.51676407774795,138.162499999458,
10.3459381770593));
#288876=CARTESIAN_POINT('Ctrl Pts',(-3.75838203887402,138.312499999457,
11.5671105274575));
#288877=CARTESIAN_POINT('Ctrl Pts',(-8.98694356407879E-14,138.462499999457,
12.7882828778556));
#288878=CARTESIAN_POINT('Ctrl Pts',(3.75838203887384,138.612499999456,11.5671105274575));
#288879=CARTESIAN_POINT('Ctrl Pts',(7.51676407774777,138.762499999455,10.3459381770593));
#288880=CARTESIAN_POINT('Ctrl Pts',(9.83957192047898,138.912499999455,7.14886745759543));
#288881=CARTESIAN_POINT('Ctrl Pts',(12.1623797632102,139.062499999454,3.95179673813153));
#288882=CARTESIAN_POINT('Ctrl Pts',(12.1623797632102,139.212499999454,-1.489461944703E-15));
#288883=CARTESIAN_POINT('Ctrl Pts',(12.1623797632102,139.362499999453,-3.95179673813154));
#288884=CARTESIAN_POINT('Ctrl Pts',(9.83957192047898,139.512499999452,-7.14886745759543));
#288885=CARTESIAN_POINT('Ctrl Pts',(7.51676407774776,139.662499999452,-10.3459381770593));
#288886=CARTESIAN_POINT('Ctrl Pts',(3.75838203887384,139.812499999451,-11.5671105274575));
#288887=CARTESIAN_POINT('Ctrl Pts',(-9.38655162152102E-14,139.962499999451,
-12.7882828778556));
#288888=CARTESIAN_POINT('Ctrl Pts',(-3.75838203887402,140.11249999945,-11.5671105274575));
#288889=CARTESIAN_POINT('Ctrl Pts',(-7.51676407774795,140.262499999449,
-10.3459381770593));
#288890=CARTESIAN_POINT('Ctrl Pts',(-9.83957192047917,140.412499999449,
-7.14886745759543));
#288891=CARTESIAN_POINT('Ctrl Pts',(-12.1623797632104,140.562499999448,
-3.95179673813153));
#288892=CARTESIAN_POINT('Ctrl Pts',(-12.1623797632104,140.712499999448,
2.97892388940601E-15));
#288893=CARTESIAN_POINT('Ctrl Pts',(-12.1623797632104,140.862499999447,
3.95179673813154));
#288894=CARTESIAN_POINT('Ctrl Pts',(-9.83957192047917,141.012499999446,
7.14886745759543));
#288895=CARTESIAN_POINT('Ctrl Pts',(-7.51676407774795,141.162499999446,
10.3459381770593));
#288896=CARTESIAN_POINT('Ctrl Pts',(-3.75838203887402,141.312499999445,
11.5671105274575));
#288897=CARTESIAN_POINT('Ctrl Pts',(-9.15971449124498E-14,141.462499999445,
12.7882828778556));
#288898=CARTESIAN_POINT('Ctrl Pts',(3.75838203887384,141.612499999444,11.5671105274575));
#288899=CARTESIAN_POINT('Ctrl Pts',(7.51676407774777,141.762499999443,10.3459381770593));
#288900=CARTESIAN_POINT('Ctrl Pts',(9.83957192047898,141.912499999443,7.14886745759543));
#288901=CARTESIAN_POINT('Ctrl Pts',(12.1623797632102,142.062499999442,3.95179673813153));
#288902=CARTESIAN_POINT('Ctrl Pts',(12.1623797632102,142.212499999442,-1.489461944703E-15));
#288903=CARTESIAN_POINT('Ctrl Pts',(12.1623797632102,142.362499999441,-3.95179673813154));
#288904=CARTESIAN_POINT('Ctrl Pts',(9.83957192047898,142.51249999944,-7.14886745759543));
#288905=CARTESIAN_POINT('Ctrl Pts',(7.51676407774776,142.66249999944,-10.3459381770593));
#288906=CARTESIAN_POINT('Ctrl Pts',(3.75838203887383,142.812499999439,-11.5671105274575));
#288907=CARTESIAN_POINT('Ctrl Pts',(-9.5593225486872E-14,142.962499999439,
-12.7882828778556));
#288908=CARTESIAN_POINT('Ctrl Pts',(-3.75838203887402,143.112499999438,
-11.5671105274575));
#288909=CARTESIAN_POINT('Ctrl Pts',(-7.51676407774795,143.262499999437,
-10.3459381770593));
#288910=CARTESIAN_POINT('Ctrl Pts',(-9.83957192047917,143.412499999437,
-7.14886745759543));
#288911=CARTESIAN_POINT('Ctrl Pts',(-12.1623797632104,143.562499999436,
-3.95179673813153));
#288912=CARTESIAN_POINT('Ctrl Pts',(-12.1623797632104,143.712499999436,
2.97892388940601E-15));
#288913=CARTESIAN_POINT('Ctrl Pts',(-12.1623797632104,143.862499999435,
3.95179673813154));
#288914=CARTESIAN_POINT('Ctrl Pts',(-9.83957192047917,144.012499999434,
7.14886745759543));
#288915=CARTESIAN_POINT('Ctrl Pts',(-7.51676407774795,144.162499999434,
10.3459381770593));
#288916=CARTESIAN_POINT('Ctrl Pts',(-3.75838203887402,144.312499999433,
11.5671105274575));
#288917=CARTESIAN_POINT('Ctrl Pts',(-9.33248541841116E-14,144.462499999433,
12.7882828778556));
#288918=CARTESIAN_POINT('Ctrl Pts',(3.75838203887384,144.612499999432,11.5671105274575));
#288919=CARTESIAN_POINT('Ctrl Pts',(7.51676407774776,144.762499999431,10.3459381770593));
#288920=CARTESIAN_POINT('Ctrl Pts',(9.83957192047898,144.912499999431,7.14886745759543));
#288921=CARTESIAN_POINT('Ctrl Pts',(12.1623797632102,145.06249999943,3.95179673813153));
#288922=CARTESIAN_POINT('Ctrl Pts',(12.1623797632102,145.21249999943,-1.489461944703E-15));
#288923=CARTESIAN_POINT('Ctrl Pts',(12.1623797632102,145.362499999429,-3.95179673813154));
#288924=CARTESIAN_POINT('Ctrl Pts',(9.83957192047898,145.512499999428,-7.14886745759543));
#288925=CARTESIAN_POINT('Ctrl Pts',(7.51676407774776,145.662499999428,-10.3459381770593));
#288926=CARTESIAN_POINT('Ctrl Pts',(3.75838203887383,145.812499999427,-11.5671105274575));
#288927=CARTESIAN_POINT('Ctrl Pts',(-9.73209347585338E-14,145.962499999427,
-12.7882828778556));
#288928=CARTESIAN_POINT('Ctrl Pts',(-3.75838203887403,146.112499999426,
-11.5671105274575));
#288929=CARTESIAN_POINT('Ctrl Pts',(-7.51676407774795,146.262499999425,
-10.3459381770593));
#288930=CARTESIAN_POINT('Ctrl Pts',(-9.83957192047917,146.412499999425,
-7.14886745759543));
#288931=CARTESIAN_POINT('Ctrl Pts',(-12.1623797632104,146.562499999424,
-3.95179673813153));
#288932=CARTESIAN_POINT('Ctrl Pts',(-12.1623797632104,146.712499999424,
2.97892388940601E-15));
#288933=CARTESIAN_POINT('Ctrl Pts',(-12.1623797632104,146.862499999423,
3.95179673813154));
#288934=CARTESIAN_POINT('Ctrl Pts',(-9.83957192047917,147.012499999422,
7.14886745759543));
#288935=CARTESIAN_POINT('Ctrl Pts',(-7.51676407774795,147.162499999422,
10.3459381770593));
#288936=CARTESIAN_POINT('Ctrl Pts',(-3.75838203887402,147.312499999421,
11.5671105274575));
#288937=CARTESIAN_POINT('Ctrl Pts',(-9.50525634557734E-14,147.462499999421,
12.7882828778556));
#288938=CARTESIAN_POINT('Ctrl Pts',(3.75838203887383,147.61249999942,11.5671105274575));
#288939=CARTESIAN_POINT('Ctrl Pts',(7.51676407774776,147.762499999419,10.3459381770593));
#288940=CARTESIAN_POINT('Ctrl Pts',(9.83957192047898,147.912499999419,7.14886745759543));
#288941=CARTESIAN_POINT('Ctrl Pts',(12.1623797632102,148.062499999418,3.95179673813153));
#288942=CARTESIAN_POINT('Ctrl Pts',(12.1623797632102,148.212499999418,-1.489461944703E-15));
#288943=CARTESIAN_POINT('Ctrl Pts',(12.1623797632102,148.362499999417,-3.95179673813154));
#288944=CARTESIAN_POINT('Ctrl Pts',(9.83957192047898,148.512499999416,-7.14886745759543));
#288945=CARTESIAN_POINT('Ctrl Pts',(7.51676407774776,148.662499999416,-10.3459381770593));
#288946=CARTESIAN_POINT('Ctrl Pts',(3.75838203887383,148.812499999415,-11.5671105274575));
#288947=CARTESIAN_POINT('Ctrl Pts',(-9.90486440301957E-14,148.962499999415,
-12.7882828778556));
#288948=CARTESIAN_POINT('Ctrl Pts',(-3.75838203887403,149.112499999414,
-11.5671105274575));
#288949=CARTESIAN_POINT('Ctrl Pts',(-7.51676407774795,149.262499999413,
-10.3459381770593));
#288950=CARTESIAN_POINT('Ctrl Pts',(-9.83957192047917,149.412499999413,
-7.14886745759543));
#288951=CARTESIAN_POINT('Ctrl Pts',(-12.1623797632104,149.562499999412,
-3.95179673813153));
#288952=CARTESIAN_POINT('Ctrl Pts',(-12.1623797632104,149.712499999412,
2.97892388940601E-15));
#288953=CARTESIAN_POINT('Ctrl Pts',(-12.1623797632104,149.862499999411,
3.95179673813154));
#288954=CARTESIAN_POINT('Ctrl Pts',(-9.83957192047917,150.01249999941,7.14886745759543));
#288955=CARTESIAN_POINT('Ctrl Pts',(-7.51676407774795,150.16249999941,10.3459381770593));
#288956=CARTESIAN_POINT('Ctrl Pts',(-3.75838203887403,150.312499999409,
11.5671105274575));
#288957=CARTESIAN_POINT('Ctrl Pts',(-9.67802727274353E-14,150.462499999409,
12.7882828778556));
#288958=CARTESIAN_POINT('Ctrl Pts',(3.75838203887383,150.612499999408,11.5671105274575));
#288959=CARTESIAN_POINT('Ctrl Pts',(7.51676407774776,150.762499999407,10.3459381770593));
#288960=CARTESIAN_POINT('Ctrl Pts',(9.83957192047898,150.912499999407,7.14886745759543));
#288961=CARTESIAN_POINT('Ctrl Pts',(12.1623797632102,151.062499999406,3.95179673813153));
#288962=CARTESIAN_POINT('Ctrl Pts',(12.1623797632102,151.212499999406,-1.489461944703E-15));
#288963=CARTESIAN_POINT('Ctrl Pts',(12.1623797632102,151.362499999405,-3.95179673813154));
#288964=CARTESIAN_POINT('Ctrl Pts',(9.83957192047897,151.512499999404,-7.14886745759543));
#288965=CARTESIAN_POINT('Ctrl Pts',(7.51676407774776,151.662499999404,-10.3459381770593));
#288966=CARTESIAN_POINT('Ctrl Pts',(3.75838203887383,151.812499999403,-11.5671105274575));
#288967=CARTESIAN_POINT('Ctrl Pts',(-1.00776353301858E-13,151.962499999403,
-12.7882828778556));
#288968=CARTESIAN_POINT('Ctrl Pts',(-3.75838203887403,152.112499999402,
-11.5671105274575));
#288969=CARTESIAN_POINT('Ctrl Pts',(-10.0514428414942,-2.06874999998125,
2.46189346052968E-15));
#288970=CARTESIAN_POINT('Ctrl Pts',(-10.0514428414942,-1.91874999998185,
3.26591175476071));
#288971=CARTESIAN_POINT('Ctrl Pts',(-8.1317880767572,-1.76874999998245,
5.90808986649102));
#288972=CARTESIAN_POINT('Ctrl Pts',(-6.21213331202023,-1.61874999998305,
8.55026797822134));
#288973=CARTESIAN_POINT('Ctrl Pts',(-3.10606665601012,-1.46874999998365,
9.5594902125713));
#288974=CARTESIAN_POINT('Ctrl Pts',(-9.77671023785295E-15,-1.31874999998425,
10.5687124469213));
#288975=CARTESIAN_POINT('Ctrl Pts',(3.1060666560101,-1.16874999998485,9.5594902125713));
#288976=CARTESIAN_POINT('Ctrl Pts',(6.21213331202021,-1.01874999998544,
8.55026797822134));
#288977=CARTESIAN_POINT('Ctrl Pts',(8.13178807675718,-0.868749999986043,
5.90808986649102));
#288978=CARTESIAN_POINT('Ctrl Pts',(10.0514428414942,-0.718749999986641,
3.2659117547607));
#288979=CARTESIAN_POINT('Ctrl Pts',(10.0514428414942,-0.568749999987242,
-1.23094673026484E-15));
#288980=CARTESIAN_POINT('Ctrl Pts',(10.0514428414942,-0.418749999987842,
-3.26591175476071));
#288981=CARTESIAN_POINT('Ctrl Pts',(8.13178807675718,-0.268749999988443,
-5.90808986649102));
#288982=CARTESIAN_POINT('Ctrl Pts',(6.2121333120202,-0.118749999989044,
-8.55026797822134));
#288983=CARTESIAN_POINT('Ctrl Pts',(3.10606665601009,0.0312500000103543,
-9.5594902125713));
#288984=CARTESIAN_POINT('Ctrl Pts',(-1.322915284753E-14,0.181250000009752,
-10.5687124469213));
#288985=CARTESIAN_POINT('Ctrl Pts',(-3.10606665601012,0.331250000009151,
-9.5594902125713));
#288986=CARTESIAN_POINT('Ctrl Pts',(-6.21213331202023,0.481250000008549,
-8.55026797822134));
#288987=CARTESIAN_POINT('Ctrl Pts',(-8.1317880767572,0.631250000007948,
-5.90808986649102));
#288988=CARTESIAN_POINT('Ctrl Pts',(-10.0514428414942,0.781250000007346,
-3.2659117547607));
#288989=CARTESIAN_POINT('Ctrl Pts',(-10.0514428414942,0.931250000006746,
2.46189346052968E-15));
#288990=CARTESIAN_POINT('Ctrl Pts',(-10.0514428414942,1.08125000000615,
3.26591175476071));
#288991=CARTESIAN_POINT('Ctrl Pts',(-8.1317880767572,1.23125000000555,5.90808986649102));
#288992=CARTESIAN_POINT('Ctrl Pts',(-6.21213331202023,1.38125000000495,
8.55026797822134));
#288993=CARTESIAN_POINT('Ctrl Pts',(-3.10606665601012,1.53125000000435,
9.5594902125713));
#288994=CARTESIAN_POINT('Ctrl Pts',(-1.15044195095148E-14,1.68125000000375,
10.5687124469213));
#288995=CARTESIAN_POINT('Ctrl Pts',(3.1060666560101,1.83125000000315,9.5594902125713));
#288996=CARTESIAN_POINT('Ctrl Pts',(6.2121333120202,1.98125000000256,8.55026797822134));
#288997=CARTESIAN_POINT('Ctrl Pts',(8.13178807675718,2.13125000000196,5.90808986649102));
#288998=CARTESIAN_POINT('Ctrl Pts',(10.0514428414942,2.28125000000136,3.2659117547607));
#288999=CARTESIAN_POINT('Ctrl Pts',(10.0514428414942,2.43125000000076,-1.23094673026484E-15));
#289000=CARTESIAN_POINT('Ctrl Pts',(10.0514428414942,2.58125000000016,-3.26591175476071));
#289001=CARTESIAN_POINT('Ctrl Pts',(8.13178807675718,2.73124999999956,-5.90808986649102));
#289002=CARTESIAN_POINT('Ctrl Pts',(6.2121333120202,2.88124999999896,-8.55026797822134));
#289003=CARTESIAN_POINT('Ctrl Pts',(3.10606665601009,3.03124999999835,-9.5594902125713));
#289004=CARTESIAN_POINT('Ctrl Pts',(-1.49568621191919E-14,3.18124999999775,
-10.5687124469213));
#289005=CARTESIAN_POINT('Ctrl Pts',(-3.10606665601012,3.33124999999715,
-9.5594902125713));
#289006=CARTESIAN_POINT('Ctrl Pts',(-6.21213331202023,3.48124999999655,
-8.55026797822134));
#289007=CARTESIAN_POINT('Ctrl Pts',(-8.13178807675721,3.63124999999595,
-5.90808986649102));
#289008=CARTESIAN_POINT('Ctrl Pts',(-10.0514428414942,3.78124999999535,
-3.2659117547607));
#289009=CARTESIAN_POINT('Ctrl Pts',(-10.0514428414942,3.93124999999475,
2.46189346052968E-15));
#289010=CARTESIAN_POINT('Ctrl Pts',(-10.0514428414942,4.08124999999415,
3.26591175476071));
#289011=CARTESIAN_POINT('Ctrl Pts',(-8.13178807675721,4.23124999999355,
5.90808986649102));
#289012=CARTESIAN_POINT('Ctrl Pts',(-6.21213331202023,4.38124999999295,
8.55026797822134));
#289013=CARTESIAN_POINT('Ctrl Pts',(-3.10606665601012,4.53124999999235,
9.5594902125713));
#289014=CARTESIAN_POINT('Ctrl Pts',(-1.32321287811766E-14,4.68124999999175,
10.5687124469213));
#289015=CARTESIAN_POINT('Ctrl Pts',(3.10606665601009,4.83124999999115,9.5594902125713));
#289016=CARTESIAN_POINT('Ctrl Pts',(6.2121333120202,4.98124999999055,8.55026797822134));
#289017=CARTESIAN_POINT('Ctrl Pts',(8.13178807675718,5.13124999998996,5.90808986649102));
#289018=CARTESIAN_POINT('Ctrl Pts',(10.0514428414942,5.28124999998936,3.2659117547607));
#289019=CARTESIAN_POINT('Ctrl Pts',(10.0514428414941,5.43124999998876,-1.23094673026484E-15));
#289020=CARTESIAN_POINT('Ctrl Pts',(10.0514428414941,5.58124999998816,-3.26591175476071));
#289021=CARTESIAN_POINT('Ctrl Pts',(8.13178807675717,5.73124999998756,-5.90808986649102));
#289022=CARTESIAN_POINT('Ctrl Pts',(6.2121333120202,5.88124999998695,-8.55026797822134));
#289023=CARTESIAN_POINT('Ctrl Pts',(3.10606665601009,6.03124999998635,-9.5594902125713));
#289024=CARTESIAN_POINT('Ctrl Pts',(-1.66845713908537E-14,6.18124999998575,
-10.5687124469213));
#289025=CARTESIAN_POINT('Ctrl Pts',(-3.10606665601012,6.33124999998515,
-9.5594902125713));
#289026=CARTESIAN_POINT('Ctrl Pts',(-6.21213331202023,6.48124999998455,
-8.55026797822134));
#289027=CARTESIAN_POINT('Ctrl Pts',(-8.13178807675721,6.63124999998395,
-5.90808986649102));
#289028=CARTESIAN_POINT('Ctrl Pts',(-10.0514428414942,6.78124999998335,
-3.2659117547607));
#289029=CARTESIAN_POINT('Ctrl Pts',(-10.0514428414942,6.93124999998275,
2.46189346052968E-15));
#289030=CARTESIAN_POINT('Ctrl Pts',(-10.0514428414942,7.08124999998215,
3.26591175476071));
#289031=CARTESIAN_POINT('Ctrl Pts',(-8.13178807675721,7.23124999998155,
5.90808986649102));
#289032=CARTESIAN_POINT('Ctrl Pts',(-6.21213331202023,7.38124999998095,
8.55026797822134));
#289033=CARTESIAN_POINT('Ctrl Pts',(-3.10606665601012,7.53124999998035,
9.5594902125713));
#289034=CARTESIAN_POINT('Ctrl Pts',(-1.49598380528385E-14,7.68124999997975,
10.5687124469213));
#289035=CARTESIAN_POINT('Ctrl Pts',(3.10606665601009,7.83124999997915,9.5594902125713));
#289036=CARTESIAN_POINT('Ctrl Pts',(6.2121333120202,7.98124999997856,8.55026797822134));
#289037=CARTESIAN_POINT('Ctrl Pts',(8.13178807675717,8.13124999997796,5.90808986649102));
#289038=CARTESIAN_POINT('Ctrl Pts',(10.0514428414942,8.28124999997736,3.2659117547607));
#289039=CARTESIAN_POINT('Ctrl Pts',(10.0514428414941,8.43124999997676,-1.23094673026484E-15));
#289040=CARTESIAN_POINT('Ctrl Pts',(10.0514428414941,8.58124999997616,-3.26591175476071));
#289041=CARTESIAN_POINT('Ctrl Pts',(8.13178807675717,8.73124999997556,-5.90808986649102));
#289042=CARTESIAN_POINT('Ctrl Pts',(6.2121333120202,8.88124999997496,-8.55026797822134));
#289043=CARTESIAN_POINT('Ctrl Pts',(3.10606665601009,9.03124999997436,-9.5594902125713));
#289044=CARTESIAN_POINT('Ctrl Pts',(-1.84122806625156E-14,9.18124999997375,
-10.5687124469213));
#289045=CARTESIAN_POINT('Ctrl Pts',(-3.10606665601013,9.33124999997315,
-9.5594902125713));
#289046=CARTESIAN_POINT('Ctrl Pts',(-6.21213331202023,9.48124999997255,
-8.55026797822134));
#289047=CARTESIAN_POINT('Ctrl Pts',(-8.13178807675721,9.63124999997195,
-5.90808986649102));
#289048=CARTESIAN_POINT('Ctrl Pts',(-10.0514428414942,9.78124999997135,
-3.2659117547607));
#289049=CARTESIAN_POINT('Ctrl Pts',(-10.0514428414942,9.93124999997075,
2.46189346052968E-15));
#289050=CARTESIAN_POINT('Ctrl Pts',(-10.0514428414942,10.0812499999701,
3.26591175476071));
#289051=CARTESIAN_POINT('Ctrl Pts',(-8.13178807675721,10.2312499999695,
5.90808986649102));
#289052=CARTESIAN_POINT('Ctrl Pts',(-6.21213331202023,10.3812499999689,
8.55026797822134));
#289053=CARTESIAN_POINT('Ctrl Pts',(-3.10606665601012,10.5312499999684,
9.5594902125713));
#289054=CARTESIAN_POINT('Ctrl Pts',(-1.66875473245003E-14,10.6812499999678,
10.5687124469213));
#289055=CARTESIAN_POINT('Ctrl Pts',(3.10606665601009,10.8312499999672,9.5594902125713));
#289056=CARTESIAN_POINT('Ctrl Pts',(6.2121333120202,10.9812499999666,8.55026797822134));
#289057=CARTESIAN_POINT('Ctrl Pts',(8.13178807675717,11.131249999966,5.90808986649102));
#289058=CARTESIAN_POINT('Ctrl Pts',(10.0514428414941,11.2812499999654,3.2659117547607));
#289059=CARTESIAN_POINT('Ctrl Pts',(10.0514428414941,11.4312499999648,-1.23094673026484E-15));
#289060=CARTESIAN_POINT('Ctrl Pts',(10.0514428414941,11.5812499999642,-3.26591175476071));
#289061=CARTESIAN_POINT('Ctrl Pts',(8.13178807675717,11.7312499999636,-5.90808986649102));
#289062=CARTESIAN_POINT('Ctrl Pts',(6.2121333120202,11.881249999963,-8.55026797822134));
#289063=CARTESIAN_POINT('Ctrl Pts',(3.10606665601009,12.0312499999624,-9.5594902125713));
#289064=CARTESIAN_POINT('Ctrl Pts',(-2.01399899341774E-14,12.1812499999618,
-10.5687124469213));
#289065=CARTESIAN_POINT('Ctrl Pts',(-3.10606665601013,12.3312499999612,
-9.5594902125713));
#289066=CARTESIAN_POINT('Ctrl Pts',(-6.21213331202024,12.4812499999605,
-8.55026797822134));
#289067=CARTESIAN_POINT('Ctrl Pts',(-8.13178807675721,12.6312499999599,
-5.90808986649102));
#289068=CARTESIAN_POINT('Ctrl Pts',(-10.0514428414942,12.7812499999593,
-3.2659117547607));
#289069=CARTESIAN_POINT('Ctrl Pts',(-10.0514428414942,12.9312499999587,
2.46189346052968E-15));
#289070=CARTESIAN_POINT('Ctrl Pts',(-10.0514428414942,13.0812499999581,
3.26591175476071));
#289071=CARTESIAN_POINT('Ctrl Pts',(-8.13178807675721,13.2312499999575,
5.90808986649102));
#289072=CARTESIAN_POINT('Ctrl Pts',(-6.21213331202023,13.3812499999569,
8.55026797822134));
#289073=CARTESIAN_POINT('Ctrl Pts',(-3.10606665601013,13.5312499999564,
9.5594902125713));
#289074=CARTESIAN_POINT('Ctrl Pts',(-1.84152565961621E-14,13.6812499999558,
10.5687124469213));
#289075=CARTESIAN_POINT('Ctrl Pts',(3.10606665601009,13.8312499999552,9.5594902125713));
#289076=CARTESIAN_POINT('Ctrl Pts',(6.2121333120202,13.9812499999546,8.55026797822134));
#289077=CARTESIAN_POINT('Ctrl Pts',(8.13178807675717,14.131249999954,5.90808986649102));
#289078=CARTESIAN_POINT('Ctrl Pts',(10.0514428414941,14.2812499999534,3.2659117547607));
#289079=CARTESIAN_POINT('Ctrl Pts',(10.0514428414941,14.4312499999528,-1.23094673026484E-15));
#289080=CARTESIAN_POINT('Ctrl Pts',(10.0514428414941,14.5812499999522,-3.26591175476071));
#289081=CARTESIAN_POINT('Ctrl Pts',(8.13178807675717,14.7312499999516,-5.90808986649102));
#289082=CARTESIAN_POINT('Ctrl Pts',(6.21213331202019,14.881249999951,-8.55026797822134));
#289083=CARTESIAN_POINT('Ctrl Pts',(3.10606665601009,15.0312499999504,-9.5594902125713));
#289084=CARTESIAN_POINT('Ctrl Pts',(-2.18676992058392E-14,15.1812499999498,
-10.5687124469213));
#289085=CARTESIAN_POINT('Ctrl Pts',(-3.10606665601013,15.3312499999492,
-9.5594902125713));
#289086=CARTESIAN_POINT('Ctrl Pts',(-6.21213331202024,15.4812499999485,
-8.55026797822134));
#289087=CARTESIAN_POINT('Ctrl Pts',(-8.13178807675721,15.6312499999479,
-5.90808986649102));
#289088=CARTESIAN_POINT('Ctrl Pts',(-10.0514428414942,15.7812499999473,
-3.2659117547607));
#289089=CARTESIAN_POINT('Ctrl Pts',(-10.0514428414942,15.9312499999467,
2.46189346052968E-15));
#289090=CARTESIAN_POINT('Ctrl Pts',(-10.0514428414942,16.0812499999461,
3.26591175476071));
#289091=CARTESIAN_POINT('Ctrl Pts',(-8.13178807675721,16.2312499999455,
5.90808986649102));
#289092=CARTESIAN_POINT('Ctrl Pts',(-6.21213331202024,16.3812499999449,
8.55026797822134));
#289093=CARTESIAN_POINT('Ctrl Pts',(-3.10606665601013,16.5312499999444,
9.5594902125713));
#289094=CARTESIAN_POINT('Ctrl Pts',(-2.0142965867824E-14,16.6812499999438,
10.5687124469213));
#289095=CARTESIAN_POINT('Ctrl Pts',(3.10606665601009,16.8312499999432,9.5594902125713));
#289096=CARTESIAN_POINT('Ctrl Pts',(6.21213331202019,16.9812499999426,8.55026797822134));
#289097=CARTESIAN_POINT('Ctrl Pts',(8.13178807675717,17.131249999942,5.90808986649102));
#289098=CARTESIAN_POINT('Ctrl Pts',(10.0514428414941,17.2812499999414,3.2659117547607));
#289099=CARTESIAN_POINT('Ctrl Pts',(10.0514428414941,17.4312499999408,-1.23094673026484E-15));
#289100=CARTESIAN_POINT('Ctrl Pts',(10.0514428414941,17.5812499999402,-3.26591175476071));
#289101=CARTESIAN_POINT('Ctrl Pts',(8.13178807675717,17.7312499999396,-5.90808986649102));
#289102=CARTESIAN_POINT('Ctrl Pts',(6.21213331202019,17.881249999939,-8.55026797822134));
#289103=CARTESIAN_POINT('Ctrl Pts',(3.10606665601008,18.0312499999384,-9.5594902125713));
#289104=CARTESIAN_POINT('Ctrl Pts',(-2.35954084775011E-14,18.1812499999378,
-10.5687124469213));
#289105=CARTESIAN_POINT('Ctrl Pts',(-3.10606665601013,18.3312499999371,
-9.5594902125713));
#289106=CARTESIAN_POINT('Ctrl Pts',(-6.21213331202024,18.4812499999365,
-8.55026797822134));
#289107=CARTESIAN_POINT('Ctrl Pts',(-8.13178807675721,18.6312499999359,
-5.90808986649102));
#289108=CARTESIAN_POINT('Ctrl Pts',(-10.0514428414942,18.7812499999353,
-3.2659117547607));
#289109=CARTESIAN_POINT('Ctrl Pts',(-10.0514428414942,18.9312499999347,
2.46189346052968E-15));
#289110=CARTESIAN_POINT('Ctrl Pts',(-10.0514428414942,19.0812499999341,
3.26591175476071));
#289111=CARTESIAN_POINT('Ctrl Pts',(-8.13178807675721,19.2312499999335,
5.90808986649102));
#289112=CARTESIAN_POINT('Ctrl Pts',(-6.21213331202024,19.381249999933,8.55026797822134));
#289113=CARTESIAN_POINT('Ctrl Pts',(-3.10606665601013,19.5312499999323,
9.5594902125713));
#289114=CARTESIAN_POINT('Ctrl Pts',(-2.18706751394858E-14,19.6812499999318,
10.5687124469213));
#289115=CARTESIAN_POINT('Ctrl Pts',(3.10606665601009,19.8312499999312,9.5594902125713));
#289116=CARTESIAN_POINT('Ctrl Pts',(6.21213331202019,19.9812499999306,8.55026797822134));
#289117=CARTESIAN_POINT('Ctrl Pts',(8.13178807675717,20.13124999993,5.90808986649102));
#289118=CARTESIAN_POINT('Ctrl Pts',(10.0514428414941,20.2812499999294,3.2659117547607));
#289119=CARTESIAN_POINT('Ctrl Pts',(10.0514428414941,20.4312499999288,-1.23094673026484E-15));
#289120=CARTESIAN_POINT('Ctrl Pts',(10.0514428414941,20.5812499999282,-3.26591175476071));
#289121=CARTESIAN_POINT('Ctrl Pts',(8.13178807675716,20.7312499999276,-5.90808986649102));
#289122=CARTESIAN_POINT('Ctrl Pts',(6.21213331202019,20.881249999927,-8.55026797822134));
#289123=CARTESIAN_POINT('Ctrl Pts',(3.10606665601008,21.0312499999264,-9.5594902125713));
#289124=CARTESIAN_POINT('Ctrl Pts',(-2.53231177491629E-14,21.1812499999258,
-10.5687124469213));
#289125=CARTESIAN_POINT('Ctrl Pts',(-3.10606665601013,21.3312499999251,
-9.5594902125713));
#289126=CARTESIAN_POINT('Ctrl Pts',(-6.21213331202024,21.4812499999245,
-8.55026797822134));
#289127=CARTESIAN_POINT('Ctrl Pts',(-8.13178807675722,21.6312499999239,
-5.90808986649102));
#289128=CARTESIAN_POINT('Ctrl Pts',(-10.0514428414942,21.7812499999233,
-3.2659117547607));
#289129=CARTESIAN_POINT('Ctrl Pts',(-10.0514428414942,21.9312499999227,
2.46189346052968E-15));
#289130=CARTESIAN_POINT('Ctrl Pts',(-10.0514428414942,22.0812499999221,
3.26591175476071));
#289131=CARTESIAN_POINT('Ctrl Pts',(-8.13178807675722,22.2312499999215,
5.90808986649102));
#289132=CARTESIAN_POINT('Ctrl Pts',(-6.21213331202024,22.3812499999209,
8.55026797822134));
#289133=CARTESIAN_POINT('Ctrl Pts',(-3.10606665601013,22.5312499999204,
9.5594902125713));
#289134=CARTESIAN_POINT('Ctrl Pts',(-2.35983844111477E-14,22.6812499999198,
10.5687124469213));
#289135=CARTESIAN_POINT('Ctrl Pts',(3.10606665601008,22.8312499999192,9.5594902125713));
#289136=CARTESIAN_POINT('Ctrl Pts',(6.21213331202019,22.9812499999186,8.55026797822134));
#289137=CARTESIAN_POINT('Ctrl Pts',(8.13178807675716,23.131249999918,5.90808986649102));
#289138=CARTESIAN_POINT('Ctrl Pts',(10.0514428414941,23.2812499999174,3.2659117547607));
#289139=CARTESIAN_POINT('Ctrl Pts',(10.0514428414941,23.4312499999168,-1.23094673026484E-15));
#289140=CARTESIAN_POINT('Ctrl Pts',(10.0514428414941,23.5812499999162,-3.26591175476071));
#289141=CARTESIAN_POINT('Ctrl Pts',(8.13178807675716,23.7312499999156,-5.90808986649102));
#289142=CARTESIAN_POINT('Ctrl Pts',(6.21213331202019,23.881249999915,-8.55026797822134));
#289143=CARTESIAN_POINT('Ctrl Pts',(3.10606665601008,24.0312499999144,-9.5594902125713));
#289144=CARTESIAN_POINT('Ctrl Pts',(-2.70508270208248E-14,24.1812499999138,
-10.5687124469213));
#289145=CARTESIAN_POINT('Ctrl Pts',(-3.10606665601014,24.3312499999131,
-9.5594902125713));
#289146=CARTESIAN_POINT('Ctrl Pts',(-6.21213331202024,24.4812499999125,
-8.55026797822134));
#289147=CARTESIAN_POINT('Ctrl Pts',(-8.13178807675722,24.6312499999119,
-5.90808986649102));
#289148=CARTESIAN_POINT('Ctrl Pts',(-10.0514428414942,24.7812499999113,
-3.2659117547607));
#289149=CARTESIAN_POINT('Ctrl Pts',(-10.0514428414942,24.9312499999107,
2.46189346052968E-15));
#289150=CARTESIAN_POINT('Ctrl Pts',(-10.0514428414942,25.0812499999101,
3.26591175476071));
#289151=CARTESIAN_POINT('Ctrl Pts',(-8.13178807675722,25.2312499999095,
5.90808986649102));
#289152=CARTESIAN_POINT('Ctrl Pts',(-6.21213331202024,25.381249999909,8.55026797822134));
#289153=CARTESIAN_POINT('Ctrl Pts',(-3.10606665601013,25.5312499999084,
9.5594902125713));
#289154=CARTESIAN_POINT('Ctrl Pts',(-2.53260936828095E-14,25.6812499999078,
10.5687124469213));
#289155=CARTESIAN_POINT('Ctrl Pts',(3.10606665601008,25.8312499999072,9.5594902125713));
#289156=CARTESIAN_POINT('Ctrl Pts',(6.21213331202019,25.9812499999066,8.55026797822134));
#289157=CARTESIAN_POINT('Ctrl Pts',(8.13178807675716,26.131249999906,5.90808986649102));
#289158=CARTESIAN_POINT('Ctrl Pts',(10.0514428414941,26.2812499999054,3.2659117547607));
#289159=CARTESIAN_POINT('Ctrl Pts',(10.0514428414941,26.4312499999048,-1.23094673026484E-15));
#289160=CARTESIAN_POINT('Ctrl Pts',(10.0514428414941,26.5812499999042,-3.26591175476071));
#289161=CARTESIAN_POINT('Ctrl Pts',(8.13178807675716,26.7312499999036,-5.90808986649102));
#289162=CARTESIAN_POINT('Ctrl Pts',(6.21213331202019,26.881249999903,-8.55026797822134));
#289163=CARTESIAN_POINT('Ctrl Pts',(3.10606665601008,27.0312499999024,-9.5594902125713));
#289164=CARTESIAN_POINT('Ctrl Pts',(-2.87785362924866E-14,27.1812499999018,
-10.5687124469213));
#289165=CARTESIAN_POINT('Ctrl Pts',(-3.10606665601014,27.3312499999011,
-9.5594902125713));
#289166=CARTESIAN_POINT('Ctrl Pts',(-6.21213331202024,27.4812499999005,
-8.55026797822134));
#289167=CARTESIAN_POINT('Ctrl Pts',(-8.13178807675722,27.6312499998999,
-5.90808986649102));
#289168=CARTESIAN_POINT('Ctrl Pts',(-10.0514428414942,27.7812499998993,
-3.2659117547607));
#289169=CARTESIAN_POINT('Ctrl Pts',(-10.0514428414942,27.9312499998987,
2.46189346052968E-15));
#289170=CARTESIAN_POINT('Ctrl Pts',(-10.0514428414942,28.0812499998981,
3.26591175476071));
#289171=CARTESIAN_POINT('Ctrl Pts',(-8.13178807675722,28.2312499998975,
5.90808986649102));
#289172=CARTESIAN_POINT('Ctrl Pts',(-6.21213331202024,28.3812499998969,
8.55026797822134));
#289173=CARTESIAN_POINT('Ctrl Pts',(-3.10606665601014,28.5312499998964,
9.5594902125713));
#289174=CARTESIAN_POINT('Ctrl Pts',(-2.70538029544713E-14,28.6812499998958,
10.5687124469213));
#289175=CARTESIAN_POINT('Ctrl Pts',(3.10606665601008,28.8312499998952,9.5594902125713));
#289176=CARTESIAN_POINT('Ctrl Pts',(6.21213331202019,28.9812499998946,8.55026797822134));
#289177=CARTESIAN_POINT('Ctrl Pts',(8.13178807675716,29.131249999894,5.90808986649102));
#289178=CARTESIAN_POINT('Ctrl Pts',(10.0514428414941,29.2812499998934,3.2659117547607));
#289179=CARTESIAN_POINT('Ctrl Pts',(10.0514428414941,29.4312499998928,-1.23094673026484E-15));
#289180=CARTESIAN_POINT('Ctrl Pts',(10.0514428414941,29.5812499998922,-3.26591175476071));
#289181=CARTESIAN_POINT('Ctrl Pts',(8.13178807675716,29.7312499998916,-5.90808986649102));
#289182=CARTESIAN_POINT('Ctrl Pts',(6.21213331202019,29.881249999891,-8.55026797822134));
#289183=CARTESIAN_POINT('Ctrl Pts',(3.10606665601008,30.0312499998904,-9.5594902125713));
#289184=CARTESIAN_POINT('Ctrl Pts',(-3.05062455641484E-14,30.1812499998898,
-10.5687124469213));
#289185=CARTESIAN_POINT('Ctrl Pts',(-3.10606665601014,30.3312499998892,
-9.5594902125713));
#289186=CARTESIAN_POINT('Ctrl Pts',(-6.21213331202025,30.4812499998885,
-8.55026797822134));
#289187=CARTESIAN_POINT('Ctrl Pts',(-8.13178807675722,30.6312499998879,
-5.90808986649102));
#289188=CARTESIAN_POINT('Ctrl Pts',(-10.0514428414942,30.7812499998873,
-3.2659117547607));
#289189=CARTESIAN_POINT('Ctrl Pts',(-10.0514428414942,30.9312499998867,
2.46189346052968E-15));
#289190=CARTESIAN_POINT('Ctrl Pts',(-10.0514428414942,31.0812499998861,
3.26591175476071));
#289191=CARTESIAN_POINT('Ctrl Pts',(-8.13178807675722,31.2312499998855,
5.90808986649102));
#289192=CARTESIAN_POINT('Ctrl Pts',(-6.21213331202024,31.381249999885,8.55026797822134));
#289193=CARTESIAN_POINT('Ctrl Pts',(-3.10606665601014,31.5312499998843,
9.5594902125713));
#289194=CARTESIAN_POINT('Ctrl Pts',(-2.87815122261332E-14,31.6812499998838,
10.5687124469213));
#289195=CARTESIAN_POINT('Ctrl Pts',(3.10606665601008,31.8312499998832,9.5594902125713));
#289196=CARTESIAN_POINT('Ctrl Pts',(6.21213331202019,31.9812499998826,8.55026797822134));
#289197=CARTESIAN_POINT('Ctrl Pts',(8.13178807675716,32.131249999882,5.90808986649102));
#289198=CARTESIAN_POINT('Ctrl Pts',(10.0514428414941,32.2812499998814,3.2659117547607));
#289199=CARTESIAN_POINT('Ctrl Pts',(10.0514428414941,32.4312499998808,-1.23094673026484E-15));
#289200=CARTESIAN_POINT('Ctrl Pts',(10.0514428414941,32.5812499998802,-3.26591175476071));
#289201=CARTESIAN_POINT('Ctrl Pts',(8.13178807675716,32.7312499998796,-5.90808986649102));
#289202=CARTESIAN_POINT('Ctrl Pts',(6.21213331202019,32.8812499998789,-8.55026797822134));
#289203=CARTESIAN_POINT('Ctrl Pts',(3.10606665601008,33.0312499998784,-9.5594902125713));
#289204=CARTESIAN_POINT('Ctrl Pts',(-3.22339548358103E-14,33.1812499998777,
-10.5687124469213));
#289205=CARTESIAN_POINT('Ctrl Pts',(-3.10606665601014,33.3312499998772,
-9.5594902125713));
#289206=CARTESIAN_POINT('Ctrl Pts',(-6.21213331202025,33.4812499998766,
-8.55026797822134));
#289207=CARTESIAN_POINT('Ctrl Pts',(-8.13178807675722,33.6312499998759,
-5.90808986649102));
#289208=CARTESIAN_POINT('Ctrl Pts',(-10.0514428414942,33.7812499998753,
-3.2659117547607));
#289209=CARTESIAN_POINT('Ctrl Pts',(-10.0514428414942,33.9312499998747,
2.46189346052968E-15));
#289210=CARTESIAN_POINT('Ctrl Pts',(-10.0514428414942,34.0812499998741,
3.26591175476071));
#289211=CARTESIAN_POINT('Ctrl Pts',(-8.13178807675722,34.2312499998735,
5.90808986649102));
#289212=CARTESIAN_POINT('Ctrl Pts',(-6.21213331202024,34.3812499998729,
8.55026797822134));
#289213=CARTESIAN_POINT('Ctrl Pts',(-3.10606665601014,34.5312499998724,
9.5594902125713));
#289214=CARTESIAN_POINT('Ctrl Pts',(-3.0509221497795E-14,34.6812499998718,
10.5687124469213));
#289215=CARTESIAN_POINT('Ctrl Pts',(3.10606665601008,34.8312499998712,9.5594902125713));
#289216=CARTESIAN_POINT('Ctrl Pts',(6.21213331202019,34.9812499998706,8.55026797822134));
#289217=CARTESIAN_POINT('Ctrl Pts',(8.13178807675716,35.13124999987,5.90808986649102));
#289218=CARTESIAN_POINT('Ctrl Pts',(10.0514428414941,35.2812499998694,3.2659117547607));
#289219=CARTESIAN_POINT('Ctrl Pts',(10.0514428414941,35.4312499998688,-1.23094673026484E-15));
#289220=CARTESIAN_POINT('Ctrl Pts',(10.0514428414941,35.5812499998682,-3.26591175476071));
#289221=CARTESIAN_POINT('Ctrl Pts',(8.13178807675716,35.7312499998676,-5.90808986649102));
#289222=CARTESIAN_POINT('Ctrl Pts',(6.21213331202018,35.881249999867,-8.55026797822134));
#289223=CARTESIAN_POINT('Ctrl Pts',(3.10606665601007,36.0312499998664,-9.5594902125713));
#289224=CARTESIAN_POINT('Ctrl Pts',(-3.39616641074721E-14,36.1812499998658,
-10.5687124469213));
#289225=CARTESIAN_POINT('Ctrl Pts',(-3.10606665601014,36.3312499998652,
-9.5594902125713));
#289226=CARTESIAN_POINT('Ctrl Pts',(-6.21213331202025,36.4812499998646,
-8.55026797822134));
#289227=CARTESIAN_POINT('Ctrl Pts',(-8.13178807675722,36.6312499998639,
-5.90808986649102));
#289228=CARTESIAN_POINT('Ctrl Pts',(-10.0514428414942,36.7812499998634,
-3.2659117547607));
#289229=CARTESIAN_POINT('Ctrl Pts',(-10.0514428414942,36.9312499998627,
2.46189346052968E-15));
#289230=CARTESIAN_POINT('Ctrl Pts',(-10.0514428414942,37.0812499998621,
3.26591175476071));
#289231=CARTESIAN_POINT('Ctrl Pts',(-8.13178807675722,37.2312499998615,
5.90808986649102));
#289232=CARTESIAN_POINT('Ctrl Pts',(-6.21213331202025,37.3812499998609,
8.55026797822134));
#289233=CARTESIAN_POINT('Ctrl Pts',(-3.10606665601014,37.5312499998603,
9.5594902125713));
#289234=CARTESIAN_POINT('Ctrl Pts',(-3.22369307694568E-14,37.6812499998598,
10.5687124469213));
#289235=CARTESIAN_POINT('Ctrl Pts',(3.10606665601008,37.8312499998592,9.5594902125713));
#289236=CARTESIAN_POINT('Ctrl Pts',(6.21213331202018,37.9812499998586,8.55026797822134));
#289237=CARTESIAN_POINT('Ctrl Pts',(8.13178807675716,38.131249999858,5.90808986649102));
#289238=CARTESIAN_POINT('Ctrl Pts',(10.0514428414941,38.2812499998574,3.2659117547607));
#289239=CARTESIAN_POINT('Ctrl Pts',(10.0514428414941,38.4312499998568,-1.23094673026484E-15));
#289240=CARTESIAN_POINT('Ctrl Pts',(10.0514428414941,38.5812499998562,-3.26591175476071));
#289241=CARTESIAN_POINT('Ctrl Pts',(8.13178807675715,38.7312499998556,-5.90808986649102));
#289242=CARTESIAN_POINT('Ctrl Pts',(6.21213331202018,38.881249999855,-8.55026797822134));
#289243=CARTESIAN_POINT('Ctrl Pts',(3.10606665601007,39.0312499998544,-9.5594902125713));
#289244=CARTESIAN_POINT('Ctrl Pts',(-3.5689373379134E-14,39.1812499998538,
-10.5687124469213));
#289245=CARTESIAN_POINT('Ctrl Pts',(-3.10606665601014,39.3312499998532,
-9.5594902125713));
#289246=CARTESIAN_POINT('Ctrl Pts',(-6.21213331202025,39.4812499998525,
-8.55026797822134));
#289247=CARTESIAN_POINT('Ctrl Pts',(-8.13178807675723,39.6312499998519,
-5.90808986649102));
#289248=CARTESIAN_POINT('Ctrl Pts',(-10.0514428414942,39.7812499998513,
-3.2659117547607));
#289249=CARTESIAN_POINT('Ctrl Pts',(-10.0514428414942,39.9312499998507,
2.46189346052968E-15));
#289250=CARTESIAN_POINT('Ctrl Pts',(-10.0514428414942,40.0812499998502,
3.26591175476071));
#289251=CARTESIAN_POINT('Ctrl Pts',(-8.13178807675723,40.2312499998495,
5.90808986649102));
#289252=CARTESIAN_POINT('Ctrl Pts',(-6.21213331202025,40.3812499998489,
8.55026797822134));
#289253=CARTESIAN_POINT('Ctrl Pts',(-3.10606665601014,40.5312499998483,
9.5594902125713));
#289254=CARTESIAN_POINT('Ctrl Pts',(-3.39646400411187E-14,40.6812499998478,
10.5687124469213));
#289255=CARTESIAN_POINT('Ctrl Pts',(3.10606665601007,40.8312499998472,9.5594902125713));
#289256=CARTESIAN_POINT('Ctrl Pts',(6.21213331202018,40.9812499998466,8.55026797822134));
#289257=CARTESIAN_POINT('Ctrl Pts',(8.13178807675715,41.131249999846,5.90808986649102));
#289258=CARTESIAN_POINT('Ctrl Pts',(10.0514428414941,41.2812499998454,3.2659117547607));
#289259=CARTESIAN_POINT('Ctrl Pts',(10.0514428414941,41.4312499998448,-1.23094673026484E-15));
#289260=CARTESIAN_POINT('Ctrl Pts',(10.0514428414941,41.5812499998442,-3.26591175476071));
#289261=CARTESIAN_POINT('Ctrl Pts',(8.13178807675715,41.7312499998436,-5.90808986649102));
#289262=CARTESIAN_POINT('Ctrl Pts',(6.21213331202018,41.881249999843,-8.55026797822134));
#289263=CARTESIAN_POINT('Ctrl Pts',(3.10606665601007,42.0312499998423,-9.5594902125713));
#289264=CARTESIAN_POINT('Ctrl Pts',(-3.74170826507958E-14,42.1812499998418,
-10.5687124469213));
#289265=CARTESIAN_POINT('Ctrl Pts',(-3.10606665601015,42.3312499998411,
-9.5594902125713));
#289266=CARTESIAN_POINT('Ctrl Pts',(-6.21213331202025,42.4812499998406,
-8.55026797822134));
#289267=CARTESIAN_POINT('Ctrl Pts',(-8.13178807675723,42.6312499998399,
-5.90808986649102));
#289268=CARTESIAN_POINT('Ctrl Pts',(-10.0514428414942,42.7812499998393,
-3.2659117547607));
#289269=CARTESIAN_POINT('Ctrl Pts',(-10.0514428414942,42.9312499998387,
2.46189346052968E-15));
#289270=CARTESIAN_POINT('Ctrl Pts',(-10.0514428414942,43.0812499998381,
3.26591175476071));
#289271=CARTESIAN_POINT('Ctrl Pts',(-8.13178807675723,43.2312499998375,
5.90808986649102));
#289272=CARTESIAN_POINT('Ctrl Pts',(-6.21213331202025,43.3812499998369,
8.55026797822134));
#289273=CARTESIAN_POINT('Ctrl Pts',(-3.10606665601014,43.5312499998363,
9.5594902125713));
#289274=CARTESIAN_POINT('Ctrl Pts',(-3.56923493127805E-14,43.6812499998357,
10.5687124469213));
#289275=CARTESIAN_POINT('Ctrl Pts',(3.10606665601007,43.8312499998352,9.5594902125713));
#289276=CARTESIAN_POINT('Ctrl Pts',(6.21213331202018,43.9812499998345,8.55026797822134));
#289277=CARTESIAN_POINT('Ctrl Pts',(8.13178807675715,44.131249999834,5.90808986649102));
#289278=CARTESIAN_POINT('Ctrl Pts',(10.0514428414941,44.2812499998334,3.2659117547607));
#289279=CARTESIAN_POINT('Ctrl Pts',(10.0514428414941,44.4312499998328,-1.23094673026484E-15));
#289280=CARTESIAN_POINT('Ctrl Pts',(10.0514428414941,44.5812499998322,-3.26591175476071));
#289281=CARTESIAN_POINT('Ctrl Pts',(8.13178807675715,44.7312499998316,-5.90808986649102));
#289282=CARTESIAN_POINT('Ctrl Pts',(6.21213331202018,44.881249999831,-8.55026797822134));
#289283=CARTESIAN_POINT('Ctrl Pts',(3.10606665601007,45.0312499998304,-9.5594902125713));
#289284=CARTESIAN_POINT('Ctrl Pts',(-3.91447919224576E-14,45.1812499998297,
-10.5687124469213));
#289285=CARTESIAN_POINT('Ctrl Pts',(-3.10606665601015,45.3312499998292,
-9.5594902125713));
#289286=CARTESIAN_POINT('Ctrl Pts',(-6.21213331202026,45.4812499998285,
-8.55026797822134));
#289287=CARTESIAN_POINT('Ctrl Pts',(-8.13178807675723,45.6312499998279,
-5.90808986649102));
#289288=CARTESIAN_POINT('Ctrl Pts',(-10.0514428414942,45.7812499998273,
-3.2659117547607));
#289289=CARTESIAN_POINT('Ctrl Pts',(-10.0514428414942,45.9312499998267,
2.46189346052968E-15));
#289290=CARTESIAN_POINT('Ctrl Pts',(-10.0514428414942,46.0812499998261,
3.26591175476071));
#289291=CARTESIAN_POINT('Ctrl Pts',(-8.13178807675723,46.2312499998255,
5.90808986649102));
#289292=CARTESIAN_POINT('Ctrl Pts',(-6.21213331202025,46.3812499998249,
8.55026797822134));
#289293=CARTESIAN_POINT('Ctrl Pts',(-3.10606665601015,46.5312499998244,
9.5594902125713));
#289294=CARTESIAN_POINT('Ctrl Pts',(-3.74200585844424E-14,46.6812499998238,
10.5687124469213));
#289295=CARTESIAN_POINT('Ctrl Pts',(3.10606665601007,46.8312499998232,9.5594902125713));
#289296=CARTESIAN_POINT('Ctrl Pts',(6.21213331202018,46.9812499998226,8.55026797822134));
#289297=CARTESIAN_POINT('Ctrl Pts',(8.13178807675715,47.131249999822,5.90808986649102));
#289298=CARTESIAN_POINT('Ctrl Pts',(10.0514428414941,47.2812499998214,3.2659117547607));
#289299=CARTESIAN_POINT('Ctrl Pts',(10.0514428414941,47.4312499998208,-1.23094673026484E-15));
#289300=CARTESIAN_POINT('Ctrl Pts',(10.0514428414941,47.5812499998202,-3.26591175476071));
#289301=CARTESIAN_POINT('Ctrl Pts',(8.13178807675715,47.7312499998196,-5.90808986649102));
#289302=CARTESIAN_POINT('Ctrl Pts',(6.21213331202017,47.881249999819,-8.55026797822134));
#289303=CARTESIAN_POINT('Ctrl Pts',(3.10606665601007,48.0312499998184,-9.5594902125713));
#289304=CARTESIAN_POINT('Ctrl Pts',(-4.08725011941195E-14,48.1812499998178,
-10.5687124469213));
#289305=CARTESIAN_POINT('Ctrl Pts',(-3.10606665601015,48.3312499998172,
-9.5594902125713));
#289306=CARTESIAN_POINT('Ctrl Pts',(-6.21213331202026,48.4812499998166,
-8.55026797822134));
#289307=CARTESIAN_POINT('Ctrl Pts',(-8.13178807675723,48.6312499998159,
-5.90808986649102));
#289308=CARTESIAN_POINT('Ctrl Pts',(-10.0514428414942,48.7812499998153,
-3.2659117547607));
#289309=CARTESIAN_POINT('Ctrl Pts',(-10.0514428414942,48.9312499998147,
2.46189346052968E-15));
#289310=CARTESIAN_POINT('Ctrl Pts',(-10.0514428414942,49.0812499998141,
3.26591175476071));
#289311=CARTESIAN_POINT('Ctrl Pts',(-8.13178807675723,49.2312499998135,
5.90808986649102));
#289312=CARTESIAN_POINT('Ctrl Pts',(-6.21213331202026,49.3812499998129,
8.55026797822134));
#289313=CARTESIAN_POINT('Ctrl Pts',(-3.10606665601015,49.5312499998124,
9.5594902125713));
#289314=CARTESIAN_POINT('Ctrl Pts',(-3.91477678561042E-14,49.6812499998117,
10.5687124469213));
#289315=CARTESIAN_POINT('Ctrl Pts',(3.10606665601007,49.8312499998111,9.5594902125713));
#289316=CARTESIAN_POINT('Ctrl Pts',(6.21213331202017,49.9812499998106,8.55026797822134));
#289317=CARTESIAN_POINT('Ctrl Pts',(8.13178807675715,50.13124999981,5.90808986649102));
#289318=CARTESIAN_POINT('Ctrl Pts',(10.0514428414941,50.2812499998094,3.2659117547607));
#289319=CARTESIAN_POINT('Ctrl Pts',(10.0514428414941,50.4312499998088,-1.23094673026484E-15));
#289320=CARTESIAN_POINT('Ctrl Pts',(10.0514428414941,50.5812499998082,-3.26591175476071));
#289321=CARTESIAN_POINT('Ctrl Pts',(8.13178807675715,50.7312499998076,-5.90808986649102));
#289322=CARTESIAN_POINT('Ctrl Pts',(6.21213331202017,50.881249999807,-8.55026797822134));
#289323=CARTESIAN_POINT('Ctrl Pts',(3.10606665601007,51.0312499998064,-9.5594902125713));
#289324=CARTESIAN_POINT('Ctrl Pts',(-4.26002104657813E-14,51.1812499998058,
-10.5687124469213));
#289325=CARTESIAN_POINT('Ctrl Pts',(-3.10606665601015,51.3312499998052,
-9.5594902125713));
#289326=CARTESIAN_POINT('Ctrl Pts',(-6.21213331202026,51.4812499998045,
-8.55026797822134));
#289327=CARTESIAN_POINT('Ctrl Pts',(-8.13178807675723,51.631249999804,-5.90808986649102));
#289328=CARTESIAN_POINT('Ctrl Pts',(-10.0514428414942,51.7812499998034,
-3.2659117547607));
#289329=CARTESIAN_POINT('Ctrl Pts',(-10.0514428414942,51.9312499998027,
2.46189346052968E-15));
#289330=CARTESIAN_POINT('Ctrl Pts',(-10.0514428414942,52.0812499998021,
3.26591175476071));
#289331=CARTESIAN_POINT('Ctrl Pts',(-8.13178807675723,52.2312499998015,
5.90808986649102));
#289332=CARTESIAN_POINT('Ctrl Pts',(-6.21213331202026,52.3812499998009,
8.55026797822134));
#289333=CARTESIAN_POINT('Ctrl Pts',(-3.10606665601015,52.5312499998004,
9.5594902125713));
#289334=CARTESIAN_POINT('Ctrl Pts',(-4.08754771277661E-14,52.6812499997998,
10.5687124469213));
#289335=CARTESIAN_POINT('Ctrl Pts',(3.10606665601007,52.8312499997991,9.5594902125713));
#289336=CARTESIAN_POINT('Ctrl Pts',(6.21213331202017,52.9812499997986,8.55026797822134));
#289337=CARTESIAN_POINT('Ctrl Pts',(8.13178807675715,53.131249999798,5.90808986649102));
#289338=CARTESIAN_POINT('Ctrl Pts',(10.0514428414941,53.2812499997974,3.2659117547607));
#289339=CARTESIAN_POINT('Ctrl Pts',(10.0514428414941,53.4312499997968,-1.23094673026484E-15));
#289340=CARTESIAN_POINT('Ctrl Pts',(10.0514428414941,53.5812499997962,-3.26591175476071));
#289341=CARTESIAN_POINT('Ctrl Pts',(8.13178807675714,53.7312499997956,-5.90808986649102));
#289342=CARTESIAN_POINT('Ctrl Pts',(6.21213331202017,53.881249999795,-8.55026797822134));
#289343=CARTESIAN_POINT('Ctrl Pts',(3.10606665601006,54.0312499997944,-9.5594902125713));
#289344=CARTESIAN_POINT('Ctrl Pts',(-4.43279197374432E-14,54.1812499997938,
-10.5687124469213));
#289345=CARTESIAN_POINT('Ctrl Pts',(-3.10606665601015,54.3312499997932,
-9.5594902125713));
#289346=CARTESIAN_POINT('Ctrl Pts',(-6.21213331202026,54.4812499997926,
-8.55026797822134));
#289347=CARTESIAN_POINT('Ctrl Pts',(-8.13178807675724,54.6312499997919,
-5.90808986649102));
#289348=CARTESIAN_POINT('Ctrl Pts',(-10.0514428414942,54.7812499997914,
-3.2659117547607));
#289349=CARTESIAN_POINT('Ctrl Pts',(-10.0514428414942,54.9312499997907,
2.46189346052968E-15));
#289350=CARTESIAN_POINT('Ctrl Pts',(-10.0514428414942,55.0812499997901,
3.26591175476071));
#289351=CARTESIAN_POINT('Ctrl Pts',(-8.13178807675724,55.2312499997895,
5.90808986649102));
#289352=CARTESIAN_POINT('Ctrl Pts',(-6.21213331202026,55.3812499997889,
8.55026797822134));
#289353=CARTESIAN_POINT('Ctrl Pts',(-3.10606665601015,55.5312499997884,
9.5594902125713));
#289354=CARTESIAN_POINT('Ctrl Pts',(-4.26031863994279E-14,55.6812499997877,
10.5687124469213));
#289355=CARTESIAN_POINT('Ctrl Pts',(3.10606665601006,55.8312499997871,9.5594902125713));
#289356=CARTESIAN_POINT('Ctrl Pts',(6.21213331202017,55.9812499997865,8.55026797822134));
#289357=CARTESIAN_POINT('Ctrl Pts',(8.13178807675714,56.131249999786,5.90808986649102));
#289358=CARTESIAN_POINT('Ctrl Pts',(10.0514428414941,56.2812499997854,3.2659117547607));
#289359=CARTESIAN_POINT('Ctrl Pts',(10.0514428414941,56.4312499997848,-1.23094673026484E-15));
#289360=CARTESIAN_POINT('Ctrl Pts',(10.0514428414941,56.5812499997842,-3.26591175476071));
#289361=CARTESIAN_POINT('Ctrl Pts',(8.13178807675714,56.7312499997836,-5.90808986649102));
#289362=CARTESIAN_POINT('Ctrl Pts',(6.21213331202017,56.881249999783,-8.55026797822134));
#289363=CARTESIAN_POINT('Ctrl Pts',(3.10606665601006,57.0312499997824,-9.5594902125713));
#289364=CARTESIAN_POINT('Ctrl Pts',(-4.6055629009105E-14,57.1812499997818,
-10.5687124469213));
#289365=CARTESIAN_POINT('Ctrl Pts',(-3.10606665601015,57.3312499997812,
-9.5594902125713));
#289366=CARTESIAN_POINT('Ctrl Pts',(-6.21213331202026,57.4812499997805,
-8.55026797822134));
#289367=CARTESIAN_POINT('Ctrl Pts',(-8.13178807675724,57.6312499997799,
-5.90808986649102));
#289368=CARTESIAN_POINT('Ctrl Pts',(-10.0514428414942,57.7812499997793,
-3.2659117547607));
#289369=CARTESIAN_POINT('Ctrl Pts',(-10.0514428414942,57.9312499997787,
2.46189346052968E-15));
#289370=CARTESIAN_POINT('Ctrl Pts',(-10.0514428414942,58.0812499997781,
3.26591175476071));
#289371=CARTESIAN_POINT('Ctrl Pts',(-8.13178807675724,58.2312499997775,
5.90808986649102));
#289372=CARTESIAN_POINT('Ctrl Pts',(-6.21213331202026,58.3812499997769,
8.55026797822134));
#289373=CARTESIAN_POINT('Ctrl Pts',(-3.10606665601015,58.5312499997763,
9.5594902125713));
#289374=CARTESIAN_POINT('Ctrl Pts',(-4.43308956710897E-14,58.6812499997758,
10.5687124469213));
#289375=CARTESIAN_POINT('Ctrl Pts',(3.10606665601006,58.8312499997751,9.5594902125713));
#289376=CARTESIAN_POINT('Ctrl Pts',(6.21213331202017,58.9812499997745,8.55026797822134));
#289377=CARTESIAN_POINT('Ctrl Pts',(8.13178807675714,59.131249999774,5.90808986649102));
#289378=CARTESIAN_POINT('Ctrl Pts',(10.0514428414941,59.2812499997734,3.2659117547607));
#289379=CARTESIAN_POINT('Ctrl Pts',(10.0514428414941,59.4312499997728,-1.23094673026484E-15));
#289380=CARTESIAN_POINT('Ctrl Pts',(10.0514428414941,59.5812499997722,-3.26591175476071));
#289381=CARTESIAN_POINT('Ctrl Pts',(8.13178807675714,59.7312499997716,-5.90808986649102));
#289382=CARTESIAN_POINT('Ctrl Pts',(6.21213331202017,59.881249999771,-8.55026797822134));
#289383=CARTESIAN_POINT('Ctrl Pts',(3.10606665601006,60.0312499997704,-9.5594902125713));
#289384=CARTESIAN_POINT('Ctrl Pts',(-4.77833382807668E-14,60.1812499997698,
-10.5687124469213));
#289385=CARTESIAN_POINT('Ctrl Pts',(-3.10606665601016,60.3312499997692,
-9.5594902125713));
#289386=CARTESIAN_POINT('Ctrl Pts',(-6.21213331202026,60.4812499997686,
-8.55026797822134));
#289387=CARTESIAN_POINT('Ctrl Pts',(-8.13178807675724,60.6312499997679,
-5.90808986649102));
#289388=CARTESIAN_POINT('Ctrl Pts',(-10.0514428414942,60.7812499997674,
-3.2659117547607));
#289389=CARTESIAN_POINT('Ctrl Pts',(-10.0514428414942,60.9312499997667,
2.46189346052968E-15));
#289390=CARTESIAN_POINT('Ctrl Pts',(-10.0514428414942,61.0812499997661,
3.26591175476071));
#289391=CARTESIAN_POINT('Ctrl Pts',(-8.13178807675724,61.2312499997655,
5.90808986649102));
#289392=CARTESIAN_POINT('Ctrl Pts',(-6.21213331202026,61.3812499997649,
8.55026797822134));
#289393=CARTESIAN_POINT('Ctrl Pts',(-3.10606665601015,61.5312499997643,
9.5594902125713));
#289394=CARTESIAN_POINT('Ctrl Pts',(-4.60586049427516E-14,61.6812499997638,
10.5687124469213));
#289395=CARTESIAN_POINT('Ctrl Pts',(3.10606665601006,61.8312499997632,9.5594902125713));
#289396=CARTESIAN_POINT('Ctrl Pts',(6.21213331202017,61.9812499997625,8.55026797822134));
#289397=CARTESIAN_POINT('Ctrl Pts',(8.13178807675714,62.131249999762,5.90808986649102));
#289398=CARTESIAN_POINT('Ctrl Pts',(10.0514428414941,62.2812499997614,3.2659117547607));
#289399=CARTESIAN_POINT('Ctrl Pts',(10.0514428414941,62.4312499997608,-1.23094673026484E-15));
#289400=CARTESIAN_POINT('Ctrl Pts',(10.0514428414941,62.5812499997602,-3.26591175476071));
#289401=CARTESIAN_POINT('Ctrl Pts',(8.13178807675714,62.7312499997596,-5.90808986649102));
#289402=CARTESIAN_POINT('Ctrl Pts',(6.21213331202017,62.881249999759,-8.55026797822134));
#289403=CARTESIAN_POINT('Ctrl Pts',(3.10606665601006,63.0312499997584,-9.5594902125713));
#289404=CARTESIAN_POINT('Ctrl Pts',(-4.95110475524287E-14,63.1812499997578,
-10.5687124469213));
#289405=CARTESIAN_POINT('Ctrl Pts',(-3.10606665601016,63.3312499997572,
-9.5594902125713));
#289406=CARTESIAN_POINT('Ctrl Pts',(-6.21213331202027,63.4812499997565,
-8.55026797822134));
#289407=CARTESIAN_POINT('Ctrl Pts',(-8.13178807675724,63.631249999756,-5.90808986649102));
#289408=CARTESIAN_POINT('Ctrl Pts',(-10.0514428414942,63.7812499997553,
-3.2659117547607));
#289409=CARTESIAN_POINT('Ctrl Pts',(-10.0514428414942,63.9312499997548,
2.46189346052968E-15));
#289410=CARTESIAN_POINT('Ctrl Pts',(-10.0514428414942,64.0812499997541,
3.26591175476071));
#289411=CARTESIAN_POINT('Ctrl Pts',(-8.13178807675724,64.2312499997535,
5.90808986649102));
#289412=CARTESIAN_POINT('Ctrl Pts',(-6.21213331202026,64.381249999753,8.55026797822134));
#289413=CARTESIAN_POINT('Ctrl Pts',(-3.10606665601016,64.5312499997523,
9.5594902125713));
#289414=CARTESIAN_POINT('Ctrl Pts',(-4.77863142144134E-14,64.6812499997518,
10.5687124469213));
#289415=CARTESIAN_POINT('Ctrl Pts',(3.10606665601006,64.8312499997512,9.5594902125713));
#289416=CARTESIAN_POINT('Ctrl Pts',(6.21213331202017,64.9812499997506,8.55026797822134));
#289417=CARTESIAN_POINT('Ctrl Pts',(8.13178807675714,65.13124999975,5.90808986649102));
#289418=CARTESIAN_POINT('Ctrl Pts',(10.0514428414941,65.2812499997493,3.2659117547607));
#289419=CARTESIAN_POINT('Ctrl Pts',(10.0514428414941,65.4312499997488,-1.23094673026484E-15));
#289420=CARTESIAN_POINT('Ctrl Pts',(10.0514428414941,65.5812499997482,-3.26591175476071));
#289421=CARTESIAN_POINT('Ctrl Pts',(8.13178807675714,65.7312499997475,-5.90808986649102));
#289422=CARTESIAN_POINT('Ctrl Pts',(6.21213331202016,65.881249999747,-8.55026797822134));
#289423=CARTESIAN_POINT('Ctrl Pts',(3.10606665601006,66.0312499997464,-9.5594902125713));
#289424=CARTESIAN_POINT('Ctrl Pts',(-5.12387568240905E-14,66.1812499997457,
-10.5687124469213));
#289425=CARTESIAN_POINT('Ctrl Pts',(-3.10606665601016,66.3312499997451,
-9.5594902125713));
#289426=CARTESIAN_POINT('Ctrl Pts',(-6.21213331202027,66.4812499997445,
-8.55026797822134));
#289427=CARTESIAN_POINT('Ctrl Pts',(-8.13178807675724,66.6312499997439,
-5.90808986649102));
#289428=CARTESIAN_POINT('Ctrl Pts',(-10.0514428414942,66.7812499997433,
-3.2659117547607));
#289429=CARTESIAN_POINT('Ctrl Pts',(-10.0514428414942,66.9312499997427,
2.46189346052968E-15));
#289430=CARTESIAN_POINT('Ctrl Pts',(-10.0514428414942,67.0812499997421,
3.26591175476071));
#289431=CARTESIAN_POINT('Ctrl Pts',(-8.13178807675724,67.2312499997416,
5.90808986649102));
#289432=CARTESIAN_POINT('Ctrl Pts',(-6.21213331202027,67.3812499997409,
8.55026797822134));
#289433=CARTESIAN_POINT('Ctrl Pts',(-3.10606665601016,67.5312499997404,
9.5594902125713));
#289434=CARTESIAN_POINT('Ctrl Pts',(-4.95140234860752E-14,67.6812499997397,
10.5687124469213));
#289435=CARTESIAN_POINT('Ctrl Pts',(3.10606665601006,67.8312499997391,9.5594902125713));
#289436=CARTESIAN_POINT('Ctrl Pts',(6.21213331202017,67.9812499997385,8.55026797822134));
#289437=CARTESIAN_POINT('Ctrl Pts',(8.13178807675714,68.1312499997379,5.90808986649102));
#289438=CARTESIAN_POINT('Ctrl Pts',(10.0514428414941,68.2812499997374,3.2659117547607));
#289439=CARTESIAN_POINT('Ctrl Pts',(10.0514428414941,68.4312499997367,-1.23094673026484E-15));
#289440=CARTESIAN_POINT('Ctrl Pts',(10.0514428414941,68.5812499997361,-3.26591175476071));
#289441=CARTESIAN_POINT('Ctrl Pts',(8.13178807675714,68.7312499997356,-5.90808986649102));
#289442=CARTESIAN_POINT('Ctrl Pts',(6.21213331202016,68.881249999735,-8.55026797822134));
#289443=CARTESIAN_POINT('Ctrl Pts',(3.10606665601006,69.0312499997344,-9.5594902125713));
#289444=CARTESIAN_POINT('Ctrl Pts',(-5.29664660957524E-14,69.1812499997337,
-10.5687124469213));
#289445=CARTESIAN_POINT('Ctrl Pts',(-3.10606665601016,69.3312499997332,
-9.5594902125713));
#289446=CARTESIAN_POINT('Ctrl Pts',(-6.21213331202027,69.4812499997326,
-8.55026797822134));
#289447=CARTESIAN_POINT('Ctrl Pts',(-8.13178807675724,69.6312499997319,
-5.90808986649102));
#289448=CARTESIAN_POINT('Ctrl Pts',(-10.0514428414942,69.7812499997313,
-3.2659117547607));
#289449=CARTESIAN_POINT('Ctrl Pts',(-10.0514428414942,69.9312499997307,
2.46189346052968E-15));
#289450=CARTESIAN_POINT('Ctrl Pts',(-10.0514428414942,70.0812499997301,
3.26591175476071));
#289451=CARTESIAN_POINT('Ctrl Pts',(-8.13178807675724,70.2312499997295,
5.90808986649102));
#289452=CARTESIAN_POINT('Ctrl Pts',(-6.21213331202027,70.3812499997289,
8.55026797822134));
#289453=CARTESIAN_POINT('Ctrl Pts',(-3.10606665601016,70.5312499997283,
9.5594902125713));
#289454=CARTESIAN_POINT('Ctrl Pts',(-5.12417327577371E-14,70.6812499997277,
10.5687124469213));
#289455=CARTESIAN_POINT('Ctrl Pts',(3.10606665601006,70.8312499997271,9.5594902125713));
#289456=CARTESIAN_POINT('Ctrl Pts',(6.21213331202016,70.9812499997265,8.55026797822134));
#289457=CARTESIAN_POINT('Ctrl Pts',(8.13178807675714,71.131249999726,5.90808986649102));
#289458=CARTESIAN_POINT('Ctrl Pts',(10.0514428414941,71.2812499997253,3.2659117547607));
#289459=CARTESIAN_POINT('Ctrl Pts',(10.0514428414941,71.4312499997248,-1.23094673026484E-15));
#289460=CARTESIAN_POINT('Ctrl Pts',(10.0514428414941,71.5812499997242,-3.26591175476071));
#289461=CARTESIAN_POINT('Ctrl Pts',(8.13178807675713,71.7312499997236,-5.90808986649102));
#289462=CARTESIAN_POINT('Ctrl Pts',(6.21213331202016,71.881249999723,-8.55026797822134));
#289463=CARTESIAN_POINT('Ctrl Pts',(3.10606665601005,72.0312499997223,-9.5594902125713));
#289464=CARTESIAN_POINT('Ctrl Pts',(-5.46941753674142E-14,72.1812499997217,
-10.5687124469213));
#289465=CARTESIAN_POINT('Ctrl Pts',(-3.10606665601016,72.3312499997212,
-9.5594902125713));
#289466=CARTESIAN_POINT('Ctrl Pts',(-6.21213331202027,72.4812499997205,
-8.55026797822134));
#289467=CARTESIAN_POINT('Ctrl Pts',(-8.13178807675725,72.63124999972,-5.90808986649102));
#289468=CARTESIAN_POINT('Ctrl Pts',(-10.0514428414942,72.7812499997193,
-3.2659117547607));
#289469=CARTESIAN_POINT('Ctrl Pts',(-10.0514428414942,72.9312499997187,
2.46189346052968E-15));
#289470=CARTESIAN_POINT('Ctrl Pts',(-10.0514428414942,73.0812499997181,
3.26591175476071));
#289471=CARTESIAN_POINT('Ctrl Pts',(-8.13178807675725,73.2312499997175,
5.90808986649102));
#289472=CARTESIAN_POINT('Ctrl Pts',(-6.21213331202027,73.381249999717,8.55026797822134));
#289473=CARTESIAN_POINT('Ctrl Pts',(-3.10606665601016,73.5312499997164,
9.5594902125713));
#289474=CARTESIAN_POINT('Ctrl Pts',(-5.29694420293989E-14,73.6812499997157,
10.5687124469213));
#289475=CARTESIAN_POINT('Ctrl Pts',(3.10606665601005,73.8312499997151,9.5594902125713));
#289476=CARTESIAN_POINT('Ctrl Pts',(6.21213331202016,73.9812499997146,8.55026797822134));
#289477=CARTESIAN_POINT('Ctrl Pts',(8.13178807675713,74.1312499997139,5.90808986649102));
#289478=CARTESIAN_POINT('Ctrl Pts',(10.0514428414941,74.2812499997134,3.2659117547607));
#289479=CARTESIAN_POINT('Ctrl Pts',(10.0514428414941,74.4312499997127,-1.23094673026484E-15));
#289480=CARTESIAN_POINT('Ctrl Pts',(10.0514428414941,74.5812499997122,-3.26591175476071));
#289481=CARTESIAN_POINT('Ctrl Pts',(8.13178807675713,74.7312499997116,-5.90808986649102));
#289482=CARTESIAN_POINT('Ctrl Pts',(6.21213331202016,74.8812499997109,-8.55026797822134));
#289483=CARTESIAN_POINT('Ctrl Pts',(3.10606665601005,75.0312499997104,-9.5594902125713));
#289484=CARTESIAN_POINT('Ctrl Pts',(-5.6421884639076E-14,75.1812499997098,
-10.5687124469213));
#289485=CARTESIAN_POINT('Ctrl Pts',(-3.10606665601016,75.3312499997092,
-9.5594902125713));
#289486=CARTESIAN_POINT('Ctrl Pts',(-6.21213331202027,75.4812499997086,
-8.55026797822134));
#289487=CARTESIAN_POINT('Ctrl Pts',(-8.13178807675725,75.6312499997079,
-5.90808986649102));
#289488=CARTESIAN_POINT('Ctrl Pts',(-10.0514428414942,75.7812499997073,
-3.2659117547607));
#289489=CARTESIAN_POINT('Ctrl Pts',(-10.0514428414942,75.9312499997068,
2.46189346052968E-15));
#289490=CARTESIAN_POINT('Ctrl Pts',(-10.0514428414942,76.0812499997061,
3.26591175476071));
#289491=CARTESIAN_POINT('Ctrl Pts',(-8.13178807675725,76.2312499997055,
5.90808986649102));
#289492=CARTESIAN_POINT('Ctrl Pts',(-6.21213331202027,76.3812499997049,
8.55026797822134));
#289493=CARTESIAN_POINT('Ctrl Pts',(-3.10606665601016,76.5312499997043,
9.5594902125713));
#289494=CARTESIAN_POINT('Ctrl Pts',(-5.46971513010608E-14,76.6812499997037,
10.5687124469213));
#289495=CARTESIAN_POINT('Ctrl Pts',(3.10606665601005,76.8312499997031,9.5594902125713));
#289496=CARTESIAN_POINT('Ctrl Pts',(6.21213331202016,76.9812499997025,8.55026797822134));
#289497=CARTESIAN_POINT('Ctrl Pts',(8.13178807675713,77.131249999702,5.90808986649102));
#289498=CARTESIAN_POINT('Ctrl Pts',(10.0514428414941,77.2812499997013,3.2659117547607));
#289499=CARTESIAN_POINT('Ctrl Pts',(10.0514428414941,77.4312499997008,-1.23094673026484E-15));
#289500=CARTESIAN_POINT('Ctrl Pts',(10.0514428414941,77.5812499997001,-3.26591175476071));
#289501=CARTESIAN_POINT('Ctrl Pts',(8.13178807675713,77.7312499996995,-5.90808986649102));
#289502=CARTESIAN_POINT('Ctrl Pts',(6.21213331202016,77.881249999699,-8.55026797822134));
#289503=CARTESIAN_POINT('Ctrl Pts',(3.10606665601005,78.0312499996984,-9.5594902125713));
#289504=CARTESIAN_POINT('Ctrl Pts',(-5.81495939107379E-14,78.1812499996978,
-10.5687124469213));
#289505=CARTESIAN_POINT('Ctrl Pts',(-3.10606665601017,78.3312499996971,
-9.5594902125713));
#289506=CARTESIAN_POINT('Ctrl Pts',(-6.21213331202028,78.4812499996966,
-8.55026797822134));
#289507=CARTESIAN_POINT('Ctrl Pts',(-8.13178807675725,78.631249999696,-5.90808986649102));
#289508=CARTESIAN_POINT('Ctrl Pts',(-10.0514428414942,78.7812499996954,
-3.2659117547607));
#289509=CARTESIAN_POINT('Ctrl Pts',(-10.0514428414942,78.9312499996948,
2.46189346052968E-15));
#289510=CARTESIAN_POINT('Ctrl Pts',(-10.0514428414942,79.0812499996942,
3.26591175476071));
#289511=CARTESIAN_POINT('Ctrl Pts',(-8.13178807675725,79.2312499996936,
5.90808986649102));
#289512=CARTESIAN_POINT('Ctrl Pts',(-6.21213331202027,79.381249999693,8.55026797822134));
#289513=CARTESIAN_POINT('Ctrl Pts',(-3.10606665601016,79.5312499996923,
9.5594902125713));
#289514=CARTESIAN_POINT('Ctrl Pts',(-5.64248605727226E-14,79.6812499996917,
10.5687124469213));
#289515=CARTESIAN_POINT('Ctrl Pts',(3.10606665601005,79.8312499996911,9.5594902125713));
#289516=CARTESIAN_POINT('Ctrl Pts',(6.21213331202016,79.9812499996905,8.55026797822134));
#289517=CARTESIAN_POINT('Ctrl Pts',(8.13178807675713,80.1312499996899,5.90808986649102));
#289518=CARTESIAN_POINT('Ctrl Pts',(10.0514428414941,80.2812499996894,3.2659117547607));
#289519=CARTESIAN_POINT('Ctrl Pts',(10.0514428414941,80.4312499996887,-1.23094673026484E-15));
#289520=CARTESIAN_POINT('Ctrl Pts',(10.0514428414941,80.5812499996882,-3.26591175476071));
#289521=CARTESIAN_POINT('Ctrl Pts',(8.13178807675713,80.7312499996875,-5.90808986649102));
#289522=CARTESIAN_POINT('Ctrl Pts',(6.21213331202016,80.881249999687,-8.55026797822134));
#289523=CARTESIAN_POINT('Ctrl Pts',(3.10606665601005,81.0312499996864,-9.5594902125713));
#289524=CARTESIAN_POINT('Ctrl Pts',(-5.98773031823997E-14,81.1812499996858,
-10.5687124469213));
#289525=CARTESIAN_POINT('Ctrl Pts',(-3.10606665601017,81.3312499996851,
-9.5594902125713));
#289526=CARTESIAN_POINT('Ctrl Pts',(-6.21213331202028,81.4812499996845,
-8.55026797822134));
#289527=CARTESIAN_POINT('Ctrl Pts',(-8.13178807675725,81.6312499996839,
-5.90808986649102));
#289528=CARTESIAN_POINT('Ctrl Pts',(-10.0514428414942,81.7812499996834,
-3.2659117547607));
#289529=CARTESIAN_POINT('Ctrl Pts',(-10.0514428414942,81.9312499996827,
2.46189346052968E-15));
#289530=CARTESIAN_POINT('Ctrl Pts',(-10.0514428414942,82.0812499996821,
3.26591175476071));
#289531=CARTESIAN_POINT('Ctrl Pts',(-8.13178807675725,82.2312499996816,
5.90808986649102));
#289532=CARTESIAN_POINT('Ctrl Pts',(-6.21213331202028,82.381249999681,8.55026797822134));
#289533=CARTESIAN_POINT('Ctrl Pts',(-3.10606665601017,82.5312499996804,
9.5594902125713));
#289534=CARTESIAN_POINT('Ctrl Pts',(-5.81525698443845E-14,82.6812499996797,
10.5687124469213));
#289535=CARTESIAN_POINT('Ctrl Pts',(3.10606665601005,82.8312499996792,9.5594902125713));
#289536=CARTESIAN_POINT('Ctrl Pts',(6.21213331202016,82.9812499996786,8.55026797822134));
#289537=CARTESIAN_POINT('Ctrl Pts',(8.13178807675713,83.131249999678,5.90808986649102));
#289538=CARTESIAN_POINT('Ctrl Pts',(10.0514428414941,83.2812499996773,3.2659117547607));
#289539=CARTESIAN_POINT('Ctrl Pts',(10.0514428414941,83.4312499996767,-1.23094673026484E-15));
#289540=CARTESIAN_POINT('Ctrl Pts',(10.0514428414941,83.5812499996761,-3.26591175476071));
#289541=CARTESIAN_POINT('Ctrl Pts',(8.13178807675713,83.7312499996756,-5.90808986649102));
#289542=CARTESIAN_POINT('Ctrl Pts',(6.21213331202016,83.8812499996749,-8.55026797822134));
#289543=CARTESIAN_POINT('Ctrl Pts',(3.10606665601005,84.0312499996743,-9.5594902125713));
#289544=CARTESIAN_POINT('Ctrl Pts',(-6.16050124540615E-14,84.1812499996738,
-10.5687124469213));
#289545=CARTESIAN_POINT('Ctrl Pts',(-3.10606665601017,84.3312499996732,
-9.5594902125713));
#289546=CARTESIAN_POINT('Ctrl Pts',(-6.21213331202028,84.4812499996725,
-8.55026797822134));
#289547=CARTESIAN_POINT('Ctrl Pts',(-8.13178807675725,84.631249999672,-5.90808986649102));
#289548=CARTESIAN_POINT('Ctrl Pts',(-10.0514428414942,84.7812499996714,
-3.2659117547607));
#289549=CARTESIAN_POINT('Ctrl Pts',(-10.0514428414942,84.9312499996708,
2.46189346052968E-15));
#289550=CARTESIAN_POINT('Ctrl Pts',(-10.0514428414942,85.0812499996701,
3.26591175476071));
#289551=CARTESIAN_POINT('Ctrl Pts',(-8.13178807675725,85.2312499996695,
5.90808986649102));
#289552=CARTESIAN_POINT('Ctrl Pts',(-6.21213331202028,85.381249999669,8.55026797822134));
#289553=CARTESIAN_POINT('Ctrl Pts',(-3.10606665601017,85.5312499996683,
9.5594902125713));
#289554=CARTESIAN_POINT('Ctrl Pts',(-5.98802791160463E-14,85.6812499996678,
10.5687124469213));
#289555=CARTESIAN_POINT('Ctrl Pts',(3.10606665601005,85.8312499996672,9.5594902125713));
#289556=CARTESIAN_POINT('Ctrl Pts',(6.21213331202016,85.9812499996666,8.55026797822134));
#289557=CARTESIAN_POINT('Ctrl Pts',(8.13178807675713,86.1312499996659,5.90808986649102));
#289558=CARTESIAN_POINT('Ctrl Pts',(10.0514428414941,86.2812499996653,3.2659117547607));
#289559=CARTESIAN_POINT('Ctrl Pts',(10.0514428414941,86.4312499996647,-1.23094673026484E-15));
#289560=CARTESIAN_POINT('Ctrl Pts',(10.0514428414941,86.5812499996642,-3.26591175476071));
#289561=CARTESIAN_POINT('Ctrl Pts',(8.13178807675713,86.7312499996635,-5.90808986649102));
#289562=CARTESIAN_POINT('Ctrl Pts',(6.21213331202015,86.8812499996629,-8.55026797822134));
#289563=CARTESIAN_POINT('Ctrl Pts',(3.10606665601004,87.0312499996624,-9.5594902125713));
#289564=CARTESIAN_POINT('Ctrl Pts',(-6.33327217257234E-14,87.1812499996618,
-10.5687124469213));
#289565=CARTESIAN_POINT('Ctrl Pts',(-3.10606665601017,87.3312499996611,
-9.5594902125713));
#289566=CARTESIAN_POINT('Ctrl Pts',(-6.21213331202028,87.4812499996605,
-8.55026797822134));
#289567=CARTESIAN_POINT('Ctrl Pts',(-8.13178807675726,87.6312499996599,
-5.90808986649102));
#289568=CARTESIAN_POINT('Ctrl Pts',(-10.0514428414942,87.7812499996594,
-3.2659117547607));
#289569=CARTESIAN_POINT('Ctrl Pts',(-10.0514428414942,87.9312499996587,
2.46189346052968E-15));
#289570=CARTESIAN_POINT('Ctrl Pts',(-10.0514428414942,88.0812499996581,
3.26591175476071));
#289571=CARTESIAN_POINT('Ctrl Pts',(-8.13178807675726,88.2312499996575,
5.90808986649102));
#289572=CARTESIAN_POINT('Ctrl Pts',(-6.21213331202028,88.3812499996569,
8.55026797822134));
#289573=CARTESIAN_POINT('Ctrl Pts',(-3.10606665601017,88.5312499996564,
9.5594902125713));
#289574=CARTESIAN_POINT('Ctrl Pts',(-6.16079883877081E-14,88.6812499996557,
10.5687124469213));
#289575=CARTESIAN_POINT('Ctrl Pts',(3.10606665601005,88.8312499996552,9.5594902125713));
#289576=CARTESIAN_POINT('Ctrl Pts',(6.21213331202016,88.9812499996546,8.55026797822134));
#289577=CARTESIAN_POINT('Ctrl Pts',(8.13178807675713,89.131249999654,5.90808986649102));
#289578=CARTESIAN_POINT('Ctrl Pts',(10.0514428414941,89.2812499996533,3.2659117547607));
#289579=CARTESIAN_POINT('Ctrl Pts',(10.0514428414941,89.4312499996527,-1.23094673026484E-15));
#289580=CARTESIAN_POINT('Ctrl Pts',(10.0514428414941,89.5812499996521,-3.26591175476071));
#289581=CARTESIAN_POINT('Ctrl Pts',(8.13178807675713,89.7312499996515,-5.90808986649102));
#289582=CARTESIAN_POINT('Ctrl Pts',(6.21213331202015,89.8812499996509,-8.55026797822134));
#289583=CARTESIAN_POINT('Ctrl Pts',(3.10606665601004,90.0312499996504,-9.5594902125713));
#289584=CARTESIAN_POINT('Ctrl Pts',(-6.50604309973852E-14,90.1812499996498,
-10.5687124469213));
#289585=CARTESIAN_POINT('Ctrl Pts',(-3.10606665601017,90.3312499996491,
-9.5594902125713));
#289586=CARTESIAN_POINT('Ctrl Pts',(-6.21213331202028,90.4812499996485,
-8.55026797822134));
#289587=CARTESIAN_POINT('Ctrl Pts',(-8.13178807675726,90.631249999648,-5.90808986649102));
#289588=CARTESIAN_POINT('Ctrl Pts',(-10.0514428414942,90.7812499996473,
-3.2659117547607));
#289589=CARTESIAN_POINT('Ctrl Pts',(-10.0514428414942,90.9312499996468,
2.46189346052968E-15));
#289590=CARTESIAN_POINT('Ctrl Pts',(-10.0514428414942,91.0812499996461,
3.26591175476071));
#289591=CARTESIAN_POINT('Ctrl Pts',(-8.13178807675726,91.2312499996455,
5.90808986649102));
#289592=CARTESIAN_POINT('Ctrl Pts',(-6.21213331202028,91.381249999645,8.55026797822134));
#289593=CARTESIAN_POINT('Ctrl Pts',(-3.10606665601017,91.5312499996443,
9.5594902125713));
#289594=CARTESIAN_POINT('Ctrl Pts',(-6.333569765937E-14,91.6812499996438,
10.5687124469213));
#289595=CARTESIAN_POINT('Ctrl Pts',(3.10606665601004,91.8312499996431,9.5594902125713));
#289596=CARTESIAN_POINT('Ctrl Pts',(6.21213331202015,91.9812499996426,8.55026797822134));
#289597=CARTESIAN_POINT('Ctrl Pts',(8.13178807675712,92.131249999642,5.90808986649102));
#289598=CARTESIAN_POINT('Ctrl Pts',(10.0514428414941,92.2812499996414,3.2659117547607));
#289599=CARTESIAN_POINT('Ctrl Pts',(10.0514428414941,92.4312499996408,-1.23094673026484E-15));
#289600=CARTESIAN_POINT('Ctrl Pts',(10.0514428414941,92.5812499996402,-3.26591175476071));
#289601=CARTESIAN_POINT('Ctrl Pts',(8.13178807675712,92.7312499996396,-5.90808986649102));
#289602=CARTESIAN_POINT('Ctrl Pts',(6.21213331202015,92.8812499996389,-8.55026797822134));
#289603=CARTESIAN_POINT('Ctrl Pts',(3.10606665601004,93.0312499996383,-9.5594902125713));
#289604=CARTESIAN_POINT('Ctrl Pts',(-6.67881402690471E-14,93.1812499996377,
-10.5687124469213));
#289605=CARTESIAN_POINT('Ctrl Pts',(-3.10606665601018,93.3312499996371,
-9.5594902125713));
#289606=CARTESIAN_POINT('Ctrl Pts',(-6.21213331202028,93.4812499996365,
-8.55026797822134));
#289607=CARTESIAN_POINT('Ctrl Pts',(-8.13178807675726,93.6312499996359,
-5.90808986649102));
#289608=CARTESIAN_POINT('Ctrl Pts',(-10.0514428414942,93.7812499996353,
-3.2659117547607));
#289609=CARTESIAN_POINT('Ctrl Pts',(-10.0514428414942,93.9312499996347,
2.46189346052968E-15));
#289610=CARTESIAN_POINT('Ctrl Pts',(-10.0514428414942,94.0812499996341,
3.26591175476071));
#289611=CARTESIAN_POINT('Ctrl Pts',(-8.13178807675726,94.2312499996335,
5.90808986649102));
#289612=CARTESIAN_POINT('Ctrl Pts',(-6.21213331202028,94.381249999633,8.55026797822134));
#289613=CARTESIAN_POINT('Ctrl Pts',(-3.10606665601017,94.5312499996324,
9.5594902125713));
#289614=CARTESIAN_POINT('Ctrl Pts',(-6.50634069310318E-14,94.6812499996317,
10.5687124469213));
#289615=CARTESIAN_POINT('Ctrl Pts',(3.10606665601004,94.8312499996312,9.5594902125713));
#289616=CARTESIAN_POINT('Ctrl Pts',(6.21213331202015,94.9812499996306,8.55026797822134));
#289617=CARTESIAN_POINT('Ctrl Pts',(8.13178807675712,95.13124999963,5.90808986649102));
#289618=CARTESIAN_POINT('Ctrl Pts',(10.0514428414941,95.2812499996293,3.2659117547607));
#289619=CARTESIAN_POINT('Ctrl Pts',(10.0514428414941,95.4312499996288,-1.23094673026484E-15));
#289620=CARTESIAN_POINT('Ctrl Pts',(10.0514428414941,95.5812499996282,-3.26591175476071));
#289621=CARTESIAN_POINT('Ctrl Pts',(8.13178807675712,95.7312499996276,-5.90808986649102));
#289622=CARTESIAN_POINT('Ctrl Pts',(6.21213331202015,95.8812499996269,-8.55026797822134));
#289623=CARTESIAN_POINT('Ctrl Pts',(3.10606665601004,96.0312499996264,-9.5594902125713));
#289624=CARTESIAN_POINT('Ctrl Pts',(-6.85158495407089E-14,96.1812499996257,
-10.5687124469213));
#289625=CARTESIAN_POINT('Ctrl Pts',(-3.10606665601018,96.3312499996252,
-9.5594902125713));
#289626=CARTESIAN_POINT('Ctrl Pts',(-6.21213331202028,96.4812499996245,
-8.55026797822134));
#289627=CARTESIAN_POINT('Ctrl Pts',(-8.13178807675726,96.6312499996239,
-5.90808986649102));
#289628=CARTESIAN_POINT('Ctrl Pts',(-10.0514428414942,96.7812499996234,
-3.2659117547607));
#289629=CARTESIAN_POINT('Ctrl Pts',(-10.0514428414942,96.9312499996227,
2.46189346052968E-15));
#289630=CARTESIAN_POINT('Ctrl Pts',(-10.0514428414942,97.0812499996221,
3.26591175476071));
#289631=CARTESIAN_POINT('Ctrl Pts',(-8.13178807675726,97.2312499996215,
5.90808986649102));
#289632=CARTESIAN_POINT('Ctrl Pts',(-6.21213331202028,97.381249999621,8.55026797822134));
#289633=CARTESIAN_POINT('Ctrl Pts',(-3.10606665601017,97.5312499996203,
9.5594902125713));
#289634=CARTESIAN_POINT('Ctrl Pts',(-6.67911162026936E-14,97.6812499996197,
10.5687124469213));
#289635=CARTESIAN_POINT('Ctrl Pts',(3.10606665601004,97.8312499996191,9.5594902125713));
#289636=CARTESIAN_POINT('Ctrl Pts',(6.21213331202015,97.9812499996186,8.55026797822134));
#289637=CARTESIAN_POINT('Ctrl Pts',(8.13178807675712,98.1312499996179,5.90808986649102));
#289638=CARTESIAN_POINT('Ctrl Pts',(10.0514428414941,98.2812499996173,3.2659117547607));
#289639=CARTESIAN_POINT('Ctrl Pts',(10.0514428414941,98.4312499996168,-1.23094673026484E-15));
#289640=CARTESIAN_POINT('Ctrl Pts',(10.0514428414941,98.5812499996162,-3.26591175476071));
#289641=CARTESIAN_POINT('Ctrl Pts',(8.13178807675712,98.7312499996156,-5.90808986649102));
#289642=CARTESIAN_POINT('Ctrl Pts',(6.21213331202015,98.8812499996149,-8.55026797822134));
#289643=CARTESIAN_POINT('Ctrl Pts',(3.10606665601004,99.0312499996143,-9.5594902125713));
#289644=CARTESIAN_POINT('Ctrl Pts',(-7.02435588123707E-14,99.1812499996138,
-10.5687124469213));
#289645=CARTESIAN_POINT('Ctrl Pts',(-3.10606665601018,99.3312499996131,
-9.5594902125713));
#289646=CARTESIAN_POINT('Ctrl Pts',(-6.21213331202028,99.4812499996125,
-8.55026797822134));
#289647=CARTESIAN_POINT('Ctrl Pts',(-8.13178807675726,99.631249999612,-5.90808986649102));
#289648=CARTESIAN_POINT('Ctrl Pts',(-10.0514428414942,99.7812499996113,
-3.2659117547607));
#289649=CARTESIAN_POINT('Ctrl Pts',(-10.0514428414942,99.9312499996108,
2.46189346052968E-15));
#289650=CARTESIAN_POINT('Ctrl Pts',(-10.0514428414942,100.08124999961,3.26591175476071));
#289651=CARTESIAN_POINT('Ctrl Pts',(-8.13178807675726,100.23124999961,5.90808986649102));
#289652=CARTESIAN_POINT('Ctrl Pts',(-6.21213331202028,100.381249999609,
8.55026797822134));
#289653=CARTESIAN_POINT('Ctrl Pts',(-3.10606665601018,100.531249999608,
9.5594902125713));
#289654=CARTESIAN_POINT('Ctrl Pts',(-6.85188254743555E-14,100.681249999608,
10.5687124469213));
#289655=CARTESIAN_POINT('Ctrl Pts',(3.10606665601004,100.831249999607,9.5594902125713));
#289656=CARTESIAN_POINT('Ctrl Pts',(6.21213331202015,100.981249999607,8.55026797822134));
#289657=CARTESIAN_POINT('Ctrl Pts',(8.13178807675712,101.131249999606,5.90808986649102));
#289658=CARTESIAN_POINT('Ctrl Pts',(10.0514428414941,101.281249999605,3.2659117547607));
#289659=CARTESIAN_POINT('Ctrl Pts',(10.0514428414941,101.431249999605,-1.23094673026484E-15));
#289660=CARTESIAN_POINT('Ctrl Pts',(10.0514428414941,101.581249999604,-3.26591175476071));
#289661=CARTESIAN_POINT('Ctrl Pts',(8.13178807675712,101.731249999604,-5.90808986649102));
#289662=CARTESIAN_POINT('Ctrl Pts',(6.21213331202014,101.881249999603,-8.55026797822134));
#289663=CARTESIAN_POINT('Ctrl Pts',(3.10606665601004,102.031249999602,-9.5594902125713));
#289664=CARTESIAN_POINT('Ctrl Pts',(-7.19712680840326E-14,102.181249999602,
-10.5687124469213));
#289665=CARTESIAN_POINT('Ctrl Pts',(-3.10606665601018,102.331249999601,
-9.5594902125713));
#289666=CARTESIAN_POINT('Ctrl Pts',(-6.21213331202029,102.481249999601,
-8.55026797822134));
#289667=CARTESIAN_POINT('Ctrl Pts',(-8.13178807675726,102.6312499996,-5.90808986649102));
#289668=CARTESIAN_POINT('Ctrl Pts',(-10.0514428414942,102.781249999599,
-3.2659117547607));
#289669=CARTESIAN_POINT('Ctrl Pts',(-10.0514428414942,102.931249999599,
2.46189346052968E-15));
#289670=CARTESIAN_POINT('Ctrl Pts',(-10.0514428414942,103.081249999598,
3.26591175476071));
#289671=CARTESIAN_POINT('Ctrl Pts',(-8.13178807675726,103.231249999598,
5.90808986649102));
#289672=CARTESIAN_POINT('Ctrl Pts',(-6.21213331202028,103.381249999597,
8.55026797822134));
#289673=CARTESIAN_POINT('Ctrl Pts',(-3.10606665601018,103.531249999596,
9.5594902125713));
#289674=CARTESIAN_POINT('Ctrl Pts',(-7.02465347460173E-14,103.681249999596,
10.5687124469213));
#289675=CARTESIAN_POINT('Ctrl Pts',(3.10606665601004,103.831249999595,9.5594902125713));
#289676=CARTESIAN_POINT('Ctrl Pts',(6.21213331202015,103.981249999595,8.55026797822134));
#289677=CARTESIAN_POINT('Ctrl Pts',(8.13178807675712,104.131249999594,5.90808986649102));
#289678=CARTESIAN_POINT('Ctrl Pts',(10.0514428414941,104.281249999593,3.2659117547607));
#289679=CARTESIAN_POINT('Ctrl Pts',(10.0514428414941,104.431249999593,-1.23094673026484E-15));
#289680=CARTESIAN_POINT('Ctrl Pts',(10.0514428414941,104.581249999592,-3.26591175476071));
#289681=CARTESIAN_POINT('Ctrl Pts',(8.13178807675712,104.731249999592,-5.90808986649102));
#289682=CARTESIAN_POINT('Ctrl Pts',(6.21213331202014,104.881249999591,-8.55026797822134));
#289683=CARTESIAN_POINT('Ctrl Pts',(3.10606665601003,105.03124999959,-9.5594902125713));
#289684=CARTESIAN_POINT('Ctrl Pts',(-7.36989773556944E-14,105.18124999959,
-10.5687124469213));
#289685=CARTESIAN_POINT('Ctrl Pts',(-3.10606665601018,105.331249999589,
-9.5594902125713));
#289686=CARTESIAN_POINT('Ctrl Pts',(-6.21213331202029,105.481249999589,
-8.55026797822134));
#289687=CARTESIAN_POINT('Ctrl Pts',(-8.13178807675726,105.631249999588,
-5.90808986649102));
#289688=CARTESIAN_POINT('Ctrl Pts',(-10.0514428414942,105.781249999587,
-3.2659117547607));
#289689=CARTESIAN_POINT('Ctrl Pts',(-10.0514428414942,105.931249999587,
2.46189346052968E-15));
#289690=CARTESIAN_POINT('Ctrl Pts',(-10.0514428414942,106.081249999586,
3.26591175476071));
#289691=CARTESIAN_POINT('Ctrl Pts',(-8.13178807675726,106.231249999586,
5.90808986649102));
#289692=CARTESIAN_POINT('Ctrl Pts',(-6.21213331202029,106.381249999585,
8.55026797822134));
#289693=CARTESIAN_POINT('Ctrl Pts',(-3.10606665601018,106.531249999584,
9.5594902125713));
#289694=CARTESIAN_POINT('Ctrl Pts',(-7.19742440176792E-14,106.681249999584,
10.5687124469213));
#289695=CARTESIAN_POINT('Ctrl Pts',(3.10606665601004,106.831249999583,9.5594902125713));
#289696=CARTESIAN_POINT('Ctrl Pts',(6.21213331202014,106.981249999583,8.55026797822134));
#289697=CARTESIAN_POINT('Ctrl Pts',(8.13178807675711,107.131249999582,5.90808986649102));
#289698=CARTESIAN_POINT('Ctrl Pts',(10.0514428414941,107.281249999581,3.2659117547607));
#289699=CARTESIAN_POINT('Ctrl Pts',(10.0514428414941,107.431249999581,-1.23094673026484E-15));
#289700=CARTESIAN_POINT('Ctrl Pts',(10.0514428414941,107.58124999958,-3.26591175476071));
#289701=CARTESIAN_POINT('Ctrl Pts',(8.13178807675711,107.73124999958,-5.90808986649102));
#289702=CARTESIAN_POINT('Ctrl Pts',(6.21213331202014,107.881249999579,-8.55026797822134));
#289703=CARTESIAN_POINT('Ctrl Pts',(3.10606665601003,108.031249999578,-9.5594902125713));
#289704=CARTESIAN_POINT('Ctrl Pts',(-7.54266866273562E-14,108.181249999578,
-10.5687124469213));
#289705=CARTESIAN_POINT('Ctrl Pts',(-3.10606665601018,108.331249999577,
-9.5594902125713));
#289706=CARTESIAN_POINT('Ctrl Pts',(-6.21213331202029,108.481249999577,
-8.55026797822134));
#289707=CARTESIAN_POINT('Ctrl Pts',(-8.13178807675727,108.631249999576,
-5.90808986649102));
#289708=CARTESIAN_POINT('Ctrl Pts',(-10.0514428414942,108.781249999575,
-3.2659117547607));
#289709=CARTESIAN_POINT('Ctrl Pts',(-10.0514428414942,108.931249999575,
2.46189346052968E-15));
#289710=CARTESIAN_POINT('Ctrl Pts',(-10.0514428414942,109.081249999574,
3.26591175476071));
#289711=CARTESIAN_POINT('Ctrl Pts',(-8.13178807675727,109.231249999574,
5.90808986649102));
#289712=CARTESIAN_POINT('Ctrl Pts',(-6.21213331202029,109.381249999573,
8.55026797822134));
#289713=CARTESIAN_POINT('Ctrl Pts',(-3.10606665601018,109.531249999572,
9.5594902125713));
#289714=CARTESIAN_POINT('Ctrl Pts',(-7.3701953289341E-14,109.681249999572,
10.5687124469213));
#289715=CARTESIAN_POINT('Ctrl Pts',(3.10606665601003,109.831249999571,9.5594902125713));
#289716=CARTESIAN_POINT('Ctrl Pts',(6.21213331202014,109.981249999571,8.55026797822134));
#289717=CARTESIAN_POINT('Ctrl Pts',(8.13178807675711,110.13124999957,5.90808986649102));
#289718=CARTESIAN_POINT('Ctrl Pts',(10.0514428414941,110.281249999569,3.2659117547607));
#289719=CARTESIAN_POINT('Ctrl Pts',(10.0514428414941,110.431249999569,-1.23094673026484E-15));
#289720=CARTESIAN_POINT('Ctrl Pts',(10.0514428414941,110.581249999568,-3.26591175476071));
#289721=CARTESIAN_POINT('Ctrl Pts',(8.13178807675711,110.731249999568,-5.90808986649102));
#289722=CARTESIAN_POINT('Ctrl Pts',(6.21213331202014,110.881249999567,-8.55026797822134));
#289723=CARTESIAN_POINT('Ctrl Pts',(3.10606665601003,111.031249999566,-9.5594902125713));
#289724=CARTESIAN_POINT('Ctrl Pts',(-7.71543958990181E-14,111.181249999566,
-10.5687124469213));
#289725=CARTESIAN_POINT('Ctrl Pts',(-3.10606665601019,111.331249999565,
-9.5594902125713));
#289726=CARTESIAN_POINT('Ctrl Pts',(-6.21213331202029,111.481249999565,
-8.55026797822134));
#289727=CARTESIAN_POINT('Ctrl Pts',(-8.13178807675727,111.631249999564,
-5.90808986649102));
#289728=CARTESIAN_POINT('Ctrl Pts',(-10.0514428414942,111.781249999563,
-3.2659117547607));
#289729=CARTESIAN_POINT('Ctrl Pts',(-10.0514428414942,111.931249999563,
2.46189346052968E-15));
#289730=CARTESIAN_POINT('Ctrl Pts',(-10.0514428414942,112.081249999562,
3.26591175476071));
#289731=CARTESIAN_POINT('Ctrl Pts',(-8.13178807675727,112.231249999562,
5.90808986649102));
#289732=CARTESIAN_POINT('Ctrl Pts',(-6.21213331202029,112.381249999561,
8.55026797822134));
#289733=CARTESIAN_POINT('Ctrl Pts',(-3.10606665601018,112.53124999956,9.5594902125713));
#289734=CARTESIAN_POINT('Ctrl Pts',(-7.54296625610028E-14,112.68124999956,
10.5687124469213));
#289735=CARTESIAN_POINT('Ctrl Pts',(3.10606665601003,112.831249999559,9.5594902125713));
#289736=CARTESIAN_POINT('Ctrl Pts',(6.21213331202014,112.981249999559,8.55026797822134));
#289737=CARTESIAN_POINT('Ctrl Pts',(8.13178807675711,113.131249999558,5.90808986649102));
#289738=CARTESIAN_POINT('Ctrl Pts',(10.0514428414941,113.281249999557,3.2659117547607));
#289739=CARTESIAN_POINT('Ctrl Pts',(10.0514428414941,113.431249999557,-1.23094673026484E-15));
#289740=CARTESIAN_POINT('Ctrl Pts',(10.0514428414941,113.581249999556,-3.26591175476071));
#289741=CARTESIAN_POINT('Ctrl Pts',(8.13178807675711,113.731249999556,-5.90808986649102));
#289742=CARTESIAN_POINT('Ctrl Pts',(6.21213331202014,113.881249999555,-8.55026797822134));
#289743=CARTESIAN_POINT('Ctrl Pts',(3.10606665601003,114.031249999554,-9.5594902125713));
#289744=CARTESIAN_POINT('Ctrl Pts',(-7.88821051706799E-14,114.181249999554,
-10.5687124469213));
#289745=CARTESIAN_POINT('Ctrl Pts',(-3.10606665601019,114.331249999553,
-9.5594902125713));
#289746=CARTESIAN_POINT('Ctrl Pts',(-6.2121333120203,114.481249999553,-8.55026797822134));
#289747=CARTESIAN_POINT('Ctrl Pts',(-8.13178807675727,114.631249999552,
-5.90808986649102));
#289748=CARTESIAN_POINT('Ctrl Pts',(-10.0514428414942,114.781249999551,
-3.2659117547607));
#289749=CARTESIAN_POINT('Ctrl Pts',(-10.0514428414942,114.931249999551,
2.46189346052968E-15));
#289750=CARTESIAN_POINT('Ctrl Pts',(-10.0514428414942,115.08124999955,3.26591175476071));
#289751=CARTESIAN_POINT('Ctrl Pts',(-8.13178807675727,115.23124999955,5.90808986649102));
#289752=CARTESIAN_POINT('Ctrl Pts',(-6.21213331202029,115.381249999549,
8.55026797822134));
#289753=CARTESIAN_POINT('Ctrl Pts',(-3.10606665601018,115.531249999548,
9.5594902125713));
#289754=CARTESIAN_POINT('Ctrl Pts',(-7.71573718326647E-14,115.681249999548,
10.5687124469213));
#289755=CARTESIAN_POINT('Ctrl Pts',(3.10606665601003,115.831249999547,9.5594902125713));
#289756=CARTESIAN_POINT('Ctrl Pts',(6.21213331202014,115.981249999547,8.55026797822134));
#289757=CARTESIAN_POINT('Ctrl Pts',(8.13178807675711,116.131249999546,5.90808986649102));
#289758=CARTESIAN_POINT('Ctrl Pts',(10.0514428414941,116.281249999545,3.2659117547607));
#289759=CARTESIAN_POINT('Ctrl Pts',(10.0514428414941,116.431249999545,-1.23094673026484E-15));
#289760=CARTESIAN_POINT('Ctrl Pts',(10.0514428414941,116.581249999544,-3.26591175476071));
#289761=CARTESIAN_POINT('Ctrl Pts',(8.13178807675711,116.731249999544,-5.90808986649102));
#289762=CARTESIAN_POINT('Ctrl Pts',(6.21213331202014,116.881249999543,-8.55026797822134));
#289763=CARTESIAN_POINT('Ctrl Pts',(3.10606665601003,117.031249999542,-9.5594902125713));
#289764=CARTESIAN_POINT('Ctrl Pts',(-8.06098144423418E-14,117.181249999542,
-10.5687124469213));
#289765=CARTESIAN_POINT('Ctrl Pts',(-3.10606665601019,117.331249999541,
-9.5594902125713));
#289766=CARTESIAN_POINT('Ctrl Pts',(-6.2121333120203,117.481249999541,-8.55026797822134));
#289767=CARTESIAN_POINT('Ctrl Pts',(-8.13178807675727,117.63124999954,-5.90808986649102));
#289768=CARTESIAN_POINT('Ctrl Pts',(-10.0514428414942,117.781249999539,
-3.2659117547607));
#289769=CARTESIAN_POINT('Ctrl Pts',(-10.0514428414942,117.931249999539,
2.46189346052968E-15));
#289770=CARTESIAN_POINT('Ctrl Pts',(-10.0514428414942,118.081249999538,
3.26591175476071));
#289771=CARTESIAN_POINT('Ctrl Pts',(-8.13178807675727,118.231249999538,
5.90808986649102));
#289772=CARTESIAN_POINT('Ctrl Pts',(-6.2121333120203,118.381249999537,8.55026797822134));
#289773=CARTESIAN_POINT('Ctrl Pts',(-3.10606665601019,118.531249999536,
9.5594902125713));
#289774=CARTESIAN_POINT('Ctrl Pts',(-7.88850811043265E-14,118.681249999536,
10.5687124469213));
#289775=CARTESIAN_POINT('Ctrl Pts',(3.10606665601003,118.831249999535,9.5594902125713));
#289776=CARTESIAN_POINT('Ctrl Pts',(6.21213331202014,118.981249999535,8.55026797822134));
#289777=CARTESIAN_POINT('Ctrl Pts',(8.13178807675711,119.131249999534,5.90808986649102));
#289778=CARTESIAN_POINT('Ctrl Pts',(10.0514428414941,119.281249999533,3.2659117547607));
#289779=CARTESIAN_POINT('Ctrl Pts',(10.0514428414941,119.431249999533,-1.23094673026484E-15));
#289780=CARTESIAN_POINT('Ctrl Pts',(10.0514428414941,119.581249999532,-3.26591175476071));
#289781=CARTESIAN_POINT('Ctrl Pts',(8.13178807675711,119.731249999532,-5.90808986649102));
#289782=CARTESIAN_POINT('Ctrl Pts',(6.21213331202013,119.881249999531,-8.55026797822134));
#289783=CARTESIAN_POINT('Ctrl Pts',(3.10606665601003,120.03124999953,-9.5594902125713));
#289784=CARTESIAN_POINT('Ctrl Pts',(-8.23375237140036E-14,120.18124999953,
-10.5687124469213));
#289785=CARTESIAN_POINT('Ctrl Pts',(-3.10606665601019,120.331249999529,
-9.5594902125713));
#289786=CARTESIAN_POINT('Ctrl Pts',(-6.2121333120203,120.481249999529,-8.55026797822134));
#289787=CARTESIAN_POINT('Ctrl Pts',(-8.13178807675727,120.631249999528,
-5.90808986649102));
#289788=CARTESIAN_POINT('Ctrl Pts',(-10.0514428414943,120.781249999527,
-3.2659117547607));
#289789=CARTESIAN_POINT('Ctrl Pts',(-10.0514428414943,120.931249999527,
2.46189346052968E-15));
#289790=CARTESIAN_POINT('Ctrl Pts',(-10.0514428414943,121.081249999526,
3.26591175476071));
#289791=CARTESIAN_POINT('Ctrl Pts',(-8.13178807675727,121.231249999526,
5.90808986649102));
#289792=CARTESIAN_POINT('Ctrl Pts',(-6.2121333120203,121.381249999525,8.55026797822134));
#289793=CARTESIAN_POINT('Ctrl Pts',(-3.10606665601019,121.531249999524,
9.5594902125713));
#289794=CARTESIAN_POINT('Ctrl Pts',(-8.06127903759884E-14,121.681249999524,
10.5687124469213));
#289795=CARTESIAN_POINT('Ctrl Pts',(3.10606665601003,121.831249999523,9.5594902125713));
#289796=CARTESIAN_POINT('Ctrl Pts',(6.21213331202014,121.981249999523,8.55026797822134));
#289797=CARTESIAN_POINT('Ctrl Pts',(8.13178807675711,122.131249999522,5.90808986649102));
#289798=CARTESIAN_POINT('Ctrl Pts',(10.0514428414941,122.281249999521,3.2659117547607));
#289799=CARTESIAN_POINT('Ctrl Pts',(10.0514428414941,122.431249999521,-1.23094673026484E-15));
#289800=CARTESIAN_POINT('Ctrl Pts',(10.0514428414941,122.58124999952,-3.26591175476071));
#289801=CARTESIAN_POINT('Ctrl Pts',(8.13178807675711,122.73124999952,-5.90808986649102));
#289802=CARTESIAN_POINT('Ctrl Pts',(6.21213331202013,122.881249999519,-8.55026797822134));
#289803=CARTESIAN_POINT('Ctrl Pts',(3.10606665601002,123.031249999518,-9.5594902125713));
#289804=CARTESIAN_POINT('Ctrl Pts',(-8.40652329856655E-14,123.181249999518,
-10.5687124469213));
#289805=CARTESIAN_POINT('Ctrl Pts',(-3.10606665601019,123.331249999517,
-9.5594902125713));
#289806=CARTESIAN_POINT('Ctrl Pts',(-6.2121333120203,123.481249999517,-8.55026797822134));
#289807=CARTESIAN_POINT('Ctrl Pts',(-8.13178807675727,123.631249999516,
-5.90808986649102));
#289808=CARTESIAN_POINT('Ctrl Pts',(-10.0514428414943,123.781249999515,
-3.2659117547607));
#289809=CARTESIAN_POINT('Ctrl Pts',(-10.0514428414943,123.931249999515,
2.46189346052968E-15));
#289810=CARTESIAN_POINT('Ctrl Pts',(-10.0514428414943,124.081249999514,
3.26591175476071));
#289811=CARTESIAN_POINT('Ctrl Pts',(-8.13178807675727,124.231249999514,
5.90808986649102));
#289812=CARTESIAN_POINT('Ctrl Pts',(-6.2121333120203,124.381249999513,8.55026797822134));
#289813=CARTESIAN_POINT('Ctrl Pts',(-3.10606665601019,124.531249999512,
9.5594902125713));
#289814=CARTESIAN_POINT('Ctrl Pts',(-8.23404996476502E-14,124.681249999512,
10.5687124469213));
#289815=CARTESIAN_POINT('Ctrl Pts',(3.10606665601002,124.831249999511,9.5594902125713));
#289816=CARTESIAN_POINT('Ctrl Pts',(6.21213331202013,124.981249999511,8.55026797822134));
#289817=CARTESIAN_POINT('Ctrl Pts',(8.13178807675711,125.13124999951,5.90808986649102));
#289818=CARTESIAN_POINT('Ctrl Pts',(10.0514428414941,125.281249999509,3.2659117547607));
#289819=CARTESIAN_POINT('Ctrl Pts',(10.0514428414941,125.431249999509,-1.23094673026484E-15));
#289820=CARTESIAN_POINT('Ctrl Pts',(10.0514428414941,125.581249999508,-3.26591175476071));
#289821=CARTESIAN_POINT('Ctrl Pts',(8.13178807675711,125.731249999508,-5.90808986649102));
#289822=CARTESIAN_POINT('Ctrl Pts',(6.21213331202013,125.881249999507,-8.55026797822134));
#289823=CARTESIAN_POINT('Ctrl Pts',(3.10606665601002,126.031249999506,-9.5594902125713));
#289824=CARTESIAN_POINT('Ctrl Pts',(-8.57929422573273E-14,126.181249999506,
-10.5687124469213));
#289825=CARTESIAN_POINT('Ctrl Pts',(-3.10606665601019,126.331249999505,
-9.5594902125713));
#289826=CARTESIAN_POINT('Ctrl Pts',(-6.2121333120203,126.481249999505,-8.55026797822134));
#289827=CARTESIAN_POINT('Ctrl Pts',(-8.13178807675728,126.631249999504,
-5.90808986649102));
#289828=CARTESIAN_POINT('Ctrl Pts',(-10.0514428414943,126.781249999503,
-3.2659117547607));
#289829=CARTESIAN_POINT('Ctrl Pts',(-10.0514428414943,126.931249999503,
2.46189346052968E-15));
#289830=CARTESIAN_POINT('Ctrl Pts',(-10.0514428414943,127.081249999502,
3.26591175476071));
#289831=CARTESIAN_POINT('Ctrl Pts',(-8.13178807675728,127.231249999502,
5.90808986649102));
#289832=CARTESIAN_POINT('Ctrl Pts',(-6.2121333120203,127.381249999501,8.55026797822134));
#289833=CARTESIAN_POINT('Ctrl Pts',(-3.10606665601019,127.5312499995,9.5594902125713));
#289834=CARTESIAN_POINT('Ctrl Pts',(-8.4068208919312E-14,127.6812499995,
10.5687124469213));
#289835=CARTESIAN_POINT('Ctrl Pts',(3.10606665601002,127.831249999499,9.5594902125713));
#289836=CARTESIAN_POINT('Ctrl Pts',(6.21213331202013,127.981249999499,8.55026797822134));
#289837=CARTESIAN_POINT('Ctrl Pts',(8.1317880767571,128.131249999498,5.90808986649102));
#289838=CARTESIAN_POINT('Ctrl Pts',(10.0514428414941,128.281249999497,3.2659117547607));
#289839=CARTESIAN_POINT('Ctrl Pts',(10.0514428414941,128.431249999497,-1.23094673026484E-15));
#289840=CARTESIAN_POINT('Ctrl Pts',(10.0514428414941,128.581249999496,-3.26591175476071));
#289841=CARTESIAN_POINT('Ctrl Pts',(8.1317880767571,128.731249999496,-5.90808986649102));
#289842=CARTESIAN_POINT('Ctrl Pts',(6.21213331202013,128.881249999495,-8.55026797822134));
#289843=CARTESIAN_POINT('Ctrl Pts',(3.10606665601002,129.031249999494,-9.5594902125713));
#289844=CARTESIAN_POINT('Ctrl Pts',(-8.75206515289892E-14,129.181249999494,
-10.5687124469213));
#289845=CARTESIAN_POINT('Ctrl Pts',(-3.1060666560102,129.331249999493,-9.5594902125713));
#289846=CARTESIAN_POINT('Ctrl Pts',(-6.2121333120203,129.481249999493,-8.55026797822134));
#289847=CARTESIAN_POINT('Ctrl Pts',(-8.13178807675728,129.631249999492,
-5.90808986649102));
#289848=CARTESIAN_POINT('Ctrl Pts',(-10.0514428414943,129.781249999491,
-3.2659117547607));
#289849=CARTESIAN_POINT('Ctrl Pts',(-10.0514428414943,129.931249999491,
2.46189346052968E-15));
#289850=CARTESIAN_POINT('Ctrl Pts',(-10.0514428414943,130.08124999949,3.26591175476071));
#289851=CARTESIAN_POINT('Ctrl Pts',(-8.13178807675728,130.23124999949,5.90808986649102));
#289852=CARTESIAN_POINT('Ctrl Pts',(-6.2121333120203,130.381249999489,8.55026797822134));
#289853=CARTESIAN_POINT('Ctrl Pts',(-3.10606665601019,130.531249999488,
9.5594902125713));
#289854=CARTESIAN_POINT('Ctrl Pts',(-8.57959181909739E-14,130.681249999488,
10.5687124469213));
#289855=CARTESIAN_POINT('Ctrl Pts',(3.10606665601002,130.831249999487,9.5594902125713));
#289856=CARTESIAN_POINT('Ctrl Pts',(6.21213331202013,130.981249999487,8.55026797822134));
#289857=CARTESIAN_POINT('Ctrl Pts',(8.1317880767571,131.131249999486,5.90808986649102));
#289858=CARTESIAN_POINT('Ctrl Pts',(10.0514428414941,131.281249999485,3.2659117547607));
#289859=CARTESIAN_POINT('Ctrl Pts',(10.0514428414941,131.431249999485,-1.23094673026484E-15));
#289860=CARTESIAN_POINT('Ctrl Pts',(10.0514428414941,131.581249999484,-3.26591175476071));
#289861=CARTESIAN_POINT('Ctrl Pts',(8.1317880767571,131.731249999484,-5.90808986649102));
#289862=CARTESIAN_POINT('Ctrl Pts',(6.21213331202012,131.881249999483,-8.55026797822134));
#289863=CARTESIAN_POINT('Ctrl Pts',(3.10606665601002,132.031249999482,-9.5594902125713));
#289864=CARTESIAN_POINT('Ctrl Pts',(-8.9248360800651E-14,132.181249999482,
-10.5687124469213));
#289865=CARTESIAN_POINT('Ctrl Pts',(-3.1060666560102,132.331249999481,-9.5594902125713));
#289866=CARTESIAN_POINT('Ctrl Pts',(-6.2121333120203,132.48124999948,-8.55026797822134));
#289867=CARTESIAN_POINT('Ctrl Pts',(-8.13178807675728,132.63124999948,-5.90808986649102));
#289868=CARTESIAN_POINT('Ctrl Pts',(-10.0514428414943,132.781249999479,
-3.2659117547607));
#289869=CARTESIAN_POINT('Ctrl Pts',(-10.0514428414943,132.931249999479,
2.46189346052968E-15));
#289870=CARTESIAN_POINT('Ctrl Pts',(-10.0514428414943,133.081249999478,
3.26591175476071));
#289871=CARTESIAN_POINT('Ctrl Pts',(-8.13178807675728,133.231249999478,
5.90808986649102));
#289872=CARTESIAN_POINT('Ctrl Pts',(-6.2121333120203,133.381249999477,8.55026797822134));
#289873=CARTESIAN_POINT('Ctrl Pts',(-3.1060666560102,133.531249999476,9.5594902125713));
#289874=CARTESIAN_POINT('Ctrl Pts',(-8.75236274626357E-14,133.681249999476,
10.5687124469213));
#289875=CARTESIAN_POINT('Ctrl Pts',(3.10606665601002,133.831249999475,9.5594902125713));
#289876=CARTESIAN_POINT('Ctrl Pts',(6.21213331202013,133.981249999475,8.55026797822134));
#289877=CARTESIAN_POINT('Ctrl Pts',(8.1317880767571,134.131249999474,5.90808986649102));
#289878=CARTESIAN_POINT('Ctrl Pts',(10.0514428414941,134.281249999473,3.2659117547607));
#289879=CARTESIAN_POINT('Ctrl Pts',(10.0514428414941,134.431249999473,-1.23094673026484E-15));
#289880=CARTESIAN_POINT('Ctrl Pts',(10.0514428414941,134.581249999472,-3.26591175476071));
#289881=CARTESIAN_POINT('Ctrl Pts',(8.1317880767571,134.731249999472,-5.90808986649102));
#289882=CARTESIAN_POINT('Ctrl Pts',(6.21213331202012,134.881249999471,-8.55026797822134));
#289883=CARTESIAN_POINT('Ctrl Pts',(3.10606665601002,135.03124999947,-9.5594902125713));
#289884=CARTESIAN_POINT('Ctrl Pts',(-9.09760700723128E-14,135.18124999947,
-10.5687124469213));
#289885=CARTESIAN_POINT('Ctrl Pts',(-3.1060666560102,135.331249999469,-9.5594902125713));
#289886=CARTESIAN_POINT('Ctrl Pts',(-6.21213331202031,135.481249999469,
-8.55026797822134));
#289887=CARTESIAN_POINT('Ctrl Pts',(-8.13178807675728,135.631249999468,
-5.90808986649102));
#289888=CARTESIAN_POINT('Ctrl Pts',(-10.0514428414943,135.781249999467,
-3.2659117547607));
#289889=CARTESIAN_POINT('Ctrl Pts',(-10.0514428414943,135.931249999467,
2.46189346052968E-15));
#289890=CARTESIAN_POINT('Ctrl Pts',(-10.0514428414943,136.081249999466,
3.26591175476071));
#289891=CARTESIAN_POINT('Ctrl Pts',(-8.13178807675728,136.231249999466,
5.90808986649102));
#289892=CARTESIAN_POINT('Ctrl Pts',(-6.2121333120203,136.381249999465,8.55026797822134));
#289893=CARTESIAN_POINT('Ctrl Pts',(-3.1060666560102,136.531249999464,9.5594902125713));
#289894=CARTESIAN_POINT('Ctrl Pts',(-8.92513367342975E-14,136.681249999464,
10.5687124469213));
#289895=CARTESIAN_POINT('Ctrl Pts',(3.10606665601002,136.831249999463,9.5594902125713));
#289896=CARTESIAN_POINT('Ctrl Pts',(6.21213331202012,136.981249999463,8.55026797822134));
#289897=CARTESIAN_POINT('Ctrl Pts',(8.1317880767571,137.131249999462,5.90808986649102));
#289898=CARTESIAN_POINT('Ctrl Pts',(10.0514428414941,137.281249999461,3.2659117547607));
#289899=CARTESIAN_POINT('Ctrl Pts',(10.0514428414941,137.431249999461,-1.23094673026484E-15));
#289900=CARTESIAN_POINT('Ctrl Pts',(10.0514428414941,137.58124999946,-3.26591175476071));
#289901=CARTESIAN_POINT('Ctrl Pts',(8.1317880767571,137.73124999946,-5.90808986649102));
#289902=CARTESIAN_POINT('Ctrl Pts',(6.21213331202012,137.881249999459,-8.55026797822134));
#289903=CARTESIAN_POINT('Ctrl Pts',(3.10606665601002,138.031249999458,-9.5594902125713));
#289904=CARTESIAN_POINT('Ctrl Pts',(-9.27037793439746E-14,138.181249999458,
-10.5687124469213));
#289905=CARTESIAN_POINT('Ctrl Pts',(-3.1060666560102,138.331249999457,-9.5594902125713));
#289906=CARTESIAN_POINT('Ctrl Pts',(-6.21213331202031,138.481249999456,
-8.55026797822134));
#289907=CARTESIAN_POINT('Ctrl Pts',(-8.13178807675728,138.631249999456,
-5.90808986649102));
#289908=CARTESIAN_POINT('Ctrl Pts',(-10.0514428414943,138.781249999455,
-3.2659117547607));
#289909=CARTESIAN_POINT('Ctrl Pts',(-10.0514428414943,138.931249999455,
2.46189346052968E-15));
#289910=CARTESIAN_POINT('Ctrl Pts',(-10.0514428414943,139.081249999454,
3.26591175476071));
#289911=CARTESIAN_POINT('Ctrl Pts',(-8.13178807675728,139.231249999454,
5.90808986649102));
#289912=CARTESIAN_POINT('Ctrl Pts',(-6.21213331202031,139.381249999453,
8.55026797822134));
#289913=CARTESIAN_POINT('Ctrl Pts',(-3.1060666560102,139.531249999452,9.5594902125713));
#289914=CARTESIAN_POINT('Ctrl Pts',(-9.09790460059594E-14,139.681249999452,
10.5687124469213));
#289915=CARTESIAN_POINT('Ctrl Pts',(3.10606665601002,139.831249999451,9.5594902125713));
#289916=CARTESIAN_POINT('Ctrl Pts',(6.21213331202012,139.981249999451,8.55026797822134));
#289917=CARTESIAN_POINT('Ctrl Pts',(8.1317880767571,140.13124999945,5.90808986649102));
#289918=CARTESIAN_POINT('Ctrl Pts',(10.0514428414941,140.281249999449,3.2659117547607));
#289919=CARTESIAN_POINT('Ctrl Pts',(10.0514428414941,140.431249999449,-1.23094673026484E-15));
#289920=CARTESIAN_POINT('Ctrl Pts',(10.0514428414941,140.581249999448,-3.26591175476071));
#289921=CARTESIAN_POINT('Ctrl Pts',(8.1317880767571,140.731249999448,-5.90808986649102));
#289922=CARTESIAN_POINT('Ctrl Pts',(6.21213331202012,140.881249999447,-8.55026797822134));
#289923=CARTESIAN_POINT('Ctrl Pts',(3.10606665601001,141.031249999446,-9.5594902125713));
#289924=CARTESIAN_POINT('Ctrl Pts',(-9.44314886156365E-14,141.181249999446,
-10.5687124469213));
#289925=CARTESIAN_POINT('Ctrl Pts',(-3.1060666560102,141.331249999445,-9.5594902125713));
#289926=CARTESIAN_POINT('Ctrl Pts',(-6.21213331202031,141.481249999445,
-8.55026797822134));
#289927=CARTESIAN_POINT('Ctrl Pts',(-8.13178807675729,141.631249999444,
-5.90808986649102));
#289928=CARTESIAN_POINT('Ctrl Pts',(-10.0514428414943,141.781249999443,
-3.2659117547607));
#289929=CARTESIAN_POINT('Ctrl Pts',(-10.0514428414943,141.931249999443,
2.46189346052968E-15));
#289930=CARTESIAN_POINT('Ctrl Pts',(-10.0514428414943,142.081249999442,
3.26591175476071));
#289931=CARTESIAN_POINT('Ctrl Pts',(-8.13178807675729,142.231249999442,
5.90808986649102));
#289932=CARTESIAN_POINT('Ctrl Pts',(-6.21213331202031,142.381249999441,
8.55026797822134));
#289933=CARTESIAN_POINT('Ctrl Pts',(-3.1060666560102,142.53124999944,9.5594902125713));
#289934=CARTESIAN_POINT('Ctrl Pts',(-9.27067552776212E-14,142.68124999944,
10.5687124469213));
#289935=CARTESIAN_POINT('Ctrl Pts',(3.10606665601001,142.831249999439,9.5594902125713));
#289936=CARTESIAN_POINT('Ctrl Pts',(6.21213331202012,142.981249999439,8.55026797822134));
#289937=CARTESIAN_POINT('Ctrl Pts',(8.1317880767571,143.131249999438,5.90808986649102));
#289938=CARTESIAN_POINT('Ctrl Pts',(10.0514428414941,143.281249999437,3.2659117547607));
#289939=CARTESIAN_POINT('Ctrl Pts',(10.0514428414941,143.431249999437,-1.23094673026484E-15));
#289940=CARTESIAN_POINT('Ctrl Pts',(10.0514428414941,143.581249999436,-3.26591175476071));
#289941=CARTESIAN_POINT('Ctrl Pts',(8.1317880767571,143.731249999436,-5.90808986649102));
#289942=CARTESIAN_POINT('Ctrl Pts',(6.21213331202012,143.881249999435,-8.55026797822134));
#289943=CARTESIAN_POINT('Ctrl Pts',(3.10606665601001,144.031249999434,-9.5594902125713));
#289944=CARTESIAN_POINT('Ctrl Pts',(-9.61591978872984E-14,144.181249999434,
-10.5687124469213));
#289945=CARTESIAN_POINT('Ctrl Pts',(-3.1060666560102,144.331249999433,-9.5594902125713));
#289946=CARTESIAN_POINT('Ctrl Pts',(-6.21213331202031,144.481249999432,
-8.55026797822134));
#289947=CARTESIAN_POINT('Ctrl Pts',(-8.13178807675729,144.631249999432,
-5.90808986649102));
#289948=CARTESIAN_POINT('Ctrl Pts',(-10.0514428414943,144.781249999431,
-3.2659117547607));
#289949=CARTESIAN_POINT('Ctrl Pts',(-10.0514428414943,144.931249999431,
2.46189346052968E-15));
#289950=CARTESIAN_POINT('Ctrl Pts',(-10.0514428414943,145.08124999943,3.26591175476071));
#289951=CARTESIAN_POINT('Ctrl Pts',(-8.13178807675729,145.23124999943,5.90808986649102));
#289952=CARTESIAN_POINT('Ctrl Pts',(-6.21213331202031,145.381249999429,
8.55026797822134));
#289953=CARTESIAN_POINT('Ctrl Pts',(-3.1060666560102,145.531249999428,9.5594902125713));
#289954=CARTESIAN_POINT('Ctrl Pts',(-9.44344645492831E-14,145.681249999428,
10.5687124469213));
#289955=CARTESIAN_POINT('Ctrl Pts',(3.10606665601001,145.831249999427,9.5594902125713));
#289956=CARTESIAN_POINT('Ctrl Pts',(6.21213331202012,145.981249999427,8.55026797822134));
#289957=CARTESIAN_POINT('Ctrl Pts',(8.13178807675709,146.131249999426,5.90808986649102));
#289958=CARTESIAN_POINT('Ctrl Pts',(10.0514428414941,146.281249999425,3.2659117547607));
#289959=CARTESIAN_POINT('Ctrl Pts',(10.0514428414941,146.431249999425,-1.23094673026484E-15));
#289960=CARTESIAN_POINT('Ctrl Pts',(10.0514428414941,146.581249999424,-3.26591175476071));
#289961=CARTESIAN_POINT('Ctrl Pts',(8.13178807675709,146.731249999424,-5.90808986649102));
#289962=CARTESIAN_POINT('Ctrl Pts',(6.21213331202012,146.881249999423,-8.55026797822134));
#289963=CARTESIAN_POINT('Ctrl Pts',(3.10606665601001,147.031249999422,-9.5594902125713));
#289964=CARTESIAN_POINT('Ctrl Pts',(-9.78869071589602E-14,147.181249999422,
-10.5687124469213));
#289965=CARTESIAN_POINT('Ctrl Pts',(-3.10606665601021,147.331249999421,
-9.5594902125713));
#289966=CARTESIAN_POINT('Ctrl Pts',(-6.21213331202032,147.481249999421,
-8.55026797822134));
#289967=CARTESIAN_POINT('Ctrl Pts',(-8.13178807675729,147.63124999942,-5.90808986649102));
#289968=CARTESIAN_POINT('Ctrl Pts',(-10.0514428414943,147.781249999419,
-3.2659117547607));
#289969=CARTESIAN_POINT('Ctrl Pts',(-10.0514428414943,147.931249999419,
2.46189346052968E-15));
#289970=CARTESIAN_POINT('Ctrl Pts',(-10.0514428414943,148.081249999418,
3.26591175476071));
#289971=CARTESIAN_POINT('Ctrl Pts',(-8.13178807675729,148.231249999418,
5.90808986649102));
#289972=CARTESIAN_POINT('Ctrl Pts',(-6.21213331202031,148.381249999417,
8.55026797822134));
#289973=CARTESIAN_POINT('Ctrl Pts',(-3.1060666560102,148.531249999416,9.5594902125713));
#289974=CARTESIAN_POINT('Ctrl Pts',(-9.61621738209449E-14,148.681249999416,
10.5687124469213));
#289975=CARTESIAN_POINT('Ctrl Pts',(3.10606665601001,148.831249999415,9.5594902125713));
#289976=CARTESIAN_POINT('Ctrl Pts',(6.21213331202012,148.981249999415,8.55026797822134));
#289977=CARTESIAN_POINT('Ctrl Pts',(8.13178807675709,149.131249999414,5.90808986649102));
#289978=CARTESIAN_POINT('Ctrl Pts',(10.0514428414941,149.281249999413,3.2659117547607));
#289979=CARTESIAN_POINT('Ctrl Pts',(10.0514428414941,149.431249999413,-1.23094673026484E-15));
#289980=CARTESIAN_POINT('Ctrl Pts',(10.0514428414941,149.581249999412,-3.26591175476071));
#289981=CARTESIAN_POINT('Ctrl Pts',(8.13178807675709,149.731249999412,-5.90808986649102));
#289982=CARTESIAN_POINT('Ctrl Pts',(6.21213331202012,149.881249999411,-8.55026797822134));
#289983=CARTESIAN_POINT('Ctrl Pts',(3.10606665601001,150.03124999941,-9.5594902125713));
#289984=CARTESIAN_POINT('Ctrl Pts',(-9.9614616430622E-14,150.18124999941,
-10.5687124469213));
#289985=CARTESIAN_POINT('Ctrl Pts',(-3.10606665601021,150.331249999409,
-9.5594902125713));
#289986=CARTESIAN_POINT('Ctrl Pts',(-6.21213331202032,150.481249999409,
-8.55026797822134));
#289987=CARTESIAN_POINT('Ctrl Pts',(-8.13178807675729,150.631249999408,
-5.90808986649102));
#289988=CARTESIAN_POINT('Ctrl Pts',(-10.0514428414943,150.781249999407,
-3.2659117547607));
#289989=CARTESIAN_POINT('Ctrl Pts',(-10.0514428414943,150.931249999407,
2.46189346052968E-15));
#289990=CARTESIAN_POINT('Ctrl Pts',(-10.0514428414943,151.081249999406,
3.26591175476071));
#289991=CARTESIAN_POINT('Ctrl Pts',(-8.13178807675729,151.231249999406,
5.90808986649102));
#289992=CARTESIAN_POINT('Ctrl Pts',(-6.21213331202032,151.381249999405,
8.55026797822134));
#289993=CARTESIAN_POINT('Ctrl Pts',(-3.10606665601021,151.531249999404,
9.5594902125713));
#289994=CARTESIAN_POINT('Ctrl Pts',(-9.78898830926068E-14,151.681249999404,
10.5687124469213));
#289995=CARTESIAN_POINT('Ctrl Pts',(3.10606665601001,151.831249999403,9.5594902125713));
#289996=CARTESIAN_POINT('Ctrl Pts',(6.21213331202012,151.981249999403,8.55026797822134));
#289997=CARTESIAN_POINT('Ctrl Pts',(8.13178807675709,152.131249999402,5.90808986649102));
#289998=CARTESIAN_POINT('Ctrl Pts',(10.0514428414941,152.281249999401,3.2659117547607));
#289999=CARTESIAN_POINT('Ctrl Pts',(10.0514428414941,152.431249999401,-1.23094673026484E-15));
#290000=CARTESIAN_POINT('Ctrl Pts',(10.0514428414941,152.5812499994,-3.26591175476071));
#290001=CARTESIAN_POINT('Ctrl Pts',(8.13178807675709,152.7312499994,-5.90808986649102));
#290002=CARTESIAN_POINT('Ctrl Pts',(6.21213331202012,152.881249999399,-8.55026797822134));
#290003=CARTESIAN_POINT('Ctrl Pts',(3.10606665601001,153.031249999398,-9.5594902125713));
#290004=CARTESIAN_POINT('Ctrl Pts',(-1.01342325702284E-13,153.181249999398,
-10.5687124469213));
#290005=CARTESIAN_POINT('Ctrl Pts',(-3.10606665601021,153.331249999397,
-9.5594902125713));
#290006=CARTESIAN_POINT('',(-8.5091557340996,76.2,5.35030577524922));
#290007=CARTESIAN_POINT('Ctrl Pts',(11.7004490057565,76.2,2.66448739229326));
#290008=CARTESIAN_POINT('Ctrl Pts',(11.2736065385016,76.2,4.07643912420469));
#290009=CARTESIAN_POINT('Ctrl Pts',(10.5879289871897,76.2,5.39657685789075));
#290010=CARTESIAN_POINT('Ctrl Pts',(8.52767436642338,76.2,8.0266839054084));
#290011=CARTESIAN_POINT('Ctrl Pts',(7.30982467417011,76.2,8.87851993633569));
#290012=CARTESIAN_POINT('Ctrl Pts',(5.2040775105915,76.2,10.1043730632371));
#290013=CARTESIAN_POINT('Ctrl Pts',(3.83447247941545,76.2,10.5921419577076));
#290014=CARTESIAN_POINT('Ctrl Pts',(1.06742512277072,76.2,11.0007660700567));
#290015=CARTESIAN_POINT('Ctrl Pts',(-0.312663875595359,76.2,10.9428078138237));
#290016=CARTESIAN_POINT('Ctrl Pts',(-2.60282640207458,76.2,10.4049192800778));
#290017=CARTESIAN_POINT('Ctrl Pts',(-4.01317621566336,76.2,9.94321112964606));
#290018=CARTESIAN_POINT('Ctrl Pts',(-6.08753010305324,76.2,8.42910175872524));
#290019=CARTESIAN_POINT('Ctrl Pts',(-6.66541282594047,76.2,7.89712047013574));
#290020=CARTESIAN_POINT('Ctrl Pts',(-7.69093052494506,76.2,6.71162715330518));
#290021=CARTESIAN_POINT('Ctrl Pts',(-8.14368210712128,76.2,6.05166491645592));
#290022=CARTESIAN_POINT('Ctrl Pts',(-8.50915573409961,76.2,5.35030577524915));
#290023=CARTESIAN_POINT('Ctrl Pts',(10.0514428414941,74.4312499997127,-1.23094673026484E-15));
#290024=CARTESIAN_POINT('Ctrl Pts',(10.0514428414941,74.5812499997121,-3.26591175476071));
#290025=CARTESIAN_POINT('Ctrl Pts',(8.13178807675713,74.7312499997116,-5.90808986649102));
#290026=CARTESIAN_POINT('Ctrl Pts',(6.21213331202016,74.8812499997109,-8.55026797822134));
#290027=CARTESIAN_POINT('Ctrl Pts',(3.10606665601005,75.0312499997104,-9.5594902125713));
#290028=CARTESIAN_POINT('Ctrl Pts',(-5.6421884639076E-14,75.1812499997097,
-10.5687124469213));
#290029=CARTESIAN_POINT('Ctrl Pts',(-3.10606665601016,75.3312499997092,
-9.5594902125713));
#290030=CARTESIAN_POINT('Ctrl Pts',(-6.21213331202027,75.4812499997086,
-8.55026797822134));
#290031=CARTESIAN_POINT('Ctrl Pts',(-8.13178807675725,75.6312499997079,
-5.90808986649102));
#290032=CARTESIAN_POINT('Ctrl Pts',(-10.0514428414942,75.7812499997073,
-3.2659117547607));
#290033=CARTESIAN_POINT('Ctrl Pts',(-10.0514428414942,75.9312499997068,
2.46189346052968E-15));
#290034=CARTESIAN_POINT('Ctrl Pts',(-10.0514428414942,76.0643266453995,
2.89744387635823));
#290035=CARTESIAN_POINT('Ctrl Pts',(-8.5091557340996,76.2,5.35030577524922));
#290036=CARTESIAN_POINT('Origin',(-3.77475828372553E-14,-1.881249999982,
2.68644078414671E-15));
#290037=CARTESIAN_POINT('Origin',(-3.77475828372553E-14,76.2,2.03817200954814E-15));
#290038=CARTESIAN_POINT('Origin',(0.,76.2,0.));
#290039=CARTESIAN_POINT('Origin',(-3.77475828372553E-14,-1.881249999982,
2.68644078414671E-15));
#290040=CARTESIAN_POINT('',(10.0514428414942,2.80624999999926,1.43603509362624E-15));
#290041=CARTESIAN_POINT('',(10.0514428414942,2.43125000000076,-1.23094673026484E-15));
#290042=CARTESIAN_POINT('',(10.0514428414941,-1.881249999982,4.14193483802857E-15));
#290043=CARTESIAN_POINT('',(7.09357268597966,2.43124999999995,7.12128708482866));
#290044=CARTESIAN_POINT('Ctrl Pts',(7.09357268597966,2.43124999999995,7.12128708482865));
#290045=CARTESIAN_POINT('Ctrl Pts',(7.66101577103565,2.46946429917804,6.55605235674466));
#290046=CARTESIAN_POINT('Ctrl Pts',(8.13178807675718,2.50625000000046,5.90808986649102));
#290047=CARTESIAN_POINT('Ctrl Pts',(10.0514428414941,2.65624999999986,3.2659117547607));
#290048=CARTESIAN_POINT('Ctrl Pts',(10.0514428414942,2.80624999999926,-1.23094673026484E-15));
#290049=CARTESIAN_POINT('Origin',(-3.77475828372553E-14,2.43125000000001,
2.65063629727636E-15));
#290050=CARTESIAN_POINT('Origin',(-3.77475828372553E-14,-1.881249999982,
2.68644078414671E-15));
#290051=CARTESIAN_POINT('',(10.0514428414941,5.80624999998726,1.42358135906264E-15));
#290052=CARTESIAN_POINT('',(10.0514428414941,5.43124999998876,1.42513807588309E-15));
#290053=CARTESIAN_POINT('',(10.0514428414941,-1.881249999982,4.14193483802857E-15));
#290054=CARTESIAN_POINT('Ctrl Pts',(10.0514428414942,2.80624999999926,-1.23094673026484E-15));
#290055=CARTESIAN_POINT('Ctrl Pts',(10.0514428414941,2.95624999999866,-3.26591175476071));
#290056=CARTESIAN_POINT('Ctrl Pts',(8.13178807675718,3.10624999999806,-5.90808986649102));
#290057=CARTESIAN_POINT('Ctrl Pts',(6.2121333120202,3.25624999999746,-8.55026797822134));
#290058=CARTESIAN_POINT('Ctrl Pts',(3.10606665601009,3.40624999999685,-9.5594902125713));
#290059=CARTESIAN_POINT('Ctrl Pts',(-1.51728257781496E-14,3.55624999999625,
-10.5687124469213));
#290060=CARTESIAN_POINT('Ctrl Pts',(-3.10606665601012,3.70624999999565,
-9.5594902125713));
#290061=CARTESIAN_POINT('Ctrl Pts',(-6.21213331202023,3.85624999999505,
-8.55026797822134));
#290062=CARTESIAN_POINT('Ctrl Pts',(-8.13178807675721,4.00624999999445,
-5.90808986649102));
#290063=CARTESIAN_POINT('Ctrl Pts',(-10.0514428414942,4.15624999999385,
-3.2659117547607));
#290064=CARTESIAN_POINT('Ctrl Pts',(-10.0514428414942,4.30624999999325,
2.46189346052968E-15));
#290065=CARTESIAN_POINT('Ctrl Pts',(-10.0514428414942,4.45624999999265,
3.26591175476071));
#290066=CARTESIAN_POINT('Ctrl Pts',(-8.13178807675721,4.60624999999205,
5.90808986649102));
#290067=CARTESIAN_POINT('Ctrl Pts',(-6.21213331202023,4.75624999999145,
8.55026797822134));
#290068=CARTESIAN_POINT('Ctrl Pts',(-3.10606665601012,4.90624999999085,
9.5594902125713));
#290069=CARTESIAN_POINT('Ctrl Pts',(-1.34480924401344E-14,5.05624999999025,
10.5687124469213));
#290070=CARTESIAN_POINT('Ctrl Pts',(3.10606665601009,5.20624999998966,9.5594902125713));
#290071=CARTESIAN_POINT('Ctrl Pts',(6.2121333120202,5.35624999998906,8.55026797822134));
#290072=CARTESIAN_POINT('Ctrl Pts',(8.13178807675718,5.50624999998846,5.90808986649102));
#290073=CARTESIAN_POINT('Ctrl Pts',(10.0514428414941,5.65624999998786,3.2659117547607));
#290074=CARTESIAN_POINT('Ctrl Pts',(10.0514428414941,5.80624999998726,-1.23094673026484E-15));
#290075=CARTESIAN_POINT('Ctrl Pts',(10.0514428414942,2.43125000000076,-1.23094673026484E-15));
#290076=CARTESIAN_POINT('Ctrl Pts',(10.0514428414941,2.58125000000016,-3.26591175476071));
#290077=CARTESIAN_POINT('Ctrl Pts',(8.13178807675718,2.73124999999956,-5.90808986649102));
#290078=CARTESIAN_POINT('Ctrl Pts',(6.2121333120202,2.88124999999896,-8.55026797822134));
#290079=CARTESIAN_POINT('Ctrl Pts',(3.10606665601009,3.03124999999835,-9.5594902125713));
#290080=CARTESIAN_POINT('Ctrl Pts',(-1.49568621191919E-14,3.18124999999775,
-10.5687124469213));
#290081=CARTESIAN_POINT('Ctrl Pts',(-3.10606665601012,3.33124999999715,
-9.5594902125713));
#290082=CARTESIAN_POINT('Ctrl Pts',(-6.21213331202023,3.48124999999655,
-8.55026797822134));
#290083=CARTESIAN_POINT('Ctrl Pts',(-8.13178807675721,3.63124999999595,
-5.90808986649102));
#290084=CARTESIAN_POINT('Ctrl Pts',(-10.0514428414942,3.78124999999535,
-3.2659117547607));
#290085=CARTESIAN_POINT('Ctrl Pts',(-10.0514428414942,3.93124999999475,
2.46189346052968E-15));
#290086=CARTESIAN_POINT('Ctrl Pts',(-10.0514428414942,4.08124999999415,
3.26591175476071));
#290087=CARTESIAN_POINT('Ctrl Pts',(-8.13178807675721,4.23124999999355,
5.90808986649102));
#290088=CARTESIAN_POINT('Ctrl Pts',(-6.21213331202023,4.38124999999295,
8.55026797822134));
#290089=CARTESIAN_POINT('Ctrl Pts',(-3.10606665601012,4.53124999999235,
9.5594902125713));
#290090=CARTESIAN_POINT('Ctrl Pts',(-1.32321287811766E-14,4.68124999999175,
10.5687124469213));
#290091=CARTESIAN_POINT('Ctrl Pts',(3.10606665601009,4.83124999999115,9.5594902125713));
#290092=CARTESIAN_POINT('Ctrl Pts',(6.2121333120202,4.98124999999056,8.55026797822134));
#290093=CARTESIAN_POINT('Ctrl Pts',(8.13178807675718,5.13124999998996,5.90808986649102));
#290094=CARTESIAN_POINT('Ctrl Pts',(10.0514428414941,5.28124999998936,3.2659117547607));
#290095=CARTESIAN_POINT('Ctrl Pts',(10.0514428414941,5.43124999998876,-1.23094673026484E-15));
#290096=CARTESIAN_POINT('Origin',(-3.77475828372553E-14,-1.881249999982,
2.68644078414671E-15));
#290097=CARTESIAN_POINT('',(10.0514428414941,8.80624999997526,1.41112762449904E-15));
#290098=CARTESIAN_POINT('',(10.0514428414941,8.43124999997676,1.41268434131949E-15));
#290099=CARTESIAN_POINT('',(10.0514428414941,-1.881249999982,4.14193483802857E-15));
#290100=CARTESIAN_POINT('Ctrl Pts',(10.0514428414941,5.80624999998726,-1.23094673026484E-15));
#290101=CARTESIAN_POINT('Ctrl Pts',(10.0514428414941,5.95624999998666,-3.26591175476071));
#290102=CARTESIAN_POINT('Ctrl Pts',(8.13178807675717,6.10624999998606,-5.90808986649102));
#290103=CARTESIAN_POINT('Ctrl Pts',(6.2121333120202,6.25624999998545,-8.55026797822134));
#290104=CARTESIAN_POINT('Ctrl Pts',(3.10606665601009,6.40624999998485,-9.5594902125713));
#290105=CARTESIAN_POINT('Ctrl Pts',(-1.69005350498115E-14,6.55624999998425,
-10.5687124469213));
#290106=CARTESIAN_POINT('Ctrl Pts',(-3.10606665601013,6.70624999998365,
-9.5594902125713));
#290107=CARTESIAN_POINT('Ctrl Pts',(-6.21213331202023,6.85624999998305,
-8.55026797822134));
#290108=CARTESIAN_POINT('Ctrl Pts',(-8.13178807675721,7.00624999998245,
-5.90808986649102));
#290109=CARTESIAN_POINT('Ctrl Pts',(-10.0514428414942,7.15624999998185,
-3.2659117547607));
#290110=CARTESIAN_POINT('Ctrl Pts',(-10.0514428414942,7.30624999998125,
2.46189346052968E-15));
#290111=CARTESIAN_POINT('Ctrl Pts',(-10.0514428414942,7.45624999998065,
3.26591175476071));
#290112=CARTESIAN_POINT('Ctrl Pts',(-8.13178807675721,7.60624999998005,
5.90808986649102));
#290113=CARTESIAN_POINT('Ctrl Pts',(-6.21213331202023,7.75624999997945,
8.55026797822134));
#290114=CARTESIAN_POINT('Ctrl Pts',(-3.10606665601012,7.90624999997885,
9.5594902125713));
#290115=CARTESIAN_POINT('Ctrl Pts',(-1.51758017117962E-14,8.05624999997825,
10.5687124469213));
#290116=CARTESIAN_POINT('Ctrl Pts',(3.10606665601009,8.20624999997765,9.5594902125713));
#290117=CARTESIAN_POINT('Ctrl Pts',(6.2121333120202,8.35624999997706,8.55026797822134));
#290118=CARTESIAN_POINT('Ctrl Pts',(8.13178807675717,8.50624999997646,5.90808986649102));
#290119=CARTESIAN_POINT('Ctrl Pts',(10.0514428414941,8.65624999997586,3.2659117547607));
#290120=CARTESIAN_POINT('Ctrl Pts',(10.0514428414941,8.80624999997526,-1.23094673026484E-15));
#290121=CARTESIAN_POINT('Ctrl Pts',(10.0514428414941,5.43124999998876,-1.23094673026484E-15));
#290122=CARTESIAN_POINT('Ctrl Pts',(10.0514428414941,5.58124999998816,-3.26591175476071));
#290123=CARTESIAN_POINT('Ctrl Pts',(8.13178807675717,5.73124999998756,-5.90808986649102));
#290124=CARTESIAN_POINT('Ctrl Pts',(6.2121333120202,5.88124999998695,-8.55026797822134));
#290125=CARTESIAN_POINT('Ctrl Pts',(3.10606665601009,6.03124999998635,-9.5594902125713));
#290126=CARTESIAN_POINT('Ctrl Pts',(-1.66845713908537E-14,6.18124999998575,
-10.5687124469213));
#290127=CARTESIAN_POINT('Ctrl Pts',(-3.10606665601012,6.33124999998515,
-9.5594902125713));
#290128=CARTESIAN_POINT('Ctrl Pts',(-6.21213331202023,6.48124999998455,
-8.55026797822134));
#290129=CARTESIAN_POINT('Ctrl Pts',(-8.13178807675721,6.63124999998395,
-5.90808986649102));
#290130=CARTESIAN_POINT('Ctrl Pts',(-10.0514428414942,6.78124999998335,
-3.2659117547607));
#290131=CARTESIAN_POINT('Ctrl Pts',(-10.0514428414942,6.93124999998275,
2.46189346052968E-15));
#290132=CARTESIAN_POINT('Ctrl Pts',(-10.0514428414942,7.08124999998215,
3.26591175476071));
#290133=CARTESIAN_POINT('Ctrl Pts',(-8.13178807675721,7.23124999998155,
5.90808986649102));
#290134=CARTESIAN_POINT('Ctrl Pts',(-6.21213331202023,7.38124999998095,
8.55026797822134));
#290135=CARTESIAN_POINT('Ctrl Pts',(-3.10606665601012,7.53124999998035,
9.5594902125713));
#290136=CARTESIAN_POINT('Ctrl Pts',(-1.49598380528385E-14,7.68124999997975,
10.5687124469213));
#290137=CARTESIAN_POINT('Ctrl Pts',(3.10606665601009,7.83124999997915,9.5594902125713));
#290138=CARTESIAN_POINT('Ctrl Pts',(6.2121333120202,7.98124999997856,8.55026797822134));
#290139=CARTESIAN_POINT('Ctrl Pts',(8.13178807675717,8.13124999997796,5.90808986649102));
#290140=CARTESIAN_POINT('Ctrl Pts',(10.0514428414941,8.28124999997736,3.2659117547607));
#290141=CARTESIAN_POINT('Ctrl Pts',(10.0514428414941,8.43124999997676,-1.23094673026484E-15));
#290142=CARTESIAN_POINT('Origin',(-3.77475828372553E-14,-1.881249999982,
2.68644078414671E-15));
#290143=CARTESIAN_POINT('',(10.0514428414941,11.8062499999633,1.39867388993544E-15));
#290144=CARTESIAN_POINT('',(10.0514428414941,11.4312499999648,1.40023060675589E-15));
#290145=CARTESIAN_POINT('',(10.0514428414941,-1.881249999982,4.14193483802857E-15));
#290146=CARTESIAN_POINT('Ctrl Pts',(10.0514428414941,8.80624999997526,-1.23094673026484E-15));
#290147=CARTESIAN_POINT('Ctrl Pts',(10.0514428414941,8.95624999997466,-3.26591175476071));
#290148=CARTESIAN_POINT('Ctrl Pts',(8.13178807675717,9.10624999997406,-5.90808986649102));
#290149=CARTESIAN_POINT('Ctrl Pts',(6.2121333120202,9.25624999997346,-8.55026797822134));
#290150=CARTESIAN_POINT('Ctrl Pts',(3.10606665601009,9.40624999997286,-9.5594902125713));
#290151=CARTESIAN_POINT('Ctrl Pts',(-1.86282443214733E-14,9.55624999997225,
-10.5687124469213));
#290152=CARTESIAN_POINT('Ctrl Pts',(-3.10606665601013,9.70624999997165,
-9.5594902125713));
#290153=CARTESIAN_POINT('Ctrl Pts',(-6.21213331202024,9.85624999997105,
-8.55026797822134));
#290154=CARTESIAN_POINT('Ctrl Pts',(-8.13178807675721,10.0062499999704,
-5.90808986649102));
#290155=CARTESIAN_POINT('Ctrl Pts',(-10.0514428414942,10.1562499999698,
-3.2659117547607));
#290156=CARTESIAN_POINT('Ctrl Pts',(-10.0514428414942,10.3062499999692,
2.46189346052968E-15));
#290157=CARTESIAN_POINT('Ctrl Pts',(-10.0514428414942,10.4562499999686,
3.26591175476071));
#290158=CARTESIAN_POINT('Ctrl Pts',(-8.13178807675721,10.606249999968,5.90808986649102));
#290159=CARTESIAN_POINT('Ctrl Pts',(-6.21213331202023,10.7562499999674,
8.55026797822134));
#290160=CARTESIAN_POINT('Ctrl Pts',(-3.10606665601013,10.9062499999668,
9.5594902125713));
#290161=CARTESIAN_POINT('Ctrl Pts',(-1.6903510983458E-14,11.0562499999663,
10.5687124469213));
#290162=CARTESIAN_POINT('Ctrl Pts',(3.10606665601009,11.2062499999657,9.5594902125713));
#290163=CARTESIAN_POINT('Ctrl Pts',(6.2121333120202,11.3562499999651,8.55026797822134));
#290164=CARTESIAN_POINT('Ctrl Pts',(8.13178807675717,11.5062499999645,5.90808986649102));
#290165=CARTESIAN_POINT('Ctrl Pts',(10.0514428414941,11.6562499999639,3.2659117547607));
#290166=CARTESIAN_POINT('Ctrl Pts',(10.0514428414941,11.8062499999633,-1.23094673026484E-15));
#290167=CARTESIAN_POINT('Ctrl Pts',(10.0514428414941,8.43124999997676,-1.23094673026484E-15));
#290168=CARTESIAN_POINT('Ctrl Pts',(10.0514428414941,8.58124999997616,-3.26591175476071));
#290169=CARTESIAN_POINT('Ctrl Pts',(8.13178807675717,8.73124999997556,-5.90808986649102));
#290170=CARTESIAN_POINT('Ctrl Pts',(6.2121333120202,8.88124999997496,-8.55026797822134));
#290171=CARTESIAN_POINT('Ctrl Pts',(3.10606665601009,9.03124999997436,-9.5594902125713));
#290172=CARTESIAN_POINT('Ctrl Pts',(-1.84122806625156E-14,9.18124999997375,
-10.5687124469213));
#290173=CARTESIAN_POINT('Ctrl Pts',(-3.10606665601013,9.33124999997315,
-9.5594902125713));
#290174=CARTESIAN_POINT('Ctrl Pts',(-6.21213331202024,9.48124999997255,
-8.55026797822134));
#290175=CARTESIAN_POINT('Ctrl Pts',(-8.13178807675721,9.63124999997195,
-5.90808986649102));
#290176=CARTESIAN_POINT('Ctrl Pts',(-10.0514428414942,9.78124999997135,
-3.2659117547607));
#290177=CARTESIAN_POINT('Ctrl Pts',(-10.0514428414942,9.93124999997075,
2.46189346052968E-15));
#290178=CARTESIAN_POINT('Ctrl Pts',(-10.0514428414942,10.0812499999701,
3.26591175476071));
#290179=CARTESIAN_POINT('Ctrl Pts',(-8.13178807675721,10.2312499999695,
5.90808986649102));
#290180=CARTESIAN_POINT('Ctrl Pts',(-6.21213331202023,10.3812499999689,
8.55026797822134));
#290181=CARTESIAN_POINT('Ctrl Pts',(-3.10606665601012,10.5312499999684,
9.5594902125713));
#290182=CARTESIAN_POINT('Ctrl Pts',(-1.66875473245003E-14,10.6812499999678,
10.5687124469213));
#290183=CARTESIAN_POINT('Ctrl Pts',(3.10606665601009,10.8312499999672,9.5594902125713));
#290184=CARTESIAN_POINT('Ctrl Pts',(6.2121333120202,10.9812499999666,8.55026797822134));
#290185=CARTESIAN_POINT('Ctrl Pts',(8.13178807675717,11.131249999966,5.90808986649102));
#290186=CARTESIAN_POINT('Ctrl Pts',(10.0514428414941,11.2812499999654,3.2659117547607));
#290187=CARTESIAN_POINT('Ctrl Pts',(10.0514428414941,11.4312499999648,-1.23094673026484E-15));
#290188=CARTESIAN_POINT('Origin',(-3.77475828372553E-14,-1.881249999982,
2.68644078414671E-15));
#290189=CARTESIAN_POINT('',(10.0514428414941,14.8062499999513,1.38622015537184E-15));
#290190=CARTESIAN_POINT('',(10.0514428414941,14.4312499999528,1.38777687219229E-15));
#290191=CARTESIAN_POINT('',(10.0514428414941,-1.881249999982,4.14193483802857E-15));
#290192=CARTESIAN_POINT('Ctrl Pts',(10.0514428414941,11.8062499999633,-1.23094673026484E-15));
#290193=CARTESIAN_POINT('Ctrl Pts',(10.0514428414941,11.9562499999627,-3.26591175476071));
#290194=CARTESIAN_POINT('Ctrl Pts',(8.13178807675717,12.1062499999621,-5.90808986649102));
#290195=CARTESIAN_POINT('Ctrl Pts',(6.2121333120202,12.2562499999615,-8.55026797822134));
#290196=CARTESIAN_POINT('Ctrl Pts',(3.10606665601009,12.4062499999609,-9.5594902125713));
#290197=CARTESIAN_POINT('Ctrl Pts',(-2.03559535931351E-14,12.5562499999603,
-10.5687124469213));
#290198=CARTESIAN_POINT('Ctrl Pts',(-3.10606665601013,12.7062499999597,
-9.5594902125713));
#290199=CARTESIAN_POINT('Ctrl Pts',(-6.21213331202024,12.856249999959,-8.55026797822134));
#290200=CARTESIAN_POINT('Ctrl Pts',(-8.13178807675721,13.0062499999584,
-5.90808986649102));
#290201=CARTESIAN_POINT('Ctrl Pts',(-10.0514428414942,13.1562499999578,
-3.2659117547607));
#290202=CARTESIAN_POINT('Ctrl Pts',(-10.0514428414942,13.3062499999572,
2.46189346052968E-15));
#290203=CARTESIAN_POINT('Ctrl Pts',(-10.0514428414942,13.4562499999566,
3.26591175476071));
#290204=CARTESIAN_POINT('Ctrl Pts',(-8.13178807675721,13.606249999956,5.90808986649102));
#290205=CARTESIAN_POINT('Ctrl Pts',(-6.21213331202023,13.7562499999554,
8.55026797822134));
#290206=CARTESIAN_POINT('Ctrl Pts',(-3.10606665601013,13.9062499999549,
9.5594902125713));
#290207=CARTESIAN_POINT('Ctrl Pts',(-1.86312202551199E-14,14.0562499999543,
10.5687124469213));
#290208=CARTESIAN_POINT('Ctrl Pts',(3.10606665601009,14.2062499999537,9.5594902125713));
#290209=CARTESIAN_POINT('Ctrl Pts',(6.2121333120202,14.3562499999531,8.55026797822134));
#290210=CARTESIAN_POINT('Ctrl Pts',(8.13178807675717,14.5062499999525,5.90808986649102));
#290211=CARTESIAN_POINT('Ctrl Pts',(10.0514428414941,14.6562499999519,3.2659117547607));
#290212=CARTESIAN_POINT('Ctrl Pts',(10.0514428414941,14.8062499999513,-1.23094673026484E-15));
#290213=CARTESIAN_POINT('Ctrl Pts',(10.0514428414941,11.4312499999648,-1.23094673026484E-15));
#290214=CARTESIAN_POINT('Ctrl Pts',(10.0514428414941,11.5812499999642,-3.26591175476071));
#290215=CARTESIAN_POINT('Ctrl Pts',(8.13178807675717,11.7312499999636,-5.90808986649102));
#290216=CARTESIAN_POINT('Ctrl Pts',(6.2121333120202,11.881249999963,-8.55026797822134));
#290217=CARTESIAN_POINT('Ctrl Pts',(3.10606665601009,12.0312499999624,-9.5594902125713));
#290218=CARTESIAN_POINT('Ctrl Pts',(-2.01399899341774E-14,12.1812499999618,
-10.5687124469213));
#290219=CARTESIAN_POINT('Ctrl Pts',(-3.10606665601013,12.3312499999612,
-9.5594902125713));
#290220=CARTESIAN_POINT('Ctrl Pts',(-6.21213331202024,12.4812499999605,
-8.55026797822134));
#290221=CARTESIAN_POINT('Ctrl Pts',(-8.13178807675721,12.6312499999599,
-5.90808986649102));
#290222=CARTESIAN_POINT('Ctrl Pts',(-10.0514428414942,12.7812499999593,
-3.2659117547607));
#290223=CARTESIAN_POINT('Ctrl Pts',(-10.0514428414942,12.9312499999587,
2.46189346052968E-15));
#290224=CARTESIAN_POINT('Ctrl Pts',(-10.0514428414942,13.0812499999581,
3.26591175476071));
#290225=CARTESIAN_POINT('Ctrl Pts',(-8.13178807675721,13.2312499999575,
5.90808986649102));
#290226=CARTESIAN_POINT('Ctrl Pts',(-6.21213331202023,13.3812499999569,
8.55026797822134));
#290227=CARTESIAN_POINT('Ctrl Pts',(-3.10606665601013,13.5312499999564,
9.5594902125713));
#290228=CARTESIAN_POINT('Ctrl Pts',(-1.84152565961621E-14,13.6812499999558,
10.5687124469213));
#290229=CARTESIAN_POINT('Ctrl Pts',(3.10606665601009,13.8312499999552,9.5594902125713));
#290230=CARTESIAN_POINT('Ctrl Pts',(6.2121333120202,13.9812499999546,8.55026797822134));
#290231=CARTESIAN_POINT('Ctrl Pts',(8.13178807675717,14.131249999954,5.90808986649102));
#290232=CARTESIAN_POINT('Ctrl Pts',(10.0514428414941,14.2812499999534,3.2659117547607));
#290233=CARTESIAN_POINT('Ctrl Pts',(10.0514428414941,14.4312499999528,-1.23094673026484E-15));
#290234=CARTESIAN_POINT('Origin',(-3.77475828372553E-14,-1.881249999982,
2.68644078414671E-15));
#290235=CARTESIAN_POINT('',(10.0514428414941,17.8062499999393,1.37376642080824E-15));
#290236=CARTESIAN_POINT('',(10.0514428414941,17.4312499999408,1.37532313762869E-15));
#290237=CARTESIAN_POINT('',(10.0514428414941,-1.881249999982,4.14193483802857E-15));
#290238=CARTESIAN_POINT('Ctrl Pts',(10.0514428414941,14.8062499999513,-1.23094673026484E-15));
#290239=CARTESIAN_POINT('Ctrl Pts',(10.0514428414941,14.9562499999507,-3.26591175476071));
#290240=CARTESIAN_POINT('Ctrl Pts',(8.13178807675717,15.1062499999501,-5.90808986649102));
#290241=CARTESIAN_POINT('Ctrl Pts',(6.21213331202019,15.2562499999495,-8.55026797822134));
#290242=CARTESIAN_POINT('Ctrl Pts',(3.10606665601009,15.4062499999489,-9.5594902125713));
#290243=CARTESIAN_POINT('Ctrl Pts',(-2.2083662864797E-14,15.5562499999482,
-10.5687124469213));
#290244=CARTESIAN_POINT('Ctrl Pts',(-3.10606665601013,15.7062499999477,
-9.5594902125713));
#290245=CARTESIAN_POINT('Ctrl Pts',(-6.21213331202024,15.856249999947,-8.55026797822134));
#290246=CARTESIAN_POINT('Ctrl Pts',(-8.13178807675721,16.0062499999464,
-5.90808986649102));
#290247=CARTESIAN_POINT('Ctrl Pts',(-10.0514428414942,16.1562499999458,
-3.2659117547607));
#290248=CARTESIAN_POINT('Ctrl Pts',(-10.0514428414942,16.3062499999452,
2.46189346052968E-15));
#290249=CARTESIAN_POINT('Ctrl Pts',(-10.0514428414942,16.4562499999446,
3.26591175476071));
#290250=CARTESIAN_POINT('Ctrl Pts',(-8.13178807675721,16.606249999944,5.90808986649102));
#290251=CARTESIAN_POINT('Ctrl Pts',(-6.21213331202024,16.7562499999434,
8.55026797822134));
#290252=CARTESIAN_POINT('Ctrl Pts',(-3.10606665601013,16.9062499999428,
9.5594902125713));
#290253=CARTESIAN_POINT('Ctrl Pts',(-2.03589295267817E-14,17.0562499999422,
10.5687124469213));
#290254=CARTESIAN_POINT('Ctrl Pts',(3.10606665601009,17.2062499999417,9.5594902125713));
#290255=CARTESIAN_POINT('Ctrl Pts',(6.2121333120202,17.3562499999411,8.55026797822134));
#290256=CARTESIAN_POINT('Ctrl Pts',(8.13178807675717,17.5062499999405,5.90808986649102));
#290257=CARTESIAN_POINT('Ctrl Pts',(10.0514428414941,17.6562499999399,3.2659117547607));
#290258=CARTESIAN_POINT('Ctrl Pts',(10.0514428414941,17.8062499999393,-1.23094673026484E-15));
#290259=CARTESIAN_POINT('Ctrl Pts',(10.0514428414941,14.4312499999528,-1.23094673026484E-15));
#290260=CARTESIAN_POINT('Ctrl Pts',(10.0514428414941,14.5812499999522,-3.26591175476071));
#290261=CARTESIAN_POINT('Ctrl Pts',(8.13178807675717,14.7312499999516,-5.90808986649102));
#290262=CARTESIAN_POINT('Ctrl Pts',(6.21213331202019,14.881249999951,-8.55026797822134));
#290263=CARTESIAN_POINT('Ctrl Pts',(3.10606665601009,15.0312499999504,-9.5594902125713));
#290264=CARTESIAN_POINT('Ctrl Pts',(-2.18676992058392E-14,15.1812499999498,
-10.5687124469213));
#290265=CARTESIAN_POINT('Ctrl Pts',(-3.10606665601013,15.3312499999492,
-9.5594902125713));
#290266=CARTESIAN_POINT('Ctrl Pts',(-6.21213331202024,15.4812499999485,
-8.55026797822134));
#290267=CARTESIAN_POINT('Ctrl Pts',(-8.13178807675721,15.6312499999479,
-5.90808986649102));
#290268=CARTESIAN_POINT('Ctrl Pts',(-10.0514428414942,15.7812499999473,
-3.2659117547607));
#290269=CARTESIAN_POINT('Ctrl Pts',(-10.0514428414942,15.9312499999467,
2.46189346052968E-15));
#290270=CARTESIAN_POINT('Ctrl Pts',(-10.0514428414942,16.0812499999461,
3.26591175476071));
#290271=CARTESIAN_POINT('Ctrl Pts',(-8.13178807675721,16.2312499999455,
5.90808986649102));
#290272=CARTESIAN_POINT('Ctrl Pts',(-6.21213331202024,16.3812499999449,
8.55026797822134));
#290273=CARTESIAN_POINT('Ctrl Pts',(-3.10606665601013,16.5312499999444,
9.5594902125713));
#290274=CARTESIAN_POINT('Ctrl Pts',(-2.0142965867824E-14,16.6812499999438,
10.5687124469213));
#290275=CARTESIAN_POINT('Ctrl Pts',(3.10606665601009,16.8312499999432,9.5594902125713));
#290276=CARTESIAN_POINT('Ctrl Pts',(6.2121333120202,16.9812499999426,8.55026797822134));
#290277=CARTESIAN_POINT('Ctrl Pts',(8.13178807675717,17.131249999942,5.90808986649102));
#290278=CARTESIAN_POINT('Ctrl Pts',(10.0514428414941,17.2812499999414,3.2659117547607));
#290279=CARTESIAN_POINT('Ctrl Pts',(10.0514428414941,17.4312499999408,-1.23094673026484E-15));
#290280=CARTESIAN_POINT('Origin',(-3.77475828372553E-14,-1.881249999982,
2.68644078414671E-15));
#290281=CARTESIAN_POINT('',(10.0514428414941,20.8062499999273,1.36131268624463E-15));
#290282=CARTESIAN_POINT('',(10.0514428414941,20.4312499999288,1.36286940306508E-15));
#290283=CARTESIAN_POINT('',(10.0514428414941,-1.881249999982,4.14193483802857E-15));
#290284=CARTESIAN_POINT('Ctrl Pts',(10.0514428414941,17.8062499999393,-1.23094673026484E-15));
#290285=CARTESIAN_POINT('Ctrl Pts',(10.0514428414941,17.9562499999387,-3.26591175476071));
#290286=CARTESIAN_POINT('Ctrl Pts',(8.13178807675717,18.1062499999381,-5.90808986649102));
#290287=CARTESIAN_POINT('Ctrl Pts',(6.21213331202019,18.2562499999375,-8.55026797822134));
#290288=CARTESIAN_POINT('Ctrl Pts',(3.10606665601008,18.4062499999369,-9.5594902125713));
#290289=CARTESIAN_POINT('Ctrl Pts',(-2.38113721364588E-14,18.5562499999362,
-10.5687124469213));
#290290=CARTESIAN_POINT('Ctrl Pts',(-3.10606665601013,18.7062499999357,
-9.5594902125713));
#290291=CARTESIAN_POINT('Ctrl Pts',(-6.21213331202024,18.856249999935,-8.55026797822134));
#290292=CARTESIAN_POINT('Ctrl Pts',(-8.13178807675721,19.0062499999344,
-5.90808986649102));
#290293=CARTESIAN_POINT('Ctrl Pts',(-10.0514428414942,19.1562499999338,
-3.2659117547607));
#290294=CARTESIAN_POINT('Ctrl Pts',(-10.0514428414942,19.3062499999332,
2.46189346052968E-15));
#290295=CARTESIAN_POINT('Ctrl Pts',(-10.0514428414942,19.4562499999326,
3.26591175476071));
#290296=CARTESIAN_POINT('Ctrl Pts',(-8.13178807675721,19.606249999932,5.90808986649102));
#290297=CARTESIAN_POINT('Ctrl Pts',(-6.21213331202024,19.7562499999314,
8.55026797822134));
#290298=CARTESIAN_POINT('Ctrl Pts',(-3.10606665601013,19.9062499999308,
9.5594902125713));
#290299=CARTESIAN_POINT('Ctrl Pts',(-2.20866387984436E-14,20.0562499999302,
10.5687124469213));
#290300=CARTESIAN_POINT('Ctrl Pts',(3.10606665601009,20.2062499999297,9.5594902125713));
#290301=CARTESIAN_POINT('Ctrl Pts',(6.21213331202019,20.356249999929,8.55026797822134));
#290302=CARTESIAN_POINT('Ctrl Pts',(8.13178807675717,20.5062499999285,5.90808986649102));
#290303=CARTESIAN_POINT('Ctrl Pts',(10.0514428414941,20.6562499999279,3.2659117547607));
#290304=CARTESIAN_POINT('Ctrl Pts',(10.0514428414941,20.8062499999273,-1.23094673026484E-15));
#290305=CARTESIAN_POINT('Ctrl Pts',(10.0514428414941,17.4312499999408,-1.23094673026484E-15));
#290306=CARTESIAN_POINT('Ctrl Pts',(10.0514428414941,17.5812499999402,-3.26591175476071));
#290307=CARTESIAN_POINT('Ctrl Pts',(8.13178807675717,17.7312499999396,-5.90808986649102));
#290308=CARTESIAN_POINT('Ctrl Pts',(6.21213331202019,17.881249999939,-8.55026797822134));
#290309=CARTESIAN_POINT('Ctrl Pts',(3.10606665601008,18.0312499999384,-9.5594902125713));
#290310=CARTESIAN_POINT('Ctrl Pts',(-2.35954084775011E-14,18.1812499999378,
-10.5687124469213));
#290311=CARTESIAN_POINT('Ctrl Pts',(-3.10606665601013,18.3312499999371,
-9.5594902125713));
#290312=CARTESIAN_POINT('Ctrl Pts',(-6.21213331202024,18.4812499999365,
-8.55026797822134));
#290313=CARTESIAN_POINT('Ctrl Pts',(-8.13178807675721,18.6312499999359,
-5.90808986649102));
#290314=CARTESIAN_POINT('Ctrl Pts',(-10.0514428414942,18.7812499999353,
-3.2659117547607));
#290315=CARTESIAN_POINT('Ctrl Pts',(-10.0514428414942,18.9312499999347,
2.46189346052968E-15));
#290316=CARTESIAN_POINT('Ctrl Pts',(-10.0514428414942,19.0812499999341,
3.26591175476071));
#290317=CARTESIAN_POINT('Ctrl Pts',(-8.13178807675721,19.2312499999335,
5.90808986649102));
#290318=CARTESIAN_POINT('Ctrl Pts',(-6.21213331202024,19.3812499999329,
8.55026797822134));
#290319=CARTESIAN_POINT('Ctrl Pts',(-3.10606665601013,19.5312499999323,
9.5594902125713));
#290320=CARTESIAN_POINT('Ctrl Pts',(-2.18706751394858E-14,19.6812499999318,
10.5687124469213));
#290321=CARTESIAN_POINT('Ctrl Pts',(3.10606665601009,19.8312499999312,9.5594902125713));
#290322=CARTESIAN_POINT('Ctrl Pts',(6.21213331202019,19.9812499999306,8.55026797822134));
#290323=CARTESIAN_POINT('Ctrl Pts',(8.13178807675717,20.13124999993,5.90808986649102));
#290324=CARTESIAN_POINT('Ctrl Pts',(10.0514428414941,20.2812499999294,3.2659117547607));
#290325=CARTESIAN_POINT('Ctrl Pts',(10.0514428414941,20.4312499999288,-1.23094673026484E-15));
#290326=CARTESIAN_POINT('Origin',(-3.77475828372553E-14,-1.881249999982,
2.68644078414671E-15));
#290327=CARTESIAN_POINT('',(10.0514428414941,23.8062499999153,1.34885895168103E-15));
#290328=CARTESIAN_POINT('',(10.0514428414941,23.4312499999168,1.35041566850148E-15));
#290329=CARTESIAN_POINT('',(10.0514428414941,-1.881249999982,4.14193483802857E-15));
#290330=CARTESIAN_POINT('Ctrl Pts',(10.0514428414941,20.8062499999273,-1.23094673026484E-15));
#290331=CARTESIAN_POINT('Ctrl Pts',(10.0514428414941,20.9562499999267,-3.26591175476071));
#290332=CARTESIAN_POINT('Ctrl Pts',(8.13178807675716,21.1062499999261,-5.90808986649102));
#290333=CARTESIAN_POINT('Ctrl Pts',(6.21213331202019,21.2562499999255,-8.55026797822134));
#290334=CARTESIAN_POINT('Ctrl Pts',(3.10606665601008,21.4062499999249,-9.5594902125713));
#290335=CARTESIAN_POINT('Ctrl Pts',(-2.55390814081206E-14,21.5562499999242,
-10.5687124469213));
#290336=CARTESIAN_POINT('Ctrl Pts',(-3.10606665601013,21.7062499999237,
-9.5594902125713));
#290337=CARTESIAN_POINT('Ctrl Pts',(-6.21213331202024,21.856249999923,-8.55026797822134));
#290338=CARTESIAN_POINT('Ctrl Pts',(-8.13178807675722,22.0062499999224,
-5.90808986649102));
#290339=CARTESIAN_POINT('Ctrl Pts',(-10.0514428414942,22.1562499999218,
-3.2659117547607));
#290340=CARTESIAN_POINT('Ctrl Pts',(-10.0514428414942,22.3062499999212,
2.46189346052968E-15));
#290341=CARTESIAN_POINT('Ctrl Pts',(-10.0514428414942,22.4562499999206,
3.26591175476071));
#290342=CARTESIAN_POINT('Ctrl Pts',(-8.13178807675722,22.60624999992,5.90808986649102));
#290343=CARTESIAN_POINT('Ctrl Pts',(-6.21213331202024,22.7562499999194,
8.55026797822134));
#290344=CARTESIAN_POINT('Ctrl Pts',(-3.10606665601013,22.9062499999188,
9.5594902125713));
#290345=CARTESIAN_POINT('Ctrl Pts',(-2.38143480701054E-14,23.0562499999182,
10.5687124469213));
#290346=CARTESIAN_POINT('Ctrl Pts',(3.10606665601008,23.2062499999177,9.5594902125713));
#290347=CARTESIAN_POINT('Ctrl Pts',(6.21213331202019,23.3562499999171,8.55026797822134));
#290348=CARTESIAN_POINT('Ctrl Pts',(8.13178807675716,23.5062499999165,5.90808986649102));
#290349=CARTESIAN_POINT('Ctrl Pts',(10.0514428414941,23.6562499999159,3.2659117547607));
#290350=CARTESIAN_POINT('Ctrl Pts',(10.0514428414941,23.8062499999153,-1.23094673026484E-15));
#290351=CARTESIAN_POINT('Ctrl Pts',(10.0514428414941,20.4312499999288,-1.23094673026484E-15));
#290352=CARTESIAN_POINT('Ctrl Pts',(10.0514428414941,20.5812499999282,-3.26591175476071));
#290353=CARTESIAN_POINT('Ctrl Pts',(8.13178807675716,20.7312499999276,-5.90808986649102));
#290354=CARTESIAN_POINT('Ctrl Pts',(6.21213331202019,20.881249999927,-8.55026797822134));
#290355=CARTESIAN_POINT('Ctrl Pts',(3.10606665601008,21.0312499999264,-9.5594902125713));
#290356=CARTESIAN_POINT('Ctrl Pts',(-2.53231177491629E-14,21.1812499999258,
-10.5687124469213));
#290357=CARTESIAN_POINT('Ctrl Pts',(-3.10606665601013,21.3312499999251,
-9.5594902125713));
#290358=CARTESIAN_POINT('Ctrl Pts',(-6.21213331202024,21.4812499999245,
-8.55026797822134));
#290359=CARTESIAN_POINT('Ctrl Pts',(-8.13178807675722,21.6312499999239,
-5.90808986649102));
#290360=CARTESIAN_POINT('Ctrl Pts',(-10.0514428414942,21.7812499999233,
-3.2659117547607));
#290361=CARTESIAN_POINT('Ctrl Pts',(-10.0514428414942,21.9312499999227,
2.46189346052968E-15));
#290362=CARTESIAN_POINT('Ctrl Pts',(-10.0514428414942,22.0812499999221,
3.26591175476071));
#290363=CARTESIAN_POINT('Ctrl Pts',(-8.13178807675722,22.2312499999215,
5.90808986649102));
#290364=CARTESIAN_POINT('Ctrl Pts',(-6.21213331202024,22.3812499999209,
8.55026797822134));
#290365=CARTESIAN_POINT('Ctrl Pts',(-3.10606665601013,22.5312499999204,
9.5594902125713));
#290366=CARTESIAN_POINT('Ctrl Pts',(-2.35983844111477E-14,22.6812499999198,
10.5687124469213));
#290367=CARTESIAN_POINT('Ctrl Pts',(3.10606665601008,22.8312499999192,9.5594902125713));
#290368=CARTESIAN_POINT('Ctrl Pts',(6.21213331202019,22.9812499999186,8.55026797822134));
#290369=CARTESIAN_POINT('Ctrl Pts',(8.13178807675716,23.131249999918,5.90808986649102));
#290370=CARTESIAN_POINT('Ctrl Pts',(10.0514428414941,23.2812499999174,3.2659117547607));
#290371=CARTESIAN_POINT('Ctrl Pts',(10.0514428414941,23.4312499999168,-1.23094673026484E-15));
#290372=CARTESIAN_POINT('Origin',(-3.77475828372553E-14,-1.881249999982,
2.68644078414671E-15));
#290373=CARTESIAN_POINT('',(10.0514428414941,26.8062499999033,1.33640521711743E-15));
#290374=CARTESIAN_POINT('',(10.0514428414941,26.4312499999048,1.33796193393788E-15));
#290375=CARTESIAN_POINT('',(10.0514428414941,-1.881249999982,4.14193483802857E-15));
#290376=CARTESIAN_POINT('Ctrl Pts',(10.0514428414941,23.8062499999153,-1.23094673026484E-15));
#290377=CARTESIAN_POINT('Ctrl Pts',(10.0514428414941,23.9562499999147,-3.26591175476071));
#290378=CARTESIAN_POINT('Ctrl Pts',(8.13178807675716,24.1062499999141,-5.90808986649102));
#290379=CARTESIAN_POINT('Ctrl Pts',(6.21213331202019,24.2562499999135,-8.55026797822134));
#290380=CARTESIAN_POINT('Ctrl Pts',(3.10606665601008,24.4062499999129,-9.5594902125713));
#290381=CARTESIAN_POINT('Ctrl Pts',(-2.72667906797825E-14,24.5562499999122,
-10.5687124469213));
#290382=CARTESIAN_POINT('Ctrl Pts',(-3.10606665601014,24.7062499999116,
-9.5594902125713));
#290383=CARTESIAN_POINT('Ctrl Pts',(-6.21213331202024,24.856249999911,-8.55026797822134));
#290384=CARTESIAN_POINT('Ctrl Pts',(-8.13178807675722,25.0062499999104,
-5.90808986649102));
#290385=CARTESIAN_POINT('Ctrl Pts',(-10.0514428414942,25.1562499999098,
-3.2659117547607));
#290386=CARTESIAN_POINT('Ctrl Pts',(-10.0514428414942,25.3062499999092,
2.46189346052968E-15));
#290387=CARTESIAN_POINT('Ctrl Pts',(-10.0514428414942,25.4562499999086,
3.26591175476071));
#290388=CARTESIAN_POINT('Ctrl Pts',(-8.13178807675722,25.6062499999081,
5.90808986649102));
#290389=CARTESIAN_POINT('Ctrl Pts',(-6.21213331202024,25.7562499999074,
8.55026797822134));
#290390=CARTESIAN_POINT('Ctrl Pts',(-3.10606665601013,25.9062499999069,
9.5594902125713));
#290391=CARTESIAN_POINT('Ctrl Pts',(-2.55420573417672E-14,26.0562499999062,
10.5687124469213));
#290392=CARTESIAN_POINT('Ctrl Pts',(3.10606665601008,26.2062499999057,9.5594902125713));
#290393=CARTESIAN_POINT('Ctrl Pts',(6.21213331202019,26.356249999905,8.55026797822134));
#290394=CARTESIAN_POINT('Ctrl Pts',(8.13178807675716,26.5062499999045,5.90808986649102));
#290395=CARTESIAN_POINT('Ctrl Pts',(10.0514428414941,26.6562499999039,3.2659117547607));
#290396=CARTESIAN_POINT('Ctrl Pts',(10.0514428414941,26.8062499999033,-1.23094673026484E-15));
#290397=CARTESIAN_POINT('Ctrl Pts',(10.0514428414941,23.4312499999168,-1.23094673026484E-15));
#290398=CARTESIAN_POINT('Ctrl Pts',(10.0514428414941,23.5812499999162,-3.26591175476071));
#290399=CARTESIAN_POINT('Ctrl Pts',(8.13178807675716,23.7312499999156,-5.90808986649102));
#290400=CARTESIAN_POINT('Ctrl Pts',(6.21213331202019,23.881249999915,-8.55026797822134));
#290401=CARTESIAN_POINT('Ctrl Pts',(3.10606665601008,24.0312499999144,-9.5594902125713));
#290402=CARTESIAN_POINT('Ctrl Pts',(-2.70508270208248E-14,24.1812499999138,
-10.5687124469213));
#290403=CARTESIAN_POINT('Ctrl Pts',(-3.10606665601014,24.3312499999131,
-9.5594902125713));
#290404=CARTESIAN_POINT('Ctrl Pts',(-6.21213331202024,24.4812499999125,
-8.55026797822134));
#290405=CARTESIAN_POINT('Ctrl Pts',(-8.13178807675722,24.6312499999119,
-5.90808986649102));
#290406=CARTESIAN_POINT('Ctrl Pts',(-10.0514428414942,24.7812499999113,
-3.2659117547607));
#290407=CARTESIAN_POINT('Ctrl Pts',(-10.0514428414942,24.9312499999107,
2.46189346052968E-15));
#290408=CARTESIAN_POINT('Ctrl Pts',(-10.0514428414942,25.0812499999101,
3.26591175476071));
#290409=CARTESIAN_POINT('Ctrl Pts',(-8.13178807675722,25.2312499999095,
5.90808986649102));
#290410=CARTESIAN_POINT('Ctrl Pts',(-6.21213331202024,25.381249999909,8.55026797822134));
#290411=CARTESIAN_POINT('Ctrl Pts',(-3.10606665601013,25.5312499999084,
9.5594902125713));
#290412=CARTESIAN_POINT('Ctrl Pts',(-2.53260936828095E-14,25.6812499999078,
10.5687124469213));
#290413=CARTESIAN_POINT('Ctrl Pts',(3.10606665601008,25.8312499999072,9.5594902125713));
#290414=CARTESIAN_POINT('Ctrl Pts',(6.21213331202019,25.9812499999066,8.55026797822134));
#290415=CARTESIAN_POINT('Ctrl Pts',(8.13178807675716,26.131249999906,5.90808986649102));
#290416=CARTESIAN_POINT('Ctrl Pts',(10.0514428414941,26.2812499999054,3.2659117547607));
#290417=CARTESIAN_POINT('Ctrl Pts',(10.0514428414941,26.4312499999048,-1.23094673026484E-15));
#290418=CARTESIAN_POINT('Origin',(-3.77475828372553E-14,-1.881249999982,
2.68644078414671E-15));
#290419=CARTESIAN_POINT('',(10.0514428414941,29.8062499998913,1.32395148255383E-15));
#290420=CARTESIAN_POINT('',(10.0514428414941,29.4312499998928,1.32550819937428E-15));
#290421=CARTESIAN_POINT('',(10.0514428414941,-1.881249999982,4.14193483802857E-15));
#290422=CARTESIAN_POINT('Ctrl Pts',(10.0514428414941,26.8062499999033,-1.23094673026484E-15));
#290423=CARTESIAN_POINT('Ctrl Pts',(10.0514428414941,26.9562499999027,-3.26591175476071));
#290424=CARTESIAN_POINT('Ctrl Pts',(8.13178807675716,27.1062499999021,-5.90808986649102));
#290425=CARTESIAN_POINT('Ctrl Pts',(6.21213331202019,27.2562499999015,-8.55026797822134));
#290426=CARTESIAN_POINT('Ctrl Pts',(3.10606665601008,27.4062499999009,-9.5594902125713));
#290427=CARTESIAN_POINT('Ctrl Pts',(-2.89944999514443E-14,27.5562499999003,
-10.5687124469213));
#290428=CARTESIAN_POINT('Ctrl Pts',(-3.10606665601014,27.7062499998996,
-9.5594902125713));
#290429=CARTESIAN_POINT('Ctrl Pts',(-6.21213331202024,27.856249999899,-8.55026797822134));
#290430=CARTESIAN_POINT('Ctrl Pts',(-8.13178807675722,28.0062499998984,
-5.90808986649102));
#290431=CARTESIAN_POINT('Ctrl Pts',(-10.0514428414942,28.1562499998978,
-3.2659117547607));
#290432=CARTESIAN_POINT('Ctrl Pts',(-10.0514428414942,28.3062499998973,
2.46189346052968E-15));
#290433=CARTESIAN_POINT('Ctrl Pts',(-10.0514428414942,28.4562499998966,
3.26591175476071));
#290434=CARTESIAN_POINT('Ctrl Pts',(-8.13178807675722,28.606249999896,5.90808986649102));
#290435=CARTESIAN_POINT('Ctrl Pts',(-6.21213331202024,28.7562499998954,
8.55026797822134));
#290436=CARTESIAN_POINT('Ctrl Pts',(-3.10606665601014,28.9062499998949,
9.5594902125713));
#290437=CARTESIAN_POINT('Ctrl Pts',(-2.72697666134291E-14,29.0562499998942,
10.5687124469213));
#290438=CARTESIAN_POINT('Ctrl Pts',(3.10606665601008,29.2062499998937,9.5594902125713));
#290439=CARTESIAN_POINT('Ctrl Pts',(6.21213331202019,29.356249999893,8.55026797822134));
#290440=CARTESIAN_POINT('Ctrl Pts',(8.13178807675716,29.5062499998925,5.90808986649102));
#290441=CARTESIAN_POINT('Ctrl Pts',(10.0514428414941,29.6562499998919,3.2659117547607));
#290442=CARTESIAN_POINT('Ctrl Pts',(10.0514428414941,29.8062499998913,-1.23094673026484E-15));
#290443=CARTESIAN_POINT('Ctrl Pts',(10.0514428414941,26.4312499999048,-1.23094673026484E-15));
#290444=CARTESIAN_POINT('Ctrl Pts',(10.0514428414941,26.5812499999042,-3.26591175476071));
#290445=CARTESIAN_POINT('Ctrl Pts',(8.13178807675716,26.7312499999036,-5.90808986649102));
#290446=CARTESIAN_POINT('Ctrl Pts',(6.21213331202019,26.881249999903,-8.55026797822134));
#290447=CARTESIAN_POINT('Ctrl Pts',(3.10606665601008,27.0312499999024,-9.5594902125713));
#290448=CARTESIAN_POINT('Ctrl Pts',(-2.87785362924866E-14,27.1812499999018,
-10.5687124469213));
#290449=CARTESIAN_POINT('Ctrl Pts',(-3.10606665601014,27.3312499999011,
-9.5594902125713));
#290450=CARTESIAN_POINT('Ctrl Pts',(-6.21213331202024,27.4812499999005,
-8.55026797822134));
#290451=CARTESIAN_POINT('Ctrl Pts',(-8.13178807675722,27.6312499998999,
-5.90808986649102));
#290452=CARTESIAN_POINT('Ctrl Pts',(-10.0514428414942,27.7812499998993,
-3.2659117547607));
#290453=CARTESIAN_POINT('Ctrl Pts',(-10.0514428414942,27.9312499998987,
2.46189346052968E-15));
#290454=CARTESIAN_POINT('Ctrl Pts',(-10.0514428414942,28.0812499998981,
3.26591175476071));
#290455=CARTESIAN_POINT('Ctrl Pts',(-8.13178807675722,28.2312499998975,
5.90808986649102));
#290456=CARTESIAN_POINT('Ctrl Pts',(-6.21213331202024,28.3812499998969,
8.55026797822134));
#290457=CARTESIAN_POINT('Ctrl Pts',(-3.10606665601014,28.5312499998964,
9.5594902125713));
#290458=CARTESIAN_POINT('Ctrl Pts',(-2.70538029544713E-14,28.6812499998958,
10.5687124469213));
#290459=CARTESIAN_POINT('Ctrl Pts',(3.10606665601008,28.8312499998952,9.5594902125713));
#290460=CARTESIAN_POINT('Ctrl Pts',(6.21213331202019,28.9812499998946,8.55026797822134));
#290461=CARTESIAN_POINT('Ctrl Pts',(8.13178807675716,29.131249999894,5.90808986649102));
#290462=CARTESIAN_POINT('Ctrl Pts',(10.0514428414941,29.2812499998934,3.2659117547607));
#290463=CARTESIAN_POINT('Ctrl Pts',(10.0514428414941,29.4312499998928,-1.23094673026484E-15));
#290464=CARTESIAN_POINT('Origin',(-3.77475828372553E-14,-1.881249999982,
2.68644078414671E-15));
#290465=CARTESIAN_POINT('',(10.0514428414941,32.8062499998793,1.31149774799023E-15));
#290466=CARTESIAN_POINT('',(10.0514428414941,32.4312499998808,1.31305446481068E-15));
#290467=CARTESIAN_POINT('',(10.0514428414941,-1.881249999982,4.14193483802857E-15));
#290468=CARTESIAN_POINT('Ctrl Pts',(10.0514428414941,29.8062499998913,-1.23094673026484E-15));
#290469=CARTESIAN_POINT('Ctrl Pts',(10.0514428414941,29.9562499998907,-3.26591175476071));
#290470=CARTESIAN_POINT('Ctrl Pts',(8.13178807675716,30.1062499998901,-5.90808986649102));
#290471=CARTESIAN_POINT('Ctrl Pts',(6.21213331202019,30.2562499998894,-8.55026797822134));
#290472=CARTESIAN_POINT('Ctrl Pts',(3.10606665601008,30.4062499998889,-9.5594902125713));
#290473=CARTESIAN_POINT('Ctrl Pts',(-3.07222092231062E-14,30.5562499998883,
-10.5687124469213));
#290474=CARTESIAN_POINT('Ctrl Pts',(-3.10606665601014,30.7062499998877,
-9.5594902125713));
#290475=CARTESIAN_POINT('Ctrl Pts',(-6.21213331202025,30.8562499998871,
-8.55026797822134));
#290476=CARTESIAN_POINT('Ctrl Pts',(-8.13178807675722,31.0062499998864,
-5.90808986649102));
#290477=CARTESIAN_POINT('Ctrl Pts',(-10.0514428414942,31.1562499998858,
-3.2659117547607));
#290478=CARTESIAN_POINT('Ctrl Pts',(-10.0514428414942,31.3062499998852,
2.46189346052968E-15));
#290479=CARTESIAN_POINT('Ctrl Pts',(-10.0514428414942,31.4562499998847,
3.26591175476071));
#290480=CARTESIAN_POINT('Ctrl Pts',(-8.13178807675722,31.606249999884,5.90808986649102));
#290481=CARTESIAN_POINT('Ctrl Pts',(-6.21213331202024,31.7562499998835,
8.55026797822134));
#290482=CARTESIAN_POINT('Ctrl Pts',(-3.10606665601014,31.9062499998829,
9.5594902125713));
#290483=CARTESIAN_POINT('Ctrl Pts',(-2.89974758850909E-14,32.0562499998822,
10.5687124469213));
#290484=CARTESIAN_POINT('Ctrl Pts',(3.10606665601008,32.2062499998816,9.5594902125713));
#290485=CARTESIAN_POINT('Ctrl Pts',(6.21213331202019,32.3562499998811,8.55026797822134));
#290486=CARTESIAN_POINT('Ctrl Pts',(8.13178807675716,32.5062499998805,5.90808986649102));
#290487=CARTESIAN_POINT('Ctrl Pts',(10.0514428414941,32.6562499998799,3.2659117547607));
#290488=CARTESIAN_POINT('Ctrl Pts',(10.0514428414941,32.8062499998793,-1.23094673026484E-15));
#290489=CARTESIAN_POINT('Ctrl Pts',(10.0514428414941,29.4312499998928,-1.23094673026484E-15));
#290490=CARTESIAN_POINT('Ctrl Pts',(10.0514428414941,29.5812499998922,-3.26591175476071));
#290491=CARTESIAN_POINT('Ctrl Pts',(8.13178807675716,29.7312499998916,-5.90808986649102));
#290492=CARTESIAN_POINT('Ctrl Pts',(6.21213331202019,29.881249999891,-8.55026797822134));
#290493=CARTESIAN_POINT('Ctrl Pts',(3.10606665601008,30.0312499998904,-9.5594902125713));
#290494=CARTESIAN_POINT('Ctrl Pts',(-3.05062455641484E-14,30.1812499998898,
-10.5687124469213));
#290495=CARTESIAN_POINT('Ctrl Pts',(-3.10606665601014,30.3312499998892,
-9.5594902125713));
#290496=CARTESIAN_POINT('Ctrl Pts',(-6.21213331202025,30.4812499998885,
-8.55026797822134));
#290497=CARTESIAN_POINT('Ctrl Pts',(-8.13178807675722,30.6312499998879,
-5.90808986649102));
#290498=CARTESIAN_POINT('Ctrl Pts',(-10.0514428414942,30.7812499998873,
-3.2659117547607));
#290499=CARTESIAN_POINT('Ctrl Pts',(-10.0514428414942,30.9312499998867,
2.46189346052968E-15));
#290500=CARTESIAN_POINT('Ctrl Pts',(-10.0514428414942,31.0812499998861,
3.26591175476071));
#290501=CARTESIAN_POINT('Ctrl Pts',(-8.13178807675722,31.2312499998855,
5.90808986649102));
#290502=CARTESIAN_POINT('Ctrl Pts',(-6.21213331202024,31.381249999885,8.55026797822134));
#290503=CARTESIAN_POINT('Ctrl Pts',(-3.10606665601014,31.5312499998843,
9.5594902125713));
#290504=CARTESIAN_POINT('Ctrl Pts',(-2.87815122261332E-14,31.6812499998838,
10.5687124469213));
#290505=CARTESIAN_POINT('Ctrl Pts',(3.10606665601008,31.8312499998832,9.5594902125713));
#290506=CARTESIAN_POINT('Ctrl Pts',(6.21213331202019,31.9812499998826,8.55026797822134));
#290507=CARTESIAN_POINT('Ctrl Pts',(8.13178807675716,32.131249999882,5.90808986649102));
#290508=CARTESIAN_POINT('Ctrl Pts',(10.0514428414941,32.2812499998814,3.2659117547607));
#290509=CARTESIAN_POINT('Ctrl Pts',(10.0514428414941,32.4312499998808,-1.23094673026484E-15));
#290510=CARTESIAN_POINT('Origin',(-3.77475828372553E-14,-1.881249999982,
2.68644078414671E-15));
#290511=CARTESIAN_POINT('',(10.0514428414941,35.8062499998673,1.29904401342663E-15));
#290512=CARTESIAN_POINT('',(10.0514428414941,35.4312499998688,1.30060073024708E-15));
#290513=CARTESIAN_POINT('',(10.0514428414941,-1.881249999982,4.14193483802857E-15));
#290514=CARTESIAN_POINT('Ctrl Pts',(10.0514428414941,32.8062499998793,-1.23094673026484E-15));
#290515=CARTESIAN_POINT('Ctrl Pts',(10.0514428414941,32.9562499998787,-3.26591175476071));
#290516=CARTESIAN_POINT('Ctrl Pts',(8.13178807675716,33.1062499998781,-5.90808986649102));
#290517=CARTESIAN_POINT('Ctrl Pts',(6.21213331202018,33.2562499998775,-8.55026797822134));
#290518=CARTESIAN_POINT('Ctrl Pts',(3.10606665601008,33.4062499998769,-9.5594902125713));
#290519=CARTESIAN_POINT('Ctrl Pts',(-3.2449918494768E-14,33.5562499998763,
-10.5687124469213));
#290520=CARTESIAN_POINT('Ctrl Pts',(-3.10606665601014,33.7062499998756,
-9.5594902125713));
#290521=CARTESIAN_POINT('Ctrl Pts',(-6.21213331202025,33.856249999875,-8.55026797822134));
#290522=CARTESIAN_POINT('Ctrl Pts',(-8.13178807675722,34.0062499998744,
-5.90808986649102));
#290523=CARTESIAN_POINT('Ctrl Pts',(-10.0514428414942,34.1562499998739,
-3.2659117547607));
#290524=CARTESIAN_POINT('Ctrl Pts',(-10.0514428414942,34.3062499998732,
2.46189346052968E-15));
#290525=CARTESIAN_POINT('Ctrl Pts',(-10.0514428414942,34.4562499998727,
3.26591175476071));
#290526=CARTESIAN_POINT('Ctrl Pts',(-8.13178807675722,34.606249999872,5.90808986649102));
#290527=CARTESIAN_POINT('Ctrl Pts',(-6.21213331202024,34.7562499998714,
8.55026797822134));
#290528=CARTESIAN_POINT('Ctrl Pts',(-3.10606665601014,34.9062499998708,
9.5594902125713));
#290529=CARTESIAN_POINT('Ctrl Pts',(-3.07251851567527E-14,35.0562499998703,
10.5687124469213));
#290530=CARTESIAN_POINT('Ctrl Pts',(3.10606665601008,35.2062499998697,9.5594902125713));
#290531=CARTESIAN_POINT('Ctrl Pts',(6.21213331202019,35.3562499998691,8.55026797822134));
#290532=CARTESIAN_POINT('Ctrl Pts',(8.13178807675716,35.5062499998685,5.90808986649102));
#290533=CARTESIAN_POINT('Ctrl Pts',(10.0514428414941,35.6562499998679,3.2659117547607));
#290534=CARTESIAN_POINT('Ctrl Pts',(10.0514428414941,35.8062499998673,-1.23094673026484E-15));
#290535=CARTESIAN_POINT('Ctrl Pts',(10.0514428414941,32.4312499998808,-1.23094673026484E-15));
#290536=CARTESIAN_POINT('Ctrl Pts',(10.0514428414941,32.5812499998802,-3.26591175476071));
#290537=CARTESIAN_POINT('Ctrl Pts',(8.13178807675716,32.7312499998796,-5.90808986649102));
#290538=CARTESIAN_POINT('Ctrl Pts',(6.21213331202018,32.8812499998789,-8.55026797822134));
#290539=CARTESIAN_POINT('Ctrl Pts',(3.10606665601008,33.0312499998784,-9.5594902125713));
#290540=CARTESIAN_POINT('Ctrl Pts',(-3.22339548358103E-14,33.1812499998777,
-10.5687124469213));
#290541=CARTESIAN_POINT('Ctrl Pts',(-3.10606665601014,33.3312499998772,
-9.5594902125713));
#290542=CARTESIAN_POINT('Ctrl Pts',(-6.21213331202025,33.4812499998765,
-8.55026797822134));
#290543=CARTESIAN_POINT('Ctrl Pts',(-8.13178807675722,33.6312499998759,
-5.90808986649102));
#290544=CARTESIAN_POINT('Ctrl Pts',(-10.0514428414942,33.7812499998753,
-3.2659117547607));
#290545=CARTESIAN_POINT('Ctrl Pts',(-10.0514428414942,33.9312499998747,
2.46189346052968E-15));
#290546=CARTESIAN_POINT('Ctrl Pts',(-10.0514428414942,34.0812499998741,
3.26591175476071));
#290547=CARTESIAN_POINT('Ctrl Pts',(-8.13178807675722,34.2312499998735,
5.90808986649102));
#290548=CARTESIAN_POINT('Ctrl Pts',(-6.21213331202024,34.3812499998729,
8.55026797822134));
#290549=CARTESIAN_POINT('Ctrl Pts',(-3.10606665601014,34.5312499998724,
9.5594902125713));
#290550=CARTESIAN_POINT('Ctrl Pts',(-3.0509221497795E-14,34.6812499998718,
10.5687124469213));
#290551=CARTESIAN_POINT('Ctrl Pts',(3.10606665601008,34.8312499998712,9.5594902125713));
#290552=CARTESIAN_POINT('Ctrl Pts',(6.21213331202019,34.9812499998706,8.55026797822134));
#290553=CARTESIAN_POINT('Ctrl Pts',(8.13178807675716,35.13124999987,5.90808986649102));
#290554=CARTESIAN_POINT('Ctrl Pts',(10.0514428414941,35.2812499998694,3.2659117547607));
#290555=CARTESIAN_POINT('Ctrl Pts',(10.0514428414941,35.4312499998688,-1.23094673026484E-15));
#290556=CARTESIAN_POINT('Origin',(-3.77475828372553E-14,-1.881249999982,
2.68644078414671E-15));
#290557=CARTESIAN_POINT('',(10.0514428414941,38.8062499998553,1.28659027886303E-15));
#290558=CARTESIAN_POINT('',(10.0514428414941,38.4312499998568,1.28814699568348E-15));
#290559=CARTESIAN_POINT('',(10.0514428414941,-1.881249999982,4.14193483802857E-15));
#290560=CARTESIAN_POINT('Ctrl Pts',(10.0514428414941,35.8062499998673,-1.23094673026484E-15));
#290561=CARTESIAN_POINT('Ctrl Pts',(10.0514428414941,35.9562499998667,-3.26591175476071));
#290562=CARTESIAN_POINT('Ctrl Pts',(8.13178807675716,36.1062499998661,-5.90808986649102));
#290563=CARTESIAN_POINT('Ctrl Pts',(6.21213331202018,36.2562499998655,-8.55026797822134));
#290564=CARTESIAN_POINT('Ctrl Pts',(3.10606665601007,36.4062499998649,-9.5594902125713));
#290565=CARTESIAN_POINT('Ctrl Pts',(-3.41776277664299E-14,36.5562499998642,
-10.5687124469213));
#290566=CARTESIAN_POINT('Ctrl Pts',(-3.10606665601014,36.7062499998636,
-9.5594902125713));
#290567=CARTESIAN_POINT('Ctrl Pts',(-6.21213331202025,36.856249999863,-8.55026797822134));
#290568=CARTESIAN_POINT('Ctrl Pts',(-8.13178807675722,37.0062499998624,
-5.90808986649102));
#290569=CARTESIAN_POINT('Ctrl Pts',(-10.0514428414942,37.1562499998618,
-3.2659117547607));
#290570=CARTESIAN_POINT('Ctrl Pts',(-10.0514428414942,37.3062499998613,
2.46189346052968E-15));
#290571=CARTESIAN_POINT('Ctrl Pts',(-10.0514428414942,37.4562499998606,
3.26591175476071));
#290572=CARTESIAN_POINT('Ctrl Pts',(-8.13178807675722,37.60624999986,5.90808986649102));
#290573=CARTESIAN_POINT('Ctrl Pts',(-6.21213331202025,37.7562499998594,
8.55026797822134));
#290574=CARTESIAN_POINT('Ctrl Pts',(-3.10606665601014,37.9062499998588,
9.5594902125713));
#290575=CARTESIAN_POINT('Ctrl Pts',(-3.24528944284146E-14,38.0562499998583,
10.5687124469213));
#290576=CARTESIAN_POINT('Ctrl Pts',(3.10606665601007,38.2062499998577,9.5594902125713));
#290577=CARTESIAN_POINT('Ctrl Pts',(6.21213331202018,38.3562499998571,8.55026797822134));
#290578=CARTESIAN_POINT('Ctrl Pts',(8.13178807675716,38.5062499998565,5.90808986649102));
#290579=CARTESIAN_POINT('Ctrl Pts',(10.0514428414941,38.6562499998559,3.2659117547607));
#290580=CARTESIAN_POINT('Ctrl Pts',(10.0514428414941,38.8062499998553,-1.23094673026484E-15));
#290581=CARTESIAN_POINT('Ctrl Pts',(10.0514428414941,35.4312499998688,-1.23094673026484E-15));
#290582=CARTESIAN_POINT('Ctrl Pts',(10.0514428414941,35.5812499998681,-3.26591175476071));
#290583=CARTESIAN_POINT('Ctrl Pts',(8.13178807675716,35.7312499998676,-5.90808986649102));
#290584=CARTESIAN_POINT('Ctrl Pts',(6.21213331202018,35.881249999867,-8.55026797822134));
#290585=CARTESIAN_POINT('Ctrl Pts',(3.10606665601007,36.0312499998664,-9.5594902125713));
#290586=CARTESIAN_POINT('Ctrl Pts',(-3.39616641074721E-14,36.1812499998658,
-10.5687124469213));
#290587=CARTESIAN_POINT('Ctrl Pts',(-3.10606665601014,36.3312499998652,
-9.5594902125713));
#290588=CARTESIAN_POINT('Ctrl Pts',(-6.21213331202025,36.4812499998645,
-8.55026797822134));
#290589=CARTESIAN_POINT('Ctrl Pts',(-8.13178807675722,36.6312499998639,
-5.90808986649102));
#290590=CARTESIAN_POINT('Ctrl Pts',(-10.0514428414942,36.7812499998633,
-3.2659117547607));
#290591=CARTESIAN_POINT('Ctrl Pts',(-10.0514428414942,36.9312499998627,
2.46189346052968E-15));
#290592=CARTESIAN_POINT('Ctrl Pts',(-10.0514428414942,37.0812499998621,
3.26591175476071));
#290593=CARTESIAN_POINT('Ctrl Pts',(-8.13178807675722,37.2312499998615,
5.90808986649102));
#290594=CARTESIAN_POINT('Ctrl Pts',(-6.21213331202025,37.3812499998609,
8.55026797822134));
#290595=CARTESIAN_POINT('Ctrl Pts',(-3.10606665601014,37.5312499998603,
9.5594902125713));
#290596=CARTESIAN_POINT('Ctrl Pts',(-3.22369307694568E-14,37.6812499998598,
10.5687124469213));
#290597=CARTESIAN_POINT('Ctrl Pts',(3.10606665601008,37.8312499998592,9.5594902125713));
#290598=CARTESIAN_POINT('Ctrl Pts',(6.21213331202018,37.9812499998586,8.55026797822134));
#290599=CARTESIAN_POINT('Ctrl Pts',(8.13178807675716,38.131249999858,5.90808986649102));
#290600=CARTESIAN_POINT('Ctrl Pts',(10.0514428414941,38.2812499998574,3.2659117547607));
#290601=CARTESIAN_POINT('Ctrl Pts',(10.0514428414941,38.4312499998568,-1.23094673026484E-15));
#290602=CARTESIAN_POINT('Origin',(-3.77475828372553E-14,-1.881249999982,
2.68644078414671E-15));
#290603=CARTESIAN_POINT('',(10.0514428414941,41.8062499998433,1.27413654429943E-15));
#290604=CARTESIAN_POINT('',(10.0514428414941,41.4312499998448,1.27569326111988E-15));
#290605=CARTESIAN_POINT('',(10.0514428414941,-1.881249999982,4.14193483802857E-15));
#290606=CARTESIAN_POINT('Ctrl Pts',(10.0514428414941,38.8062499998553,-1.23094673026484E-15));
#290607=CARTESIAN_POINT('Ctrl Pts',(10.0514428414941,38.9562499998547,-3.26591175476071));
#290608=CARTESIAN_POINT('Ctrl Pts',(8.13178807675715,39.1062499998541,-5.90808986649102));
#290609=CARTESIAN_POINT('Ctrl Pts',(6.21213331202018,39.2562499998535,-8.55026797822134));
#290610=CARTESIAN_POINT('Ctrl Pts',(3.10606665601007,39.4062499998529,-9.5594902125713));
#290611=CARTESIAN_POINT('Ctrl Pts',(-3.59053370380917E-14,39.5562499998522,
-10.5687124469213));
#290612=CARTESIAN_POINT('Ctrl Pts',(-3.10606665601014,39.7062499998516,
-9.5594902125713));
#290613=CARTESIAN_POINT('Ctrl Pts',(-6.21213331202025,39.856249999851,-8.55026797822134));
#290614=CARTESIAN_POINT('Ctrl Pts',(-8.13178807675723,40.0062499998505,
-5.90808986649102));
#290615=CARTESIAN_POINT('Ctrl Pts',(-10.0514428414942,40.1562499998499,
-3.2659117547607));
#290616=CARTESIAN_POINT('Ctrl Pts',(-10.0514428414942,40.3062499998493,
2.46189346052968E-15));
#290617=CARTESIAN_POINT('Ctrl Pts',(-10.0514428414942,40.4562499998487,
3.26591175476071));
#290618=CARTESIAN_POINT('Ctrl Pts',(-8.13178807675723,40.606249999848,5.90808986649102));
#290619=CARTESIAN_POINT('Ctrl Pts',(-6.21213331202025,40.7562499998474,
8.55026797822134));
#290620=CARTESIAN_POINT('Ctrl Pts',(-3.10606665601014,40.9062499998468,
9.5594902125713));
#290621=CARTESIAN_POINT('Ctrl Pts',(-3.41806037000764E-14,41.0562499998463,
10.5687124469213));
#290622=CARTESIAN_POINT('Ctrl Pts',(3.10606665601007,41.2062499998457,9.5594902125713));
#290623=CARTESIAN_POINT('Ctrl Pts',(6.21213331202018,41.3562499998451,8.55026797822134));
#290624=CARTESIAN_POINT('Ctrl Pts',(8.13178807675715,41.5062499998444,5.90808986649102));
#290625=CARTESIAN_POINT('Ctrl Pts',(10.0514428414941,41.6562499998439,3.2659117547607));
#290626=CARTESIAN_POINT('Ctrl Pts',(10.0514428414941,41.8062499998433,-1.23094673026484E-15));
#290627=CARTESIAN_POINT('Ctrl Pts',(10.0514428414941,38.4312499998568,-1.23094673026484E-15));
#290628=CARTESIAN_POINT('Ctrl Pts',(10.0514428414941,38.5812499998562,-3.26591175476071));
#290629=CARTESIAN_POINT('Ctrl Pts',(8.13178807675715,38.7312499998556,-5.90808986649102));
#290630=CARTESIAN_POINT('Ctrl Pts',(6.21213331202018,38.881249999855,-8.55026797822134));
#290631=CARTESIAN_POINT('Ctrl Pts',(3.10606665601007,39.0312499998544,-9.5594902125713));
#290632=CARTESIAN_POINT('Ctrl Pts',(-3.5689373379134E-14,39.1812499998537,
-10.5687124469213));
#290633=CARTESIAN_POINT('Ctrl Pts',(-3.10606665601014,39.3312499998532,
-9.5594902125713));
#290634=CARTESIAN_POINT('Ctrl Pts',(-6.21213331202025,39.4812499998525,
-8.55026797822134));
#290635=CARTESIAN_POINT('Ctrl Pts',(-8.13178807675723,39.6312499998519,
-5.90808986649102));
#290636=CARTESIAN_POINT('Ctrl Pts',(-10.0514428414942,39.7812499998513,
-3.2659117547607));
#290637=CARTESIAN_POINT('Ctrl Pts',(-10.0514428414942,39.9312499998507,
2.46189346052968E-15));
#290638=CARTESIAN_POINT('Ctrl Pts',(-10.0514428414942,40.0812499998501,
3.26591175476071));
#290639=CARTESIAN_POINT('Ctrl Pts',(-8.13178807675723,40.2312499998495,
5.90808986649102));
#290640=CARTESIAN_POINT('Ctrl Pts',(-6.21213331202025,40.3812499998489,
8.55026797822134));
#290641=CARTESIAN_POINT('Ctrl Pts',(-3.10606665601014,40.5312499998483,
9.5594902125713));
#290642=CARTESIAN_POINT('Ctrl Pts',(-3.39646400411187E-14,40.6812499998478,
10.5687124469213));
#290643=CARTESIAN_POINT('Ctrl Pts',(3.10606665601007,40.8312499998472,9.5594902125713));
#290644=CARTESIAN_POINT('Ctrl Pts',(6.21213331202018,40.9812499998465,8.55026797822134));
#290645=CARTESIAN_POINT('Ctrl Pts',(8.13178807675715,41.131249999846,5.90808986649102));
#290646=CARTESIAN_POINT('Ctrl Pts',(10.0514428414941,41.2812499998454,3.2659117547607));
#290647=CARTESIAN_POINT('Ctrl Pts',(10.0514428414941,41.4312499998448,-1.23094673026484E-15));
#290648=CARTESIAN_POINT('Origin',(-3.77475828372553E-14,-1.881249999982,
2.68644078414671E-15));
#290649=CARTESIAN_POINT('',(10.0514428414941,44.8062499998313,1.26168280973582E-15));
#290650=CARTESIAN_POINT('',(10.0514428414941,44.4312499998328,1.26323952655627E-15));
#290651=CARTESIAN_POINT('',(10.0514428414941,-1.881249999982,4.14193483802857E-15));
#290652=CARTESIAN_POINT('Ctrl Pts',(10.0514428414941,41.8062499998433,-1.23094673026484E-15));
#290653=CARTESIAN_POINT('Ctrl Pts',(10.0514428414941,41.9562499998427,-3.26591175476071));
#290654=CARTESIAN_POINT('Ctrl Pts',(8.13178807675715,42.1062499998421,-5.90808986649102));
#290655=CARTESIAN_POINT('Ctrl Pts',(6.21213331202018,42.2562499998415,-8.55026797822134));
#290656=CARTESIAN_POINT('Ctrl Pts',(3.10606665601007,42.4062499998408,-9.5594902125713));
#290657=CARTESIAN_POINT('Ctrl Pts',(-3.76330463097535E-14,42.5562499998402,
-10.5687124469213));
#290658=CARTESIAN_POINT('Ctrl Pts',(-3.10606665601015,42.7062499998396,
-9.5594902125713));
#290659=CARTESIAN_POINT('Ctrl Pts',(-6.21213331202025,42.8562499998391,
-8.55026797822134));
#290660=CARTESIAN_POINT('Ctrl Pts',(-8.13178807675723,43.0062499998385,
-5.90808986649102));
#290661=CARTESIAN_POINT('Ctrl Pts',(-10.0514428414942,43.1562499998379,
-3.2659117547607));
#290662=CARTESIAN_POINT('Ctrl Pts',(-10.0514428414942,43.3062499998373,
2.46189346052968E-15));
#290663=CARTESIAN_POINT('Ctrl Pts',(-10.0514428414942,43.4562499998366,
3.26591175476071));
#290664=CARTESIAN_POINT('Ctrl Pts',(-8.13178807675723,43.6062499998361,
5.90808986649102));
#290665=CARTESIAN_POINT('Ctrl Pts',(-6.21213331202025,43.7562499998354,
8.55026797822134));
#290666=CARTESIAN_POINT('Ctrl Pts',(-3.10606665601014,43.9062499998348,
9.5594902125713));
#290667=CARTESIAN_POINT('Ctrl Pts',(-3.59083129717383E-14,44.0562499998343,
10.5687124469213));
#290668=CARTESIAN_POINT('Ctrl Pts',(3.10606665601007,44.2062499998337,9.5594902125713));
#290669=CARTESIAN_POINT('Ctrl Pts',(6.21213331202018,44.356249999833,8.55026797822134));
#290670=CARTESIAN_POINT('Ctrl Pts',(8.13178807675715,44.5062499998324,5.90808986649102));
#290671=CARTESIAN_POINT('Ctrl Pts',(10.0514428414941,44.6562499998319,3.2659117547607));
#290672=CARTESIAN_POINT('Ctrl Pts',(10.0514428414941,44.8062499998313,-1.23094673026484E-15));
#290673=CARTESIAN_POINT('Ctrl Pts',(10.0514428414941,41.4312499998448,-1.23094673026484E-15));
#290674=CARTESIAN_POINT('Ctrl Pts',(10.0514428414941,41.5812499998442,-3.26591175476071));
#290675=CARTESIAN_POINT('Ctrl Pts',(8.13178807675715,41.7312499998436,-5.90808986649102));
#290676=CARTESIAN_POINT('Ctrl Pts',(6.21213331202018,41.881249999843,-8.55026797822134));
#290677=CARTESIAN_POINT('Ctrl Pts',(3.10606665601007,42.0312499998423,-9.5594902125713));
#290678=CARTESIAN_POINT('Ctrl Pts',(-3.74170826507958E-14,42.1812499998418,
-10.5687124469213));
#290679=CARTESIAN_POINT('Ctrl Pts',(-3.10606665601015,42.3312499998411,
-9.5594902125713));
#290680=CARTESIAN_POINT('Ctrl Pts',(-6.21213331202025,42.4812499998405,
-8.55026797822134));
#290681=CARTESIAN_POINT('Ctrl Pts',(-8.13178807675723,42.6312499998399,
-5.90808986649102));
#290682=CARTESIAN_POINT('Ctrl Pts',(-10.0514428414942,42.7812499998393,
-3.2659117547607));
#290683=CARTESIAN_POINT('Ctrl Pts',(-10.0514428414942,42.9312499998387,
2.46189346052968E-15));
#290684=CARTESIAN_POINT('Ctrl Pts',(-10.0514428414942,43.0812499998381,
3.26591175476071));
#290685=CARTESIAN_POINT('Ctrl Pts',(-8.13178807675723,43.2312499998375,
5.90808986649102));
#290686=CARTESIAN_POINT('Ctrl Pts',(-6.21213331202025,43.3812499998369,
8.55026797822134));
#290687=CARTESIAN_POINT('Ctrl Pts',(-3.10606665601014,43.5312499998363,
9.5594902125713));
#290688=CARTESIAN_POINT('Ctrl Pts',(-3.56923493127805E-14,43.6812499998357,
10.5687124469213));
#290689=CARTESIAN_POINT('Ctrl Pts',(3.10606665601007,43.8312499998352,9.5594902125713));
#290690=CARTESIAN_POINT('Ctrl Pts',(6.21213331202018,43.9812499998345,8.55026797822134));
#290691=CARTESIAN_POINT('Ctrl Pts',(8.13178807675715,44.131249999834,5.90808986649102));
#290692=CARTESIAN_POINT('Ctrl Pts',(10.0514428414941,44.2812499998334,3.2659117547607));
#290693=CARTESIAN_POINT('Ctrl Pts',(10.0514428414941,44.4312499998328,-1.23094673026484E-15));
#290694=CARTESIAN_POINT('Origin',(-3.77475828372553E-14,-1.881249999982,
2.68644078414671E-15));
#290695=CARTESIAN_POINT('',(10.0514428414941,47.8062499998193,1.24922907517222E-15));
#290696=CARTESIAN_POINT('',(10.0514428414941,47.4312499998208,1.25078579199267E-15));
#290697=CARTESIAN_POINT('',(10.0514428414941,-1.881249999982,4.14193483802857E-15));
#290698=CARTESIAN_POINT('Ctrl Pts',(10.0514428414941,44.8062499998313,-1.23094673026484E-15));
#290699=CARTESIAN_POINT('Ctrl Pts',(10.0514428414941,44.9562499998307,-3.26591175476071));
#290700=CARTESIAN_POINT('Ctrl Pts',(8.13178807675715,45.1062499998301,-5.90808986649102));
#290701=CARTESIAN_POINT('Ctrl Pts',(6.21213331202018,45.2562499998295,-8.55026797822134));
#290702=CARTESIAN_POINT('Ctrl Pts',(3.10606665601007,45.4062499998289,-9.5594902125713));
#290703=CARTESIAN_POINT('Ctrl Pts',(-3.93607555814154E-14,45.5562499998282,
-10.5687124469213));
#290704=CARTESIAN_POINT('Ctrl Pts',(-3.10606665601015,45.7062499998276,
-9.5594902125713));
#290705=CARTESIAN_POINT('Ctrl Pts',(-6.21213331202026,45.856249999827,-8.55026797822134));
#290706=CARTESIAN_POINT('Ctrl Pts',(-8.13178807675723,46.0062499998265,
-5.90808986649102));
#290707=CARTESIAN_POINT('Ctrl Pts',(-10.0514428414942,46.1562499998259,
-3.2659117547607));
#290708=CARTESIAN_POINT('Ctrl Pts',(-10.0514428414942,46.3062499998252,
2.46189346052968E-15));
#290709=CARTESIAN_POINT('Ctrl Pts',(-10.0514428414942,46.4562499998246,
3.26591175476071));
#290710=CARTESIAN_POINT('Ctrl Pts',(-8.13178807675723,46.606249999824,5.90808986649102));
#290711=CARTESIAN_POINT('Ctrl Pts',(-6.21213331202025,46.7562499998235,
8.55026797822134));
#290712=CARTESIAN_POINT('Ctrl Pts',(-3.10606665601015,46.9062499998228,
9.5594902125713));
#290713=CARTESIAN_POINT('Ctrl Pts',(-3.76360222434001E-14,47.0562499998223,
10.5687124469213));
#290714=CARTESIAN_POINT('Ctrl Pts',(3.10606665601007,47.2062499998217,9.5594902125713));
#290715=CARTESIAN_POINT('Ctrl Pts',(6.21213331202018,47.356249999821,8.55026797822134));
#290716=CARTESIAN_POINT('Ctrl Pts',(8.13178807675715,47.5062499998204,5.90808986649102));
#290717=CARTESIAN_POINT('Ctrl Pts',(10.0514428414941,47.6562499998198,3.2659117547607));
#290718=CARTESIAN_POINT('Ctrl Pts',(10.0514428414941,47.8062499998193,-1.23094673026484E-15));
#290719=CARTESIAN_POINT('Ctrl Pts',(10.0514428414941,44.4312499998328,-1.23094673026484E-15));
#290720=CARTESIAN_POINT('Ctrl Pts',(10.0514428414941,44.5812499998322,-3.26591175476071));
#290721=CARTESIAN_POINT('Ctrl Pts',(8.13178807675715,44.7312499998316,-5.90808986649102));
#290722=CARTESIAN_POINT('Ctrl Pts',(6.21213331202018,44.881249999831,-8.55026797822134));
#290723=CARTESIAN_POINT('Ctrl Pts',(3.10606665601007,45.0312499998304,-9.5594902125713));
#290724=CARTESIAN_POINT('Ctrl Pts',(-3.91447919224576E-14,45.1812499998297,
-10.5687124469213));
#290725=CARTESIAN_POINT('Ctrl Pts',(-3.10606665601015,45.3312499998292,
-9.5594902125713));
#290726=CARTESIAN_POINT('Ctrl Pts',(-6.21213331202026,45.4812499998285,
-8.55026797822134));
#290727=CARTESIAN_POINT('Ctrl Pts',(-8.13178807675723,45.6312499998279,
-5.90808986649102));
#290728=CARTESIAN_POINT('Ctrl Pts',(-10.0514428414942,45.7812499998273,
-3.2659117547607));
#290729=CARTESIAN_POINT('Ctrl Pts',(-10.0514428414942,45.9312499998267,
2.46189346052968E-15));
#290730=CARTESIAN_POINT('Ctrl Pts',(-10.0514428414942,46.0812499998261,
3.26591175476071));
#290731=CARTESIAN_POINT('Ctrl Pts',(-8.13178807675723,46.2312499998255,
5.90808986649102));
#290732=CARTESIAN_POINT('Ctrl Pts',(-6.21213331202025,46.3812499998249,
8.55026797822134));
#290733=CARTESIAN_POINT('Ctrl Pts',(-3.10606665601015,46.5312499998244,
9.5594902125713));
#290734=CARTESIAN_POINT('Ctrl Pts',(-3.74200585844424E-14,46.6812499998238,
10.5687124469213));
#290735=CARTESIAN_POINT('Ctrl Pts',(3.10606665601007,46.8312499998232,9.5594902125713));
#290736=CARTESIAN_POINT('Ctrl Pts',(6.21213331202018,46.9812499998225,8.55026797822134));
#290737=CARTESIAN_POINT('Ctrl Pts',(8.13178807675715,47.131249999822,5.90808986649102));
#290738=CARTESIAN_POINT('Ctrl Pts',(10.0514428414941,47.2812499998214,3.2659117547607));
#290739=CARTESIAN_POINT('Ctrl Pts',(10.0514428414941,47.4312499998208,-1.23094673026484E-15));
#290740=CARTESIAN_POINT('Origin',(-3.77475828372553E-14,-1.881249999982,
2.68644078414671E-15));
#290741=CARTESIAN_POINT('',(10.0514428414941,50.8062499998072,1.23677534060862E-15));
#290742=CARTESIAN_POINT('',(10.0514428414941,50.4312499998088,1.23833205742907E-15));
#290743=CARTESIAN_POINT('',(10.0514428414941,-1.881249999982,4.14193483802857E-15));
#290744=CARTESIAN_POINT('Ctrl Pts',(10.0514428414941,47.8062499998193,-1.23094673026484E-15));
#290745=CARTESIAN_POINT('Ctrl Pts',(10.0514428414941,47.9562499998187,-3.26591175476071));
#290746=CARTESIAN_POINT('Ctrl Pts',(8.13178807675715,48.1062499998181,-5.90808986649102));
#290747=CARTESIAN_POINT('Ctrl Pts',(6.21213331202018,48.2562499998174,-8.55026797822134));
#290748=CARTESIAN_POINT('Ctrl Pts',(3.10606665601007,48.4062499998169,-9.5594902125713));
#290749=CARTESIAN_POINT('Ctrl Pts',(-4.10884648530772E-14,48.5562499998163,
-10.5687124469213));
#290750=CARTESIAN_POINT('Ctrl Pts',(-3.10606665601015,48.7062499998157,
-9.5594902125713));
#290751=CARTESIAN_POINT('Ctrl Pts',(-6.21213331202026,48.8562499998151,
-8.55026797822134));
#290752=CARTESIAN_POINT('Ctrl Pts',(-8.13178807675723,49.0062499998145,
-5.90808986649102));
#290753=CARTESIAN_POINT('Ctrl Pts',(-10.0514428414942,49.1562499998139,
-3.2659117547607));
#290754=CARTESIAN_POINT('Ctrl Pts',(-10.0514428414942,49.3062499998132,
2.46189346052968E-15));
#290755=CARTESIAN_POINT('Ctrl Pts',(-10.0514428414942,49.4562499998126,
3.26591175476071));
#290756=CARTESIAN_POINT('Ctrl Pts',(-8.13178807675723,49.6062499998121,
5.90808986649102));
#290757=CARTESIAN_POINT('Ctrl Pts',(-6.21213331202025,49.7562499998114,
8.55026797822134));
#290758=CARTESIAN_POINT('Ctrl Pts',(-3.10606665601015,49.9062499998109,
9.5594902125713));
#290759=CARTESIAN_POINT('Ctrl Pts',(-3.9363731515062E-14,50.0562499998103,
10.5687124469213));
#290760=CARTESIAN_POINT('Ctrl Pts',(3.10606665601007,50.2062499998097,9.5594902125713));
#290761=CARTESIAN_POINT('Ctrl Pts',(6.21213331202018,50.3562499998091,8.55026797822134));
#290762=CARTESIAN_POINT('Ctrl Pts',(8.13178807675715,50.5062499998085,5.90808986649102));
#290763=CARTESIAN_POINT('Ctrl Pts',(10.0514428414941,50.6562499998078,3.2659117547607));
#290764=CARTESIAN_POINT('Ctrl Pts',(10.0514428414941,50.8062499998072,-1.23094673026484E-15));
#290765=CARTESIAN_POINT('Ctrl Pts',(10.0514428414941,47.4312499998208,-1.23094673026484E-15));
#290766=CARTESIAN_POINT('Ctrl Pts',(10.0514428414941,47.5812499998202,-3.26591175476071));
#290767=CARTESIAN_POINT('Ctrl Pts',(8.13178807675715,47.7312499998196,-5.90808986649102));
#290768=CARTESIAN_POINT('Ctrl Pts',(6.21213331202018,47.881249999819,-8.55026797822134));
#290769=CARTESIAN_POINT('Ctrl Pts',(3.10606665601007,48.0312499998184,-9.5594902125713));
#290770=CARTESIAN_POINT('Ctrl Pts',(-4.08725011941195E-14,48.1812499998178,
-10.5687124469213));
#290771=CARTESIAN_POINT('Ctrl Pts',(-3.10606665601015,48.3312499998172,
-9.5594902125713));
#290772=CARTESIAN_POINT('Ctrl Pts',(-6.21213331202026,48.4812499998166,
-8.55026797822134));
#290773=CARTESIAN_POINT('Ctrl Pts',(-8.13178807675723,48.6312499998159,
-5.90808986649102));
#290774=CARTESIAN_POINT('Ctrl Pts',(-10.0514428414942,48.7812499998153,
-3.2659117547607));
#290775=CARTESIAN_POINT('Ctrl Pts',(-10.0514428414942,48.9312499998147,
2.46189346052968E-15));
#290776=CARTESIAN_POINT('Ctrl Pts',(-10.0514428414942,49.0812499998141,
3.26591175476071));
#290777=CARTESIAN_POINT('Ctrl Pts',(-8.13178807675723,49.2312499998135,
5.90808986649102));
#290778=CARTESIAN_POINT('Ctrl Pts',(-6.21213331202025,49.3812499998129,
8.55026797822134));
#290779=CARTESIAN_POINT('Ctrl Pts',(-3.10606665601015,49.5312499998124,
9.5594902125713));
#290780=CARTESIAN_POINT('Ctrl Pts',(-3.91477678561042E-14,49.6812499998118,
10.5687124469213));
#290781=CARTESIAN_POINT('Ctrl Pts',(3.10606665601007,49.8312499998111,9.5594902125713));
#290782=CARTESIAN_POINT('Ctrl Pts',(6.21213331202018,49.9812499998106,8.55026797822134));
#290783=CARTESIAN_POINT('Ctrl Pts',(8.13178807675715,50.13124999981,5.90808986649102));
#290784=CARTESIAN_POINT('Ctrl Pts',(10.0514428414941,50.2812499998094,3.2659117547607));
#290785=CARTESIAN_POINT('Ctrl Pts',(10.0514428414941,50.4312499998088,-1.23094673026484E-15));
#290786=CARTESIAN_POINT('Origin',(-3.77475828372553E-14,-1.881249999982,
2.68644078414671E-15));
#290787=CARTESIAN_POINT('',(10.0514428414941,53.8062499997953,1.22432160604502E-15));
#290788=CARTESIAN_POINT('',(10.0514428414941,53.4312499997968,1.22587832286547E-15));
#290789=CARTESIAN_POINT('',(10.0514428414941,-1.881249999982,4.14193483802857E-15));
#290790=CARTESIAN_POINT('Ctrl Pts',(10.0514428414941,50.8062499998072,-1.23094673026484E-15));
#290791=CARTESIAN_POINT('Ctrl Pts',(10.0514428414941,50.9562499998067,-3.26591175476071));
#290792=CARTESIAN_POINT('Ctrl Pts',(8.13178807675715,51.1062499998061,-5.90808986649102));
#290793=CARTESIAN_POINT('Ctrl Pts',(6.21213331202017,51.2562499998054,-8.55026797822134));
#290794=CARTESIAN_POINT('Ctrl Pts',(3.10606665601006,51.4062499998048,-9.5594902125713));
#290795=CARTESIAN_POINT('Ctrl Pts',(-4.2816174124739E-14,51.5562499998043,
-10.5687124469213));
#290796=CARTESIAN_POINT('Ctrl Pts',(-3.10606665601015,51.7062499998037,
-9.5594902125713));
#290797=CARTESIAN_POINT('Ctrl Pts',(-6.21213331202026,51.856249999803,-8.55026797822134));
#290798=CARTESIAN_POINT('Ctrl Pts',(-8.13178807675723,52.0062499998025,
-5.90808986649102));
#290799=CARTESIAN_POINT('Ctrl Pts',(-10.0514428414942,52.1562499998019,
-3.2659117547607));
#290800=CARTESIAN_POINT('Ctrl Pts',(-10.0514428414942,52.3062499998012,
2.46189346052968E-15));
#290801=CARTESIAN_POINT('Ctrl Pts',(-10.0514428414942,52.4562499998006,
3.26591175476071));
#290802=CARTESIAN_POINT('Ctrl Pts',(-8.13178807675723,52.6062499998,5.90808986649102));
#290803=CARTESIAN_POINT('Ctrl Pts',(-6.21213331202026,52.7562499997994,
8.55026797822134));
#290804=CARTESIAN_POINT('Ctrl Pts',(-3.10606665601015,52.9062499997988,
9.5594902125713));
#290805=CARTESIAN_POINT('Ctrl Pts',(-4.10914407867238E-14,53.0562499997983,
10.5687124469213));
#290806=CARTESIAN_POINT('Ctrl Pts',(3.10606665601007,53.2062499997976,9.5594902125713));
#290807=CARTESIAN_POINT('Ctrl Pts',(6.21213331202018,53.356249999797,8.55026797822134));
#290808=CARTESIAN_POINT('Ctrl Pts',(8.13178807675715,53.5062499997965,5.90808986649102));
#290809=CARTESIAN_POINT('Ctrl Pts',(10.0514428414941,53.6562499997959,3.2659117547607));
#290810=CARTESIAN_POINT('Ctrl Pts',(10.0514428414941,53.8062499997953,-1.23094673026484E-15));
#290811=CARTESIAN_POINT('Ctrl Pts',(10.0514428414941,50.4312499998088,-1.23094673026484E-15));
#290812=CARTESIAN_POINT('Ctrl Pts',(10.0514428414941,50.5812499998082,-3.26591175476071));
#290813=CARTESIAN_POINT('Ctrl Pts',(8.13178807675715,50.7312499998076,-5.90808986649102));
#290814=CARTESIAN_POINT('Ctrl Pts',(6.21213331202017,50.881249999807,-8.55026797822134));
#290815=CARTESIAN_POINT('Ctrl Pts',(3.10606665601007,51.0312499998064,-9.5594902125713));
#290816=CARTESIAN_POINT('Ctrl Pts',(-4.26002104657813E-14,51.1812499998058,
-10.5687124469213));
#290817=CARTESIAN_POINT('Ctrl Pts',(-3.10606665601015,51.3312499998052,
-9.5594902125713));
#290818=CARTESIAN_POINT('Ctrl Pts',(-6.21213331202026,51.4812499998045,
-8.55026797822134));
#290819=CARTESIAN_POINT('Ctrl Pts',(-8.13178807675723,51.631249999804,-5.90808986649102));
#290820=CARTESIAN_POINT('Ctrl Pts',(-10.0514428414942,51.7812499998033,
-3.2659117547607));
#290821=CARTESIAN_POINT('Ctrl Pts',(-10.0514428414942,51.9312499998027,
2.46189346052968E-15));
#290822=CARTESIAN_POINT('Ctrl Pts',(-10.0514428414942,52.0812499998021,
3.26591175476071));
#290823=CARTESIAN_POINT('Ctrl Pts',(-8.13178807675723,52.2312499998015,
5.90808986649102));
#290824=CARTESIAN_POINT('Ctrl Pts',(-6.21213331202026,52.3812499998009,
8.55026797822134));
#290825=CARTESIAN_POINT('Ctrl Pts',(-3.10606665601015,52.5312499998004,
9.5594902125713));
#290826=CARTESIAN_POINT('Ctrl Pts',(-4.08754771277661E-14,52.6812499997997,
10.5687124469213));
#290827=CARTESIAN_POINT('Ctrl Pts',(3.10606665601007,52.8312499997991,9.5594902125713));
#290828=CARTESIAN_POINT('Ctrl Pts',(6.21213331202018,52.9812499997985,8.55026797822134));
#290829=CARTESIAN_POINT('Ctrl Pts',(8.13178807675715,53.131249999798,5.90808986649102));
#290830=CARTESIAN_POINT('Ctrl Pts',(10.0514428414941,53.2812499997974,3.2659117547607));
#290831=CARTESIAN_POINT('Ctrl Pts',(10.0514428414941,53.4312499997968,-1.23094673026484E-15));
#290832=CARTESIAN_POINT('Origin',(-3.77475828372553E-14,-1.881249999982,
2.68644078414671E-15));
#290833=CARTESIAN_POINT('',(10.0514428414941,56.8062499997833,1.21186787148142E-15));
#290834=CARTESIAN_POINT('',(10.0514428414941,56.4312499997848,1.21342458830187E-15));
#290835=CARTESIAN_POINT('',(10.0514428414941,-1.881249999982,4.14193483802857E-15));
#290836=CARTESIAN_POINT('Ctrl Pts',(10.0514428414941,53.8062499997953,-1.23094673026484E-15));
#290837=CARTESIAN_POINT('Ctrl Pts',(10.0514428414941,53.9562499997946,-3.26591175476071));
#290838=CARTESIAN_POINT('Ctrl Pts',(8.13178807675714,54.106249999794,-5.90808986649102));
#290839=CARTESIAN_POINT('Ctrl Pts',(6.21213331202017,54.2562499997934,-8.55026797822134));
#290840=CARTESIAN_POINT('Ctrl Pts',(3.10606665601006,54.4062499997928,-9.5594902125713));
#290841=CARTESIAN_POINT('Ctrl Pts',(-4.45438833964009E-14,54.5562499997923,
-10.5687124469213));
#290842=CARTESIAN_POINT('Ctrl Pts',(-3.10606665601015,54.7062499997917,
-9.5594902125713));
#290843=CARTESIAN_POINT('Ctrl Pts',(-6.21213331202026,54.856249999791,-8.55026797822134));
#290844=CARTESIAN_POINT('Ctrl Pts',(-8.13178807675724,55.0062499997905,
-5.90808986649102));
#290845=CARTESIAN_POINT('Ctrl Pts',(-10.0514428414942,55.1562499997898,
-3.2659117547607));
#290846=CARTESIAN_POINT('Ctrl Pts',(-10.0514428414942,55.3062499997893,
2.46189346052968E-15));
#290847=CARTESIAN_POINT('Ctrl Pts',(-10.0514428414942,55.4562499997886,
3.26591175476071));
#290848=CARTESIAN_POINT('Ctrl Pts',(-8.13178807675724,55.606249999788,5.90808986649102));
#290849=CARTESIAN_POINT('Ctrl Pts',(-6.21213331202026,55.7562499997874,
8.55026797822134));
#290850=CARTESIAN_POINT('Ctrl Pts',(-3.10606665601015,55.9062499997869,
9.5594902125713));
#290851=CARTESIAN_POINT('Ctrl Pts',(-4.28191500583856E-14,56.0562499997862,
10.5687124469213));
#290852=CARTESIAN_POINT('Ctrl Pts',(3.10606665601006,56.2062499997857,9.5594902125713));
#290853=CARTESIAN_POINT('Ctrl Pts',(6.21213331202017,56.356249999785,8.55026797822134));
#290854=CARTESIAN_POINT('Ctrl Pts',(8.13178807675714,56.5062499997845,5.90808986649102));
#290855=CARTESIAN_POINT('Ctrl Pts',(10.0514428414941,56.6562499997839,3.2659117547607));
#290856=CARTESIAN_POINT('Ctrl Pts',(10.0514428414941,56.8062499997833,-1.23094673026484E-15));
#290857=CARTESIAN_POINT('Ctrl Pts',(10.0514428414941,53.4312499997968,-1.23094673026484E-15));
#290858=CARTESIAN_POINT('Ctrl Pts',(10.0514428414941,53.5812499997962,-3.26591175476071));
#290859=CARTESIAN_POINT('Ctrl Pts',(8.13178807675714,53.7312499997956,-5.90808986649102));
#290860=CARTESIAN_POINT('Ctrl Pts',(6.21213331202017,53.881249999795,-8.55026797822134));
#290861=CARTESIAN_POINT('Ctrl Pts',(3.10606665601006,54.0312499997944,-9.5594902125713));
#290862=CARTESIAN_POINT('Ctrl Pts',(-4.43279197374432E-14,54.1812499997938,
-10.5687124469213));
#290863=CARTESIAN_POINT('Ctrl Pts',(-3.10606665601015,54.3312499997932,
-9.5594902125713));
#290864=CARTESIAN_POINT('Ctrl Pts',(-6.21213331202026,54.4812499997926,
-8.55026797822134));
#290865=CARTESIAN_POINT('Ctrl Pts',(-8.13178807675724,54.6312499997919,
-5.90808986649102));
#290866=CARTESIAN_POINT('Ctrl Pts',(-10.0514428414942,54.7812499997913,
-3.2659117547607));
#290867=CARTESIAN_POINT('Ctrl Pts',(-10.0514428414942,54.9312499997907,
2.46189346052968E-15));
#290868=CARTESIAN_POINT('Ctrl Pts',(-10.0514428414942,55.0812499997901,
3.26591175476071));
#290869=CARTESIAN_POINT('Ctrl Pts',(-8.13178807675724,55.2312499997895,
5.90808986649102));
#290870=CARTESIAN_POINT('Ctrl Pts',(-6.21213331202026,55.3812499997889,
8.55026797822134));
#290871=CARTESIAN_POINT('Ctrl Pts',(-3.10606665601015,55.5312499997884,
9.5594902125713));
#290872=CARTESIAN_POINT('Ctrl Pts',(-4.26031863994279E-14,55.6812499997877,
10.5687124469213));
#290873=CARTESIAN_POINT('Ctrl Pts',(3.10606665601006,55.8312499997871,9.5594902125713));
#290874=CARTESIAN_POINT('Ctrl Pts',(6.21213331202017,55.9812499997865,8.55026797822134));
#290875=CARTESIAN_POINT('Ctrl Pts',(8.13178807675714,56.131249999786,5.90808986649102));
#290876=CARTESIAN_POINT('Ctrl Pts',(10.0514428414941,56.2812499997854,3.2659117547607));
#290877=CARTESIAN_POINT('Ctrl Pts',(10.0514428414941,56.4312499997848,-1.23094673026484E-15));
#290878=CARTESIAN_POINT('Origin',(-3.77475828372553E-14,-1.881249999982,
2.68644078414671E-15));
#290879=CARTESIAN_POINT('',(10.0514428414941,59.8062499997713,1.19941413691782E-15));
#290880=CARTESIAN_POINT('',(10.0514428414941,59.4312499997728,1.20097085373827E-15));
#290881=CARTESIAN_POINT('',(10.0514428414941,-1.881249999982,4.14193483802857E-15));
#290882=CARTESIAN_POINT('Ctrl Pts',(10.0514428414941,56.8062499997833,-1.23094673026484E-15));
#290883=CARTESIAN_POINT('Ctrl Pts',(10.0514428414941,56.9562499997827,-3.26591175476071));
#290884=CARTESIAN_POINT('Ctrl Pts',(8.13178807675714,57.1062499997821,-5.90808986649102));
#290885=CARTESIAN_POINT('Ctrl Pts',(6.21213331202017,57.2562499997814,-8.55026797822134));
#290886=CARTESIAN_POINT('Ctrl Pts',(3.10606665601006,57.4062499997808,-9.5594902125713));
#290887=CARTESIAN_POINT('Ctrl Pts',(-4.62715926680627E-14,57.5562499997802,
-10.5687124469213));
#290888=CARTESIAN_POINT('Ctrl Pts',(-3.10606665601015,57.7062499997797,
-9.5594902125713));
#290889=CARTESIAN_POINT('Ctrl Pts',(-6.21213331202026,57.856249999779,-8.55026797822134));
#290890=CARTESIAN_POINT('Ctrl Pts',(-8.13178807675724,58.0062499997784,
-5.90808986649102));
#290891=CARTESIAN_POINT('Ctrl Pts',(-10.0514428414942,58.1562499997778,
-3.2659117547607));
#290892=CARTESIAN_POINT('Ctrl Pts',(-10.0514428414942,58.3062499997773,
2.46189346052968E-15));
#290893=CARTESIAN_POINT('Ctrl Pts',(-10.0514428414942,58.4562499997766,
3.26591175476071));
#290894=CARTESIAN_POINT('Ctrl Pts',(-8.13178807675724,58.6062499997761,
5.90808986649102));
#290895=CARTESIAN_POINT('Ctrl Pts',(-6.21213331202026,58.7562499997754,
8.55026797822134));
#290896=CARTESIAN_POINT('Ctrl Pts',(-3.10606665601015,58.9062499997749,
9.5594902125713));
#290897=CARTESIAN_POINT('Ctrl Pts',(-4.45468593300475E-14,59.0562499997742,
10.5687124469213));
#290898=CARTESIAN_POINT('Ctrl Pts',(3.10606665601006,59.2062499997736,9.5594902125713));
#290899=CARTESIAN_POINT('Ctrl Pts',(6.21213331202017,59.356249999773,8.55026797822134));
#290900=CARTESIAN_POINT('Ctrl Pts',(8.13178807675714,59.5062499997725,5.90808986649102));
#290901=CARTESIAN_POINT('Ctrl Pts',(10.0514428414941,59.6562499997719,3.2659117547607));
#290902=CARTESIAN_POINT('Ctrl Pts',(10.0514428414941,59.8062499997713,-1.23094673026484E-15));
#290903=CARTESIAN_POINT('Ctrl Pts',(10.0514428414941,56.4312499997848,-1.23094673026484E-15));
#290904=CARTESIAN_POINT('Ctrl Pts',(10.0514428414941,56.5812499997842,-3.26591175476071));
#290905=CARTESIAN_POINT('Ctrl Pts',(8.13178807675714,56.7312499997836,-5.90808986649102));
#290906=CARTESIAN_POINT('Ctrl Pts',(6.21213331202017,56.881249999783,-8.55026797822134));
#290907=CARTESIAN_POINT('Ctrl Pts',(3.10606665601006,57.0312499997824,-9.5594902125713));
#290908=CARTESIAN_POINT('Ctrl Pts',(-4.6055629009105E-14,57.1812499997818,
-10.5687124469213));
#290909=CARTESIAN_POINT('Ctrl Pts',(-3.10606665601015,57.3312499997812,
-9.5594902125713));
#290910=CARTESIAN_POINT('Ctrl Pts',(-6.21213331202026,57.4812499997805,
-8.55026797822134));
#290911=CARTESIAN_POINT('Ctrl Pts',(-8.13178807675724,57.6312499997799,
-5.90808986649102));
#290912=CARTESIAN_POINT('Ctrl Pts',(-10.0514428414942,57.7812499997793,
-3.2659117547607));
#290913=CARTESIAN_POINT('Ctrl Pts',(-10.0514428414942,57.9312499997787,
2.46189346052968E-15));
#290914=CARTESIAN_POINT('Ctrl Pts',(-10.0514428414942,58.0812499997781,
3.26591175476071));
#290915=CARTESIAN_POINT('Ctrl Pts',(-8.13178807675724,58.2312499997775,
5.90808986649102));
#290916=CARTESIAN_POINT('Ctrl Pts',(-6.21213331202026,58.3812499997769,
8.55026797822134));
#290917=CARTESIAN_POINT('Ctrl Pts',(-3.10606665601015,58.5312499997763,
9.5594902125713));
#290918=CARTESIAN_POINT('Ctrl Pts',(-4.43308956710897E-14,58.6812499997757,
10.5687124469213));
#290919=CARTESIAN_POINT('Ctrl Pts',(3.10606665601006,58.8312499997751,9.5594902125713));
#290920=CARTESIAN_POINT('Ctrl Pts',(6.21213331202017,58.9812499997745,8.55026797822134));
#290921=CARTESIAN_POINT('Ctrl Pts',(8.13178807675714,59.131249999774,5.90808986649102));
#290922=CARTESIAN_POINT('Ctrl Pts',(10.0514428414941,59.2812499997734,3.2659117547607));
#290923=CARTESIAN_POINT('Ctrl Pts',(10.0514428414941,59.4312499997728,-1.23094673026484E-15));
#290924=CARTESIAN_POINT('Origin',(-3.77475828372553E-14,-1.881249999982,
2.68644078414671E-15));
#290925=CARTESIAN_POINT('',(10.0514428414941,92.8062499996392,1.0624230567182E-15));
#290926=CARTESIAN_POINT('',(10.0514428414941,92.4312499996408,1.06397977353865E-15));
#290927=CARTESIAN_POINT('',(10.0514428414941,-1.881249999982,4.14193483802857E-15));
#290928=CARTESIAN_POINT('',(-9.73188510064473,91.186,-2.51434197826683));
#290929=CARTESIAN_POINT('Ctrl Pts',(-9.73188510064473,91.186,-2.51434197826683));
#290930=CARTESIAN_POINT('Ctrl Pts',(-10.0514428414942,91.2475767399999,
-1.27747792244231));
#290931=CARTESIAN_POINT('Ctrl Pts',(-10.0514428414942,91.3062499996452,
2.46189346052968E-15));
#290932=CARTESIAN_POINT('Ctrl Pts',(-10.0514428414942,91.4562499996446,
3.26591175476071));
#290933=CARTESIAN_POINT('Ctrl Pts',(-8.13178807675726,91.606249999644,5.90808986649102));
#290934=CARTESIAN_POINT('Ctrl Pts',(-6.21213331202028,91.7562499996434,
8.55026797822134));
#290935=CARTESIAN_POINT('Ctrl Pts',(-3.10606665601017,91.9062499996429,
9.5594902125713));
#290936=CARTESIAN_POINT('Ctrl Pts',(-6.35516613183277E-14,92.0562499996422,
10.5687124469213));
#290937=CARTESIAN_POINT('Ctrl Pts',(3.10606665601004,92.2062499996417,9.5594902125713));
#290938=CARTESIAN_POINT('Ctrl Pts',(6.21213331202015,92.3562499996411,8.55026797822134));
#290939=CARTESIAN_POINT('Ctrl Pts',(8.13178807675712,92.5062499996404,5.90808986649102));
#290940=CARTESIAN_POINT('Ctrl Pts',(10.0514428414941,92.6562499996398,3.2659117547607));
#290941=CARTESIAN_POINT('Ctrl Pts',(10.0514428414941,92.8062499996392,-1.23094673026484E-15));
#290942=CARTESIAN_POINT('',(-8.66397270809404,91.1859999999999,5.09579043026958));
#290943=CARTESIAN_POINT('Origin',(-3.77475828372553E-14,91.186,1.91375089876756E-15));
#290944=CARTESIAN_POINT('Ctrl Pts',(-8.66397270809405,91.1859999999999,
5.09579043026958));
#290945=CARTESIAN_POINT('Ctrl Pts',(-8.41752315772121,91.2089229318145,
5.51480926700787));
#290946=CARTESIAN_POINT('Ctrl Pts',(-8.13178807675726,91.2312499996455,
5.90808986649102));
#290947=CARTESIAN_POINT('Ctrl Pts',(-6.21213331202028,91.381249999645,8.55026797822134));
#290948=CARTESIAN_POINT('Ctrl Pts',(-3.10606665601017,91.5312499996443,
9.5594902125713));
#290949=CARTESIAN_POINT('Ctrl Pts',(-6.333569765937E-14,91.6812499996438,
10.5687124469213));
#290950=CARTESIAN_POINT('Ctrl Pts',(3.10606665601004,91.8312499996431,9.5594902125713));
#290951=CARTESIAN_POINT('Ctrl Pts',(6.21213331202015,91.9812499996426,8.55026797822134));
#290952=CARTESIAN_POINT('Ctrl Pts',(8.13178807675712,92.131249999642,5.90808986649102));
#290953=CARTESIAN_POINT('Ctrl Pts',(10.0514428414941,92.2812499996413,3.2659117547607));
#290954=CARTESIAN_POINT('Ctrl Pts',(10.0514428414941,92.4312499996408,-1.23094673026484E-15));
#290955=CARTESIAN_POINT('Origin',(-3.77475828372553E-14,-1.881249999982,
2.68644078414671E-15));
#290956=CARTESIAN_POINT('',(10.0514428414941,95.8062499996273,1.0499693221546E-15));
#290957=CARTESIAN_POINT('',(10.0514428414941,95.4312499996288,1.05152603897505E-15));
#290958=CARTESIAN_POINT('',(10.0514428414941,-1.881249999982,4.14193483802857E-15));
#290959=CARTESIAN_POINT('Ctrl Pts',(10.0514428414941,92.8062499996392,-1.23094673026484E-15));
#290960=CARTESIAN_POINT('Ctrl Pts',(10.0514428414941,92.9562499996387,-3.26591175476071));
#290961=CARTESIAN_POINT('Ctrl Pts',(8.13178807675712,93.1062499996381,-5.90808986649102));
#290962=CARTESIAN_POINT('Ctrl Pts',(6.21213331202015,93.2562499996374,-8.55026797822134));
#290963=CARTESIAN_POINT('Ctrl Pts',(3.10606665601004,93.4062499996369,-9.5594902125713));
#290964=CARTESIAN_POINT('Ctrl Pts',(-6.70041039280048E-14,93.5562499996362,
-10.5687124469213));
#290965=CARTESIAN_POINT('Ctrl Pts',(-3.10606665601018,93.7062499996357,
-9.5594902125713));
#290966=CARTESIAN_POINT('Ctrl Pts',(-6.21213331202028,93.856249999635,-8.55026797822134));
#290967=CARTESIAN_POINT('Ctrl Pts',(-8.13178807675726,94.0062499996344,
-5.90808986649102));
#290968=CARTESIAN_POINT('Ctrl Pts',(-10.0514428414942,94.1562499996338,
-3.2659117547607));
#290969=CARTESIAN_POINT('Ctrl Pts',(-10.0514428414942,94.3062499996333,
2.46189346052968E-15));
#290970=CARTESIAN_POINT('Ctrl Pts',(-10.0514428414942,94.4562499996326,
3.26591175476071));
#290971=CARTESIAN_POINT('Ctrl Pts',(-8.13178807675726,94.606249999632,5.90808986649102));
#290972=CARTESIAN_POINT('Ctrl Pts',(-6.21213331202028,94.7562499996315,
8.55026797822134));
#290973=CARTESIAN_POINT('Ctrl Pts',(-3.10606665601017,94.9062499996309,
9.5594902125713));
#290974=CARTESIAN_POINT('Ctrl Pts',(-6.52793705899895E-14,95.0562499996302,
10.5687124469213));
#290975=CARTESIAN_POINT('Ctrl Pts',(3.10606665601004,95.2062499996296,9.5594902125713));
#290976=CARTESIAN_POINT('Ctrl Pts',(6.21213331202015,95.3562499996291,8.55026797822134));
#290977=CARTESIAN_POINT('Ctrl Pts',(8.13178807675712,95.5062499996285,5.90808986649102));
#290978=CARTESIAN_POINT('Ctrl Pts',(10.0514428414941,95.6562499996278,3.2659117547607));
#290979=CARTESIAN_POINT('Ctrl Pts',(10.0514428414941,95.8062499996273,-1.23094673026484E-15));
#290980=CARTESIAN_POINT('Ctrl Pts',(10.0514428414941,92.4312499996408,-1.23094673026484E-15));
#290981=CARTESIAN_POINT('Ctrl Pts',(10.0514428414941,92.5812499996402,-3.26591175476071));
#290982=CARTESIAN_POINT('Ctrl Pts',(8.13178807675712,92.7312499996396,-5.90808986649102));
#290983=CARTESIAN_POINT('Ctrl Pts',(6.21213331202015,92.8812499996389,-8.55026797822134));
#290984=CARTESIAN_POINT('Ctrl Pts',(3.10606665601004,93.0312499996383,-9.5594902125713));
#290985=CARTESIAN_POINT('Ctrl Pts',(-6.67881402690471E-14,93.1812499996377,
-10.5687124469213));
#290986=CARTESIAN_POINT('Ctrl Pts',(-3.10606665601018,93.3312499996371,
-9.5594902125713));
#290987=CARTESIAN_POINT('Ctrl Pts',(-6.21213331202028,93.4812499996365,
-8.55026797822134));
#290988=CARTESIAN_POINT('Ctrl Pts',(-8.13178807675726,93.6312499996359,
-5.90808986649102));
#290989=CARTESIAN_POINT('Ctrl Pts',(-10.0514428414942,93.7812499996353,
-3.2659117547607));
#290990=CARTESIAN_POINT('Ctrl Pts',(-10.0514428414942,93.9312499996347,
2.46189346052968E-15));
#290991=CARTESIAN_POINT('Ctrl Pts',(-10.0514428414942,94.0812499996341,
3.26591175476071));
#290992=CARTESIAN_POINT('Ctrl Pts',(-8.13178807675726,94.2312499996335,
5.90808986649102));
#290993=CARTESIAN_POINT('Ctrl Pts',(-6.21213331202028,94.3812499996329,
8.55026797822134));
#290994=CARTESIAN_POINT('Ctrl Pts',(-3.10606665601017,94.5312499996324,
9.5594902125713));
#290995=CARTESIAN_POINT('Ctrl Pts',(-6.50634069310318E-14,94.6812499996317,
10.5687124469213));
#290996=CARTESIAN_POINT('Ctrl Pts',(3.10606665601004,94.8312499996312,9.5594902125713));
#290997=CARTESIAN_POINT('Ctrl Pts',(6.21213331202015,94.9812499996305,8.55026797822134));
#290998=CARTESIAN_POINT('Ctrl Pts',(8.13178807675712,95.13124999963,5.90808986649102));
#290999=CARTESIAN_POINT('Ctrl Pts',(10.0514428414941,95.2812499996293,3.2659117547607));
#291000=CARTESIAN_POINT('Ctrl Pts',(10.0514428414941,95.4312499996288,-1.23094673026484E-15));
#291001=CARTESIAN_POINT('Origin',(-3.77475828372553E-14,-1.881249999982,
2.68644078414671E-15));
#291002=CARTESIAN_POINT('',(10.0514428414941,98.8062499996153,1.037515587591E-15));
#291003=CARTESIAN_POINT('',(10.0514428414941,98.4312499996168,1.03907230441145E-15));
#291004=CARTESIAN_POINT('',(10.0514428414941,-1.881249999982,4.14193483802857E-15));
#291005=CARTESIAN_POINT('Ctrl Pts',(10.0514428414941,95.8062499996273,-1.23094673026484E-15));
#291006=CARTESIAN_POINT('Ctrl Pts',(10.0514428414941,95.9562499996266,-3.26591175476071));
#291007=CARTESIAN_POINT('Ctrl Pts',(8.13178807675712,96.1062499996261,-5.90808986649102));
#291008=CARTESIAN_POINT('Ctrl Pts',(6.21213331202015,96.2562499996255,-8.55026797822134));
#291009=CARTESIAN_POINT('Ctrl Pts',(3.10606665601004,96.4062499996248,-9.5594902125713));
#291010=CARTESIAN_POINT('Ctrl Pts',(-6.87318131996666E-14,96.5562499996243,
-10.5687124469213));
#291011=CARTESIAN_POINT('Ctrl Pts',(-3.10606665601018,96.7062499996236,
-9.5594902125713));
#291012=CARTESIAN_POINT('Ctrl Pts',(-6.21213331202028,96.856249999623,-8.55026797822134));
#291013=CARTESIAN_POINT('Ctrl Pts',(-8.13178807675726,97.0062499996224,
-5.90808986649102));
#291014=CARTESIAN_POINT('Ctrl Pts',(-10.0514428414942,97.1562499996218,
-3.2659117547607));
#291015=CARTESIAN_POINT('Ctrl Pts',(-10.0514428414942,97.3062499996212,
2.46189346052968E-15));
#291016=CARTESIAN_POINT('Ctrl Pts',(-10.0514428414942,97.4562499996206,
3.26591175476071));
#291017=CARTESIAN_POINT('Ctrl Pts',(-8.13178807675726,97.60624999962,5.90808986649102));
#291018=CARTESIAN_POINT('Ctrl Pts',(-6.21213331202028,97.7562499996194,
8.55026797822134));
#291019=CARTESIAN_POINT('Ctrl Pts',(-3.10606665601018,97.9062499996189,
9.5594902125713));
#291020=CARTESIAN_POINT('Ctrl Pts',(-6.70070798616514E-14,98.0562499996182,
10.5687124469213));
#291021=CARTESIAN_POINT('Ctrl Pts',(3.10606665601004,98.2062499996177,9.5594902125713));
#291022=CARTESIAN_POINT('Ctrl Pts',(6.21213331202015,98.3562499996171,8.55026797822134));
#291023=CARTESIAN_POINT('Ctrl Pts',(8.13178807675712,98.5062499996165,5.90808986649102));
#291024=CARTESIAN_POINT('Ctrl Pts',(10.0514428414941,98.6562499996158,3.2659117547607));
#291025=CARTESIAN_POINT('Ctrl Pts',(10.0514428414941,98.8062499996153,-1.23094673026484E-15));
#291026=CARTESIAN_POINT('Ctrl Pts',(10.0514428414941,95.4312499996288,-1.23094673026484E-15));
#291027=CARTESIAN_POINT('Ctrl Pts',(10.0514428414941,95.5812499996282,-3.26591175476071));
#291028=CARTESIAN_POINT('Ctrl Pts',(8.13178807675712,95.7312499996276,-5.90808986649102));
#291029=CARTESIAN_POINT('Ctrl Pts',(6.21213331202015,95.8812499996269,-8.55026797822134));
#291030=CARTESIAN_POINT('Ctrl Pts',(3.10606665601004,96.0312499996264,-9.5594902125713));
#291031=CARTESIAN_POINT('Ctrl Pts',(-6.85158495407089E-14,96.1812499996257,
-10.5687124469213));
#291032=CARTESIAN_POINT('Ctrl Pts',(-3.10606665601018,96.3312499996252,
-9.5594902125713));
#291033=CARTESIAN_POINT('Ctrl Pts',(-6.21213331202028,96.4812499996245,
-8.55026797822134));
#291034=CARTESIAN_POINT('Ctrl Pts',(-8.13178807675726,96.6312499996239,
-5.90808986649102));
#291035=CARTESIAN_POINT('Ctrl Pts',(-10.0514428414942,96.7812499996234,
-3.2659117547607));
#291036=CARTESIAN_POINT('Ctrl Pts',(-10.0514428414942,96.9312499996227,
2.46189346052968E-15));
#291037=CARTESIAN_POINT('Ctrl Pts',(-10.0514428414942,97.0812499996221,
3.26591175476071));
#291038=CARTESIAN_POINT('Ctrl Pts',(-8.13178807675726,97.2312499996215,
5.90808986649102));
#291039=CARTESIAN_POINT('Ctrl Pts',(-6.21213331202028,97.381249999621,8.55026797822134));
#291040=CARTESIAN_POINT('Ctrl Pts',(-3.10606665601017,97.5312499996203,
9.5594902125713));
#291041=CARTESIAN_POINT('Ctrl Pts',(-6.67911162026936E-14,97.6812499996198,
10.5687124469213));
#291042=CARTESIAN_POINT('Ctrl Pts',(3.10606665601004,97.8312499996191,9.5594902125713));
#291043=CARTESIAN_POINT('Ctrl Pts',(6.21213331202015,97.9812499996186,8.55026797822134));
#291044=CARTESIAN_POINT('Ctrl Pts',(8.13178807675712,98.1312499996179,5.90808986649102));
#291045=CARTESIAN_POINT('Ctrl Pts',(10.0514428414941,98.2812499996173,3.2659117547607));
#291046=CARTESIAN_POINT('Ctrl Pts',(10.0514428414941,98.4312499996168,-1.23094673026484E-15));
#291047=CARTESIAN_POINT('Origin',(-3.77475828372553E-14,-1.881249999982,
2.68644078414671E-15));
#291048=CARTESIAN_POINT('',(10.0514428414941,101.806249999603,1.0250618530274E-15));
#291049=CARTESIAN_POINT('',(10.0514428414941,101.431249999605,1.02661856984785E-15));
#291050=CARTESIAN_POINT('',(10.0514428414941,-1.881249999982,4.14193483802857E-15));
#291051=CARTESIAN_POINT('Ctrl Pts',(10.0514428414941,98.8062499996153,-1.23094673026484E-15));
#291052=CARTESIAN_POINT('Ctrl Pts',(10.0514428414941,98.9562499996147,-3.26591175476071));
#291053=CARTESIAN_POINT('Ctrl Pts',(8.13178807675712,99.1062499996141,-5.90808986649102));
#291054=CARTESIAN_POINT('Ctrl Pts',(6.21213331202014,99.2562499996134,-8.55026797822134));
#291055=CARTESIAN_POINT('Ctrl Pts',(3.10606665601004,99.4062499996129,-9.5594902125713));
#291056=CARTESIAN_POINT('Ctrl Pts',(-7.04595224713285E-14,99.5562499996122,
-10.5687124469213));
#291057=CARTESIAN_POINT('Ctrl Pts',(-3.10606665601018,99.7062499996117,
-9.5594902125713));
#291058=CARTESIAN_POINT('Ctrl Pts',(-6.21213331202029,99.856249999611,-8.55026797822134));
#291059=CARTESIAN_POINT('Ctrl Pts',(-8.13178807675726,100.00624999961,-5.90808986649102));
#291060=CARTESIAN_POINT('Ctrl Pts',(-10.0514428414942,100.15624999961,-3.2659117547607));
#291061=CARTESIAN_POINT('Ctrl Pts',(-10.0514428414942,100.306249999609,
2.46189346052968E-15));
#291062=CARTESIAN_POINT('Ctrl Pts',(-10.0514428414942,100.456249999609,
3.26591175476071));
#291063=CARTESIAN_POINT('Ctrl Pts',(-8.13178807675726,100.606249999608,
5.90808986649102));
#291064=CARTESIAN_POINT('Ctrl Pts',(-6.21213331202028,100.756249999607,
8.55026797822134));
#291065=CARTESIAN_POINT('Ctrl Pts',(-3.10606665601018,100.906249999607,
9.5594902125713));
#291066=CARTESIAN_POINT('Ctrl Pts',(-6.87347891333132E-14,101.056249999606,
10.5687124469213));
#291067=CARTESIAN_POINT('Ctrl Pts',(3.10606665601004,101.206249999606,9.5594902125713));
#291068=CARTESIAN_POINT('Ctrl Pts',(6.21213331202015,101.356249999605,8.55026797822134));
#291069=CARTESIAN_POINT('Ctrl Pts',(8.13178807675712,101.506249999604,5.90808986649102));
#291070=CARTESIAN_POINT('Ctrl Pts',(10.0514428414941,101.656249999604,3.2659117547607));
#291071=CARTESIAN_POINT('Ctrl Pts',(10.0514428414941,101.806249999603,-1.23094673026484E-15));
#291072=CARTESIAN_POINT('Ctrl Pts',(10.0514428414941,98.4312499996168,-1.23094673026484E-15));
#291073=CARTESIAN_POINT('Ctrl Pts',(10.0514428414941,98.5812499996162,-3.26591175476071));
#291074=CARTESIAN_POINT('Ctrl Pts',(8.13178807675712,98.7312499996156,-5.90808986649102));
#291075=CARTESIAN_POINT('Ctrl Pts',(6.21213331202014,98.8812499996149,-8.55026797822134));
#291076=CARTESIAN_POINT('Ctrl Pts',(3.10606665601004,99.0312499996143,-9.5594902125713));
#291077=CARTESIAN_POINT('Ctrl Pts',(-7.02435588123707E-14,99.1812499996138,
-10.5687124469213));
#291078=CARTESIAN_POINT('Ctrl Pts',(-3.10606665601018,99.3312499996131,
-9.5594902125713));
#291079=CARTESIAN_POINT('Ctrl Pts',(-6.21213331202029,99.4812499996125,
-8.55026797822134));
#291080=CARTESIAN_POINT('Ctrl Pts',(-8.13178807675726,99.631249999612,-5.90808986649102));
#291081=CARTESIAN_POINT('Ctrl Pts',(-10.0514428414942,99.7812499996114,
-3.2659117547607));
#291082=CARTESIAN_POINT('Ctrl Pts',(-10.0514428414942,99.9312499996108,
2.46189346052968E-15));
#291083=CARTESIAN_POINT('Ctrl Pts',(-10.0514428414942,100.08124999961,3.26591175476071));
#291084=CARTESIAN_POINT('Ctrl Pts',(-8.13178807675726,100.23124999961,5.90808986649102));
#291085=CARTESIAN_POINT('Ctrl Pts',(-6.21213331202028,100.381249999609,
8.55026797822134));
#291086=CARTESIAN_POINT('Ctrl Pts',(-3.10606665601018,100.531249999608,
9.5594902125713));
#291087=CARTESIAN_POINT('Ctrl Pts',(-6.85188254743555E-14,100.681249999608,
10.5687124469213));
#291088=CARTESIAN_POINT('Ctrl Pts',(3.10606665601004,100.831249999607,9.5594902125713));
#291089=CARTESIAN_POINT('Ctrl Pts',(6.21213331202015,100.981249999607,8.55026797822134));
#291090=CARTESIAN_POINT('Ctrl Pts',(8.13178807675712,101.131249999606,5.90808986649102));
#291091=CARTESIAN_POINT('Ctrl Pts',(10.0514428414941,101.281249999605,3.2659117547607));
#291092=CARTESIAN_POINT('Ctrl Pts',(10.0514428414941,101.431249999605,-1.23094673026484E-15));
#291093=CARTESIAN_POINT('Origin',(-3.77475828372553E-14,-1.881249999982,
2.68644078414671E-15));
#291094=CARTESIAN_POINT('',(10.0514428414941,104.806249999591,1.0126081184638E-15));
#291095=CARTESIAN_POINT('',(10.0514428414941,104.431249999593,1.01416483528425E-15));
#291096=CARTESIAN_POINT('',(10.0514428414941,-1.881249999982,4.14193483802857E-15));
#291097=CARTESIAN_POINT('Ctrl Pts',(10.0514428414941,101.806249999603,-1.23094673026484E-15));
#291098=CARTESIAN_POINT('Ctrl Pts',(10.0514428414941,101.956249999603,-3.26591175476071));
#291099=CARTESIAN_POINT('Ctrl Pts',(8.13178807675712,102.106249999602,-5.90808986649102));
#291100=CARTESIAN_POINT('Ctrl Pts',(6.21213331202014,102.256249999601,-8.55026797822134));
#291101=CARTESIAN_POINT('Ctrl Pts',(3.10606665601004,102.406249999601,-9.5594902125713));
#291102=CARTESIAN_POINT('Ctrl Pts',(-7.21872317429903E-14,102.5562499996,
-10.5687124469213));
#291103=CARTESIAN_POINT('Ctrl Pts',(-3.10606665601018,102.7062499996,-9.5594902125713));
#291104=CARTESIAN_POINT('Ctrl Pts',(-6.21213331202029,102.856249999599,
-8.55026797822134));
#291105=CARTESIAN_POINT('Ctrl Pts',(-8.13178807675726,103.006249999598,
-5.90808986649102));
#291106=CARTESIAN_POINT('Ctrl Pts',(-10.0514428414942,103.156249999598,
-3.2659117547607));
#291107=CARTESIAN_POINT('Ctrl Pts',(-10.0514428414942,103.306249999597,
2.46189346052968E-15));
#291108=CARTESIAN_POINT('Ctrl Pts',(-10.0514428414942,103.456249999597,
3.26591175476071));
#291109=CARTESIAN_POINT('Ctrl Pts',(-8.13178807675726,103.606249999596,
5.90808986649102));
#291110=CARTESIAN_POINT('Ctrl Pts',(-6.21213331202029,103.756249999595,
8.55026797822134));
#291111=CARTESIAN_POINT('Ctrl Pts',(-3.10606665601018,103.906249999595,
9.5594902125713));
#291112=CARTESIAN_POINT('Ctrl Pts',(-7.0462498404975E-14,104.056249999594,
10.5687124469213));
#291113=CARTESIAN_POINT('Ctrl Pts',(3.10606665601004,104.206249999594,9.5594902125713));
#291114=CARTESIAN_POINT('Ctrl Pts',(6.21213331202014,104.356249999593,8.55026797822134));
#291115=CARTESIAN_POINT('Ctrl Pts',(8.13178807675712,104.506249999592,5.90808986649102));
#291116=CARTESIAN_POINT('Ctrl Pts',(10.0514428414941,104.656249999592,3.2659117547607));
#291117=CARTESIAN_POINT('Ctrl Pts',(10.0514428414941,104.806249999591,-1.23094673026484E-15));
#291118=CARTESIAN_POINT('Ctrl Pts',(10.0514428414941,101.431249999605,-1.23094673026484E-15));
#291119=CARTESIAN_POINT('Ctrl Pts',(10.0514428414941,101.581249999604,-3.26591175476071));
#291120=CARTESIAN_POINT('Ctrl Pts',(8.13178807675712,101.731249999604,-5.90808986649102));
#291121=CARTESIAN_POINT('Ctrl Pts',(6.21213331202014,101.881249999603,-8.55026797822134));
#291122=CARTESIAN_POINT('Ctrl Pts',(3.10606665601004,102.031249999602,-9.5594902125713));
#291123=CARTESIAN_POINT('Ctrl Pts',(-7.19712680840326E-14,102.181249999602,
-10.5687124469213));
#291124=CARTESIAN_POINT('Ctrl Pts',(-3.10606665601018,102.331249999601,
-9.5594902125713));
#291125=CARTESIAN_POINT('Ctrl Pts',(-6.21213331202029,102.481249999601,
-8.55026797822134));
#291126=CARTESIAN_POINT('Ctrl Pts',(-8.13178807675726,102.6312499996,-5.90808986649102));
#291127=CARTESIAN_POINT('Ctrl Pts',(-10.0514428414942,102.781249999599,
-3.2659117547607));
#291128=CARTESIAN_POINT('Ctrl Pts',(-10.0514428414942,102.931249999599,
2.46189346052968E-15));
#291129=CARTESIAN_POINT('Ctrl Pts',(-10.0514428414942,103.081249999598,
3.26591175476071));
#291130=CARTESIAN_POINT('Ctrl Pts',(-8.13178807675726,103.231249999598,
5.90808986649102));
#291131=CARTESIAN_POINT('Ctrl Pts',(-6.21213331202029,103.381249999597,
8.55026797822134));
#291132=CARTESIAN_POINT('Ctrl Pts',(-3.10606665601018,103.531249999596,
9.5594902125713));
#291133=CARTESIAN_POINT('Ctrl Pts',(-7.02465347460173E-14,103.681249999596,
10.5687124469213));
#291134=CARTESIAN_POINT('Ctrl Pts',(3.10606665601004,103.831249999595,9.5594902125713));
#291135=CARTESIAN_POINT('Ctrl Pts',(6.21213331202014,103.981249999595,8.55026797822134));
#291136=CARTESIAN_POINT('Ctrl Pts',(8.13178807675712,104.131249999594,5.90808986649102));
#291137=CARTESIAN_POINT('Ctrl Pts',(10.0514428414941,104.281249999593,3.2659117547607));
#291138=CARTESIAN_POINT('Ctrl Pts',(10.0514428414941,104.431249999593,-1.23094673026484E-15));
#291139=CARTESIAN_POINT('Origin',(-3.77475828372553E-14,-1.881249999982,
2.68644078414671E-15));
#291140=CARTESIAN_POINT('',(10.0514428414941,107.806249999579,1.0001543839002E-15));
#291141=CARTESIAN_POINT('',(10.0514428414941,107.431249999581,1.00171110072065E-15));
#291142=CARTESIAN_POINT('',(10.0514428414941,-1.881249999982,4.14193483802857E-15));
#291143=CARTESIAN_POINT('Ctrl Pts',(10.0514428414941,104.806249999591,-1.23094673026484E-15));
#291144=CARTESIAN_POINT('Ctrl Pts',(10.0514428414941,104.956249999591,-3.26591175476071));
#291145=CARTESIAN_POINT('Ctrl Pts',(8.13178807675712,105.10624999959,-5.90808986649102));
#291146=CARTESIAN_POINT('Ctrl Pts',(6.21213331202014,105.256249999589,-8.55026797822134));
#291147=CARTESIAN_POINT('Ctrl Pts',(3.10606665601003,105.406249999589,-9.5594902125713));
#291148=CARTESIAN_POINT('Ctrl Pts',(-7.39149410146522E-14,105.556249999588,
-10.5687124469213));
#291149=CARTESIAN_POINT('Ctrl Pts',(-3.10606665601018,105.706249999588,
-9.5594902125713));
#291150=CARTESIAN_POINT('Ctrl Pts',(-6.21213331202029,105.856249999587,
-8.55026797822134));
#291151=CARTESIAN_POINT('Ctrl Pts',(-8.13178807675726,106.006249999586,
-5.90808986649102));
#291152=CARTESIAN_POINT('Ctrl Pts',(-10.0514428414942,106.156249999586,
-3.2659117547607));
#291153=CARTESIAN_POINT('Ctrl Pts',(-10.0514428414942,106.306249999585,
2.46189346052968E-15));
#291154=CARTESIAN_POINT('Ctrl Pts',(-10.0514428414942,106.456249999585,
3.26591175476071));
#291155=CARTESIAN_POINT('Ctrl Pts',(-8.13178807675726,106.606249999584,
5.90808986649102));
#291156=CARTESIAN_POINT('Ctrl Pts',(-6.21213331202029,106.756249999583,
8.55026797822134));
#291157=CARTESIAN_POINT('Ctrl Pts',(-3.10606665601018,106.906249999583,
9.5594902125713));
#291158=CARTESIAN_POINT('Ctrl Pts',(-7.21902076766369E-14,107.056249999582,
10.5687124469213));
#291159=CARTESIAN_POINT('Ctrl Pts',(3.10606665601003,107.206249999582,9.5594902125713));
#291160=CARTESIAN_POINT('Ctrl Pts',(6.21213331202014,107.356249999581,8.55026797822134));
#291161=CARTESIAN_POINT('Ctrl Pts',(8.13178807675711,107.50624999958,5.90808986649102));
#291162=CARTESIAN_POINT('Ctrl Pts',(10.0514428414941,107.65624999958,3.2659117547607));
#291163=CARTESIAN_POINT('Ctrl Pts',(10.0514428414941,107.806249999579,-1.23094673026484E-15));
#291164=CARTESIAN_POINT('Ctrl Pts',(10.0514428414941,104.431249999593,-1.23094673026484E-15));
#291165=CARTESIAN_POINT('Ctrl Pts',(10.0514428414941,104.581249999592,-3.26591175476071));
#291166=CARTESIAN_POINT('Ctrl Pts',(8.13178807675712,104.731249999592,-5.90808986649102));
#291167=CARTESIAN_POINT('Ctrl Pts',(6.21213331202014,104.881249999591,-8.55026797822134));
#291168=CARTESIAN_POINT('Ctrl Pts',(3.10606665601003,105.03124999959,-9.5594902125713));
#291169=CARTESIAN_POINT('Ctrl Pts',(-7.36989773556944E-14,105.18124999959,
-10.5687124469213));
#291170=CARTESIAN_POINT('Ctrl Pts',(-3.10606665601018,105.331249999589,
-9.5594902125713));
#291171=CARTESIAN_POINT('Ctrl Pts',(-6.21213331202029,105.481249999589,
-8.55026797822134));
#291172=CARTESIAN_POINT('Ctrl Pts',(-8.13178807675726,105.631249999588,
-5.90808986649102));
#291173=CARTESIAN_POINT('Ctrl Pts',(-10.0514428414942,105.781249999587,
-3.2659117547607));
#291174=CARTESIAN_POINT('Ctrl Pts',(-10.0514428414942,105.931249999587,
2.46189346052968E-15));
#291175=CARTESIAN_POINT('Ctrl Pts',(-10.0514428414942,106.081249999586,
3.26591175476071));
#291176=CARTESIAN_POINT('Ctrl Pts',(-8.13178807675726,106.231249999586,
5.90808986649102));
#291177=CARTESIAN_POINT('Ctrl Pts',(-6.21213331202029,106.381249999585,
8.55026797822134));
#291178=CARTESIAN_POINT('Ctrl Pts',(-3.10606665601018,106.531249999584,
9.5594902125713));
#291179=CARTESIAN_POINT('Ctrl Pts',(-7.19742440176792E-14,106.681249999584,
10.5687124469213));
#291180=CARTESIAN_POINT('Ctrl Pts',(3.10606665601004,106.831249999583,9.5594902125713));
#291181=CARTESIAN_POINT('Ctrl Pts',(6.21213331202014,106.981249999583,8.55026797822134));
#291182=CARTESIAN_POINT('Ctrl Pts',(8.13178807675711,107.131249999582,5.90808986649102));
#291183=CARTESIAN_POINT('Ctrl Pts',(10.0514428414941,107.281249999581,3.2659117547607));
#291184=CARTESIAN_POINT('Ctrl Pts',(10.0514428414941,107.431249999581,-1.23094673026484E-15));
#291185=CARTESIAN_POINT('Origin',(-3.77475828372553E-14,-1.881249999982,
2.68644078414671E-15));
#291186=CARTESIAN_POINT('',(10.0514428414941,110.806249999567,9.87700649336596E-16));
#291187=CARTESIAN_POINT('',(10.0514428414941,110.431249999569,9.89257366157046E-16));
#291188=CARTESIAN_POINT('',(10.0514428414941,-1.881249999982,4.14193483802857E-15));
#291189=CARTESIAN_POINT('Ctrl Pts',(10.0514428414941,107.806249999579,-1.23094673026484E-15));
#291190=CARTESIAN_POINT('Ctrl Pts',(10.0514428414941,107.956249999579,-3.26591175476071));
#291191=CARTESIAN_POINT('Ctrl Pts',(8.13178807675711,108.106249999578,-5.90808986649102));
#291192=CARTESIAN_POINT('Ctrl Pts',(6.21213331202014,108.256249999577,-8.55026797822134));
#291193=CARTESIAN_POINT('Ctrl Pts',(3.10606665601003,108.406249999577,-9.5594902125713));
#291194=CARTESIAN_POINT('Ctrl Pts',(-7.5642650286314E-14,108.556249999576,
-10.5687124469213));
#291195=CARTESIAN_POINT('Ctrl Pts',(-3.10606665601018,108.706249999576,
-9.5594902125713));
#291196=CARTESIAN_POINT('Ctrl Pts',(-6.21213331202029,108.856249999575,
-8.55026797822134));
#291197=CARTESIAN_POINT('Ctrl Pts',(-8.13178807675727,109.006249999574,
-5.90808986649102));
#291198=CARTESIAN_POINT('Ctrl Pts',(-10.0514428414942,109.156249999574,
-3.2659117547607));
#291199=CARTESIAN_POINT('Ctrl Pts',(-10.0514428414942,109.306249999573,
2.46189346052968E-15));
#291200=CARTESIAN_POINT('Ctrl Pts',(-10.0514428414942,109.456249999573,
3.26591175476071));
#291201=CARTESIAN_POINT('Ctrl Pts',(-8.13178807675727,109.606249999572,
5.90808986649102));
#291202=CARTESIAN_POINT('Ctrl Pts',(-6.21213331202029,109.756249999571,
8.55026797822134));
#291203=CARTESIAN_POINT('Ctrl Pts',(-3.10606665601018,109.906249999571,
9.5594902125713));
#291204=CARTESIAN_POINT('Ctrl Pts',(-7.39179169482987E-14,110.05624999957,
10.5687124469213));
#291205=CARTESIAN_POINT('Ctrl Pts',(3.10606665601003,110.20624999957,9.5594902125713));
#291206=CARTESIAN_POINT('Ctrl Pts',(6.21213331202014,110.356249999569,8.55026797822134));
#291207=CARTESIAN_POINT('Ctrl Pts',(8.13178807675711,110.506249999568,5.90808986649102));
#291208=CARTESIAN_POINT('Ctrl Pts',(10.0514428414941,110.656249999568,3.2659117547607));
#291209=CARTESIAN_POINT('Ctrl Pts',(10.0514428414941,110.806249999567,-1.23094673026484E-15));
#291210=CARTESIAN_POINT('Ctrl Pts',(10.0514428414941,107.431249999581,-1.23094673026484E-15));
#291211=CARTESIAN_POINT('Ctrl Pts',(10.0514428414941,107.58124999958,-3.26591175476071));
#291212=CARTESIAN_POINT('Ctrl Pts',(8.13178807675711,107.73124999958,-5.90808986649102));
#291213=CARTESIAN_POINT('Ctrl Pts',(6.21213331202014,107.881249999579,-8.55026797822134));
#291214=CARTESIAN_POINT('Ctrl Pts',(3.10606665601003,108.031249999578,-9.5594902125713));
#291215=CARTESIAN_POINT('Ctrl Pts',(-7.54266866273562E-14,108.181249999578,
-10.5687124469213));
#291216=CARTESIAN_POINT('Ctrl Pts',(-3.10606665601018,108.331249999577,
-9.5594902125713));
#291217=CARTESIAN_POINT('Ctrl Pts',(-6.21213331202029,108.481249999577,
-8.55026797822134));
#291218=CARTESIAN_POINT('Ctrl Pts',(-8.13178807675727,108.631249999576,
-5.90808986649102));
#291219=CARTESIAN_POINT('Ctrl Pts',(-10.0514428414942,108.781249999575,
-3.2659117547607));
#291220=CARTESIAN_POINT('Ctrl Pts',(-10.0514428414942,108.931249999575,
2.46189346052968E-15));
#291221=CARTESIAN_POINT('Ctrl Pts',(-10.0514428414942,109.081249999574,
3.26591175476071));
#291222=CARTESIAN_POINT('Ctrl Pts',(-8.13178807675727,109.231249999574,
5.90808986649102));
#291223=CARTESIAN_POINT('Ctrl Pts',(-6.21213331202029,109.381249999573,
8.55026797822134));
#291224=CARTESIAN_POINT('Ctrl Pts',(-3.10606665601018,109.531249999572,
9.5594902125713));
#291225=CARTESIAN_POINT('Ctrl Pts',(-7.3701953289341E-14,109.681249999572,
10.5687124469213));
#291226=CARTESIAN_POINT('Ctrl Pts',(3.10606665601003,109.831249999571,9.5594902125713));
#291227=CARTESIAN_POINT('Ctrl Pts',(6.21213331202014,109.981249999571,8.55026797822134));
#291228=CARTESIAN_POINT('Ctrl Pts',(8.13178807675711,110.13124999957,5.90808986649102));
#291229=CARTESIAN_POINT('Ctrl Pts',(10.0514428414941,110.281249999569,3.2659117547607));
#291230=CARTESIAN_POINT('Ctrl Pts',(10.0514428414941,110.431249999569,-1.23094673026484E-15));
#291231=CARTESIAN_POINT('Origin',(-3.77475828372553E-14,-1.881249999982,
2.68644078414671E-15));
#291232=CARTESIAN_POINT('',(10.0514428414941,113.806249999555,9.75246914772995E-16));
#291233=CARTESIAN_POINT('',(10.0514428414941,113.431249999557,9.76803631593445E-16));
#291234=CARTESIAN_POINT('',(10.0514428414941,-1.881249999982,4.14193483802857E-15));
#291235=CARTESIAN_POINT('Ctrl Pts',(10.0514428414941,110.806249999567,-1.23094673026484E-15));
#291236=CARTESIAN_POINT('Ctrl Pts',(10.0514428414941,110.956249999567,-3.26591175476071));
#291237=CARTESIAN_POINT('Ctrl Pts',(8.13178807675711,111.106249999566,-5.90808986649102));
#291238=CARTESIAN_POINT('Ctrl Pts',(6.21213331202014,111.256249999565,-8.55026797822134));
#291239=CARTESIAN_POINT('Ctrl Pts',(3.10606665601003,111.406249999565,-9.5594902125713));
#291240=CARTESIAN_POINT('Ctrl Pts',(-7.73703595579758E-14,111.556249999564,
-10.5687124469213));
#291241=CARTESIAN_POINT('Ctrl Pts',(-3.10606665601019,111.706249999564,
-9.5594902125713));
#291242=CARTESIAN_POINT('Ctrl Pts',(-6.21213331202029,111.856249999563,
-8.55026797822134));
#291243=CARTESIAN_POINT('Ctrl Pts',(-8.13178807675727,112.006249999562,
-5.90808986649102));
#291244=CARTESIAN_POINT('Ctrl Pts',(-10.0514428414942,112.156249999562,
-3.2659117547607));
#291245=CARTESIAN_POINT('Ctrl Pts',(-10.0514428414942,112.306249999561,
2.46189346052968E-15));
#291246=CARTESIAN_POINT('Ctrl Pts',(-10.0514428414942,112.456249999561,
3.26591175476071));
#291247=CARTESIAN_POINT('Ctrl Pts',(-8.13178807675727,112.60624999956,5.90808986649102));
#291248=CARTESIAN_POINT('Ctrl Pts',(-6.21213331202029,112.756249999559,
8.55026797822134));
#291249=CARTESIAN_POINT('Ctrl Pts',(-3.10606665601018,112.906249999559,
9.5594902125713));
#291250=CARTESIAN_POINT('Ctrl Pts',(-7.56456262199606E-14,113.056249999558,
10.5687124469213));
#291251=CARTESIAN_POINT('Ctrl Pts',(3.10606665601003,113.206249999558,9.5594902125713));
#291252=CARTESIAN_POINT('Ctrl Pts',(6.21213331202014,113.356249999557,8.55026797822134));
#291253=CARTESIAN_POINT('Ctrl Pts',(8.13178807675711,113.506249999556,5.90808986649102));
#291254=CARTESIAN_POINT('Ctrl Pts',(10.0514428414941,113.656249999556,3.2659117547607));
#291255=CARTESIAN_POINT('Ctrl Pts',(10.0514428414941,113.806249999555,-1.23094673026484E-15));
#291256=CARTESIAN_POINT('Ctrl Pts',(10.0514428414941,110.431249999569,-1.23094673026484E-15));
#291257=CARTESIAN_POINT('Ctrl Pts',(10.0514428414941,110.581249999568,-3.26591175476071));
#291258=CARTESIAN_POINT('Ctrl Pts',(8.13178807675711,110.731249999568,-5.90808986649102));
#291259=CARTESIAN_POINT('Ctrl Pts',(6.21213331202014,110.881249999567,-8.55026797822134));
#291260=CARTESIAN_POINT('Ctrl Pts',(3.10606665601003,111.031249999566,-9.5594902125713));
#291261=CARTESIAN_POINT('Ctrl Pts',(-7.71543958990181E-14,111.181249999566,
-10.5687124469213));
#291262=CARTESIAN_POINT('Ctrl Pts',(-3.10606665601019,111.331249999565,
-9.5594902125713));
#291263=CARTESIAN_POINT('Ctrl Pts',(-6.21213331202029,111.481249999565,
-8.55026797822134));
#291264=CARTESIAN_POINT('Ctrl Pts',(-8.13178807675727,111.631249999564,
-5.90808986649102));
#291265=CARTESIAN_POINT('Ctrl Pts',(-10.0514428414942,111.781249999563,
-3.2659117547607));
#291266=CARTESIAN_POINT('Ctrl Pts',(-10.0514428414942,111.931249999563,
2.46189346052968E-15));
#291267=CARTESIAN_POINT('Ctrl Pts',(-10.0514428414942,112.081249999562,
3.26591175476071));
#291268=CARTESIAN_POINT('Ctrl Pts',(-8.13178807675727,112.231249999562,
5.90808986649102));
#291269=CARTESIAN_POINT('Ctrl Pts',(-6.21213331202029,112.381249999561,
8.55026797822134));
#291270=CARTESIAN_POINT('Ctrl Pts',(-3.10606665601018,112.53124999956,9.5594902125713));
#291271=CARTESIAN_POINT('Ctrl Pts',(-7.54296625610028E-14,112.68124999956,
10.5687124469213));
#291272=CARTESIAN_POINT('Ctrl Pts',(3.10606665601003,112.831249999559,9.5594902125713));
#291273=CARTESIAN_POINT('Ctrl Pts',(6.21213331202014,112.981249999559,8.55026797822134));
#291274=CARTESIAN_POINT('Ctrl Pts',(8.13178807675711,113.131249999558,5.90808986649102));
#291275=CARTESIAN_POINT('Ctrl Pts',(10.0514428414941,113.281249999557,3.2659117547607));
#291276=CARTESIAN_POINT('Ctrl Pts',(10.0514428414941,113.431249999557,-1.23094673026484E-15));
#291277=CARTESIAN_POINT('Origin',(-3.77475828372553E-14,-1.881249999982,
2.68644078414671E-15));
#291278=CARTESIAN_POINT('',(10.0514428414941,116.806249999543,9.62793180209394E-16));
#291279=CARTESIAN_POINT('',(10.0514428414941,116.431249999545,9.64349897029844E-16));
#291280=CARTESIAN_POINT('',(10.0514428414941,-1.881249999982,4.14193483802857E-15));
#291281=CARTESIAN_POINT('Ctrl Pts',(10.0514428414941,113.806249999555,-1.23094673026484E-15));
#291282=CARTESIAN_POINT('Ctrl Pts',(10.0514428414941,113.956249999555,-3.26591175476071));
#291283=CARTESIAN_POINT('Ctrl Pts',(8.13178807675711,114.106249999554,-5.90808986649102));
#291284=CARTESIAN_POINT('Ctrl Pts',(6.21213331202014,114.256249999553,-8.55026797822134));
#291285=CARTESIAN_POINT('Ctrl Pts',(3.10606665601003,114.406249999553,-9.5594902125713));
#291286=CARTESIAN_POINT('Ctrl Pts',(-7.90980688296377E-14,114.556249999552,
-10.5687124469213));
#291287=CARTESIAN_POINT('Ctrl Pts',(-3.10606665601019,114.706249999552,
-9.5594902125713));
#291288=CARTESIAN_POINT('Ctrl Pts',(-6.21213331202029,114.856249999551,
-8.55026797822134));
#291289=CARTESIAN_POINT('Ctrl Pts',(-8.13178807675727,115.00624999955,-5.90808986649102));
#291290=CARTESIAN_POINT('Ctrl Pts',(-10.0514428414942,115.15624999955,-3.2659117547607));
#291291=CARTESIAN_POINT('Ctrl Pts',(-10.0514428414942,115.306249999549,
2.46189346052968E-15));
#291292=CARTESIAN_POINT('Ctrl Pts',(-10.0514428414942,115.456249999549,
3.26591175476071));
#291293=CARTESIAN_POINT('Ctrl Pts',(-8.13178807675727,115.606249999548,
5.90808986649102));
#291294=CARTESIAN_POINT('Ctrl Pts',(-6.21213331202029,115.756249999547,
8.55026797822134));
#291295=CARTESIAN_POINT('Ctrl Pts',(-3.10606665601019,115.906249999547,
9.5594902125713));
#291296=CARTESIAN_POINT('Ctrl Pts',(-7.73733354916224E-14,116.056249999546,
10.5687124469213));
#291297=CARTESIAN_POINT('Ctrl Pts',(3.10606665601003,116.206249999546,9.5594902125713));
#291298=CARTESIAN_POINT('Ctrl Pts',(6.21213331202014,116.356249999545,8.55026797822134));
#291299=CARTESIAN_POINT('Ctrl Pts',(8.13178807675711,116.506249999544,5.90808986649102));
#291300=CARTESIAN_POINT('Ctrl Pts',(10.0514428414941,116.656249999544,3.2659117547607));
#291301=CARTESIAN_POINT('Ctrl Pts',(10.0514428414941,116.806249999543,-1.23094673026484E-15));
#291302=CARTESIAN_POINT('Ctrl Pts',(10.0514428414941,113.431249999557,-1.23094673026484E-15));
#291303=CARTESIAN_POINT('Ctrl Pts',(10.0514428414941,113.581249999556,-3.26591175476071));
#291304=CARTESIAN_POINT('Ctrl Pts',(8.13178807675711,113.731249999556,-5.90808986649102));
#291305=CARTESIAN_POINT('Ctrl Pts',(6.21213331202014,113.881249999555,-8.55026797822134));
#291306=CARTESIAN_POINT('Ctrl Pts',(3.10606665601003,114.031249999554,-9.5594902125713));
#291307=CARTESIAN_POINT('Ctrl Pts',(-7.88821051706799E-14,114.181249999554,
-10.5687124469213));
#291308=CARTESIAN_POINT('Ctrl Pts',(-3.10606665601019,114.331249999553,
-9.5594902125713));
#291309=CARTESIAN_POINT('Ctrl Pts',(-6.21213331202029,114.481249999553,
-8.55026797822134));
#291310=CARTESIAN_POINT('Ctrl Pts',(-8.13178807675727,114.631249999552,
-5.90808986649102));
#291311=CARTESIAN_POINT('Ctrl Pts',(-10.0514428414942,114.781249999551,
-3.2659117547607));
#291312=CARTESIAN_POINT('Ctrl Pts',(-10.0514428414942,114.931249999551,
2.46189346052968E-15));
#291313=CARTESIAN_POINT('Ctrl Pts',(-10.0514428414942,115.08124999955,3.26591175476071));
#291314=CARTESIAN_POINT('Ctrl Pts',(-8.13178807675727,115.23124999955,5.90808986649102));
#291315=CARTESIAN_POINT('Ctrl Pts',(-6.21213331202029,115.381249999549,
8.55026797822134));
#291316=CARTESIAN_POINT('Ctrl Pts',(-3.10606665601018,115.531249999548,
9.5594902125713));
#291317=CARTESIAN_POINT('Ctrl Pts',(-7.71573718326647E-14,115.681249999548,
10.5687124469213));
#291318=CARTESIAN_POINT('Ctrl Pts',(3.10606665601003,115.831249999547,9.5594902125713));
#291319=CARTESIAN_POINT('Ctrl Pts',(6.21213331202014,115.981249999547,8.55026797822134));
#291320=CARTESIAN_POINT('Ctrl Pts',(8.13178807675711,116.131249999546,5.90808986649102));
#291321=CARTESIAN_POINT('Ctrl Pts',(10.0514428414941,116.281249999545,3.2659117547607));
#291322=CARTESIAN_POINT('Ctrl Pts',(10.0514428414941,116.431249999545,-1.23094673026484E-15));
#291323=CARTESIAN_POINT('Origin',(-3.77475828372553E-14,-1.881249999982,
2.68644078414671E-15));
#291324=CARTESIAN_POINT('',(10.0514428414941,119.806249999531,9.50339445645792E-16));
#291325=CARTESIAN_POINT('',(10.0514428414941,119.431249999533,9.51896162466242E-16));
#291326=CARTESIAN_POINT('',(10.0514428414941,-1.881249999982,4.14193483802857E-15));
#291327=CARTESIAN_POINT('Ctrl Pts',(10.0514428414941,116.806249999543,-1.23094673026484E-15));
#291328=CARTESIAN_POINT('Ctrl Pts',(10.0514428414941,116.956249999543,-3.26591175476071));
#291329=CARTESIAN_POINT('Ctrl Pts',(8.13178807675711,117.106249999542,-5.90808986649102));
#291330=CARTESIAN_POINT('Ctrl Pts',(6.21213331202014,117.256249999541,-8.55026797822134));
#291331=CARTESIAN_POINT('Ctrl Pts',(3.10606665601003,117.406249999541,-9.5594902125713));
#291332=CARTESIAN_POINT('Ctrl Pts',(-8.08257781012995E-14,117.55624999954,
-10.5687124469213));
#291333=CARTESIAN_POINT('Ctrl Pts',(-3.10606665601019,117.70624999954,-9.5594902125713));
#291334=CARTESIAN_POINT('Ctrl Pts',(-6.2121333120203,117.856249999539,-8.55026797822134));
#291335=CARTESIAN_POINT('Ctrl Pts',(-8.13178807675727,118.006249999538,
-5.90808986649102));
#291336=CARTESIAN_POINT('Ctrl Pts',(-10.0514428414942,118.156249999538,
-3.2659117547607));
#291337=CARTESIAN_POINT('Ctrl Pts',(-10.0514428414942,118.306249999537,
2.46189346052968E-15));
#291338=CARTESIAN_POINT('Ctrl Pts',(-10.0514428414942,118.456249999537,
3.26591175476071));
#291339=CARTESIAN_POINT('Ctrl Pts',(-8.13178807675727,118.606249999536,
5.90808986649102));
#291340=CARTESIAN_POINT('Ctrl Pts',(-6.21213331202029,118.756249999535,
8.55026797822134));
#291341=CARTESIAN_POINT('Ctrl Pts',(-3.10606665601019,118.906249999535,
9.5594902125713));
#291342=CARTESIAN_POINT('Ctrl Pts',(-7.91010447632842E-14,119.056249999534,
10.5687124469213));
#291343=CARTESIAN_POINT('Ctrl Pts',(3.10606665601003,119.206249999534,9.5594902125713));
#291344=CARTESIAN_POINT('Ctrl Pts',(6.21213331202014,119.356249999533,8.55026797822134));
#291345=CARTESIAN_POINT('Ctrl Pts',(8.13178807675711,119.506249999532,5.90808986649102));
#291346=CARTESIAN_POINT('Ctrl Pts',(10.0514428414941,119.656249999532,3.2659117547607));
#291347=CARTESIAN_POINT('Ctrl Pts',(10.0514428414941,119.806249999531,-1.23094673026484E-15));
#291348=CARTESIAN_POINT('Ctrl Pts',(10.0514428414941,116.431249999545,-1.23094673026484E-15));
#291349=CARTESIAN_POINT('Ctrl Pts',(10.0514428414941,116.581249999544,-3.26591175476071));
#291350=CARTESIAN_POINT('Ctrl Pts',(8.13178807675711,116.731249999544,-5.90808986649102));
#291351=CARTESIAN_POINT('Ctrl Pts',(6.21213331202014,116.881249999543,-8.55026797822134));
#291352=CARTESIAN_POINT('Ctrl Pts',(3.10606665601003,117.031249999542,-9.5594902125713));
#291353=CARTESIAN_POINT('Ctrl Pts',(-8.06098144423418E-14,117.181249999542,
-10.5687124469213));
#291354=CARTESIAN_POINT('Ctrl Pts',(-3.10606665601019,117.331249999541,
-9.5594902125713));
#291355=CARTESIAN_POINT('Ctrl Pts',(-6.2121333120203,117.481249999541,-8.55026797822134));
#291356=CARTESIAN_POINT('Ctrl Pts',(-8.13178807675727,117.63124999954,-5.90808986649102));
#291357=CARTESIAN_POINT('Ctrl Pts',(-10.0514428414942,117.781249999539,
-3.2659117547607));
#291358=CARTESIAN_POINT('Ctrl Pts',(-10.0514428414942,117.931249999539,
2.46189346052968E-15));
#291359=CARTESIAN_POINT('Ctrl Pts',(-10.0514428414942,118.081249999538,
3.26591175476071));
#291360=CARTESIAN_POINT('Ctrl Pts',(-8.13178807675727,118.231249999538,
5.90808986649102));
#291361=CARTESIAN_POINT('Ctrl Pts',(-6.21213331202029,118.381249999537,
8.55026797822134));
#291362=CARTESIAN_POINT('Ctrl Pts',(-3.10606665601019,118.531249999536,
9.5594902125713));
#291363=CARTESIAN_POINT('Ctrl Pts',(-7.88850811043265E-14,118.681249999536,
10.5687124469213));
#291364=CARTESIAN_POINT('Ctrl Pts',(3.10606665601003,118.831249999535,9.5594902125713));
#291365=CARTESIAN_POINT('Ctrl Pts',(6.21213331202014,118.981249999535,8.55026797822134));
#291366=CARTESIAN_POINT('Ctrl Pts',(8.13178807675711,119.131249999534,5.90808986649102));
#291367=CARTESIAN_POINT('Ctrl Pts',(10.0514428414941,119.281249999533,3.2659117547607));
#291368=CARTESIAN_POINT('Ctrl Pts',(10.0514428414941,119.431249999533,-1.23094673026484E-15));
#291369=CARTESIAN_POINT('Origin',(-3.77475828372553E-14,-1.881249999982,
2.68644078414671E-15));
#291370=CARTESIAN_POINT('',(10.0514428414941,122.806249999519,9.37885711082191E-16));
#291371=CARTESIAN_POINT('',(10.0514428414941,122.431249999521,9.39442427902641E-16));
#291372=CARTESIAN_POINT('',(10.0514428414941,-1.881249999982,4.14193483802857E-15));
#291373=CARTESIAN_POINT('Ctrl Pts',(10.0514428414941,119.806249999531,-1.23094673026484E-15));
#291374=CARTESIAN_POINT('Ctrl Pts',(10.0514428414941,119.956249999531,-3.26591175476071));
#291375=CARTESIAN_POINT('Ctrl Pts',(8.13178807675711,120.10624999953,-5.90808986649102));
#291376=CARTESIAN_POINT('Ctrl Pts',(6.21213331202013,120.256249999529,-8.55026797822134));
#291377=CARTESIAN_POINT('Ctrl Pts',(3.10606665601003,120.406249999529,-9.5594902125713));
#291378=CARTESIAN_POINT('Ctrl Pts',(-8.25534873729613E-14,120.556249999528,
-10.5687124469213));
#291379=CARTESIAN_POINT('Ctrl Pts',(-3.10606665601019,120.706249999528,
-9.5594902125713));
#291380=CARTESIAN_POINT('Ctrl Pts',(-6.2121333120203,120.856249999527,-8.55026797822134));
#291381=CARTESIAN_POINT('Ctrl Pts',(-8.13178807675727,121.006249999526,
-5.90808986649102));
#291382=CARTESIAN_POINT('Ctrl Pts',(-10.0514428414943,121.156249999526,
-3.2659117547607));
#291383=CARTESIAN_POINT('Ctrl Pts',(-10.0514428414943,121.306249999525,
2.46189346052968E-15));
#291384=CARTESIAN_POINT('Ctrl Pts',(-10.0514428414943,121.456249999525,
3.26591175476071));
#291385=CARTESIAN_POINT('Ctrl Pts',(-8.13178807675727,121.606249999524,
5.90808986649102));
#291386=CARTESIAN_POINT('Ctrl Pts',(-6.2121333120203,121.756249999523,8.55026797822134));
#291387=CARTESIAN_POINT('Ctrl Pts',(-3.10606665601019,121.906249999523,
9.5594902125713));
#291388=CARTESIAN_POINT('Ctrl Pts',(-8.08287540349461E-14,122.056249999522,
10.5687124469213));
#291389=CARTESIAN_POINT('Ctrl Pts',(3.10606665601003,122.206249999522,9.5594902125713));
#291390=CARTESIAN_POINT('Ctrl Pts',(6.21213331202014,122.356249999521,8.55026797822134));
#291391=CARTESIAN_POINT('Ctrl Pts',(8.13178807675711,122.50624999952,5.90808986649102));
#291392=CARTESIAN_POINT('Ctrl Pts',(10.0514428414941,122.65624999952,3.2659117547607));
#291393=CARTESIAN_POINT('Ctrl Pts',(10.0514428414941,122.806249999519,-1.23094673026484E-15));
#291394=CARTESIAN_POINT('Ctrl Pts',(10.0514428414941,119.431249999533,-1.23094673026484E-15));
#291395=CARTESIAN_POINT('Ctrl Pts',(10.0514428414941,119.581249999532,-3.26591175476071));
#291396=CARTESIAN_POINT('Ctrl Pts',(8.13178807675711,119.731249999532,-5.90808986649102));
#291397=CARTESIAN_POINT('Ctrl Pts',(6.21213331202013,119.881249999531,-8.55026797822134));
#291398=CARTESIAN_POINT('Ctrl Pts',(3.10606665601003,120.03124999953,-9.5594902125713));
#291399=CARTESIAN_POINT('Ctrl Pts',(-8.23375237140036E-14,120.18124999953,
-10.5687124469213));
#291400=CARTESIAN_POINT('Ctrl Pts',(-3.10606665601019,120.331249999529,
-9.5594902125713));
#291401=CARTESIAN_POINT('Ctrl Pts',(-6.2121333120203,120.481249999529,-8.55026797822134));
#291402=CARTESIAN_POINT('Ctrl Pts',(-8.13178807675727,120.631249999528,
-5.90808986649102));
#291403=CARTESIAN_POINT('Ctrl Pts',(-10.0514428414943,120.781249999527,
-3.2659117547607));
#291404=CARTESIAN_POINT('Ctrl Pts',(-10.0514428414943,120.931249999527,
2.46189346052968E-15));
#291405=CARTESIAN_POINT('Ctrl Pts',(-10.0514428414943,121.081249999526,
3.26591175476071));
#291406=CARTESIAN_POINT('Ctrl Pts',(-8.13178807675727,121.231249999526,
5.90808986649102));
#291407=CARTESIAN_POINT('Ctrl Pts',(-6.2121333120203,121.381249999525,8.55026797822134));
#291408=CARTESIAN_POINT('Ctrl Pts',(-3.10606665601019,121.531249999524,
9.5594902125713));
#291409=CARTESIAN_POINT('Ctrl Pts',(-8.06127903759884E-14,121.681249999524,
10.5687124469213));
#291410=CARTESIAN_POINT('Ctrl Pts',(3.10606665601003,121.831249999523,9.5594902125713));
#291411=CARTESIAN_POINT('Ctrl Pts',(6.21213331202014,121.981249999523,8.55026797822134));
#291412=CARTESIAN_POINT('Ctrl Pts',(8.13178807675711,122.131249999522,5.90808986649102));
#291413=CARTESIAN_POINT('Ctrl Pts',(10.0514428414941,122.281249999521,3.2659117547607));
#291414=CARTESIAN_POINT('Ctrl Pts',(10.0514428414941,122.431249999521,-1.23094673026484E-15));
#291415=CARTESIAN_POINT('Origin',(-3.77475828372553E-14,-1.881249999982,
2.68644078414671E-15));
#291416=CARTESIAN_POINT('',(10.0514428414941,125.806249999507,9.2543197651859E-16));
#291417=CARTESIAN_POINT('',(10.0514428414941,125.431249999509,9.2698869333904E-16));
#291418=CARTESIAN_POINT('',(10.0514428414941,-1.881249999982,4.14193483802857E-15));
#291419=CARTESIAN_POINT('Ctrl Pts',(10.0514428414941,122.806249999519,-1.23094673026484E-15));
#291420=CARTESIAN_POINT('Ctrl Pts',(10.0514428414941,122.956249999519,-3.26591175476071));
#291421=CARTESIAN_POINT('Ctrl Pts',(8.13178807675711,123.106249999518,-5.90808986649102));
#291422=CARTESIAN_POINT('Ctrl Pts',(6.21213331202013,123.256249999517,-8.55026797822134));
#291423=CARTESIAN_POINT('Ctrl Pts',(3.10606665601002,123.406249999517,-9.5594902125713));
#291424=CARTESIAN_POINT('Ctrl Pts',(-8.42811966446232E-14,123.556249999516,
-10.5687124469213));
#291425=CARTESIAN_POINT('Ctrl Pts',(-3.10606665601019,123.706249999516,
-9.5594902125713));
#291426=CARTESIAN_POINT('Ctrl Pts',(-6.2121333120203,123.856249999515,-8.55026797822134));
#291427=CARTESIAN_POINT('Ctrl Pts',(-8.13178807675727,124.006249999514,
-5.90808986649102));
#291428=CARTESIAN_POINT('Ctrl Pts',(-10.0514428414943,124.156249999514,
-3.2659117547607));
#291429=CARTESIAN_POINT('Ctrl Pts',(-10.0514428414943,124.306249999513,
2.46189346052968E-15));
#291430=CARTESIAN_POINT('Ctrl Pts',(-10.0514428414943,124.456249999513,
3.26591175476071));
#291431=CARTESIAN_POINT('Ctrl Pts',(-8.13178807675727,124.606249999512,
5.90808986649102));
#291432=CARTESIAN_POINT('Ctrl Pts',(-6.2121333120203,124.756249999511,8.55026797822134));
#291433=CARTESIAN_POINT('Ctrl Pts',(-3.10606665601019,124.906249999511,
9.5594902125713));
#291434=CARTESIAN_POINT('Ctrl Pts',(-8.25564633066079E-14,125.05624999951,
10.5687124469213));
#291435=CARTESIAN_POINT('Ctrl Pts',(3.10606665601002,125.20624999951,9.5594902125713));
#291436=CARTESIAN_POINT('Ctrl Pts',(6.21213331202013,125.356249999509,8.55026797822134));
#291437=CARTESIAN_POINT('Ctrl Pts',(8.13178807675711,125.506249999508,5.90808986649102));
#291438=CARTESIAN_POINT('Ctrl Pts',(10.0514428414941,125.656249999508,3.2659117547607));
#291439=CARTESIAN_POINT('Ctrl Pts',(10.0514428414941,125.806249999507,-1.23094673026484E-15));
#291440=CARTESIAN_POINT('Ctrl Pts',(10.0514428414941,122.431249999521,-1.23094673026484E-15));
#291441=CARTESIAN_POINT('Ctrl Pts',(10.0514428414941,122.58124999952,-3.26591175476071));
#291442=CARTESIAN_POINT('Ctrl Pts',(8.13178807675711,122.73124999952,-5.90808986649102));
#291443=CARTESIAN_POINT('Ctrl Pts',(6.21213331202013,122.881249999519,-8.55026797822134));
#291444=CARTESIAN_POINT('Ctrl Pts',(3.10606665601002,123.031249999518,-9.5594902125713));
#291445=CARTESIAN_POINT('Ctrl Pts',(-8.40652329856655E-14,123.181249999518,
-10.5687124469213));
#291446=CARTESIAN_POINT('Ctrl Pts',(-3.10606665601019,123.331249999517,
-9.5594902125713));
#291447=CARTESIAN_POINT('Ctrl Pts',(-6.2121333120203,123.481249999517,-8.55026797822134));
#291448=CARTESIAN_POINT('Ctrl Pts',(-8.13178807675727,123.631249999516,
-5.90808986649102));
#291449=CARTESIAN_POINT('Ctrl Pts',(-10.0514428414943,123.781249999515,
-3.2659117547607));
#291450=CARTESIAN_POINT('Ctrl Pts',(-10.0514428414943,123.931249999515,
2.46189346052968E-15));
#291451=CARTESIAN_POINT('Ctrl Pts',(-10.0514428414943,124.081249999514,
3.26591175476071));
#291452=CARTESIAN_POINT('Ctrl Pts',(-8.13178807675727,124.231249999514,
5.90808986649102));
#291453=CARTESIAN_POINT('Ctrl Pts',(-6.2121333120203,124.381249999513,8.55026797822134));
#291454=CARTESIAN_POINT('Ctrl Pts',(-3.10606665601019,124.531249999512,
9.5594902125713));
#291455=CARTESIAN_POINT('Ctrl Pts',(-8.23404996476502E-14,124.681249999512,
10.5687124469213));
#291456=CARTESIAN_POINT('Ctrl Pts',(3.10606665601002,124.831249999511,9.5594902125713));
#291457=CARTESIAN_POINT('Ctrl Pts',(6.21213331202013,124.981249999511,8.55026797822134));
#291458=CARTESIAN_POINT('Ctrl Pts',(8.13178807675711,125.13124999951,5.90808986649102));
#291459=CARTESIAN_POINT('Ctrl Pts',(10.0514428414941,125.281249999509,3.2659117547607));
#291460=CARTESIAN_POINT('Ctrl Pts',(10.0514428414941,125.431249999509,-1.23094673026484E-15));
#291461=CARTESIAN_POINT('Origin',(-3.77475828372553E-14,-1.881249999982,
2.68644078414671E-15));
#291462=CARTESIAN_POINT('',(10.0514428414941,128.806249999495,9.12978241954989E-16));
#291463=CARTESIAN_POINT('',(10.0514428414941,128.431249999497,9.14534958775439E-16));
#291464=CARTESIAN_POINT('',(10.0514428414941,-1.881249999982,4.14193483802857E-15));
#291465=CARTESIAN_POINT('Ctrl Pts',(10.0514428414941,125.806249999507,-1.23094673026484E-15));
#291466=CARTESIAN_POINT('Ctrl Pts',(10.0514428414941,125.956249999507,-3.26591175476071));
#291467=CARTESIAN_POINT('Ctrl Pts',(8.13178807675711,126.106249999506,-5.90808986649102));
#291468=CARTESIAN_POINT('Ctrl Pts',(6.21213331202013,126.256249999505,-8.55026797822134));
#291469=CARTESIAN_POINT('Ctrl Pts',(3.10606665601002,126.406249999505,-9.5594902125713));
#291470=CARTESIAN_POINT('Ctrl Pts',(-8.6008905916285E-14,126.556249999504,
-10.5687124469213));
#291471=CARTESIAN_POINT('Ctrl Pts',(-3.10606665601019,126.706249999504,
-9.5594902125713));
#291472=CARTESIAN_POINT('Ctrl Pts',(-6.2121333120203,126.856249999503,-8.55026797822134));
#291473=CARTESIAN_POINT('Ctrl Pts',(-8.13178807675728,127.006249999502,
-5.90808986649102));
#291474=CARTESIAN_POINT('Ctrl Pts',(-10.0514428414943,127.156249999502,
-3.2659117547607));
#291475=CARTESIAN_POINT('Ctrl Pts',(-10.0514428414943,127.306249999501,
2.46189346052968E-15));
#291476=CARTESIAN_POINT('Ctrl Pts',(-10.0514428414943,127.456249999501,
3.26591175476071));
#291477=CARTESIAN_POINT('Ctrl Pts',(-8.13178807675728,127.6062499995,5.90808986649102));
#291478=CARTESIAN_POINT('Ctrl Pts',(-6.2121333120203,127.756249999499,8.55026797822134));
#291479=CARTESIAN_POINT('Ctrl Pts',(-3.10606665601019,127.906249999499,
9.5594902125713));
#291480=CARTESIAN_POINT('Ctrl Pts',(-8.42841725782698E-14,128.056249999498,
10.5687124469213));
#291481=CARTESIAN_POINT('Ctrl Pts',(3.10606665601002,128.206249999498,9.5594902125713));
#291482=CARTESIAN_POINT('Ctrl Pts',(6.21213331202013,128.356249999497,8.55026797822134));
#291483=CARTESIAN_POINT('Ctrl Pts',(8.1317880767571,128.506249999496,5.90808986649102));
#291484=CARTESIAN_POINT('Ctrl Pts',(10.0514428414941,128.656249999496,3.2659117547607));
#291485=CARTESIAN_POINT('Ctrl Pts',(10.0514428414941,128.806249999495,-1.23094673026484E-15));
#291486=CARTESIAN_POINT('Ctrl Pts',(10.0514428414941,125.431249999509,-1.23094673026484E-15));
#291487=CARTESIAN_POINT('Ctrl Pts',(10.0514428414941,125.581249999508,-3.26591175476071));
#291488=CARTESIAN_POINT('Ctrl Pts',(8.13178807675711,125.731249999508,-5.90808986649102));
#291489=CARTESIAN_POINT('Ctrl Pts',(6.21213331202013,125.881249999507,-8.55026797822134));
#291490=CARTESIAN_POINT('Ctrl Pts',(3.10606665601002,126.031249999506,-9.5594902125713));
#291491=CARTESIAN_POINT('Ctrl Pts',(-8.57929422573273E-14,126.181249999506,
-10.5687124469213));
#291492=CARTESIAN_POINT('Ctrl Pts',(-3.10606665601019,126.331249999505,
-9.5594902125713));
#291493=CARTESIAN_POINT('Ctrl Pts',(-6.2121333120203,126.481249999505,-8.55026797822134));
#291494=CARTESIAN_POINT('Ctrl Pts',(-8.13178807675728,126.631249999504,
-5.90808986649102));
#291495=CARTESIAN_POINT('Ctrl Pts',(-10.0514428414943,126.781249999503,
-3.2659117547607));
#291496=CARTESIAN_POINT('Ctrl Pts',(-10.0514428414943,126.931249999503,
2.46189346052968E-15));
#291497=CARTESIAN_POINT('Ctrl Pts',(-10.0514428414943,127.081249999502,
3.26591175476071));
#291498=CARTESIAN_POINT('Ctrl Pts',(-8.13178807675728,127.231249999502,
5.90808986649102));
#291499=CARTESIAN_POINT('Ctrl Pts',(-6.2121333120203,127.381249999501,8.55026797822134));
#291500=CARTESIAN_POINT('Ctrl Pts',(-3.10606665601019,127.5312499995,9.5594902125713));
#291501=CARTESIAN_POINT('Ctrl Pts',(-8.4068208919312E-14,127.6812499995,
10.5687124469213));
#291502=CARTESIAN_POINT('Ctrl Pts',(3.10606665601002,127.831249999499,9.5594902125713));
#291503=CARTESIAN_POINT('Ctrl Pts',(6.21213331202013,127.981249999499,8.55026797822134));
#291504=CARTESIAN_POINT('Ctrl Pts',(8.1317880767571,128.131249999498,5.90808986649102));
#291505=CARTESIAN_POINT('Ctrl Pts',(10.0514428414941,128.281249999497,3.2659117547607));
#291506=CARTESIAN_POINT('Ctrl Pts',(10.0514428414941,128.431249999497,-1.23094673026484E-15));
#291507=CARTESIAN_POINT('Origin',(-8.79029313101884E-14,130.96875,0.));
#291508=CARTESIAN_POINT('',(-12.0000000000001,128.431249999496,-7.19625340030961E-14));
#291509=CARTESIAN_POINT('',(-12.0000000000001,128.806249999496,-1.6694244058475E-14));
#291510=CARTESIAN_POINT('',(-12.0000000000001,130.96875,-1.46957615897682E-15));
#291511=CARTESIAN_POINT('',(-7.3010839424065,128.868749999999,9.52334884722529));
#291512=CARTESIAN_POINT('Ctrl Pts',(-12.0000000000001,128.431249999496,
-3.80251385934116E-14));
#291513=CARTESIAN_POINT('Ctrl Pts',(-12.0000000000001,128.481970002,1.31839422452174));
#291514=CARTESIAN_POINT('Ctrl Pts',(-11.7827260639574,128.53512719973,2.62954328634065));
#291515=CARTESIAN_POINT('Ctrl Pts',(-10.9745647540102,128.636212850368,
4.99453327094218));
#291516=CARTESIAN_POINT('Ctrl Pts',(-10.4318751626277,128.683474543101,
6.04670312147143));
#291517=CARTESIAN_POINT('Ctrl Pts',(-9.05815403570474,128.774185332047,
7.95825182936078));
#291518=CARTESIAN_POINT('Ctrl Pts',(-8.23482414938436,128.821172544027,
8.8074960793686));
#291519=CARTESIAN_POINT('Ctrl Pts',(-7.30108394240603,128.868749999998,
9.52334884722502));
#291520=CARTESIAN_POINT('',(-11.8941677855641,128.86875,1.59021152330489));
#291521=CARTESIAN_POINT('Origin',(-8.66935348200203E-14,128.86875,0.));
#291522=CARTESIAN_POINT('Ctrl Pts',(-11.8941677855641,128.86875,1.59021152330492));
#291523=CARTESIAN_POINT('Ctrl Pts',(-11.9646919997276,128.84757520719,1.06271764974586));
#291524=CARTESIAN_POINT('Ctrl Pts',(-12.0000000000001,128.826697189287,
0.531495575654397));
#291525=CARTESIAN_POINT('Ctrl Pts',(-12.0000000000001,128.806249999496,
3.24740234702858E-14));
#291526=CARTESIAN_POINT('Origin',(-8.79029313101884E-14,130.96875,0.));
#291527=CARTESIAN_POINT('',(-12.0000000000001,125.431249999508,-2.53890049450429E-15));
#291528=CARTESIAN_POINT('',(-12.0000000000001,125.806249999508,7.85073803031321E-14));
#291529=CARTESIAN_POINT('',(-12.0000000000001,130.96875,-1.46957615897682E-15));
#291530=CARTESIAN_POINT('Ctrl Pts',(-12.0000000000001,125.431249999508,
-1.0547118733939E-14));
#291531=CARTESIAN_POINT('Ctrl Pts',(-12.0000000000001,125.489596886951,
1.51664423554858));
#291532=CARTESIAN_POINT('Ctrl Pts',(-11.7124672914376,125.55104013437,3.02034889816076));
#291533=CARTESIAN_POINT('Ctrl Pts',(-10.5808995167431,125.674745188536,
5.86821693033722));
#291534=CARTESIAN_POINT('Ctrl Pts',(-9.73743272163847,125.733338542766,
7.1814939780729));
#291535=CARTESIAN_POINT('Ctrl Pts',(-7.58142249067642,125.857439407559,
9.43349532883263));
#291536=CARTESIAN_POINT('Ctrl Pts',(-6.28242507135789,125.921600081592,
10.3440797672615));
#291537=CARTESIAN_POINT('Ctrl Pts',(-3.41418066711554,126.045560539419,
11.6098695739462));
#291538=CARTESIAN_POINT('Ctrl Pts',(-1.87371932800542,126.105456460553,
11.9555370942489));
#291539=CARTESIAN_POINT('Ctrl Pts',(1.23871898742655,126.231357235109,12.0360651439063));
#291540=CARTESIAN_POINT('Ctrl Pts',(2.7809719944347,126.292274471604,11.7757047301857));
#291541=CARTESIAN_POINT('Ctrl Pts',(5.71429353463594,126.414546669267,10.6704915883421));
#291542=CARTESIAN_POINT('Ctrl Pts',(7.07223692666379,126.47913085024,9.82322725908423));
#291543=CARTESIAN_POINT('Ctrl Pts',(9.35495050356998,126.604937420233,7.67387871961371));
#291544=CARTESIAN_POINT('Ctrl Pts',(10.2670744395895,126.663281529632,6.40239705975796));
#291545=CARTESIAN_POINT('Ctrl Pts',(11.561755155871,126.788326898164,3.57268807209495));
#291546=CARTESIAN_POINT('Ctrl Pts',(11.9280794377078,126.851890498091,2.03946880008667));
#291547=CARTESIAN_POINT('Ctrl Pts',(12.053496278001,126.974201142343,-1.0990717883848));
#291548=CARTESIAN_POINT('Ctrl Pts',(11.8043524772866,127.036581899792,-2.67438299002925));
#291549=CARTESIAN_POINT('Ctrl Pts',(10.7217182551911,127.162926241768,-5.60675502470455));
#291550=CARTESIAN_POINT('Ctrl Pts',(9.9108203693828,127.22192765558,-6.94021692903948));
#291551=CARTESIAN_POINT('Ctrl Pts',(7.80834131296282,127.345583714989,-9.24718977833398));
#291552=CARTESIAN_POINT('Ctrl Pts',(6.52853819589473,127.409909036468,-10.191117730139));
#291553=CARTESIAN_POINT('Ctrl Pts',(3.69184433991172,127.534430944573,-11.52394689137));
#291554=CARTESIAN_POINT('Ctrl Pts',(2.16489556008747,127.593678134542,-11.9056393604222));
#291555=CARTESIAN_POINT('Ctrl Pts',(-0.942572912478038,127.719377874731,
-12.0632149041181));
#291556=CARTESIAN_POINT('Ctrl Pts',(-2.49342240453255,127.781329203651,
-11.8402681046257));
#291557=CARTESIAN_POINT('Ctrl Pts',(-5.45863081898636,127.903003901638,
-10.8040734135506));
#291558=CARTESIAN_POINT('Ctrl Pts',(-6.83961692526329,127.967619763625,
-9.98719220398577));
#291559=CARTESIAN_POINT('Ctrl Pts',(-9.17288875238684,128.093835926364,
-7.89020427402746));
#291560=CARTESIAN_POINT('Ctrl Pts',(-10.1133256482652,128.152136931153,
-6.64212901323631));
#291561=CARTESIAN_POINT('Ctrl Pts',(-11.4754003004398,128.27686797732,-3.84248800492933));
#291562=CARTESIAN_POINT('Ctrl Pts',(-11.8782216827375,128.340681306605,
-2.31463600074324));
#291563=CARTESIAN_POINT('Ctrl Pts',(-11.9921423568023,128.411850799235,
-0.501701477445237));
#291564=CARTESIAN_POINT('Ctrl Pts',(-12.0000000000001,128.421604405312,
-0.250723482590127));
#291565=CARTESIAN_POINT('Ctrl Pts',(-12.0000000000001,128.431249999496,
1.73472347597681E-15));
#291566=CARTESIAN_POINT('Ctrl Pts',(-12.0000000000001,128.806249999496,
-4.57273108267486E-14));
#291567=CARTESIAN_POINT('Ctrl Pts',(-12.0000000000001,128.794332493682,
-0.309778589508634));
#291568=CARTESIAN_POINT('Ctrl Pts',(-11.9880049278405,128.78226205016,-0.619635141726521));
#291569=CARTESIAN_POINT('Ctrl Pts',(-11.8980136235725,128.736545834021,
-1.778723119345));
#291570=CARTESIAN_POINT('Ctrl Pts',(-11.7416705872724,128.702261315831,
-2.61910140635539));
#291571=CARTESIAN_POINT('Ctrl Pts',(-11.0465766482761,128.604085546726,
-4.94519098084889));
#291572=CARTESIAN_POINT('Ctrl Pts',(-10.3026821784156,128.542403594453,
-6.35108656262286));
#291573=CARTESIAN_POINT('Ctrl Pts',(-8.32158736574728,128.419673735816,
-8.78617588549032));
#291574=CARTESIAN_POINT('Ctrl Pts',(-7.10697201666228,128.355945463055,
-9.79471613563536));
#291575=CARTESIAN_POINT('Ctrl Pts',(-4.37245333378446,128.231097693156,
-11.281882612525));
#291576=CARTESIAN_POINT('Ctrl Pts',(-2.88126249839227,128.172799515821,
-11.751490889311));
#291577=CARTESIAN_POINT('Ctrl Pts',(0.235470080245203,128.04672503467,-12.1022565541906));
#291578=CARTESIAN_POINT('Ctrl Pts',(1.83268362734837,127.982116389507,-11.9650152362571));
#291579=CARTESIAN_POINT('Ctrl Pts',(4.84604017671202,127.860223556581,-11.0870123571411));
#291580=CARTESIAN_POINT('Ctrl Pts',(6.23714114056861,127.798661069928,-10.3684338391067));
#291581=CARTESIAN_POINT('Ctrl Pts',(8.67617998441893,127.672887425654,-8.43563337672419));
#291582=CARTESIAN_POINT('Ctrl Pts',(9.69864245837801,127.613427163644,-7.23687647571405));
#291583=CARTESIAN_POINT('Ctrl Pts',(11.2334836328764,127.489101896387,-4.50391835817245));
#291584=CARTESIAN_POINT('Ctrl Pts',(11.7266830329195,127.424831418766,-2.99354903217779));
#291585=CARTESIAN_POINT('Ctrl Pts',(12.0987618481939,127.301010723956,0.104097835807391));
#291586=CARTESIAN_POINT('Ctrl Pts',(11.9847153130956,127.242175748738,1.66055259173718));
#291587=CARTESIAN_POINT('Ctrl Pts',(11.1628945228536,127.115781636673,4.67896175004949));
#291588=CARTESIAN_POINT('Ctrl Pts',(10.4494920965024,127.052982022215,6.10824039252744));
#291589=CARTESIAN_POINT('Ctrl Pts',(8.52281591676635,126.930912282871,8.59046691788869));
#291590=CARTESIAN_POINT('Ctrl Pts',(7.33486129463653,126.867446574144,9.6246594640949));
#291591=CARTESIAN_POINT('Ctrl Pts',(4.63764878122555,126.742298608303,11.1757992658842));
#291592=CARTESIAN_POINT('Ctrl Pts',(3.15569205951511,126.683900424763,11.6810916275616));
#291593=CARTESIAN_POINT('Ctrl Pts',(0.0494360069800742,126.558249727994,
12.1039500516553));
#291594=CARTESIAN_POINT('Ctrl Pts',(-1.54667912891781,126.493685514498,
12.0048332356448));
#291595=CARTESIAN_POINT('Ctrl Pts',(-4.57443637444229,126.371210161175,
11.2014841669797));
#291596=CARTESIAN_POINT('Ctrl Pts',(-5.98050056719766,126.310620638141,
10.5181997613387));
#291597=CARTESIAN_POINT('Ctrl Pts',(-8.46866339045471,126.184652585968,
8.64483615362303));
#291598=CARTESIAN_POINT('Ctrl Pts',(-9.52315613199515,126.124486320596,
7.46732454508722));
#291599=CARTESIAN_POINT('Ctrl Pts',(-11.1224854645179,126.000734282678,
4.77022018048739));
#291600=CARTESIAN_POINT('Ctrl Pts',(-11.650494800803,125.936640580968,3.27575632643063));
#291601=CARTESIAN_POINT('Ctrl Pts',(-11.9586682352639,125.851029796291,
1.15055753302113));
#291602=CARTESIAN_POINT('Ctrl Pts',(-12.0000000000001,125.828372379491,
0.575039758716343));
#291603=CARTESIAN_POINT('Ctrl Pts',(-12.0000000000001,125.806249999508,
-9.29811783123569E-15));
#291604=CARTESIAN_POINT('Origin',(-8.79029313101884E-14,130.96875,0.));
#291605=CARTESIAN_POINT('',(-12.0000000000001,122.43124999952,-1.91922458638816E-14));
#291606=CARTESIAN_POINT('',(-12.0000000000001,122.80624999952,1.20810221360561E-15));
#291607=CARTESIAN_POINT('',(-12.0000000000001,130.96875,-1.46957615897682E-15));
#291608=CARTESIAN_POINT('Ctrl Pts',(-12.0000000000001,122.43124999952,2.62637134262889E-14));
#291609=CARTESIAN_POINT('Ctrl Pts',(-12.0000000000001,122.435732938321,
0.116527609076827));
#291610=CARTESIAN_POINT('Ctrl Pts',(-11.9983026721942,122.440239705659,
0.233123111782995));
#291611=CARTESIAN_POINT('Ctrl Pts',(-11.9486246694461,122.506405303043,
1.93686221448914));
#291612=CARTESIAN_POINT('Ctrl Pts',(-11.5878069745041,122.571015519303,
3.49907598592701));
#291613=CARTESIAN_POINT('Ctrl Pts',(-10.295123242127,122.697114835668,6.35682970576345));
#291614=CARTESIAN_POINT('Ctrl Pts',(-9.38960619474072,122.755412061665,
7.63113068561021));
#291615=CARTESIAN_POINT('Ctrl Pts',(-7.13326534584562,122.880240022951,
9.77561936761895));
#291616=CARTESIAN_POINT('Ctrl Pts',(-5.79976689993488,122.94398331222,10.621162644329));
#291617=CARTESIAN_POINT('Ctrl Pts',(-2.87341254255409,123.06675240564,11.75686397533));
#291618=CARTESIAN_POINT('Ctrl Pts',(-1.30723980981329,123.128371038424,
12.0321100813843));
#291619=CARTESIAN_POINT('Ctrl Pts',(1.81358360631128,123.254610997428,11.9625647420134));
#291620=CARTESIAN_POINT('Ctrl Pts',(3.33866915744452,123.314001523729,11.6295020408271));
#291621=CARTESIAN_POINT('Ctrl Pts',(6.20683349161236,123.437320363311,10.3905875210183));
#291622=CARTESIAN_POINT('Ctrl Pts',(7.51766930637064,123.501739063548,9.48544504376199));
#291623=CARTESIAN_POINT('Ctrl Pts',(9.69912485336729,123.626629113384,7.23527423550305));
#291624=CARTESIAN_POINT('Ctrl Pts',(10.5547516636117,123.685523610693,5.91771783856675));
#291625=CARTESIAN_POINT('Ctrl Pts',(11.7145004189305,123.811073663117,3.0310482601749));
#291626=CARTESIAN_POINT('Ctrl Pts',(12.0082060367235,123.873839015107,1.48965046616972));
#291627=CARTESIAN_POINT('Ctrl Pts',(11.9912446250076,123.995076604622,-1.65623689768775));
#291628=CARTESIAN_POINT('Ctrl Pts',(11.6661213753513,124.059693561683,-3.23022371496439));
#291629=CARTESIAN_POINT('Ctrl Pts',(10.4381304385326,124.186169495528,-6.11878703324379));
#291630=CARTESIAN_POINT('Ctrl Pts',(9.56305485397843,124.244532792525,-7.41229666342868));
#291631=CARTESIAN_POINT('Ctrl Pts',(7.35564800647638,124.36902414678,-9.60998003718757));
#291632=CARTESIAN_POINT('Ctrl Pts',(6.038725950634,124.432989253204,-10.4876680518474));
#291633=CARTESIAN_POINT('Ctrl Pts',(3.14054067387461,124.556362899663,-11.6875673834738));
#291634=CARTESIAN_POINT('Ctrl Pts',(1.58696921632692,124.617055746233,-11.9976591489136));
#291635=CARTESIAN_POINT('Ctrl Pts',(-1.52992798780065,124.743136886626,
-12.0022826425887));
#291636=CARTESIAN_POINT('Ctrl Pts',(-3.06356722876761,124.803200686683,
-11.7051236054165));
#291637=CARTESIAN_POINT('Ctrl Pts',(-5.96443528226193,124.926021949361,
-10.5321492263498));
#291638=CARTESIAN_POINT('Ctrl Pts',(-7.29891290370308,124.990539696528,
-9.6553811402027));
#291639=CARTESIAN_POINT('Ctrl Pts',(-9.53086438296879,125.115902420437,
-7.45483206289494));
#291640=CARTESIAN_POINT('Ctrl Pts',(-10.4146403136237,125.174446596594,
-6.16012410562965));
#291641=CARTESIAN_POINT('Ctrl Pts',(-11.6416510156975,125.299763148066,
-3.30137878322185));
#291642=CARTESIAN_POINT('Ctrl Pts',(-11.9715069422521,125.363044440324,
-1.76364841004787));
#291643=CARTESIAN_POINT('Ctrl Pts',(-11.9994118426542,125.425963812243,
-0.137215804927733));
#291644=CARTESIAN_POINT('Ctrl Pts',(-12.0000000000001,125.428611080214,
-0.0685949484236192));
#291645=CARTESIAN_POINT('Ctrl Pts',(-12.0000000000001,125.431249999508,
2.73285667600019E-15));
#291646=CARTESIAN_POINT('Ctrl Pts',(-12.0000000000001,125.806249999508,
-1.0547118733939E-14));
#291647=CARTESIAN_POINT('Ctrl Pts',(-12.0000000000001,125.769125942516,
-0.964986985673901));
#291648=CARTESIAN_POINT('Ctrl Pts',(-11.8836046085516,125.730603060961,
-1.92851526825847));
#291649=CARTESIAN_POINT('Ctrl Pts',(-11.2718009128407,125.627383811719,
-4.41276556604046));
#291650=CARTESIAN_POINT('Ctrl Pts',(-10.5889399812926,125.56332599208,-5.86512219781751));
#291651=CARTESIAN_POINT('Ctrl Pts',(-8.71656853591449,125.441944357557,
-8.39315212868226));
#291652=CARTESIAN_POINT('Ctrl Pts',(-7.55538743852935,125.378769778022,
-9.45195081641037));
#291653=CARTESIAN_POINT('Ctrl Pts',(-4.89580690723992,125.253368317505,
-11.0655482010172));
#291654=CARTESIAN_POINT('Ctrl Pts',(-3.42309837976009,125.194717237643,
-11.6059347670923));
#291655=CARTESIAN_POINT('Ctrl Pts',(-0.328008361997646,125.069518216469,
-12.0991251932609));
#291656=CARTESIAN_POINT('Ctrl Pts',(1.26618304560651,125.005031819417,-12.0371639804595));
#291657=CARTESIAN_POINT('Ctrl Pts',(4.30697724794929,124.882029110113,-11.3068065663843));
#291658=CARTESIAN_POINT('Ctrl Pts',(5.72744418487154,124.822223078081,-10.6578786238672));
#291659=CARTESIAN_POINT('Ctrl Pts',(8.26302605911904,124.696083445389,-8.842565323223));
#291660=CARTESIAN_POINT('Ctrl Pts',(9.34855021222853,124.635077726409,-7.68590015126261));
#291661=CARTESIAN_POINT('Ctrl Pts',(11.0095892765376,124.51191564796,-5.02418165010607));
#291662=CARTESIAN_POINT('Ctrl Pts',(11.5706872712687,124.448026028093,-3.54577376973066));
#291663=CARTESIAN_POINT('Ctrl Pts',(12.0900654713141,124.323409893459,-0.475311047824805));
#291664=CARTESIAN_POINT('Ctrl Pts',(12.0505338417015,124.265087752431,1.08637342597683));
#291665=CARTESIAN_POINT('Ctrl Pts',(11.3713292922706,124.138742241242,4.14985809937313));
#291666=CARTESIAN_POINT('Ctrl Pts',(10.7219775170637,124.074123727343,5.61853715041643));
#291667=CARTESIAN_POINT('Ctrl Pts',(8.90984038756518,123.952660229812,8.18700872245728));
#291668=CARTESIAN_POINT('Ctrl Pts',(7.77644366969167,123.8903211212,9.27037657699587));
#291669=CARTESIAN_POINT('Ctrl Pts',(5.15594158714334,123.764693450601,10.9472748861876));
#291670=CARTESIAN_POINT('Ctrl Pts',(3.69284093342787,123.70562855315,11.5234342032408));
#291671=CARTESIAN_POINT('Ctrl Pts',(0.609990526536278,123.580924634636,
12.087706928294));
#291672=CARTESIAN_POINT('Ctrl Pts',(-0.981399707504531,123.516551547435,
12.0632353700333));
#291673=CARTESIAN_POINT('Ctrl Pts',(-4.03434702382668,123.393057234344,
11.4068132083855));
#291674=CARTESIAN_POINT('Ctrl Pts',(-5.46918910028784,123.333876771955,
10.792557749552));
#291675=CARTESIAN_POINT('Ctrl Pts',(-8.05221336441863,123.207582119441,
9.03602339714975));
#291676=CARTESIAN_POINT('Ctrl Pts',(-9.16889223660466,123.145582038152,
7.90057035870083));
#291677=CARTESIAN_POINT('Ctrl Pts',(-10.8911261633591,123.023045994957,
5.27500816840282));
#291678=CARTESIAN_POINT('Ctrl Pts',(-11.4847996170347,122.959392917648,
3.81333328315813));
#291679=CARTESIAN_POINT('Ctrl Pts',(-11.9272030519174,122.865878822449,
1.52631316037461));
#291680=CARTESIAN_POINT('Ctrl Pts',(-12.0000000000001,122.835609410272,
0.763156065843486));
#291681=CARTESIAN_POINT('Ctrl Pts',(-12.0000000000001,122.80624999952,-9.43689570931383E-15));
#291682=CARTESIAN_POINT('Origin',(-8.79029313101884E-14,130.96875,0.));
#291683=CARTESIAN_POINT('',(-12.0000000000001,119.431249999532,8.29482724016328E-14));
#291684=CARTESIAN_POINT('',(-12.0000000000001,119.806249999532,-5.81888296038403E-14));
#291685=CARTESIAN_POINT('',(-12.0000000000001,130.96875,-1.46957615897682E-15));
#291686=CARTESIAN_POINT('Ctrl Pts',(-12.0000000000001,119.431249999532,
4.51721993144361E-14));
#291687=CARTESIAN_POINT('Ctrl Pts',(-12.0000000000001,119.443085102611,
0.307636647781991));
#291688=CARTESIAN_POINT('Ctrl Pts',(-11.9881702429117,119.455080866568,
0.615605725182721));
#291689=CARTESIAN_POINT('Ctrl Pts',(-11.8428535024459,119.529346228598,
2.4988117637302));
#291690=CARTESIAN_POINT('Ctrl Pts',(-11.4112356703933,119.593838282962,
4.03494972594653));
#291691=CARTESIAN_POINT('Ctrl Pts',(-9.9895647574198,119.719065609207,6.82812682905568));
#291692=CARTESIAN_POINT('Ctrl Pts',(-9.02238025756206,119.777697052648,
8.06296059190003));
#291693=CARTESIAN_POINT('Ctrl Pts',(-6.66877251628973,119.903084360385,
10.0970981483154));
#291694=CARTESIAN_POINT('Ctrl Pts',(-5.30386420471749,119.966277482577,
10.8762702578697));
#291695=CARTESIAN_POINT('Ctrl Pts',(-2.32256894648718,120.087701862772,
11.8797953199349));
#291696=CARTESIAN_POINT('Ctrl Pts',(-0.731034154377956,120.151679046811,
12.0826371615092));
#291697=CARTESIAN_POINT('Ctrl Pts',(2.39650174146898,120.278190531324,11.8595432877569));
#291698=CARTESIAN_POINT('Ctrl Pts',(3.90344614359641,120.336697353249,11.4522985786249));
#291699=CARTESIAN_POINT('Ctrl Pts',(6.70081111332831,120.460920120084,10.0779192792414));
#291700=CARTESIAN_POINT('Ctrl Pts',(7.96056234169184,120.525025626629,9.11563735429559));
#291701=CARTESIAN_POINT('Ctrl Pts',(10.034755997471,120.648813760085,6.76417815612786));
#291702=CARTESIAN_POINT('Ctrl Pts',(10.8306278056746,120.708932157215,5.39888360513246));
#291703=CARTESIAN_POINT('Ctrl Pts',(11.8478136055881,120.834888821484,2.45532321880896));
#291704=CARTESIAN_POINT('Ctrl Pts',(12.0654965891985,120.895533083184,0.907129236787544));
#291705=CARTESIAN_POINT('Ctrl Pts',(11.8985223670227,121.01797392093,-2.22129273422858));
#291706=CARTESIAN_POINT('Ctrl Pts',(11.5017561957471,121.08254188909,-3.77072795845864));
#291707=CARTESIAN_POINT('Ctrl Pts',(10.1437069246306,121.20821972362,-6.59628730733561));
#291708=CARTESIAN_POINT('Ctrl Pts',(9.20710805602347,121.266607157818,-7.85079237476785));
#291709=CARTESIAN_POINT('Ctrl Pts',(6.90141739958207,121.391737867082,-9.94008999640738));
#291710=CARTESIAN_POINT('Ctrl Pts',(5.55171625469305,121.455220721204,-10.7523786624008));
#291711=CARTESIAN_POINT('Ctrl Pts',(2.59730531844547,121.57733225951,-11.8218076510319));
#291712=CARTESIAN_POINT('Ctrl Pts',(1.01831374391615,121.640058343302,-12.0608691629107));
#291713=CARTESIAN_POINT('Ctrl Pts',(-2.10611302272581,121.766444060896,
-11.9144920478712));
#291714=CARTESIAN_POINT('Ctrl Pts',(-3.62219495019258,121.825306122227,
-11.5442874849623));
#291715=CARTESIAN_POINT('Ctrl Pts',(-6.45545251682648,121.949098843524,
-10.237397172522));
#291716=CARTESIAN_POINT('Ctrl Pts',(-7.74107895185393,122.013379111644,
-9.30337920646476));
#291717=CARTESIAN_POINT('Ctrl Pts',(-9.8693148984103,122.137738651117,-7.00227036660378));
#291718=CARTESIAN_POINT('Ctrl Pts',(-10.6952971812211,122.197160624728,
-5.66089624038417));
#291719=CARTESIAN_POINT('Ctrl Pts',(-11.7433895056935,122.318206030773,
-2.85503915504212));
#291720=CARTESIAN_POINT('Ctrl Pts',(-12.0000000000001,122.376129690943,
-1.43277391352303));
#291721=CARTESIAN_POINT('Ctrl Pts',(-12.0000000000001,122.43124999952,1.02695629777827E-14));
#291722=CARTESIAN_POINT('Ctrl Pts',(-12.0000000000001,122.80624999952,3.87190279838023E-14));
#291723=CARTESIAN_POINT('Ctrl Pts',(-12.0000000000001,122.776270810373,
-0.77926632248526));
#291724=CARTESIAN_POINT('Ctrl Pts',(-11.9240970835404,122.745345702254,
-1.55845810881199));
#291725=CARTESIAN_POINT('Ctrl Pts',(-11.4647743595056,122.650188016398,
-3.88270361944645));
#291726=CARTESIAN_POINT('Ctrl Pts',(-10.8516651212801,122.585588979386,
-5.36265231065594));
#291727=CARTESIAN_POINT('Ctrl Pts',(-9.10542162693431,122.463516494878,
-7.96836377170369));
#291728=CARTESIAN_POINT('Ctrl Pts',(-8.00084636519117,122.402264711622,
-9.07691102421512));
#291729=CARTESIAN_POINT('Ctrl Pts',(-5.42135353959798,122.276430632389,
-10.818934968515));
#291730=CARTESIAN_POINT('Ctrl Pts',(-3.9683912202721,122.216774796399,-11.4320744239647));
#291731=CARTESIAN_POINT('Ctrl Pts',(-0.899079105758544,122.092618513315,
-12.0691561732302));
#291732=CARTESIAN_POINT('Ctrl Pts',(0.688547655362349,122.028397661792,
-12.0829942621337));
#291733=CARTESIAN_POINT('Ctrl Pts',(3.75286824811511,121.904443290005,-11.5024782379153));
#291734=CARTESIAN_POINT('Ctrl Pts',(5.20225852444924,121.845730570123,-10.9237121701835));
#291735=CARTESIAN_POINT('Ctrl Pts',(7.83339548366492,121.719296722212,-9.22754491337953));
#291736=CARTESIAN_POINT('Ctrl Pts',(8.98177696327284,121.656131531625,-8.11399197794614));
#291737=CARTESIAN_POINT('Ctrl Pts',(10.765503539707,121.53426676251,-5.52585877431411));
#291738=CARTESIAN_POINT('Ctrl Pts',(11.3916501947226,121.470886064425,-4.08181518174822));
#291739=CARTESIAN_POINT('Ctrl Pts',(12.0549842028282,121.345656672567,-1.04218578921163));
#291740=CARTESIAN_POINT('Ctrl Pts',(12.0885988775717,121.287197801041,0.524022283936685));
#291741=CARTESIAN_POINT('Ctrl Pts',(11.552275802476,121.161680708871,3.61239839010473));
#291742=CARTESIAN_POINT('Ctrl Pts',(10.9757082466759,121.097136594324,5.10279256238657));
#291743=CARTESIAN_POINT('Ctrl Pts',(9.29592360412163,120.974496271202,7.74485796939733));
#291744=CARTESIAN_POINT('Ctrl Pts',(8.22018348407914,120.914162802098,8.87838696232961));
#291745=CARTESIAN_POINT('Ctrl Pts',(5.68195640921952,120.788140573221,10.6851216295968));
#291746=CARTESIAN_POINT('Ctrl Pts',(4.23931932328379,120.727734068384,11.335104213746));
#291747=CARTESIAN_POINT('Ctrl Pts',(1.18436608857568,120.60415861419,12.0440240616632));
#291748=CARTESIAN_POINT('Ctrl Pts',(-0.398660321286915,120.540123850784,
12.0955451771913));
#291749=CARTESIAN_POINT('Ctrl Pts',(-3.47312595407421,120.415759103507,
11.5900991948286));
#291750=CARTESIAN_POINT('Ctrl Pts',(-4.9367061390559,120.357336819557,11.0463519815541));
#291751=CARTESIAN_POINT('Ctrl Pts',(-7.6148521868453,120.230785634668,9.40995216834716));
#291752=CARTESIAN_POINT('Ctrl Pts',(-8.79431168759276,120.166330990559,
8.3182012252389));
#291753=CARTESIAN_POINT('Ctrl Pts',(-10.6375639830793,120.045157411401,
5.76737559864589));
#291754=CARTESIAN_POINT('Ctrl Pts',(-11.2948745591418,119.982073881331,
4.34118223713426));
#291755=CARTESIAN_POINT('Ctrl Pts',(-11.8869206891821,119.880796684097,
1.90099319300707));
#291756=CARTESIAN_POINT('Ctrl Pts',(-12.0000000000001,119.842841437673,
0.951142317236447));
#291757=CARTESIAN_POINT('Ctrl Pts',(-12.0000000000001,119.806249999532,
3.05311331771918E-14));
#291758=CARTESIAN_POINT('Origin',(-8.79029313101884E-14,130.96875,0.));
#291759=CARTESIAN_POINT('',(-12.0000000000001,116.431249999544,5.60947529935118E-14));
#291760=CARTESIAN_POINT('',(-12.0000000000001,116.806249999544,-9.27792157148178E-14));
#291761=CARTESIAN_POINT('',(-12.0000000000001,130.96875,-1.46957615897682E-15));
#291762=CARTESIAN_POINT('Ctrl Pts',(-12.0000000000001,116.431249999544,
-1.13797860024079E-14));
#291763=CARTESIAN_POINT('Ctrl Pts',(-12.0000000000001,116.450519136619,
0.500873773198305));
#291764=CARTESIAN_POINT('Ctrl Pts',(-11.9686420792505,116.470199718424,
1.00225366006863));
#291765=CARTESIAN_POINT('Ctrl Pts',(-11.7089771942863,116.552670958819,
3.06160585470905));
#291766=CARTESIAN_POINT('Ctrl Pts',(-11.2073618931561,116.616902187071,
4.56822045722642));
#291767=CARTESIAN_POINT('Ctrl Pts',(-9.6569671432679,116.741093193354,7.29263498896614));
#291768=CARTESIAN_POINT('Ctrl Pts',(-8.62681581704463,116.800707940273,
8.48631601045096));
#291769=CARTESIAN_POINT('Ctrl Pts',(-6.17596786986063,116.926529824619,
10.4048915410279));
#291770=CARTESIAN_POINT('Ctrl Pts',(-4.78126553006508,116.98784374612,11.1150124322844));
#291771=CARTESIAN_POINT('Ctrl Pts',(-1.7643663240107,117.10987988252,11.9751588681878));
#291772=CARTESIAN_POINT('Ctrl Pts',(-0.167335355273029,117.174481142232,
12.1032712798306));
#291773=CARTESIAN_POINT('Ctrl Pts',(2.94697813853509,117.300457769347,11.7352472424878));
#291774=CARTESIAN_POINT('Ctrl Pts',(4.43598025015591,117.3587653613,11.2571218222671));
#291775=CARTESIAN_POINT('Ctrl Pts',(7.1616829743892,117.483688624386,9.75464608989288));
#291776=CARTESIAN_POINT('Ctrl Pts',(8.36998823367536,117.547357307896,8.73992698006901));
#291777=CARTESIAN_POINT('Ctrl Pts',(10.3381688774826,117.669933227142,6.29353728685221));
#291778=CARTESIAN_POINT('Ctrl Pts',(11.0748361719961,117.731867143341,4.88206941562071));
#291779=CARTESIAN_POINT('Ctrl Pts',(11.9515988639792,117.858152680848,1.88433420432893));
#291780=CARTESIAN_POINT('Ctrl Pts',(12.0947296000952,117.917367252942,0.330082711652782));
#291781=CARTESIAN_POINT('Ctrl Pts',(11.7802236931385,118.040832147053,-2.77702219578679));
#291782=CARTESIAN_POINT('Ctrl Pts',(11.3138892864885,118.105213315824,-4.29899774607966));
#291783=CARTESIAN_POINT('Ctrl Pts',(9.82855002991664,118.229949232127,-7.05871424878508));
#291784=CARTESIAN_POINT('Ctrl Pts',(8.8304088319451,118.288983648681,-8.27343176695405));
#291785=CARTESIAN_POINT('Ctrl Pts',(6.42879631823223,118.414598265921,-10.2510567167147));
#291786=CARTESIAN_POINT('Ctrl Pts',(5.04912863955706,118.477008455727,-10.9963301642431));
#291787=CARTESIAN_POINT('Ctrl Pts',(2.04732776269366,118.598433851882,-11.9305466432727));
#291788=CARTESIAN_POINT('Ctrl Pts',(0.44986907729023,118.663052413097,-12.0965614184918));
#291789=CARTESIAN_POINT('Ctrl Pts',(-2.67412136042386,118.789420480815,
-11.8001856782115));
#291790=CARTESIAN_POINT('Ctrl Pts',(-4.17212545624418,118.847748257556,
-11.3573195903235));
#291791=CARTESIAN_POINT('Ctrl Pts',(-6.93396204596735,118.972343476991,
-9.91837487743489));
#291792=CARTESIAN_POINT('Ctrl Pts',(-8.16816599184413,119.036246259063,
-8.92945641981678));
#291793=CARTESIAN_POINT('Ctrl Pts',(-10.1895003983347,119.159444745716,
-6.5300423601243));
#291794=CARTESIAN_POINT('Ctrl Pts',(-10.9558841274651,119.22039573402,-5.14160249984191));
#291795=CARTESIAN_POINT('Ctrl Pts',(-11.80930185404,119.334044878749,-2.46474708173146));
#291796=CARTESIAN_POINT('Ctrl Pts',(-12.0000000000001,119.383732705891,
-1.23514436925128));
#291797=CARTESIAN_POINT('Ctrl Pts',(-12.0000000000001,119.431249999532,
-3.27515792264421E-14));
#291798=CARTESIAN_POINT('Ctrl Pts',(-12.0000000000001,119.806249999532,
2.692290834716E-14));
#291799=CARTESIAN_POINT('Ctrl Pts',(-12.0000000000001,119.783277972883,
-0.597125113647374));
#291800=CARTESIAN_POINT('Ctrl Pts',(-11.9554325127281,119.759730929568,
-1.19471611211129));
#291801=CARTESIAN_POINT('Ctrl Pts',(-11.6308449637883,119.672791989272,
-3.34910515005578));
#291802=CARTESIAN_POINT('Ctrl Pts',(-11.0897504983799,119.608334559506,
-4.84877198070028));
#291803=CARTESIAN_POINT('Ctrl Pts',(-9.47454580744222,119.485186418556,
-7.52502068711062));
#291804=CARTESIAN_POINT('Ctrl Pts',(-8.42662162912825,119.42557711517,-8.68245593268385));
#291805=CARTESIAN_POINT('Ctrl Pts',(-5.92843279303923,119.299391062744,
-10.5511886788847));
#291806=CARTESIAN_POINT('Ctrl Pts',(-4.49594034728034,119.238114606867,
-11.2365595976314));
#291807=CARTESIAN_POINT('Ctrl Pts',(-1.4555755876238,119.115129268884,-12.0138062962249));
#291808=CARTESIAN_POINT('Ctrl Pts',(0.122259056921303,119.051304516797,
-12.1010385489323));
#291809=CARTESIAN_POINT('Ctrl Pts',(3.20537086773915,118.926590024272,-11.6671580584952));
#291810=CARTESIAN_POINT('Ctrl Pts',(4.68230336517048,118.868287043019,-11.1567464555144));
#291811=CARTESIAN_POINT('Ctrl Pts',(7.3959683167439,118.742051657471,-9.58251626242619));
#291812=CARTESIAN_POINT('Ctrl Pts',(8.59852163498118,118.677435153814,-8.5200164017129));
#291813=CARTESIAN_POINT('Ctrl Pts',(10.4975241771352,118.555791084917,-6.01760343772505));
#291814=CARTESIAN_POINT('Ctrl Pts',(11.1871642645573,118.493784188957,-4.6105778085268));
#291815=CARTESIAN_POINT('Ctrl Pts',(11.9938522491681,118.368094869886,-1.60557179364514));
#291816=CARTESIAN_POINT('Ctrl Pts',(12.1007908177156,118.308875546012,-0.0354984191383897));
#291817=CARTESIAN_POINT('Ctrl Pts',(11.7061277760934,118.184326743795,3.07373650387339));
#291818=CARTESIAN_POINT('Ctrl Pts',(11.2020091660397,118.119994177238,4.5821718769257));
#291819=CARTESIAN_POINT('Ctrl Pts',(9.6542340162482,117.996361433865,7.29292631911161));
#291820=CARTESIAN_POINT('Ctrl Pts',(8.63516107596953,117.937335124396,8.47496175593411));
#291821=CARTESIAN_POINT('Ctrl Pts',(6.17874626117698,117.81099789906,10.4075496139555));
#291822=CARTESIAN_POINT('Ctrl Pts',(4.75697882722234,117.748673835196,11.1294576150518));
#291823=CARTESIAN_POINT('Ctrl Pts',(1.73247376269937,117.626330035357,11.9765439283481));
#291824=CARTESIAN_POINT('Ctrl Pts',(0.160766521532632,117.562753141943,
12.100123861986));
#291825=CARTESIAN_POINT('Ctrl Pts',(-2.93016092852451,117.43772250017,11.7395612500877));
#291826=CARTESIAN_POINT('Ctrl Pts',(-4.42060094658391,117.379384307779,
11.2632781652628));
#291827=CARTESIAN_POINT('Ctrl Pts',(-7.16846560687761,117.253556389344,
9.75325728399708));
#291828=CARTESIAN_POINT('Ctrl Pts',(-8.39282136547194,117.188969784549,
8.72202340899157));
#291829=CARTESIAN_POINT('Ctrl Pts',(-10.3476250584071,117.06672636511,6.27120636193096));
#291830=CARTESIAN_POINT('Ctrl Pts',(-11.0701893390789,117.005761656376,
4.88390755713557));
#291831=CARTESIAN_POINT('Ctrl Pts',(-11.8352255782078,116.896502075798,
2.29243572099499));
#291832=CARTESIAN_POINT('Ctrl Pts',(-12.0000000000001,116.850419884796,
1.14813325590528));
#291833=CARTESIAN_POINT('Ctrl Pts',(-12.0000000000001,116.806249999544,
1.63757896132211E-14));
#291834=CARTESIAN_POINT('Origin',(-8.79029313101884E-14,130.96875,0.));
#291835=CARTESIAN_POINT('',(-12.0000000000001,113.431249999556,-1.70623322603542E-15));
#291836=CARTESIAN_POINT('',(-12.0000000000001,113.806249999556,-1.1130606243825E-13));
#291837=CARTESIAN_POINT('',(-12.0000000000001,130.96875,-1.46957615897682E-15));
#291838=CARTESIAN_POINT('Ctrl Pts',(-12.0000000000001,113.431249999556,
5.82867087928207E-15));
#291839=CARTESIAN_POINT('Ctrl Pts',(-12.0000000000001,113.457825190305,
0.690784232431625));
#291840=CARTESIAN_POINT('Ctrl Pts',(-11.9403554096789,113.485156143997,
1.38183374397962));
#291841=CARTESIAN_POINT('Ctrl Pts',(-11.5514681472104,113.575642332941,
3.60753621479684));
#291842=CARTESIAN_POINT('Ctrl Pts',(-10.9828317388839,113.63948040642,5.08215484118498));
#291843=CARTESIAN_POINT('Ctrl Pts',(-9.30767226272974,113.762501690871,
7.73562560296991));
#291844=CARTESIAN_POINT('Ctrl Pts',(-8.21499357640178,113.823722415958,
8.88744539519899));
#291845=CARTESIAN_POINT('Ctrl Pts',(-5.66850236442309,113.949899202563,
10.6893059180563));
#291846=CARTESIAN_POINT('Ctrl Pts',(-4.24472700301189,114.009547185458,
11.3302881273245));
#291847=CARTESIAN_POINT('Ctrl Pts',(-1.20105788221068,114.132666187656,
12.0437244646561));
#291848=CARTESIAN_POINT('Ctrl Pts',(0.392567991437235,114.197129708379,
12.0970917713889));
#291849=CARTESIAN_POINT('Ctrl Pts',(3.48493930206807,114.322218755539,11.587619026558));
#291850=CARTESIAN_POINT('Ctrl Pts',(4.95547101554945,114.38095050263,11.0390659981908));
#291851=CARTESIAN_POINT('Ctrl Pts',(7.6061616336417,114.506404940095,9.41100456735867));
#291852=CARTESIAN_POINT('Ctrl Pts',(8.76103716219917,114.569507126276,8.34657176380249));
#291853=CARTESIAN_POINT('Ctrl Pts',(10.6206625015808,114.690723095543,5.80796595342873));
#291854=CARTESIAN_POINT('Ctrl Pts',(11.2963358913733,114.755096313423,4.35022984652544));
#291855=CARTESIAN_POINT('Ctrl Pts',(12.0293491926827,114.881641011308,1.29905112196894));
#291856=CARTESIAN_POINT('Ctrl Pts',(12.0964796858635,114.94007598164,-0.260766983788003));
#291857=CARTESIAN_POINT('Ctrl Pts',(11.6316057612974,115.064417264866,-3.34179484746409));
#291858=CARTESIAN_POINT('Ctrl Pts',(11.0954841507373,115.128464233674,-4.83240810857913));
#291859=CARTESIAN_POINT('Ctrl Pts',(9.48106461331453,115.252075785788,-7.52095764001368));
#291860=CARTESIAN_POINT('Ctrl Pts',(8.41901860617005,115.312432377127,-8.69341978411619));
#291861=CARTESIAN_POINT('Ctrl Pts',(5.9192982166187,115.438443734786,-10.5526971298546));
#291862=CARTESIAN_POINT('Ctrl Pts',(4.50972010974552,115.498827989115,-11.2276343318953));
#291863=CARTESIAN_POINT('Ctrl Pts',(1.47870553517511,115.621435104166,-12.0132767706304));
#291864=CARTESIAN_POINT('Ctrl Pts',(-0.117019989849763,115.68598355757,
-12.1033683611737));
#291865=CARTESIAN_POINT('Ctrl Pts',(-3.22065113350542,115.811528074544,
-11.6634342756433));
#291866=CARTESIAN_POINT('Ctrl Pts',(-4.7003849565096,115.869973461379,-11.1496479264714));
#291867=CARTESIAN_POINT('Ctrl Pts',(-7.38857458390202,115.995186606646,
-9.58334783932789));
#291868=CARTESIAN_POINT('Ctrl Pts',(-8.57009823916183,116.05858483444,-8.54314197267345));
#291869=CARTESIAN_POINT('Ctrl Pts',(-10.4837014045556,116.180491570798,
-6.04977764603272));
#291870=CARTESIAN_POINT('Ctrl Pts',(-11.1897627199188,116.243581245614,
-4.61491991065847));
#291871=CARTESIAN_POINT('Ctrl Pts',(-11.8650162131259,116.349694596727,
-2.07605764573233));
#291872=CARTESIAN_POINT('Ctrl Pts',(-12.0000000000001,116.391271532176,
-1.03918331784912));
#291873=CARTESIAN_POINT('Ctrl Pts',(-12.0000000000001,116.431249999544,
4.16333634234434E-15));
#291874=CARTESIAN_POINT('Ctrl Pts',(-12.0000000000001,116.806249999544,
2.76861866765898E-14));
#291875=CARTESIAN_POINT('Ctrl Pts',(-12.0000000000001,116.79048398263,-0.40981515411806));
#291876=CARTESIAN_POINT('Ctrl Pts',(-11.979007200241,116.774437557422,-0.82009814833851));
#291877=CARTESIAN_POINT('Ctrl Pts',(-11.7759002586227,116.696021448289,
-2.79241977131035));
#291878=CARTESIAN_POINT('Ctrl Pts',(-11.309428417977,116.631851765499,-4.30885338971805));
#291879=CARTESIAN_POINT('Ctrl Pts',(-9.83047366907497,116.50777186963,-7.05359202791613));
#291880=CARTESIAN_POINT('Ctrl Pts',(-8.84066915635196,116.449162423424,
-8.26038103683867));
#291881=CARTESIAN_POINT('Ctrl Pts',(-6.42689296455462,116.322691881841,
-10.2572630045548));
#291882=CARTESIAN_POINT('Ctrl Pts',(-5.01622766426787,116.259160670949,
-11.0160469934526));
#291883=CARTESIAN_POINT('Ctrl Pts',(-2.00853060107773,116.137496769046,
-11.9328865761613));
#291884=CARTESIAN_POINT('Ctrl Pts',(-0.443768785237827,116.074200823988,
-12.0925909409474));
#291885=CARTESIAN_POINT('Ctrl Pts',(2.65392175167885,115.948896609605,-11.80542678572));
#291886=CARTESIAN_POINT('Ctrl Pts',(4.15771200471099,115.890365913736,-11.3633123313233));
#291887=CARTESIAN_POINT('Ctrl Pts',(6.9386714237031,115.764980553746,-9.91745581711915));
#291888=CARTESIAN_POINT('Ctrl Pts',(8.18390177819024,115.700458739542,-8.91767835283168));
#291889=CARTESIAN_POINT('Ctrl Pts',(10.1932370278195,115.577663391961,-6.51870429084006));
#291890=CARTESIAN_POINT('Ctrl Pts',(10.9481940148213,115.517561718441,-5.15099467981093));
#291891=CARTESIAN_POINT('Ctrl Pts',(11.9033774238926,115.391488981224,-2.18427134454457));
#291892=CARTESIAN_POINT('Ctrl Pts',(12.0866899624146,115.330838674002,-0.610980294446826));
#291893=CARTESIAN_POINT('Ctrl Pts',(11.8376023441408,115.207435578478,2.51577393725414));
#291894=CARTESIAN_POINT('Ctrl Pts',(11.4080289538783,115.143460160531,4.03914695105162));
#291895=CARTESIAN_POINT('Ctrl Pts',(9.99673848720598,115.018986808815,6.81609837161942));
#291896=CARTESIAN_POINT('Ctrl Pts',(9.03556009573234,114.960616136635,8.04689953179336));
#291897=CARTESIAN_POINT('Ctrl Pts',(6.66537138938319,114.834122177736,10.1047594233466));
#291898=CARTESIAN_POINT('Ctrl Pts',(5.26778424110486,114.769505796758,10.8988130867691));
#291899=CARTESIAN_POINT('Ctrl Pts',(2.27957664384873,114.648300534033,11.883608380707));
#291900=CARTESIAN_POINT('Ctrl Pts',(0.722438874997024,114.585473265916,
12.0787176302905));
#291901=CARTESIAN_POINT('Ctrl Pts',(-2.38105346608099,114.459934363625,
11.863901263394));
#291902=CARTESIAN_POINT('Ctrl Pts',(-3.89783877408231,114.401062257605,
11.4554995754585));
#291903=CARTESIAN_POINT('Ctrl Pts',(-6.71033303018463,114.276146264562,
10.0727879054382));
#291904=CARTESIAN_POINT('Ctrl Pts',(-7.97522204452457,114.21172148225,9.10414927996976));
#291905=CARTESIAN_POINT('Ctrl Pts',(-10.0370462972033,114.08842795567,6.75646747682689));
#291906=CARTESIAN_POINT('Ctrl Pts',(-10.8234227591233,114.029005854449,
5.40792805678477));
#291907=CARTESIAN_POINT('Ctrl Pts',(-11.7747831448269,113.912041481627,
2.67672150532812));
#291908=CARTESIAN_POINT('Ctrl Pts',(-12.0000000000001,113.857888696239,
1.34227437121494));
#291909=CARTESIAN_POINT('Ctrl Pts',(-12.0000000000001,113.806249999556,
9.71445146547012E-15));
#291910=CARTESIAN_POINT('Origin',(-8.79029313101884E-14,130.96875,0.));
#291911=CARTESIAN_POINT('',(-12.0000000000001,110.431249999568,-1.01716837888022E-14));
#291912=CARTESIAN_POINT('',(-12.0000000000001,110.806249999568,3.54084502355313E-16));
#291913=CARTESIAN_POINT('',(-12.0000000000001,130.96875,-1.46957615897682E-15));
#291914=CARTESIAN_POINT('Ctrl Pts',(-12.0000000000001,110.431249999568,
-1.74860126378462E-14));
#291915=CARTESIAN_POINT('Ctrl Pts',(-12.0000000000001,110.465115924226,
0.880296476203017));
#291916=CARTESIAN_POINT('Ctrl Pts',(-11.9031394395545,110.500166049423,
1.75990265488635));
#291917=CARTESIAN_POINT('Ctrl Pts',(-11.3692619648579,110.598537238417,
4.14345429566384));
#291918=CARTESIAN_POINT('Ctrl Pts',(-10.7356906174076,110.661850372262,
5.58332922324425));
#291919=CARTESIAN_POINT('Ctrl Pts',(-8.93782980140339,110.783554748739,
8.16270075587147));
#291920=CARTESIAN_POINT('Ctrl Pts',(-7.78210399224986,110.847011607531,
9.27113220442497));
#291921=CARTESIAN_POINT('Ctrl Pts',(-5.13984413787133,110.973474930871,
10.9532298014104));
#291922=CARTESIAN_POINT('Ctrl Pts',(-3.68709432736107,111.032103901031,
11.523741709725));
#291923=CARTESIAN_POINT('Ctrl Pts',(-0.620285349530542,111.156158930108,
12.0865763507926));
#291924=CARTESIAN_POINT('Ctrl Pts',(0.966336225591075,111.220339121004,
12.0638434327127));
#291925=CARTESIAN_POINT('Ctrl Pts',(4.03235325847998,111.344362115236,11.4098263448967));
#291926=CARTESIAN_POINT('Ctrl Pts',(5.48291136998425,111.404179853104,10.7880339859718));
#291927=CARTESIAN_POINT('Ctrl Pts',(8.05274987745621,111.530059705669,9.03079685556067));
#291928=CARTESIAN_POINT('Ctrl Pts',(9.15056396922682,111.591080896714,7.91637343568581));
#291929=CARTESIAN_POINT('Ctrl Pts',(10.8812710005861,111.713290272981,5.30205556549628));
#291930=CARTESIAN_POINT('Ctrl Pts',(11.4858356836687,111.777879619812,3.81958246250681));
#291931=CARTESIAN_POINT('Ctrl Pts',(12.0770307530136,111.903732565958,0.740305302302331));
#291932=CARTESIAN_POINT('Ctrl Pts',(12.0715928814009,111.962064297098,-0.824235712880048));
#291933=CARTESIAN_POINT('Ctrl Pts',(11.4636098970648,112.08707745876,-3.87622914728557));
#291934=CARTESIAN_POINT('Ctrl Pts',(10.8623097381496,112.150669900599,-5.33384983312881));
#291935=CARTESIAN_POINT('Ctrl Pts',(9.12567953174611,112.273052622388,-7.95074901703718));
#291936=CARTESIAN_POINT('Ctrl Pts',(8.00161470651909,112.335310435219,-9.08112915652761));
#291937=CARTESIAN_POINT('Ctrl Pts',(5.40736674584077,112.461639222265,-10.8236510627333));
#291938=CARTESIAN_POINT('Ctrl Pts',(3.96912835756686,112.520695384853,-11.4296579216072));
#291939=CARTESIAN_POINT('Ctrl Pts',(0.91344063540796,112.644300549689,-12.0684562331533));
#291940=CARTESIAN_POINT('Ctrl Pts',(-0.677155773912495,112.708641526006,
-12.0840159153029));
#291941=CARTESIAN_POINT('Ctrl Pts',(-3.75695067726136,112.833221846805,
-11.5028231922881));
#291942=CARTESIAN_POINT('Ctrl Pts',(-5.21772308801828,112.892408916726,
-10.9181014267066));
#291943=CARTESIAN_POINT('Ctrl Pts',(-7.82876549740021,113.018085923719,
-9.22610798019146));
#291944=CARTESIAN_POINT('Ctrl Pts',(-8.955499396414,113.080158694416,-8.13690020602289));
#291945=CARTESIAN_POINT('Ctrl Pts',(-10.752452768734,113.201766616298,-5.55974102688885));
#291946=CARTESIAN_POINT('Ctrl Pts',(-11.3934535376065,113.266383763236,
-4.08838410163288));
#291947=CARTESIAN_POINT('Ctrl Pts',(-11.909628104702,113.364715251788,-1.70011239393634));
#291948=CARTESIAN_POINT('Ctrl Pts',(-12.0000000000001,113.398538036134,
-0.850300897476276));
#291949=CARTESIAN_POINT('Ctrl Pts',(-12.0000000000001,113.431249999556,
-6.21724893790088E-14));
#291950=CARTESIAN_POINT('Ctrl Pts',(-12.0000000000001,113.806249999556,
6.10622663543836E-14));
#291951=CARTESIAN_POINT('Ctrl Pts',(-12.0000000000001,113.797455107568,
-0.228610690666172));
#291952=CARTESIAN_POINT('Ctrl Pts',(-11.9934672441515,113.788570061458,
-0.45744218831683));
#291953=CARTESIAN_POINT('Ctrl Pts',(-11.8898190120987,113.717659267,-2.26698993984803));
#291954=CARTESIAN_POINT('Ctrl Pts',(-11.4872988731828,113.653101432803,
-3.81429216865722));
#291955=CARTESIAN_POINT('Ctrl Pts',(-10.1187640137248,113.527495091212,
-6.63458618622984));
#291956=CARTESIAN_POINT('Ctrl Pts',(-9.17714746409585,113.469078172581,
-7.88587738051025));
#291957=CARTESIAN_POINT('Ctrl Pts',(-6.86355088241269,113.343902531598,
-9.96618318978778));
#291958=CARTESIAN_POINT('Ctrl Pts',(-5.51130420365368,113.280464935998,
-10.7730647239246));
#291959=CARTESIAN_POINT('Ctrl Pts',(-2.55243275192805,113.15846339173,-11.8317281566572));
#291960=CARTESIAN_POINT('Ctrl Pts',(-0.97137790623552,113.095543061264,
-12.064889759129));
#291961=CARTESIAN_POINT('Ctrl Pts',(2.15358968078377,112.969135467026,-11.9060031991555));
#291962=CARTESIAN_POINT('Ctrl Pts',(3.66819178657938,112.910343101329,-11.5297558769136));
#291963=CARTESIAN_POINT('Ctrl Pts',(6.49566732729766,112.786477290939,-10.2118332717201));
#291964=CARTESIAN_POINT('Ctrl Pts',(7.77712174052835,112.722223028237,-9.27316675891725));
#291965=CARTESIAN_POINT('Ctrl Pts',(9.89660650128791,112.597953813618,-6.96381187199637));
#291966=CARTESIAN_POINT('Ctrl Pts',(10.7177142680202,112.538429915866,-5.61854633965747));
#291967=CARTESIAN_POINT('Ctrl Pts',(11.7950102695258,112.412635919089,-2.69874525153756));
#291968=CARTESIAN_POINT('Ctrl Pts',(12.0447056237293,112.351178829674,-1.15333520888798));
#291969=CARTESIAN_POINT('Ctrl Pts',(11.9409784320375,112.229225628947,1.98296153828977));
#291970=CARTESIAN_POINT('Ctrl Pts',(11.574318636668,112.164619830901,3.54316225105717));
#291971=CARTESIAN_POINT('Ctrl Pts',(10.2710279476328,112.038586094515,6.39576490361487));
#291972=CARTESIAN_POINT('Ctrl Pts',(9.36048981331488,111.980285079213,7.66688091650389));
#291973=CARTESIAN_POINT('Ctrl Pts',(7.09613388102823,111.855405387036,9.80251350578982));
#291974=CARTESIAN_POINT('Ctrl Pts',(5.75996790521609,111.791701845441,10.6427135154324));
#291975=CARTESIAN_POINT('Ctrl Pts',(2.82903220130612,111.66903620831,11.7677579487339));
#291976=CARTESIAN_POINT('Ctrl Pts',(1.26078481853545,111.607249816787,12.0372005843419));
#291977=CARTESIAN_POINT('Ctrl Pts',(-1.86064935753329,111.480985152024,
11.9553197569415));
#291978=CARTESIAN_POINT('Ctrl Pts',(-3.38429918801148,111.421691090299,
11.6162905055771));
#291979=CARTESIAN_POINT('Ctrl Pts',(-6.24692957529679,111.298293293233,
10.3664383288339));
#291980=CARTESIAN_POINT('Ctrl Pts',(-7.55376660389433,111.233894356657,
9.45662322434075));
#291981=CARTESIAN_POINT('Ctrl Pts',(-9.72673952276036,111.109086673137,
7.19824128289136));
#291982=CARTESIAN_POINT('Ctrl Pts',(-10.5776405378452,111.050118849626,
5.87687081016613));
#291983=CARTESIAN_POINT('Ctrl Pts',(-11.7125327347171,110.926016024765,
3.0197434655804));
#291984=CARTESIAN_POINT('Ctrl Pts',(-12.0000000000001,110.864590449283,
1.51647689596978));
#291985=CARTESIAN_POINT('Ctrl Pts',(-12.0000000000001,110.806249999568,
-2.22044604925031E-14));
#291986=CARTESIAN_POINT('Origin',(-8.79029313101884E-14,130.96875,0.));
#291987=CARTESIAN_POINT('',(-12.0000000000001,107.43124999958,-1.00342610070077E-13));
#291988=CARTESIAN_POINT('',(-12.0000000000001,107.80624999958,1.16164430694665E-14));
#291989=CARTESIAN_POINT('',(-12.0000000000001,130.96875,-1.46957615897682E-15));
#291990=CARTESIAN_POINT('Ctrl Pts',(-12.0000000000001,107.43124999958,-2.35922392732846E-14));
#291991=CARTESIAN_POINT('Ctrl Pts',(-12.0000000000001,107.472475829027,
1.0716067184754));
#291992=CARTESIAN_POINT('Ctrl Pts',(-11.8564608278089,107.515392780944,
2.14053305265728));
#291993=CARTESIAN_POINT('Ctrl Pts',(-11.1605739263003,107.621569699177,
4.6743434535674));
#291994=CARTESIAN_POINT('Ctrl Pts',(-10.4632702917257,107.683319400101,
6.0767941236516));
#291995=CARTESIAN_POINT('Ctrl Pts',(-8.5512486899399,107.805106347455,8.56729714134744));
#291996=CARTESIAN_POINT('Ctrl Pts',(-7.34357041189055,107.869719085032,
9.62258470436895));
#291997=CARTESIAN_POINT('Ctrl Pts',(-4.62189680058411,107.995863404523,
11.1819618222427));
#291998=CARTESIAN_POINT('Ctrl Pts',(-3.14182651482416,108.054160447384,
11.6844830099114));
#291999=CARTESIAN_POINT('Ctrl Pts',(-0.0568141277773715,108.178951819832,
12.1014150897439));
#292000=CARTESIAN_POINT('Ctrl Pts',(1.51967651284923,108.242722205819,12.0057583846512));
#292001=CARTESIAN_POINT('Ctrl Pts',(4.5564574303511,108.365562574341,11.2123528821052));
#292002=CARTESIAN_POINT('Ctrl Pts',(5.98650151062605,108.427067136739,10.5185617850649));
#292003=CARTESIAN_POINT('Ctrl Pts',(8.47510348932741,108.553289670874,8.63509949614269));
#292004=CARTESIAN_POINT('Ctrl Pts',(9.51639107407667,108.612749709332,7.47198794670194));
#292005=CARTESIAN_POINT('Ctrl Pts',(11.116123688399,108.736013143636,4.78771517132547));
#292006=CARTESIAN_POINT('Ctrl Pts',(11.6487272945608,108.800444999749,3.28595424396765));
#292007=CARTESIAN_POINT('Ctrl Pts',(12.0990450148902,108.92539154911,0.184463751769529));
#292008=CARTESIAN_POINT('Ctrl Pts',(12.0210207858086,108.984237724039,-1.38417049431514));
#292009=CARTESIAN_POINT('Ctrl Pts',(11.2707328709427,109.10976338588,-4.40324796613719));
#292010=CARTESIAN_POINT('Ctrl Pts',(10.6059494256205,109.17266439157,-5.82504154546219));
#292011=CARTESIAN_POINT('Ctrl Pts',(8.74928869642534,109.293831307012,-8.36566466196085));
#292012=CARTESIAN_POINT('Ctrl Pts',(7.56355668864608,109.358446893393,-9.45127849098679));
#292013=CARTESIAN_POINT('Ctrl Pts',(4.87605914739465,109.48496203341,-11.073291084806));
#292014=CARTESIAN_POINT('Ctrl Pts',(3.40927519642272,109.543341920951,-11.609074510916));
#292015=CARTESIAN_POINT('Ctrl Pts',(0.332653773135498,109.667793871786,
-12.0974309104079));
#292016=CARTESIAN_POINT('Ctrl Pts',(-1.24920411698429,109.731781367575,
-12.0373623932641));
#292017=CARTESIAN_POINT('Ctrl Pts',(-4.30075360512462,109.855219137329,
-11.3121123245655));
#292018=CARTESIAN_POINT('Ctrl Pts',(-5.74099588501373,109.915819683157,
-10.6537031827515));
#292019=CARTESIAN_POINT('Ctrl Pts',(-8.26972566093404,110.041882442436,
-8.83219195748779));
#292020=CARTESIAN_POINT('Ctrl Pts',(-9.33885324364083,110.10202934897,-7.69296290720051));
#292021=CARTESIAN_POINT('Ctrl Pts',(-11.0033260464683,110.224793971897,
-5.04269138549187));
#292022=CARTESIAN_POINT('Ctrl Pts',(-11.5714789179734,110.289320479752,
-3.55002077741768));
#292023=CARTESIAN_POINT('Ctrl Pts',(-11.9446631888315,110.379350140444,
-1.33108289701475));
#292024=CARTESIAN_POINT('Ctrl Pts',(-12.0000000000001,110.405652480965,
-0.665371037497507));
#292025=CARTESIAN_POINT('Ctrl Pts',(-12.0000000000001,110.431249999568,
-5.02375918642883E-14));
#292026=CARTESIAN_POINT('Ctrl Pts',(-12.0000000000001,110.806249999568,
2.17774516368745E-15));
#292027=CARTESIAN_POINT('Ctrl Pts',(-12.0000000000001,110.804838357927,
-0.0366936138490478));
#292028=CARTESIAN_POINT('Ctrl Pts',(-11.999831697421,110.803424321145,-0.073394801155502));
#292029=CARTESIAN_POINT('Ctrl Pts',(-11.9848975174662,110.740622205456,
-1.70099394016176));
#292030=CARTESIAN_POINT('Ctrl Pts',(-11.6540662341939,110.676004008975,
-3.27315832183884));
#292031=CARTESIAN_POINT('Ctrl Pts',(-10.4157421801185,110.54958555311,-6.15687014859585));
#292032=CARTESIAN_POINT('Ctrl Pts',(-9.53582486973339,110.491242982813,
-7.44733605075462));
#292033=CARTESIAN_POINT('Ctrl Pts',(-7.32059686431816,110.366695474867,
-9.63661626355309));
#292034=CARTESIAN_POINT('Ctrl Pts',(-6.00099254844588,110.302763449472,
-10.5092211258972));
#292035=CARTESIAN_POINT('Ctrl Pts',(-3.09828244396946,110.179483361799,
-11.6989576253021));
#292036=CARTESIAN_POINT('Ctrl Pts',(-1.54270457224186,110.118653710383,
-12.0035458220116));
#292037=CARTESIAN_POINT('Ctrl Pts',(1.57484202992488,109.992546301288,-11.9964432460054));
#292038=CARTESIAN_POINT('Ctrl Pts',(3.10713791958133,109.932599558695,-11.6936044440958));
#292039=CARTESIAN_POINT('Ctrl Pts',(6.00290068011063,109.809697043666,-10.5101858809725));
#292040=CARTESIAN_POINT('Ctrl Pts',(7.33368685836178,109.745192702931,-9.6289008134264));
#292041=CARTESIAN_POINT('Ctrl Pts',(9.55771326639455,109.619902138368,-7.42047872440394));
#292042=CARTESIAN_POINT('Ctrl Pts',(10.4370687726621,109.561312846305,-6.12216827482664));
#292043=CARTESIAN_POINT('Ctrl Pts',(11.6535135321669,109.435957947521,-3.25899308580099));
#292044=CARTESIAN_POINT('Ctrl Pts',(11.9776928605359,109.372723534638,-1.72063683666438));
#292045=CARTESIAN_POINT('Ctrl Pts',(12.0204952786623,109.251203487661,1.42419635463371));
#292046=CARTESIAN_POINT('Ctrl Pts',(11.726835375321,109.187405635287,3.00043341259854));
#292047=CARTESIAN_POINT('Ctrl Pts',(10.5582919242157,109.06091014305,5.90882078243624));
#292048=CARTESIAN_POINT('Ctrl Pts',(9.70973094131579,109.002364951962,7.21892400700678));
#292049=CARTESIAN_POINT('Ctrl Pts',(7.54539904661067,108.878198378943,9.46223515898262));
#292050=CARTESIAN_POINT('Ctrl Pts',(6.24346505458509,108.814066835585,10.3675525596455));
#292051=CARTESIAN_POINT('Ctrl Pts',(3.37034905226605,108.690198148285,11.6227774571493));
#292052=CARTESIAN_POINT('Ctrl Pts',(1.82777399968561,108.630185010958,11.962752625575));
#292053=CARTESIAN_POINT('Ctrl Pts',(-1.28540795349743,108.504254155623,
12.0311231925084));
#292054=CARTESIAN_POINT('Ctrl Pts',(-2.82629089884275,108.44348471512,11.7648649134983));
#292055=CARTESIAN_POINT('Ctrl Pts',(-5.75448372048115,108.32112190543,10.6487816912335));
#292056=CARTESIAN_POINT('Ctrl Pts',(-7.1087191713167,108.256546002343,9.79676197411502));
#292057=CARTESIAN_POINT('Ctrl Pts',(-9.38336545307885,108.130807819236,
7.63918600453096));
#292058=CARTESIAN_POINT('Ctrl Pts',(-10.290979608285,108.072442298752,6.36399529241569));
#292059=CARTESIAN_POINT('Ctrl Pts',(-11.5749065627175,107.947350868096,
3.52959487641761));
#292060=CARTESIAN_POINT('Ctrl Pts',(-11.9354229698167,107.883830039254,
1.99560028495009));
#292061=CARTESIAN_POINT('Ctrl Pts',(-11.9973672522598,107.817453322316,
0.290358986012273));
#292062=CARTESIAN_POINT('Ctrl Pts',(-12.0000000000001,107.811833224361,
0.145127975993206));
#292063=CARTESIAN_POINT('Ctrl Pts',(-12.0000000000001,107.80624999958,3.19189119579733E-14));
#292064=CARTESIAN_POINT('Origin',(-8.79029313101884E-14,130.96875,0.));
#292065=CARTESIAN_POINT('',(-12.0000000000001,104.431249999592,-1.27681852051471E-13));
#292066=CARTESIAN_POINT('',(-12.0000000000001,104.806249999592,1.19342770927626E-13));
#292067=CARTESIAN_POINT('',(-12.0000000000001,130.96875,-1.46957615897682E-15));
#292068=CARTESIAN_POINT('Ctrl Pts',(-12.0000000000001,104.431249999592,
-3.8441472227646E-13));
#292069=CARTESIAN_POINT('Ctrl Pts',(-12.0000000000001,104.478870965931,
1.23783919338978));
#292070=CARTESIAN_POINT('Ctrl Pts',(-11.8084687407335,104.528670746041,
2.4700812688676));
#292071=CARTESIAN_POINT('Ctrl Pts',(-10.9524960498144,104.642422247347,
5.14876714220476));
#292072=CARTESIAN_POINT('Ctrl Pts',(-10.1852917659291,104.703348111406,
6.53656683948058));
#292073=CARTESIAN_POINT('Ctrl Pts',(-8.16248778483741,104.826563392885,
8.93466456822427));
#292074=CARTESIAN_POINT('Ctrl Pts',(-6.92757065129571,104.890472222916,
9.92285577526435));
#292075=CARTESIAN_POINT('Ctrl Pts',(-4.16474079504433,105.015057717378,
11.3600243563759));
#292076=CARTESIAN_POINT('Ctrl Pts',(-2.66648802844724,105.073388293074,
11.8019078210812));
#292077=CARTESIAN_POINT('Ctrl Pts',(0.457759258577007,105.199766750565,
12.096279340879));
#292078=CARTESIAN_POINT('Ctrl Pts',(2.05521741175009,105.264385290251,11.9292042769213));
#292079=CARTESIAN_POINT('Ctrl Pts',(5.05658115232668,105.385793003872,10.9929181357832));
#292080=CARTESIAN_POINT('Ctrl Pts',(6.4358250306347,105.448236295316,10.2466597324239));
#292081=CARTESIAN_POINT('Ctrl Pts',(8.83605220345876,105.573844849345,8.26738303399802));
#292082=CARTESIAN_POINT('Ctrl Pts',(9.83329452454308,105.632865363677,7.05207833591719));
#292083=CARTESIAN_POINT('Ctrl Pts',(11.3167954709383,105.757616045139,4.29138073074682));
#292084=CARTESIAN_POINT('Ctrl Pts',(11.7821299805779,105.82200091017,2.76898421521227));
#292085=CARTESIAN_POINT('Ctrl Pts',(12.094500037319,105.945452126676,-0.338459142171763));
#292086=CARTESIAN_POINT('Ctrl Pts',(11.9502904496381,106.004682712918,-1.89262718076547));
#292087=CARTESIAN_POINT('Ctrl Pts',(11.0714914325709,106.130964004916,-4.88959039396011));
#292088=CARTESIAN_POINT('Ctrl Pts',(10.3339629765012,106.192867469903,-6.3003952609892));
#292089=CARTESIAN_POINT('Ctrl Pts',(8.36424401652176,106.315461815542,-8.74544262989015));
#292090=CARTESIAN_POINT('Ctrl Pts',(7.15518653768962,106.379137687194,-9.75942872072018));
#292091=CARTESIAN_POINT('Ctrl Pts',(4.42843243854746,106.504052097933,-11.2600850432998));
#292092=CARTESIAN_POINT('Ctrl Pts',(2.93916954508338,106.562358094017,-11.7371975382882));
#292093=CARTESIAN_POINT('Ctrl Pts',(-0.175434345152722,106.688346467914,
-12.1031707379278));
#292094=CARTESIAN_POINT('Ctrl Pts',(-1.77248965636175,106.7529487123,-11.9739735782117));
#292095=CARTESIAN_POINT('Ctrl Pts',(-4.81797147125956,106.876141039515,
-11.1034148887432));
#292096=CARTESIAN_POINT('Ctrl Pts',(-6.23716913870021,106.938733989896,
-10.3728859618237));
#292097=CARTESIAN_POINT('Ctrl Pts',(-8.68365988620488,107.065104145652,
-8.42525379333561));
#292098=CARTESIAN_POINT('Ctrl Pts',(-9.6959044275387,107.12401750548,-7.23742505899842));
#292099=CARTESIAN_POINT('Ctrl Pts',(-11.2276591634751,107.247758596914,
-4.51864891526425));
#292100=CARTESIAN_POINT('Ctrl Pts',(-11.7230049203476,107.31205641737,-3.00826624484089));
#292101=CARTESIAN_POINT('Ctrl Pts',(-11.9709415925415,107.393768648943,
-0.96483267613689));
#292102=CARTESIAN_POINT('Ctrl Pts',(-12.0000000000001,107.41270083742,-0.482159050745271));
#292103=CARTESIAN_POINT('Ctrl Pts',(-12.0000000000001,107.43124999958,-2.77555756156289E-16));
#292104=CARTESIAN_POINT('Ctrl Pts',(-12.0000000000001,107.80624999958,-3.46944695195361E-14));
#292105=CARTESIAN_POINT('Ctrl Pts',(-12.0000000000001,107.751124737303,
-1.43290267791645));
#292106=CARTESIAN_POINT('Ctrl Pts',(-11.7433421899126,107.693187065922,
-2.85551674708468));
#292107=CARTESIAN_POINT('Ctrl Pts',(-10.6998000168058,107.572695216503,
-5.6484633501225));
#292108=CARTESIAN_POINT('Ctrl Pts',(-9.88373255926775,107.513770095995,
-6.97873356384564));
#292109=CARTESIAN_POINT('Ctrl Pts',(-7.77272003673247,107.390040611035,
-9.27704927235111));
#292110=CARTESIAN_POINT('Ctrl Pts',(-6.4898226139486,107.32573893502,-10.2157237852365));
#292111=CARTESIAN_POINT('Ctrl Pts',(-3.64807500368188,107.201303237798,
-11.5379711509711));
#292112=CARTESIAN_POINT('Ctrl Pts',(-2.11898203155151,107.141964623298,
-11.9139876813583));
#292113=CARTESIAN_POINT('Ctrl Pts',(0.989299535718332,107.016231992737,
-12.0594117922852));
#292114=CARTESIAN_POINT('Ctrl Pts',(2.53880322870443,106.954454867829,-11.8305601284356));
#292115=CARTESIAN_POINT('Ctrl Pts',(5.4990534278353,106.832683293425,-10.7834665636903));
#292116=CARTESIAN_POINT('Ctrl Pts',(6.87645816728897,106.768070055141,-9.96176637459719));
#292117=CARTESIAN_POINT('Ctrl Pts',(9.201821943112,106.641915764979,-7.85649621287418));
#292118=CARTESIAN_POINT('Ctrl Pts',(10.1378238393358,106.583618488968,-6.60474111275065));
#292119=CARTESIAN_POINT('Ctrl Pts',(11.4893568080365,106.458835346254,-3.80032072830849));
#292120=CARTESIAN_POINT('Ctrl Pts',(11.8864585551809,106.395058977097,-2.27157102790158));
#292121=CARTESIAN_POINT('Ctrl Pts',(12.0720896196125,106.27220278525,0.861585505856075));
#292122=CARTESIAN_POINT('Ctrl Pts',(11.8551147849263,106.210723377283,2.43600242799914));
#292123=CARTESIAN_POINT('Ctrl Pts',(10.8346985368866,106.08450475685,5.38532235547232));
#292124=CARTESIAN_POINT('Ctrl Pts',(10.0510979590871,106.025028943484,6.73556216159971));
#292125=CARTESIAN_POINT('Ctrl Pts',(7.99389367644074,105.901777922586,9.08781508319591));
#292126=CARTESIAN_POINT('Ctrl Pts',(6.73071709669543,105.837343197422,10.0592288540481));
#292127=CARTESIAN_POINT('Ctrl Pts',(3.92098548417948,105.712384132381,11.4475545198986));
#292128=CARTESIAN_POINT('Ctrl Pts',(2.40534971244001,105.653548439328,11.8589576328111));
#292129=CARTESIAN_POINT('Ctrl Pts',(-0.697680398376329,105.528028234643,
12.0802124876522));
#292130=CARTESIAN_POINT('Ctrl Pts',(-2.25552011584,105.46509677064,11.8882367252435));
#292131=CARTESIAN_POINT('Ctrl Pts',(-5.24627778918792,105.343945647858,
10.9092283541567));
#292132=CARTESIAN_POINT('Ctrl Pts',(-6.64570423226648,105.2793304235,10.1177549085152));
#292133=CARTESIAN_POINT('Ctrl Pts',(-9.02001057303937,105.152806623237,
8.06430737183463));
#292134=CARTESIAN_POINT('Ctrl Pts',(-9.98350661690994,105.094422794686,
6.83544294611026));
#292135=CARTESIAN_POINT('Ctrl Pts',(-11.4002871497796,104.969979671626,
4.0610611070136));
#292136=CARTESIAN_POINT('Ctrl Pts',(-11.8328494888336,104.905987249946,
2.53821727375672));
#292137=CARTESIAN_POINT('Ctrl Pts',(-11.9867964501751,104.831436008067,
0.650384324452592));
#292138=CARTESIAN_POINT('Ctrl Pts',(-12.0000000000001,104.818753455413,
0.325009525372273));
#292139=CARTESIAN_POINT('Ctrl Pts',(-12.0000000000001,104.806249999592,
4.41244263349461E-13));
#292140=CARTESIAN_POINT('Origin',(-8.79029313101884E-14,130.96875,0.));
#292141=CARTESIAN_POINT('',(-12.0000000000001,101.431249999604,-3.74068423616381E-14));
#292142=CARTESIAN_POINT('',(-12.0000000000001,101.806249999604,8.20462161941248E-14));
#292143=CARTESIAN_POINT('',(-12.0000000000001,130.96875,-1.46957615897682E-15));
#292144=CARTESIAN_POINT('Ctrl Pts',(-12.0000000000001,101.431249999604,
-2.08166817117217E-14));
#292145=CARTESIAN_POINT('Ctrl Pts',(-12.0000000000001,101.486480368325,
1.43563477022792));
#292146=CARTESIAN_POINT('Ctrl Pts',(-11.7423637223291,101.544523597783,
2.86067474786727));
#292147=CARTESIAN_POINT('Ctrl Pts',(-10.6913465639717,101.665674294721,
5.66831838384956));
#292148=CARTESIAN_POINT('Ctrl Pts',(-9.864509629537,101.725078834577,7.00900948680852));
#292149=CARTESIAN_POINT('Ctrl Pts',(-7.7347392825375,101.849454122691,9.30866876971111));
#292150=CARTESIAN_POINT('Ctrl Pts',(-6.44838210482864,101.913738856922,
10.2418687926062));
#292151=CARTESIAN_POINT('Ctrl Pts',(-3.61411194849174,102.037518624373,
11.5468205756838));
#292152=CARTESIAN_POINT('Ctrl Pts',(-2.09777054167503,102.096393398676,
11.9159637947213));
#292153=CARTESIAN_POINT('Ctrl Pts',(1.02655990456309,102.222775220028,12.0601440246069));
#292154=CARTESIAN_POINT('Ctrl Pts',(2.60518842577862,102.285467588493,11.8200466266539));
#292155=CARTESIAN_POINT('Ctrl Pts',(5.55881291589413,102.407598360007,10.7487262681341));
#292156=CARTESIAN_POINT('Ctrl Pts',(6.90806435611422,102.4710890811,9.93548776383274));
#292157=CARTESIAN_POINT('Ctrl Pts',(9.21236286066618,102.596211774256,7.84461115492276));
#292158=CARTESIAN_POINT('Ctrl Pts',(10.1480793037009,102.654594451917,6.58954141103041));
#292159=CARTESIAN_POINT('Ctrl Pts',(11.5042826036013,102.780284760786,3.76305801707942));
#292160=CARTESIAN_POINT('Ctrl Pts',(11.9000354126918,102.844854416412,2.2132496682374));
#292161=CARTESIAN_POINT('Ctrl Pts',(12.0648754059926,102.9672792705,-0.915450283366411));
#292162=CARTESIAN_POINT('Ctrl Pts',(11.8461129143289,103.027949013678,-2.46355219734727));
#292163=CARTESIAN_POINT('Ctrl Pts',(10.8268982536332,103.153900398374,-5.40631613185324));
#292164=CARTESIAN_POINT('Ctrl Pts',(10.0301736577837,103.213996901955,-6.77093711946924));
#292165=CARTESIAN_POINT('Ctrl Pts',(7.95445010979591,103.337801653831,-9.12098954731558));
#292166=CARTESIAN_POINT('Ctrl Pts',(6.69396284264352,103.401912566859,-10.0824857902304));
#292167=CARTESIAN_POINT('Ctrl Pts',(3.89557572687022,103.526123852328,-11.4549753373937));
#292168=CARTESIAN_POINT('Ctrl Pts',(2.3883726505594,103.584638296435,-11.8611803475485));
#292169=CARTESIAN_POINT('Ctrl Pts',(-0.739082770733267,103.711146525683,
-12.0821196279082));
#292170=CARTESIAN_POINT('Ctrl Pts',(-2.33026894912346,103.775086642228,
-11.8782593431249));
#292171=CARTESIAN_POINT('Ctrl Pts',(-5.31082446606679,103.896530727792,
-10.8728873364844));
#292172=CARTESIAN_POINT('Ctrl Pts',(-6.67531879768973,103.959732378726,
-10.0927867264592));
#292173=CARTESIAN_POINT('Ctrl Pts',(-9.02759927654267,104.085113094283,
-8.05709960715809));
#292174=CARTESIAN_POINT('Ctrl Pts',(-9.99393082580769,104.143735651335,
-6.82171458919567));
#292175=CARTESIAN_POINT('Ctrl Pts',(-11.4138370934978,104.268976015867,
-4.02762520637223));
#292176=CARTESIAN_POINT('Ctrl Pts',(-11.8444903102128,104.333470643599,
-2.49110693061898));
#292177=CARTESIAN_POINT('Ctrl Pts',(-11.9883717226644,104.407624235863,
-0.610339821600662));
#292178=CARTESIAN_POINT('Ctrl Pts',(-12.0000000000001,104.419516116535,
-0.305005577473783));
#292179=CARTESIAN_POINT('Ctrl Pts',(-12.0000000000001,104.431249999592,
-4.09186573513409E-13));
#292180=CARTESIAN_POINT('Ctrl Pts',(-12.0000000000001,104.806249999592,
4.56856774633252E-13));
#292181=CARTESIAN_POINT('Ctrl Pts',(-12.0000000000001,104.758601490836,
-1.23855511927143));
#292182=CARTESIAN_POINT('Ctrl Pts',(-11.8082468123864,104.708767224827,
-2.47162149771696));
#292183=CARTESIAN_POINT('Ctrl Pts',(-10.9583504590709,104.595896362933,
-5.12939072557227));
#292184=CARTESIAN_POINT('Ctrl Pts',(-10.2060230595981,104.535730732699,
-6.49869718555533));
#292185=CARTESIAN_POINT('Ctrl Pts',(-8.20109956593658,104.412978757805,
-8.90191931904317));
#292186=CARTESIAN_POINT('Ctrl Pts',(-6.95754137383397,104.348450357766,
-9.90427530766931));
#292187=CARTESIAN_POINT('Ctrl Pts',(-4.17924700902458,104.223027513568,
-11.3553764834465));
#292188=CARTESIAN_POINT('Ctrl Pts',(-2.67654250396623,104.164518418188,
-11.8002868100017));
#292189=CARTESIAN_POINT('Ctrl Pts',(0.420634824484783,104.039234963523,
-12.0934553377146));
#292190=CARTESIAN_POINT('Ctrl Pts',(1.98599508233998,103.975914810977,-11.9366957236708));
#292191=CARTESIAN_POINT('Ctrl Pts',(4.99510223067139,103.854193869933,-11.0255561725828));
#292192=CARTESIAN_POINT('Ctrl Pts',(6.40669019810106,103.790767354196,-10.2698003364113));
#292193=CARTESIAN_POINT('Ctrl Pts',(8.8239865738571,103.664307010339,-8.27819238721138));
#292194=CARTESIAN_POINT('Ctrl Pts',(9.81620057244571,103.605669864452,-7.07343347616651));
#292195=CARTESIAN_POINT('Ctrl Pts',(11.3008354362689,103.481625073801,-4.33145292931322));
#292196=CARTESIAN_POINT('Ctrl Pts',(11.7704103186201,103.4174406109,-2.81564336233957));
#292197=CARTESIAN_POINT('Ctrl Pts',(12.097616008431,103.293403808774,0.30220106981476));
#292198=CARTESIAN_POINT('Ctrl Pts',(11.9554270961315,103.233603145005,1.87386889975548));
#292199=CARTESIAN_POINT('Ctrl Pts',(11.0801151872735,103.10772795905,4.86140899493031));
#292200=CARTESIAN_POINT('Ctrl Pts',(10.3602688336532,103.046683455066,6.25034332769341));
#292201=CARTESIAN_POINT('Ctrl Pts',(8.41005808803819,102.924488069061,8.70546181073995));
#292202=CARTESIAN_POINT('Ctrl Pts',(7.18748045059645,102.859897634335,9.7393041406602));
#292203=CARTESIAN_POINT('Ctrl Pts',(4.44241821737085,102.734034473329,11.2546644811422));
#292204=CARTESIAN_POINT('Ctrl Pts',(2.95309570322389,102.675705230097,11.733787715922));
#292205=CARTESIAN_POINT('Ctrl Pts',(-0.137221574066131,102.55069927033,
12.1004522758571));
#292206=CARTESIAN_POINT('Ctrl Pts',(-1.70946979472838,102.487100493836,
11.9798876915772));
#292207=CARTESIAN_POINT('Ctrl Pts',(-4.73533018511225,102.364701869915,
11.1386076462919));
#292208=CARTESIAN_POINT('Ctrl Pts',(-6.15800372262147,102.302471030129,
10.4197516925769));
#292209=CARTESIAN_POINT('Ctrl Pts',(-8.61792563958917,102.176145716897,
8.49249195173133));
#292210=CARTESIAN_POINT('Ctrl Pts',(-9.63941404855684,102.1170771611,7.31250848129084));
#292211=CARTESIAN_POINT('Ctrl Pts',(-11.1928508050391,101.993483328734,
4.60460504283106));
#292212=CARTESIAN_POINT('Ctrl Pts',(-11.7000709570479,101.929138946295,
3.09687028481685));
#292213=CARTESIAN_POINT('Ctrl Pts',(-11.9672392841743,101.846070331329,
1.02442820521571));
#292214=CARTESIAN_POINT('Ctrl Pts',(-12.0000000000001,101.825945438085,
0.511954871078143));
#292215=CARTESIAN_POINT('Ctrl Pts',(-12.0000000000001,101.806249999604,
3.75394160201381E-13));
#292216=CARTESIAN_POINT('Origin',(-8.79029313101884E-14,130.96875,0.));
#292217=CARTESIAN_POINT('',(-12.0000000000001,98.431249999616,-7.39612622723935E-15));
#292218=CARTESIAN_POINT('',(-12.0000000000001,98.806249999616,-1.70623322603542E-15));
#292219=CARTESIAN_POINT('',(-12.0000000000001,130.96875,-1.46957615897682E-15));
#292220=CARTESIAN_POINT('Ctrl Pts',(-12.0000000000001,98.431249999616,2.73285667600019E-15));
#292221=CARTESIAN_POINT('Ctrl Pts',(-12.0000000000001,98.4339838995247,
0.0710638342315633));
#292222=CARTESIAN_POINT('Ctrl Pts',(-11.999368742607,98.4367267560416,0.142155374774367));
#292223=CARTESIAN_POINT('Ctrl Pts',(-11.970413553221,98.499757391063,1.77113884620319));
#292224=CARTESIAN_POINT('Ctrl Pts',(-11.6395687683053,98.5630467688966,
3.30875809283163));
#292225=CARTESIAN_POINT('Ctrl Pts',(-10.4107184215545,98.6883565337207,
6.16672926919503));
#292226=CARTESIAN_POINT('Ctrl Pts',(-9.52617270723465,98.746893233943,7.4608093385413));
#292227=CARTESIAN_POINT('Ctrl Pts',(-7.29284135606745,98.872268443788,9.6599843247105));
#292228=CARTESIAN_POINT('Ctrl Pts',(-5.95772174749821,98.9367884426156,
10.5359634928269));
#292229=CARTESIAN_POINT('Ctrl Pts',(-3.05596584100162,99.0595954362412,
11.7071157123083));
#292230=CARTESIAN_POINT('Ctrl Pts',(-1.52209266533542,99.1196800579496,
12.0032840633594));
#292231=CARTESIAN_POINT('Ctrl Pts',(1.59469019289135,99.2457565729532,11.9966155425732));
#292232=CARTESIAN_POINT('Ctrl Pts',(3.14791120094077,99.3064259324189,11.6855641658905));
#292233=CARTESIAN_POINT('Ctrl Pts',(6.04530459772022,99.4298158168412,10.4838919607646));
#292234=CARTESIAN_POINT('Ctrl Pts',(7.36175649343294,99.4937866150215,9.60531743954377));
#292235=CARTESIAN_POINT('Ctrl Pts',(9.56779607296812,99.6182680624296,7.40616884991388));
#292236=CARTESIAN_POINT('Ctrl Pts',(10.4420261374425,99.676635375023,6.11212812404449));
#292237=CARTESIAN_POINT('Ctrl Pts',(11.6682109103662,99.803121251764,3.22271949610166));
#292238=CARTESIAN_POINT('Ctrl Pts',(11.9923361918725,99.8677379023339,1.64841638612066));
#292239=CARTESIAN_POINT('Ctrl Pts',(12.0072192913573,99.9889576944574,-1.49768364446297));
#292240=CARTESIAN_POINT('Ctrl Pts',(11.7124578522839,100.051757106291,-3.03898249246358));
#292241=CARTESIAN_POINT('Ctrl Pts',(10.5507336771395,100.177301021367,-5.92485068641402));
#292242=CARTESIAN_POINT('Ctrl Pts',(9.69428116035566,100.236183130822,-7.24174002038604));
#292243=CARTESIAN_POINT('Ctrl Pts',(7.5113436058091,100.361087484542,-9.49047261996084));
#292244=CARTESIAN_POINT('Ctrl Pts',(6.19980993931202,100.425509546752,-10.3947959861688));
#292245=CARTESIAN_POINT('Ctrl Pts',(3.33067993774254,100.548814456576,-11.6317955142732));
#292246=CARTESIAN_POINT('Ctrl Pts',(1.80534352002713,100.608222320188,-11.9638139311181));
#292247=CARTESIAN_POINT('Ctrl Pts',(-1.31537176120697,100.734457905044,
-12.0312005576569));
#292248=CARTESIAN_POINT('Ctrl Pts',(-2.88118079495719,100.796047579945,
-11.7549390802658));
#292249=CARTESIAN_POINT('Ctrl Pts',(-5.80673038534638,100.918834693939,
-10.6173721643633));
#292250=CARTESIAN_POINT('Ctrl Pts',(-7.13975940039004,100.982584856503,
-9.77089369112507));
#292251=CARTESIAN_POINT('Ctrl Pts',(-9.39469398919182,101.107403640946,
-7.62485542228049));
#292252=CARTESIAN_POINT('Ctrl Pts',(-10.2993311285907,101.165700631305,
-6.34999679352737));
#292253=CARTESIAN_POINT('Ctrl Pts',(-11.5901541926833,101.291811339783,
-3.49134238417836));
#292254=CARTESIAN_POINT('Ctrl Pts',(-11.9499467466854,101.356422234309,
-1.92877789368869));
#292255=CARTESIAN_POINT('Ctrl Pts',(-11.9983815360636,101.422472161457,
-0.227641529534562));
#292256=CARTESIAN_POINT('Ctrl Pts',(-12.0000000000001,101.42687244655,-0.113788256692766));
#292257=CARTESIAN_POINT('Ctrl Pts',(-12.0000000000001,101.431249999604,
1.59594559789866E-14));
#292258=CARTESIAN_POINT('Ctrl Pts',(-12.0000000000001,101.806249999604,
4.54081217071689E-13));
#292259=CARTESIAN_POINT('Ctrl Pts',(-12.0000000000001,101.766230467423,
-1.04025073916514));
#292260=CARTESIAN_POINT('Ctrl Pts',(-11.8647387182924,101.724607547189,
-2.07823021252408));
#292261=CARTESIAN_POINT('Ctrl Pts',(-11.1964684722288,101.619699777096,
-4.58802411045548));
#292262=CARTESIAN_POINT('Ctrl Pts',(-10.5095366854714,101.557599891377,
-5.99666408431447));
#292263=CARTESIAN_POINT('Ctrl Pts',(-8.6151392416733,101.436006797544,-8.50327148822433));
#292264=CARTESIAN_POINT('Ctrl Pts',(-7.41440413156253,101.371389422096,
-9.56831056394794));
#292265=CARTESIAN_POINT('Ctrl Pts',(-4.70357623074547,101.245122398749,
-11.1477762603995));
#292266=CARTESIAN_POINT('Ctrl Pts',(-3.22775165344605,101.186815296669,
-11.6609686402055));
#292267=CARTESIAN_POINT('Ctrl Pts',(-0.145323019961658,101.062128439248,
-12.1008215457449));
#292268=CARTESIAN_POINT('Ctrl Pts',(1.43297481961014,100.998284950528,-12.0165610469654));
#292269=CARTESIAN_POINT('Ctrl Pts',(4.47459070255941,100.875249003546,-11.2450105826866));
#292270=CARTESIAN_POINT('Ctrl Pts',(5.90794163155401,100.814050914446,-10.562603188016));
#292271=CARTESIAN_POINT('Ctrl Pts',(8.40949900348915,100.687877932815,-8.69905657155727));
#292272=CARTESIAN_POINT('Ctrl Pts',(9.45975726268865,100.628213979255,-7.54362017860402));
#292273=CARTESIAN_POINT('Ctrl Pts',(11.0803977678472,100.505106926566,-4.87020570611372));
#292274=CARTESIAN_POINT('Ctrl Pts',(11.6244761419959,100.440640950313,-3.371286252466));
#292275=CARTESIAN_POINT('Ctrl Pts',(12.0972265307051,100.315540412315,-0.273081860755084));
#292276=CARTESIAN_POINT('Ctrl Pts',(12.030816350728,100.256817412875,1.29494252459816));
#292277=CARTESIAN_POINT('Ctrl Pts',(11.3032575658423,100.131368363954,4.31941369468196));
#292278=CARTESIAN_POINT('Ctrl Pts',(10.6485546742428,100.068258588068,5.7471365668539));
#292279=CARTESIAN_POINT('Ctrl Pts',(8.81030383113319,99.947025338931,8.30113829994723));
#292280=CARTESIAN_POINT('Ctrl Pts',(7.63347054879219,99.8826852300756,9.39474500493053));
#292281=CARTESIAN_POINT('Ctrl Pts',(4.95929109759016,99.7561432023647,11.0362192328815));
#292282=CARTESIAN_POINT('Ctrl Pts',(3.49690740949452,99.6977028757142,11.5829351373832));
#292283=CARTESIAN_POINT('Ctrl Pts',(0.423259818640735,99.5733712189287,
12.0947502380544));
#292284=CARTESIAN_POINT('Ctrl Pts',(-1.16019061442988,99.5093193034237,
12.046417704419));
#292285=CARTESIAN_POINT('Ctrl Pts',(-4.21639957800431,99.3856930539296,
11.3435862127409));
#292286=CARTESIAN_POINT('Ctrl Pts',(-5.65992487123753,99.3253566684579,
10.696740333296));
#292287=CARTESIAN_POINT('Ctrl Pts',(-8.20168150789831,99.1993497667033,
8.89550832667992));
#292288=CARTESIAN_POINT('Ctrl Pts',(-9.27988138373904,99.1389446082995,
7.76410238086659));
#292289=CARTESIAN_POINT('Ctrl Pts',(-10.9653551504483,99.0163510890256,
5.12510208173164));
#292290=CARTESIAN_POINT('Ctrl Pts',(-11.5450497092688,98.951800902559,3.63556610340489));
#292291=CARTESIAN_POINT('Ctrl Pts',(-11.9397038585928,98.8604536395862,
1.38935501476442));
#292292=CARTESIAN_POINT('Ctrl Pts',(-12.0000000000001,98.8329699508869,
0.694547076025101));
#292293=CARTESIAN_POINT('Ctrl Pts',(-12.0000000000001,98.806249999616,1.94289029309402E-15));
#292294=CARTESIAN_POINT('Origin',(-8.79029313101884E-14,130.96875,0.));
#292295=CARTESIAN_POINT('',(-12.0000000000001,95.431249999628,6.27560911412627E-14));
#292296=CARTESIAN_POINT('',(-12.0000000000001,95.806249999628,-2.51596946212419E-14));
#292297=CARTESIAN_POINT('',(-12.0000000000001,130.96875,-1.46957615897682E-15));
#292298=CARTESIAN_POINT('Ctrl Pts',(-12.0000000000001,95.431249999628,-8.60422844084496E-15));
#292299=CARTESIAN_POINT('Ctrl Pts',(-12.0000000000001,95.4409906235063,
0.253193644134754));
#292300=CARTESIAN_POINT('Ctrl Pts',(-11.9919867672329,95.4508413495118,
0.506645579091207));
#292301=CARTESIAN_POINT('Ctrl Pts',(-11.8767809487482,95.5221231903685,
2.32208286579897));
#292302=CARTESIAN_POINT('Ctrl Pts',(-11.4729702276523,95.5859428304934,
3.84977745561648));
#292303=CARTESIAN_POINT('Ctrl Pts',(-10.1090728697394,95.7106647582825,
6.6485892116695));
#292304=CARTESIAN_POINT('Ctrl Pts',(-9.16786888107841,95.7689668056092,
7.89602750012452));
#292305=CARTESIAN_POINT('Ctrl Pts',(-6.83322973383029,95.8951935824947,
9.99157989034653));
#292306=CARTESIAN_POINT('Ctrl Pts',(-5.45162528538409,95.9598098091461,
10.8076253621462));
#292307=CARTESIAN_POINT('Ctrl Pts',(-2.48556070131359,96.0814676265569,
11.8419316653302));
#292308=CARTESIAN_POINT('Ctrl Pts',(-0.934478472913705,96.1434495513518,
12.063855455804));
#292309=CARTESIAN_POINT('Ctrl Pts',(2.17284804789866,96.2691435494718,11.9041750318455));
#292310=CARTESIAN_POINT('Ctrl Pts',(3.6994249245477,96.3283753205453,11.5214995860526));
#292311=CARTESIAN_POINT('Ctrl Pts',(6.53524039790862,96.4529120720883,10.1868371422895));
#292312=CARTESIAN_POINT('Ctrl Pts',(7.81450496390696,96.5172414001135,9.24199942925195));
#292313=CARTESIAN_POINT('Ctrl Pts',(9.91550239210979,96.640884615364,6.93352749959648));
#292314=CARTESIAN_POINT('Ctrl Pts',(10.7255035305225,96.6998997042907,5.59951240890465));
#292315=CARTESIAN_POINT('Ctrl Pts',(11.8060931249998,96.8262401279026,2.66657788672909));
#292316=CARTESIAN_POINT('Ctrl Pts',(12.0541788218455,96.8885895765476,1.09129317018687));
#292317=CARTESIAN_POINT('Ctrl Pts',(11.9267881891096,97.0109185137701,-2.0470815939593));
#292318=CARTESIAN_POINT('Ctrl Pts',(11.5594557310219,97.0744894536273,-3.58016408067849));
#292319=CARTESIAN_POINT('Ctrl Pts',(10.2629091491639,97.1995267154807,-6.40905609030048));
#292320=CARTESIAN_POINT('Ctrl Pts',(9.35000251967587,97.2578675135338,-7.67989349432511));
#292321=CARTESIAN_POINT('Ctrl Pts',(7.06588919238247,97.3836858653614,-9.82781096885908));
#292322=CARTESIAN_POINT('Ctrl Pts',(5.70730328442144,97.448271393592,-10.6742476144214));
#292323=CARTESIAN_POINT('Ctrl Pts',(2.77309298937273,97.5705277384726,-11.7775707460928));
#292324=CARTESIAN_POINT('Ctrl Pts',(1.23060221857106,97.6314710942121,-12.036905859078));
#292325=CARTESIAN_POINT('Ctrl Pts',(-1.88170570409498,97.7573665942699,
-11.9542646404877));
#292326=CARTESIAN_POINT('Ctrl Pts',(-3.42179911890718,97.8172425508346,
-11.6076079183399));
#292327=CARTESIAN_POINT('Ctrl Pts',(-6.28919379484739,97.9412188725106,
-10.3399813514453));
#292328=CARTESIAN_POINT('Ctrl Pts',(-7.58767823178803,98.0053845234396,
-9.42848153263456));
#292329=CARTESIAN_POINT('Ctrl Pts',(-9.74223853888837,98.1294738432075,
-7.17497009917505));
#292330=CARTESIAN_POINT('Ctrl Pts',(-10.5848186442503,98.1880760149103,
-5.86114108318552));
#292331=CARTESIAN_POINT('Ctrl Pts',(-11.7134943203517,98.3116777809989,
-3.01501817768779));
#292332=CARTESIAN_POINT('Ctrl Pts',(-12.0000000000001,98.3730074168523,
-1.5139329839569));
#292333=CARTESIAN_POINT('Ctrl Pts',(-12.0000000000001,98.431249999616,-3.80251385934116E-14));
#292334=CARTESIAN_POINT('Ctrl Pts',(-12.0000000000001,98.806249999616,-7.21644966006352E-15));
#292335=CARTESIAN_POINT('Ctrl Pts',(-12.0000000000001,98.7735434882751,
-0.850159178381908));
#292336=CARTESIAN_POINT('Ctrl Pts',(-11.909658234483,98.7397261048303,-1.69984007587557));
#292337=CARTESIAN_POINT('Ctrl Pts',(-11.3998801877238,98.6425987099933,
-4.05889143789282));
#292338=CARTESIAN_POINT('Ctrl Pts',(-10.776497725326,98.5791933670716,-5.50447377851174));
#292339=CARTESIAN_POINT('Ctrl Pts',(-8.99802596747649,98.457269553505,-8.09584915261635));
#292340=CARTESIAN_POINT('Ctrl Pts',(-7.85236943941162,98.3942105106125,
-9.21129759630602));
#292341=CARTESIAN_POINT('Ctrl Pts',(-5.22536157044818,98.2677878683712,
-10.9126767647559));
#292342=CARTESIAN_POINT('Ctrl Pts',(-3.77721877718979,98.2090417087292,
-11.4945021231782));
#292343=CARTESIAN_POINT('Ctrl Pts',(-0.713835593063138,98.0851252559177,
-12.0815691625026));
#292344=CARTESIAN_POINT('Ctrl Pts',(0.87415130039543,98.0208898367353,-12.0710295258403));
#292345=CARTESIAN_POINT('Ctrl Pts',(3.94467066967295,97.8966847191707,-11.4402247482499));
#292346=CARTESIAN_POINT('Ctrl Pts',(5.39851955746572,97.8370865391971,-10.8302874243549));
#292347=CARTESIAN_POINT('Ctrl Pts',(7.98157939540233,97.7112696433552,-9.09389575881817));
#292348=CARTESIAN_POINT('Ctrl Pts',(9.08865504458853,97.6499302204276,-7.98752451712976));
#292349=CARTESIAN_POINT('Ctrl Pts',(10.8406367502923,97.5279089383564,-5.38500844837757));
#292350=CARTESIAN_POINT('Ctrl Pts',(11.4569020000997,97.46330681163,-3.90600489478107));
#292351=CARTESIAN_POINT('Ctrl Pts',(12.071059380927,97.3373198579925,-0.830705307969824));
#292352=CARTESIAN_POINT('Ctrl Pts',(12.0773796214608,97.2790136755807,0.73311161381929));
#292353=CARTESIAN_POINT('Ctrl Pts',(11.4925352314639,97.1540981915476,3.79008424243644));
#292354=CARTESIAN_POINT('Ctrl Pts',(10.9016839261066,97.0904231884907,5.25324602785943));
#292355=CARTESIAN_POINT('Ctrl Pts',(9.18477025462278,96.9678310714679,7.88199443316276));
#292356=CARTESIAN_POINT('Ctrl Pts',(8.07081539852554,96.9059239276573,9.01931404370743));
#292357=CARTESIAN_POINT('Ctrl Pts',(5.49193281263632,96.7796421210471,10.7810086478598));
#292358=CARTESIAN_POINT('Ctrl Pts',(4.0583444278431,96.7204134801818,11.3983034025011));
#292359=CARTESIAN_POINT('Ctrl Pts',(1.0064215525226,96.5969606065995,12.0612161585608));
#292360=CARTESIAN_POINT('Ctrl Pts',(-0.585248825613923,96.532576187332,
12.0889723081148));
#292361=CARTESIAN_POINT('Ctrl Pts',(-3.66921114597413,96.4078272909733,
11.5309332747356));
#292362=CARTESIAN_POINT('Ctrl Pts',(-5.13316546952277,96.3488051013711,
10.9579238728703));
#292363=CARTESIAN_POINT('Ctrl Pts',(-7.75714219069866,96.2231958129574,
9.28658112039682));
#292364=CARTESIAN_POINT('Ctrl Pts',(-8.89298840814305,96.1607565336721,
8.20536316575725));
#292365=CARTESIAN_POINT('Ctrl Pts',(-10.7107000481564,96.0393466788323,
5.64009722731743));
#292366=CARTESIAN_POINT('Ctrl Pts',(-11.3631176146055,95.9747281350808,
4.17241353627881));
#292367=CARTESIAN_POINT('Ctrl Pts',(-11.9033212497446,95.8750998425117,
1.75824077268344));
#292368=CARTESIAN_POINT('Ctrl Pts',(-12.0000000000001,95.8400841254468,
0.87946991067202));
#292369=CARTESIAN_POINT('Ctrl Pts',(-12.0000000000001,95.806249999628,1.83186799063151E-14));
#292370=CARTESIAN_POINT('Origin',(-8.79029313101884E-14,130.96875,0.));
#292371=CARTESIAN_POINT('',(-12.0000000000001,92.43124999964,6.31640258511681E-16));
#292372=CARTESIAN_POINT('',(-12.0000000000001,92.80624999964,-6.20746101900283E-14));
#292373=CARTESIAN_POINT('',(-12.0000000000001,130.96875,-1.46957615897682E-15));
#292374=CARTESIAN_POINT('Ctrl Pts',(-12.0000000000001,92.43124999964,-1.42941214420489E-14));
#292375=CARTESIAN_POINT('Ctrl Pts',(-12.0000000000001,92.4479877578223,
0.435074184339853));
#292376=CARTESIAN_POINT('Ctrl Pts',(-11.9763397243295,92.4650400989585,
0.870637814920657));
#292377=CARTESIAN_POINT('Ctrl Pts',(-11.7578816109529,92.5446073612302,
2.86789412608426));
#292378=CARTESIAN_POINT('Ctrl Pts',(-11.2813220363684,92.60882420549,4.38227593627422));
#292379=CARTESIAN_POINT('Ctrl Pts',(-9.7839069954388,92.7327888285159,7.11802010863116));
#292380=CARTESIAN_POINT('Ctrl Pts',(-8.78626776826647,92.7914926820686,
8.31820295371068));
#292381=CARTESIAN_POINT('Ctrl Pts',(-6.36105190107423,92.9179295500625,
10.2979232987543));
#292382=CARTESIAN_POINT('Ctrl Pts',(-4.94739221745984,92.9811237805496,
11.0468557946528));
#292383=CARTESIAN_POINT('Ctrl Pts',(-1.93512718985598,93.1029724604937,
11.9451331339142));
#292384=CARTESIAN_POINT('Ctrl Pts',(-0.368436712215726,93.1663464215603,
12.095243007058));
#292385=CARTESIAN_POINT('Ctrl Pts',(2.72755667704737,93.2915819848791,11.7885297563894));
#292386=CARTESIAN_POINT('Ctrl Pts',(4.2278077709974,93.3500461678424,11.3373130914935));
#292387=CARTESIAN_POINT('Ctrl Pts',(7.00006279564588,93.4755527368303,9.87437813894915));
#292388=CARTESIAN_POINT('Ctrl Pts',(8.2398257586959,93.5400951580834,8.86620875460888));
#292389=CARTESIAN_POINT('Ctrl Pts',(10.2347651696407,93.6627481361002,6.4534083692514));
#292390=CARTESIAN_POINT('Ctrl Pts',(10.9811476841064,93.7230623550284,5.08049611460835));
#292391=CARTESIAN_POINT('Ctrl Pts',(11.9168157767857,93.8490887220024,2.10863719708276));
#292392=CARTESIAN_POINT('Ctrl Pts',(12.0900709513035,93.9095144585482,0.535718606429136));
#292393=CARTESIAN_POINT('Ctrl Pts',(11.8219379208979,94.0330760816248,-2.58896809368176));
#292394=CARTESIAN_POINT('Ctrl Pts',(11.3826137977506,94.0971061475619,-4.11059339897155));
#292395=CARTESIAN_POINT('Ctrl Pts',(9.95341939221315,94.2214798181759,-6.87913640890142));
#292396=CARTESIAN_POINT('Ctrl Pts',(8.98467968699075,94.2798974166537,-8.10361418915103));
#292397=CARTESIAN_POINT('Ctrl Pts',(6.60175557235523,94.4064510604421,-10.1464555512627));
#292398=CARTESIAN_POINT('Ctrl Pts',(5.19922467694068,94.4709369435709,-10.9316516553147));
#292399=CARTESIAN_POINT('Ctrl Pts',(2.20405011418617,94.5920942996898,-11.8979958893954));
#292400=CARTESIAN_POINT('Ctrl Pts',(0.644716337823207,94.6551706759385,
-12.083217628931));
#292401=CARTESIAN_POINT('Ctrl Pts',(-2.45713397727001,94.7806431568839,
-11.8482499914944));
#292402=CARTESIAN_POINT('Ctrl Pts',(-3.97031478326955,94.8394051439292,
-11.4304497851616));
#292403=CARTESIAN_POINT('Ctrl Pts',(-6.77412900177955,94.964455180782,-10.0301533882426));
#292404=CARTESIAN_POINT('Ctrl Pts',(-8.03363115892578,95.028910254409,-9.05282638295034));
#292405=CARTESIAN_POINT('Ctrl Pts',(-10.0809540083812,95.1520694815291,
-6.6908335429643));
#292406=CARTESIAN_POINT('Ctrl Pts',(-10.8586243610838,95.2116641683148,
-5.33696550272215));
#292407=CARTESIAN_POINT('Ctrl Pts',(-11.7836034241284,95.3275863308543,
-2.6242779117785));
#292408=CARTESIAN_POINT('Ctrl Pts',(-12.0000000000001,95.3806324966463,
-1.31572989543491));
#292409=CARTESIAN_POINT('Ctrl Pts',(-12.0000000000001,95.431249999628,1.11022302462516E-15));
#292410=CARTESIAN_POINT('Ctrl Pts',(-12.0000000000001,95.806249999628,-3.30291349825984E-14));
#292411=CARTESIAN_POINT('Ctrl Pts',(-12.0000000000001,95.780812263331,-0.661217724041314));
#292412=CARTESIAN_POINT('Ctrl Pts',(-11.9453518514414,95.7546782580322,
-1.3227777092535));
#292413=CARTESIAN_POINT('Ctrl Pts',(-11.5776573376204,95.6654340297677,
-3.52308312258341));
#292414=CARTESIAN_POINT('Ctrl Pts',(-11.019331674726,95.601525930069,-5.00287214507789));
#292415=CARTESIAN_POINT('Ctrl Pts',(-9.36347959868558,95.4783126788969,
-7.66760616295407));
#292416=CARTESIAN_POINT('Ctrl Pts',(-8.28057849027473,95.4173837817315,
-8.82604402484954));
#292417=CARTESIAN_POINT('Ctrl Pts',(-5.74899845438352,95.2912579992088,
-10.6462828662507));
#292418=CARTESIAN_POINT('Ctrl Pts',(-4.32974559250291,95.2313918879129,
-11.2981215440558));
#292419=CARTESIAN_POINT('Ctrl Pts',(-1.29001781704521,95.1084323164824,
-12.0346740357956));
#292420=CARTESIAN_POINT('Ctrl Pts',(0.30436940379332,95.0439379986191,-12.0997835588058));
#292421=CARTESIAN_POINT('Ctrl Pts',(3.40044253566307,94.9186992096441,-11.6125564471109));
#292422=CARTESIAN_POINT('Ctrl Pts',(4.87394485420319,94.8600755841093,-11.075156778205));
#292423=CARTESIAN_POINT('Ctrl Pts',(7.53676439822538,94.7346940694898,-9.46685640644819));
#292424=CARTESIAN_POINT('Ctrl Pts',(8.70024479373768,94.6714934487501,-8.41012717739552));
#292425=CARTESIAN_POINT('Ctrl Pts',(10.5772679268381,94.5500517449144,-5.88597332086489));
#292426=CARTESIAN_POINT('Ctrl Pts',(11.2627500519815,94.4861071516647,-4.43558346711482));
#292427=CARTESIAN_POINT('Ctrl Pts',(12.0188163963501,94.3595985278966,-1.39283282560082));
#292428=CARTESIAN_POINT('Ctrl Pts',(12.0981145963205,94.3010850127693,0.16613584188054));
#292429=CARTESIAN_POINT('Ctrl Pts',(11.6572931019273,94.1768723370203,3.25163584565223));
#292430=CARTESIAN_POINT('Ctrl Pts',(11.1322499388105,94.1127620762655,4.74749389657754));
#292431=CARTESIAN_POINT('Ctrl Pts',(9.53843214039509,93.9889593322919,7.44770709885618));
#292432=CARTESIAN_POINT('Ctrl Pts',(8.48669257446584,93.928860188331,8.62705540376232));
#292433=CARTESIAN_POINT('Ctrl Pts',(6.00274500242889,93.8029081645055,10.5055466789873));
#292434=CARTESIAN_POINT('Ctrl Pts',(4.59796298894832,93.7422415095144,11.1918712782594));
#292435=CARTESIAN_POINT('Ctrl Pts',(1.57140633397644,93.6198147210993,12.0016647936709));
#292436=CARTESIAN_POINT('Ctrl Pts',(-0.0248383326823098,93.5552452679742,
12.1040681564932));
#292437=CARTESIAN_POINT('Ctrl Pts',(-3.13203640672852,93.4295564656351,
11.687426784496));
#292438=CARTESIAN_POINT('Ctrl Pts',(-4.61479899631361,93.371173219743,11.1852228902824));
#292439=CARTESIAN_POINT('Ctrl Pts',(-7.31527872105174,93.2460495556566,
9.63960211418373));
#292440=CARTESIAN_POINT('Ctrl Pts',(-8.5055637399146,93.1825597841818,8.60760504109358));
#292441=CARTESIAN_POINT('Ctrl Pts',(-10.4369820617429,93.0604313361305,
6.12943631487414));
#292442=CARTESIAN_POINT('Ctrl Pts',(-11.1530457820141,92.9977348986901,
4.70218511139591));
#292443=CARTESIAN_POINT('Ctrl Pts',(-11.8565225469263,92.8903720861421,
2.14001517296361));
#292444=CARTESIAN_POINT('Ctrl Pts',(-12.0000000000001,92.8474669725009,
1.07137650413103));
#292445=CARTESIAN_POINT('Ctrl Pts',(-12.0000000000001,92.80624999964,-2.63677968348475E-14));
#292446=CARTESIAN_POINT('Origin',(-8.79029313101884E-14,130.96875,0.));
#292447=CARTESIAN_POINT('',(-12.,56.4312499997839,-1.48567922702232E-13));
#292448=CARTESIAN_POINT('',(-12.,56.806249999784,-3.42843401048799E-14));
#292449=CARTESIAN_POINT('',(-12.0000000000001,130.96875,-1.46957615897682E-15));
#292450=CARTESIAN_POINT('',(9.41568944744514,58.25,-7.43940805637581));
#292451=CARTESIAN_POINT('Ctrl Pts',(-12.,56.4312499997839,-2.08444372873373E-13));
#292452=CARTESIAN_POINT('Ctrl Pts',(-12.0000000000001,56.4796005831921,
1.25680454989647));
#292453=CARTESIAN_POINT('Ctrl Pts',(-11.8025538465919,56.5301936043954,
2.5077439321711));
#292454=CARTESIAN_POINT('Ctrl Pts',(-10.9351216314112,56.643788730521,5.17864163026471));
#292455=CARTESIAN_POINT('Ctrl Pts',(-10.1767968959666,56.7038100819498,
6.54430442895148));
#292456=CARTESIAN_POINT('Ctrl Pts',(-8.16181553223068,56.8266606028225,
8.93782778686641));
#292457=CARTESIAN_POINT('Ctrl Pts',(-6.91444955693021,56.8911736378425,
9.93429658204381));
#292458=CARTESIAN_POINT('Ctrl Pts',(-4.13008267255682,57.0165105871442,
11.3734270421349));
#292459=CARTESIAN_POINT('Ctrl Pts',(-2.62490142548079,57.0750705066934,
11.8119550341771));
#292460=CARTESIAN_POINT('Ctrl Pts',(0.47343692183443,57.200400925558,12.0914175547538));
#292461=CARTESIAN_POINT('Ctrl Pts',(2.03742327080079,57.2636655023219,11.9279388370427));
#292462=CARTESIAN_POINT('Ctrl Pts',(5.04330248025586,57.3852558704958,11.0037895935951));
#292463=CARTESIAN_POINT('Ctrl Pts',(6.45278041867523,57.4489229198579,10.2411184393772));
#292464=CARTESIAN_POINT('Ctrl Pts',(8.86203277851051,57.5754063519648,8.2374677951918));
#292465=CARTESIAN_POINT('Ctrl Pts',(9.8487426438822,57.6339819585794,7.02807344505916));
#292466=CARTESIAN_POINT('Ctrl Pts',(11.3203984451319,57.758106490958,4.27980297250595));
#292467=CARTESIAN_POINT('Ctrl Pts',(11.7828840712243,57.8222568315178,2.76257692820836));
#292468=CARTESIAN_POINT('Ctrl Pts',(12.093882992487,57.9452495710872,-0.333394483159807));
#292469=CARTESIAN_POINT('Ctrl Pts',(11.9512678995239,58.0042455402168,-1.88158108678264));
#292470=CARTESIAN_POINT('Ctrl Pts',(11.0874436001478,58.1289659147518,-4.84283605448112));
#292471=CARTESIAN_POINT('Ctrl Pts',(10.3729381859985,58.1898675005961,-6.22786585061494));
#292472=CARTESIAN_POINT('Ctrl Pts',(9.41568944744502,58.25,-7.43940805637597));
#292473=CARTESIAN_POINT('',(11.9139873655789,58.25,1.43419142823616));
#292474=CARTESIAN_POINT('Origin',(-4.60239784438011E-14,58.25,0.));
#292475=CARTESIAN_POINT('Ctrl Pts',(11.9139873655789,58.25,1.43419142823616));
#292476=CARTESIAN_POINT('Ctrl Pts',(11.7419322810054,58.1928633911005,2.86347211101975));
#292477=CARTESIAN_POINT('Ctrl Pts',(11.3140783609753,58.1341670582794,4.25018151571504));
#292478=CARTESIAN_POINT('Ctrl Pts',(9.99471722983137,58.0198787276206,6.7922574722224));
#292479=CARTESIAN_POINT('Ctrl Pts',(9.11862808992739,57.9661217678065,7.92967429883511));
#292480=CARTESIAN_POINT('Ctrl Pts',(6.88763929437055,57.8449802717658,9.95400993085742));
#292481=CARTESIAN_POINT('Ctrl Pts',(5.51132648159584,57.7803680058085,10.7771721335172));
#292482=CARTESIAN_POINT('Ctrl Pts',(2.55258779755992,57.6585671957128,11.8275757293221));
#292483=CARTESIAN_POINT('Ctrl Pts',(1.00349369270896,57.5968421723381,12.058220919922));
#292484=CARTESIAN_POINT('Ctrl Pts',(-2.10503272518202,57.4710996373618,
11.9164883058773));
#292485=CARTESIAN_POINT('Ctrl Pts',(-3.63477613369994,57.4117324362029,
11.5421964925761));
#292486=CARTESIAN_POINT('Ctrl Pts',(-6.47805324817245,57.2873231041572,
10.223163188254));
#292487=CARTESIAN_POINT('Ctrl Pts',(-7.76188571802245,57.2230287850605,
9.28608507812353));
#292488=CARTESIAN_POINT('Ctrl Pts',(-9.87548389609288,57.0992772380319,
6.99040032187376));
#292489=CARTESIAN_POINT('Ctrl Pts',(-10.6931193539723,57.0403744014441,
5.66109909495666));
#292490=CARTESIAN_POINT('Ctrl Pts',(-11.7416233824511,56.9196975169164,
2.86495497233163));
#292491=CARTESIAN_POINT('Ctrl Pts',(-12.,56.8615595351003,1.43769259310665));
#292492=CARTESIAN_POINT('Ctrl Pts',(-12.,56.806249999784,-1.0547118733939E-14));
#292493=CARTESIAN_POINT('Origin',(-8.79029313101884E-14,130.96875,0.));
#292494=CARTESIAN_POINT('',(-12.,53.431249999796,4.29975907498869E-14));
#292495=CARTESIAN_POINT('',(-12.,53.806249999796,7.34788079488412E-16));
#292496=CARTESIAN_POINT('',(-12.0000000000001,130.96875,-1.46957615897682E-15));
#292497=CARTESIAN_POINT('Ctrl Pts',(-12.,53.431249999796,3.88578058618805E-15));
#292498=CARTESIAN_POINT('Ctrl Pts',(-12.,53.4871296062859,1.45251078131059));
#292499=CARTESIAN_POINT('Ctrl Pts',(-11.7362697676557,53.545887435454,2.8941457146946));
#292500=CARTESIAN_POINT('Ctrl Pts',(-10.6723591125893,53.6671358170952,
5.7001391743692));
#292501=CARTESIAN_POINT('Ctrl Pts',(-9.84987352654367,53.725972253639,7.02644046693785));
#292502=CARTESIAN_POINT('Ctrl Pts',(-7.72828533595836,53.8497914258214,
9.31397212620167));
#292503=CARTESIAN_POINT('Ctrl Pts',(-6.44157098951665,53.9140624414862,
10.2461035663569));
#292504=CARTESIAN_POINT('Ctrl Pts',(-3.59357279785099,54.038389583625,11.5551820820907));
#292505=CARTESIAN_POINT('Ctrl Pts',(-2.06181728169446,54.0978477387845,
11.9241297682562));
#292506=CARTESIAN_POINT('Ctrl Pts',(1.04746123863136,54.2236206969434,12.0544267391436));
#292507=CARTESIAN_POINT('Ctrl Pts',(2.59528430838765,54.2851867498183,11.8182264369422));
#292508=CARTESIAN_POINT('Ctrl Pts',(5.54932503645201,54.4070775499409,10.7575718149213));
#292509=CARTESIAN_POINT('Ctrl Pts',(6.9222436218604,54.471686284401,9.92988638851982));
#292510=CARTESIAN_POINT('Ctrl Pts',(9.23772823991195,54.5977621257001,7.8143181733086));
#292511=CARTESIAN_POINT('Ctrl Pts',(10.1681933239522,54.6560602355255,6.55797590019966));
#292512=CARTESIAN_POINT('Ctrl Pts',(11.5065573354667,54.7809069275133,3.74762478934861));
#292513=CARTESIAN_POINT('Ctrl Pts',(11.8965194259829,54.8446360238262,2.21778406412077));
#292514=CARTESIAN_POINT('Ctrl Pts',(12.0681892059812,54.9673680294498,-0.916680721945098));
#292515=CARTESIAN_POINT('Ctrl Pts',(11.8437757627918,55.0290465072021,-2.49132058677692));
#292516=CARTESIAN_POINT('Ctrl Pts',(10.8089621012139,55.1552954021812,-5.43674945472044));
#292517=CARTESIAN_POINT('Ctrl Pts',(10.0190430503885,55.2146507485608,-6.78311694484928));
#292518=CARTESIAN_POINT('Ctrl Pts',(7.95132789589228,55.3379980910645,-9.12495403364958));
#292519=CARTESIAN_POINT('Ctrl Pts',(6.6842604992068,55.4024097965215,-10.0900443803154));
#292520=CARTESIAN_POINT('Ctrl Pts',(3.86824730793014,55.5272703674442,-11.4655816809358));
#292521=CARTESIAN_POINT('Ctrl Pts',(2.34999462310856,55.5861907204487,-11.8701464395861));
#292522=CARTESIAN_POINT('Ctrl Pts',(-0.754084089986135,55.7117533419867,
-12.0767338211216));
#292523=CARTESIAN_POINT('Ctrl Pts',(-2.31032311118788,55.774449098957,-11.8776203671417));
#292524=CARTESIAN_POINT('Ctrl Pts',(-5.29526061035131,55.895723166354,-10.8854303487974));
#292525=CARTESIAN_POINT('Ctrl Pts',(-6.6904886906033,55.9603406693356,-10.088082516988));
#292526=CARTESIAN_POINT('Ctrl Pts',(-9.05540439012356,56.0867960754365,
-8.02458642659485));
#292527=CARTESIAN_POINT('Ctrl Pts',(-10.0136161072456,56.1451514874907,
-6.79130808557009));
#292528=CARTESIAN_POINT('Ctrl Pts',(-11.4178762637581,56.26966311311,-4.01107750314829));
#292529=CARTESIAN_POINT('Ctrl Pts',(-11.8436234943505,56.333616439539,-2.48703553226478));
#292530=CARTESIAN_POINT('Ctrl Pts',(-11.9881437725539,56.4073920033214,
-0.61630231526467));
#292531=CARTESIAN_POINT('Ctrl Pts',(-12.,56.4194016589986,-0.307980743108728));
#292532=CARTESIAN_POINT('Ctrl Pts',(-12.,56.431249999784,-1.83880688453542E-13));
#292533=CARTESIAN_POINT('Ctrl Pts',(-12.,56.806249999784,-1.2490009027033E-15));
#292534=CARTESIAN_POINT('Ctrl Pts',(-12.,56.8008357843213,-0.14073481947853));
#292535=CARTESIAN_POINT('Ctrl Pts',(-11.9975242302304,56.7953868674467,
-0.281567226368526));
#292536=CARTESIAN_POINT('Ctrl Pts',(-11.9376166255646,56.7292090376622,
-1.98230049374114));
#292537=CARTESIAN_POINT('Ctrl Pts',(-11.5788604387752,56.6657013356079,
-3.51652580330893));
#292538=CARTESIAN_POINT('Ctrl Pts',(-10.2981943560748,56.5405961595996,
-6.35234303161689));
#292539=CARTESIAN_POINT('Ctrl Pts',(-9.3919473084131,56.482223365065,-7.62865707923812));
#292540=CARTESIAN_POINT('Ctrl Pts',(-7.1197472580277,56.3565060811356,-9.78872100964218));
#292541=CARTESIAN_POINT('Ctrl Pts',(-5.76663779028911,56.2919328603437,
-10.6421776962415));
#292542=CARTESIAN_POINT('Ctrl Pts',(-2.84000231878984,56.1695428275062,
-11.7615493915576));
#292543=CARTESIAN_POINT('Ctrl Pts',(-1.29953472732787,56.1088172837461,
-12.0295922776977));
#292544=CARTESIAN_POINT('Ctrl Pts',(1.8138700773441,55.9828774138792,-11.9649010019541));
#292545=CARTESIAN_POINT('Ctrl Pts',(3.35708379228035,55.9228280131136,-11.6266489732502));
#292546=CARTESIAN_POINT('Ctrl Pts',(6.23166838906527,55.7989872672075,-10.3746205954368));
#292547=CARTESIAN_POINT('Ctrl Pts',(7.53448615261147,55.7348647064474,-9.47089739641282));
#292548=CARTESIAN_POINT('Ctrl Pts',(9.70132975098782,55.6106784867606,-7.2302169988211));
#292549=CARTESIAN_POINT('Ctrl Pts',(10.5514300340919,55.5521470124149,-5.92107369846786));
#292550=CARTESIAN_POINT('Ctrl Pts',(11.7234859051004,55.425645911933,-3.01368180469527));
#292551=CARTESIAN_POINT('Ctrl Pts',(12.018968228371,55.3617859544397,-1.43741489019202));
#292552=CARTESIAN_POINT('Ctrl Pts',(11.9795299887659,55.2402991338749,1.70764771572582));
#292553=CARTESIAN_POINT('Ctrl Pts',(11.6570644007191,55.1770790288273,3.24618888105004));
#292554=CARTESIAN_POINT('Ctrl Pts',(10.4438112629329,55.0517127580189,6.11069669039277));
#292555=CARTESIAN_POINT('Ctrl Pts',(9.5657907603954,54.9931091100837,7.41009407699998));
#292556=CARTESIAN_POINT('Ctrl Pts',(7.34415819072201,54.8678404916379,9.62088798132063));
#292557=CARTESIAN_POINT('Ctrl Pts',(6.01448847362389,54.8033403588107,10.503532747568));
#292558=CARTESIAN_POINT('Ctrl Pts',(3.12026983466767,54.6804135344638,11.6900990248898));
#292559=CARTESIAN_POINT('Ctrl Pts',(1.58837964561655,54.6205013061338,11.9946500945103));
#292560=CARTESIAN_POINT('Ctrl Pts',(-1.52936066374502,54.4943860614182,
12.0052882362664));
#292561=CARTESIAN_POINT('Ctrl Pts',(-3.08554247314003,54.4335144510827,
11.7023598441195));
#292562=CARTESIAN_POINT('Ctrl Pts',(-5.98961160773956,54.3102627229801,
10.5156866498795));
#292563=CARTESIAN_POINT('Ctrl Pts',(-7.31002011518611,54.2463408201135,
9.64461440052666));
#292564=CARTESIAN_POINT('Ctrl Pts',(-9.5276000616501,54.1217765985134,7.45786840585217));
#292565=CARTESIAN_POINT('Ctrl Pts',(-10.4089750696479,54.0634395118941,
6.16831971457848));
#292566=CARTESIAN_POINT('Ctrl Pts',(-11.6504069111924,53.9370385412999,
3.28607217389276));
#292567=CARTESIAN_POINT('Ctrl Pts',(-11.9829544758109,53.8724201434715,
1.7144602120856));
#292568=CARTESIAN_POINT('Ctrl Pts',(-11.999787336411,53.8094266493438,0.0825033819025622));
#292569=CARTESIAN_POINT('Ctrl Pts',(-12.,53.8078368125135,0.0412469364927481));
#292570=CARTESIAN_POINT('Ctrl Pts',(-12.,53.806249999796,2.93915231795365E-15));
#292571=CARTESIAN_POINT('Origin',(-8.79029313101884E-14,130.96875,0.));
#292572=CARTESIAN_POINT('',(-12.,50.431249999808,-4.62056866567646E-15));
#292573=CARTESIAN_POINT('',(-12.,50.806249999808,6.52193984771498E-14));
#292574=CARTESIAN_POINT('',(-12.0000000000001,130.96875,-1.46957615897682E-15));
#292575=CARTESIAN_POINT('Ctrl Pts',(-12.,50.431249999808,2.93915231795365E-15));
#292576=CARTESIAN_POINT('Ctrl Pts',(-12.,50.4333746432347,0.0552270797444227));
#292577=CARTESIAN_POINT('Ctrl Pts',(-11.9996187466256,50.4355046952934,
0.110470872436941));
#292578=CARTESIAN_POINT('Ctrl Pts',(-11.9768936043853,50.4990861513974,
1.75579641839743));
#292579=CARTESIAN_POINT('Ctrl Pts',(-11.6390809684786,50.5637046711776,
3.32570082480313));
#292580=CARTESIAN_POINT('Ctrl Pts',(-10.3881127909486,50.6900514144101,
6.20344025906615));
#292581=CARTESIAN_POINT('Ctrl Pts',(-9.50226042672603,50.7483738478049,
7.49016928165803));
#292582=CARTESIAN_POINT('Ctrl Pts',(-7.27746453080368,50.8729888469884,
9.66911900238871));
#292583=CARTESIAN_POINT('Ctrl Pts',(-5.95459568647555,50.936879186898,10.5354773982616));
#292584=CARTESIAN_POINT('Ctrl Pts',(-3.04636173817073,51.060043252087,11.7127312485299));
#292585=CARTESIAN_POINT('Ctrl Pts',(-1.48832533954868,51.1210459751629,
12.0105532498137));
#292586=CARTESIAN_POINT('Ctrl Pts',(1.63000466665062,51.2471850736166,11.9890404478604));
#292587=CARTESIAN_POINT('Ctrl Pts',(3.16064508284471,51.3069934116536,11.6792235396826));
#292588=CARTESIAN_POINT('Ctrl Pts',(6.05010037198389,51.4299944549249,10.4829795379728));
#292589=CARTESIAN_POINT('Ctrl Pts',(7.37632612828183,51.4944811634555,9.59615917197936));
#292590=CARTESIAN_POINT('Ctrl Pts',(9.59058322802632,51.6196817306165,7.37807593840257));
#292591=CARTESIAN_POINT('Ctrl Pts',(10.4644911620606,51.6783317258522,6.07533323433215));
#292592=CARTESIAN_POINT('Ctrl Pts',(11.6679105771596,51.8037324189243,3.20673549708131));
#292593=CARTESIAN_POINT('Ctrl Pts',(11.9850988204085,51.8669080122012,1.66763663857078));
#292594=CARTESIAN_POINT('Ctrl Pts',(12.0141746424869,51.9882919802791,-1.47811941699711));
#292595=CARTESIAN_POINT('Ctrl Pts',(11.7130740031476,52.0523453898995,-3.05447428151856));
#292596=CARTESIAN_POINT('Ctrl Pts',(10.530191958422,52.1788634877723,-5.95879036118455));
#292597=CARTESIAN_POINT('Ctrl Pts',(9.67534739336931,52.2373551303859,-7.26497244843828));
#292598=CARTESIAN_POINT('Ctrl Pts',(7.50077083482246,52.3616012930252,-9.49753044946365));
#292599=CARTESIAN_POINT('Ctrl Pts',(6.19523966964062,52.4256956418871,-10.3963324217276));
#292600=CARTESIAN_POINT('Ctrl Pts',(3.31613883858384,52.5494496519484,-11.6384967577646));
#292601=CARTESIAN_POINT('Ctrl Pts',(1.7709568382787,52.6096132908761,-11.9714288361293));
#292602=CARTESIAN_POINT('Ctrl Pts',(-1.34312935883758,52.7355807236463,
-12.0247635155693));
#292603=CARTESIAN_POINT('Ctrl Pts',(-2.88231279120065,52.7961732160391,
-11.7512130832305));
#292604=CARTESIAN_POINT('Ctrl Pts',(-5.80412602816963,52.918646690625,-10.6216947176347));
#292605=CARTESIAN_POINT('Ctrl Pts',(-7.1537488290025,52.9832111124131,-9.76380911854804));
#292606=CARTESIAN_POINT('Ctrl Pts',(-9.41838431356261,53.1088632934264,
-7.59607158678609));
#292607=CARTESIAN_POINT('Ctrl Pts',(-10.3204048871767,53.1672608749328,
-6.31628776693271));
#292608=CARTESIAN_POINT('Ctrl Pts',(-11.5909871582565,53.292407903375,-3.4761062152077));
#292609=CARTESIAN_POINT('Ctrl Pts',(-11.9443028041032,53.3558745509222,
-1.9411803201662));
#292610=CARTESIAN_POINT('Ctrl Pts',(-11.9979789277012,53.421437949922,-0.254393574972973));
#292611=CARTESIAN_POINT('Ctrl Pts',(-12.,53.4263581727884,-0.127156075625299));
#292612=CARTESIAN_POINT('Ctrl Pts',(-12.,53.431249999796,2.34187669256869E-14));
#292613=CARTESIAN_POINT('Ctrl Pts',(-12.,53.806249999796,1.4432899320127E-14));
#292614=CARTESIAN_POINT('Ctrl Pts',(-12.,53.7480939148037,-1.51168459759066));
#292615=CARTESIAN_POINT('Ctrl Pts',(-11.7143465683857,53.6868690266145,
-3.01032393715114));
#292616=CARTESIAN_POINT('Ctrl Pts',(-10.5844918994098,53.562939921336,-5.86457248065474));
#292617=CARTESIAN_POINT('Ctrl Pts',(-9.73501285958027,53.5039492278736,
-7.18708934061602));
#292618=CARTESIAN_POINT('Ctrl Pts',(-7.56459251217115,53.3791664941359,
-9.44793524513585));
#292619=CARTESIAN_POINT('Ctrl Pts',(-6.25896026340131,53.3147736776583,
-10.3591511846968));
#292620=CARTESIAN_POINT('Ctrl Pts',(-3.39799737004919,53.1913523776906,
-11.6122869664658));
#292621=CARTESIAN_POINT('Ctrl Pts',(-1.87477951714514,53.1320864243024,
-11.9531081269277));
#292622=CARTESIAN_POINT('Ctrl Pts',(1.24683572774671,53.0058144351521,-12.0386941530778));
#292623=CARTESIAN_POINT('Ctrl Pts',(2.81570505813728,52.9439768965327,-11.7709951509428));
#292624=CARTESIAN_POINT('Ctrl Pts',(5.74801110444513,52.8213424941071,-10.6491505166484));
#292625=CARTESIAN_POINT('Ctrl Pts',(7.08497336545378,52.7576510477283,-9.81055520606376));
#292626=CARTESIAN_POINT('Ctrl Pts',(9.35172990701891,52.6327560522224,-7.67758313712671));
#292627=CARTESIAN_POINT('Ctrl Pts',(10.263773913544,52.5744530895322,-6.40742326293614));
#292628=CARTESIAN_POINT('Ctrl Pts',(11.5702421647988,52.4484392107677,-3.55636923351588));
#292629=CARTESIAN_POINT('Ctrl Pts',(11.9386514798297,52.3838349192808,-1.99677613501637));
#292630=CARTESIAN_POINT('Ctrl Pts',(12.0460453155768,52.2618526617759,1.13908453685275));
#292631=CARTESIAN_POINT('Ctrl Pts',(11.7982071860678,52.200445948804,2.68465914904394));
#292632=CARTESIAN_POINT('Ctrl Pts',(10.7243954194677,52.0746421717493,5.60584655808609));
#292633=CARTESIAN_POINT('Ctrl Pts',(9.90474876030528,52.0150868999077,6.95227710948971));
#292634=CARTESIAN_POINT('Ctrl Pts',(7.78788701011688,51.8908449260673,9.26409655473338));
#292635=CARTESIAN_POINT('Ctrl Pts',(6.50768448347384,51.8265986328547,10.2041509569471));
#292636=CARTESIAN_POINT('Ctrl Pts',(3.68194428913401,51.702711177516,11.5253724153568));
#292637=CARTESIAN_POINT('Ctrl Pts',(2.16778571004633,51.6439387737841,11.9034275032323));
#292638=CARTESIAN_POINT('Ctrl Pts',(-0.957341155162895,51.517524736608,
12.0660569027066));
#292639=CARTESIAN_POINT('Ctrl Pts',(-2.53901199783854,51.4545455404943,
11.8346610204564));
#292640=CARTESIAN_POINT('Ctrl Pts',(-5.49921221111154,51.3325770637309,
10.7792172403802));
#292641=CARTESIAN_POINT('Ctrl Pts',(-6.85221550876325,51.2691531618878,
9.97395304151869));
#292642=CARTESIAN_POINT('Ctrl Pts',(-9.1681705344409,51.1439643127511,7.8963378369432));
#292643=CARTESIAN_POINT('Ctrl Pts',(-10.1112860675465,51.0855377818822,
6.64600774787707));
#292644=CARTESIAN_POINT('Ctrl Pts',(-11.4829497441587,50.959952982895,3.82729031393066));
#292645=CARTESIAN_POINT('Ctrl Pts',(-11.887186090446,50.8953983536027,2.2806290215588));
#292646=CARTESIAN_POINT('Ctrl Pts',(-11.9931989855778,50.8242908749857,
0.466737071064205));
#292647=CARTESIAN_POINT('Ctrl Pts',(-12.,50.8152236502517,0.233257262100788));
#292648=CARTESIAN_POINT('Ctrl Pts',(-12.,50.806249999808,2.15313877838241E-13));
#292649=CARTESIAN_POINT('Origin',(-8.79029313101884E-14,130.96875,0.));
#292650=CARTESIAN_POINT('',(-12.,47.43124999982,8.60360801888715E-14));
#292651=CARTESIAN_POINT('',(-12.,47.80624999982,1.14936573298645E-13));
#292652=CARTESIAN_POINT('',(-12.0000000000001,130.96875,-1.46957615897682E-15));
#292653=CARTESIAN_POINT('Ctrl Pts',(-12.,47.43124999982,2.31065167000111E-13));
#292654=CARTESIAN_POINT('Ctrl Pts',(-12.,47.4407678727725,0.247403551082924));
#292655=CARTESIAN_POINT('Ctrl Pts',(-11.9923490646664,47.4503907550039,
0.495050729214709));
#292656=CARTESIAN_POINT('Ctrl Pts',(-11.8790644606491,47.5220984700527,
2.32218224939318));
#292657=CARTESIAN_POINT('Ctrl Pts',(-11.4696027511409,47.5866428237261,
3.86687861825634));
#292658=CARTESIAN_POINT('Ctrl Pts',(-10.0884088594892,47.7121614098843,
6.68077838944382));
#292659=CARTESIAN_POINT('Ctrl Pts',(-9.14072251871325,47.7706195334804,
7.92817496660893));
#292660=CARTESIAN_POINT('Ctrl Pts',(-6.81758560523962,47.89584804637,9.99757334818262));
#292661=CARTESIAN_POINT('Ctrl Pts',(-5.46228610104156,47.9592297004385,
10.7979002123034));
#292662=CARTESIAN_POINT('Ctrl Pts',(-2.49804490039839,48.0810967543812,
11.8435163598417));
#292663=CARTESIAN_POINT('Ctrl Pts',(-0.914496854331955,48.1442578249945,
12.0695190218114));
#292664=CARTESIAN_POINT('Ctrl Pts',(2.21110912803724,48.2706912428669,11.8954602673166));
#292665=CARTESIAN_POINT('Ctrl Pts',(3.72391114734811,48.3294052303618,11.5118855378486));
#292666=CARTESIAN_POINT('Ctrl Pts',(6.54433692350144,48.4533581435511,10.1805963520437));
#292667=CARTESIAN_POINT('Ctrl Pts',(7.82070636620124,48.5175795628426,9.23631232192927));
#292668=CARTESIAN_POINT('Ctrl Pts',(9.9295451305108,48.6417377379988,6.91697463000914));
#292669=CARTESIAN_POINT('Ctrl Pts',(10.7447224853498,48.7013913232631,5.5669845201973));
#292670=CARTESIAN_POINT('Ctrl Pts',(11.8078795147673,48.8272247409165,2.64156471203725));
#292671=CARTESIAN_POINT('Ctrl Pts',(12.0500395478662,48.8884798877763,1.09548931021175));
#292672=CARTESIAN_POINT('Ctrl Pts',(11.9314334482903,49.0105503990855,-2.03902230824284));
#292673=CARTESIAN_POINT('Ctrl Pts',(11.5576773465329,49.0751495604682,-3.59674478067195));
#292674=CARTESIAN_POINT('Ctrl Pts',(10.2414947097431,49.2011021244793,-6.44304862520994));
#292675=CARTESIAN_POINT('Ctrl Pts',(9.32484211207299,49.2594133717901,-7.71027961852137));
#292676=CARTESIAN_POINT('Ctrl Pts',(7.05074793878167,49.3843545943596,-9.8350965442519));
#292677=CARTESIAN_POINT('Ctrl Pts',(5.71135946361982,49.4480085240933,-10.6687745641359));
#292678=CARTESIAN_POINT('Ctrl Pts',(2.77487011449975,49.5705467408296,-11.7808159513214));
#292679=CARTESIAN_POINT('Ctrl Pts',(1.2040981552789,49.6325432062857,-12.043169752985));
#292680=CARTESIAN_POINT('Ctrl Pts',(-1.91806513933708,49.7588373645131,
-11.9462280010008));
#292681=CARTESIAN_POINT('Ctrl Pts',(-3.43995695565266,49.8180196669659,
-11.5999157144062));
#292682=CARTESIAN_POINT('Ctrl Pts',(-6.29579415143742,49.941512382835,-10.3367213702745));
#292683=CARTESIAN_POINT('Ctrl Pts',(-7.59772347007663,50.0058859134419,
-9.42121991920977));
#292684=CARTESIAN_POINT('Ctrl Pts',(-9.76030732451788,50.1305915776529,
-7.15282943528729));
#292685=CARTESIAN_POINT('Ctrl Pts',(-10.6054210782084,50.1896547997765,
-5.82679696083733));
#292686=CARTESIAN_POINT('Ctrl Pts',(-11.7198746329126,50.3130500057532,
-2.98142224388078));
#292687=CARTESIAN_POINT('Ctrl Pts',(-12.,50.3736594394224,-1.49698459091494));
#292688=CARTESIAN_POINT('Ctrl Pts',(-12.,50.431249999808,-3.60822483003176E-15));
#292689=CARTESIAN_POINT('Ctrl Pts',(-12.,50.806249999808,2.11775041947249E-13));
#292690=CARTESIAN_POINT('Ctrl Pts',(-12.,50.7557911893547,-1.31160490918796));
#292691=CARTESIAN_POINT('Ctrl Pts',(-11.784958795216,50.7029229735181,-2.61596775665401));
#292692=CARTESIAN_POINT('Ctrl Pts',(-10.8579681788226,50.586384972594,-5.34400959596382));
#292693=CARTESIAN_POINT('Ctrl Pts',(-10.0683905445584,50.526101142349,-6.71426830879258));
#292694=CARTESIAN_POINT('Ctrl Pts',(-8.00548678663434,50.4024364306604,
-9.07607578521367));
#292695=CARTESIAN_POINT('Ctrl Pts',(-6.75117323967514,50.3383716329531,
-10.0441298842934));
#292696=CARTESIAN_POINT('Ctrl Pts',(-3.96136200713807,50.2140653698115,
-11.4324177395091));
#292697=CARTESIAN_POINT('Ctrl Pts',(-2.45632658584548,50.1556104973947,
-11.8473194713069));
#292698=CARTESIAN_POINT('Ctrl Pts',(0.6717896556587,50.0290755374074,-12.086283174021));
#292699=CARTESIAN_POINT('Ctrl Pts',(2.26588548555627,49.9648219505577,-11.8909449059983));
#292700=CARTESIAN_POINT('Ctrl Pts',(5.25260223989149,49.8435434241694,-10.9010162838714));
#292701=CARTESIAN_POINT('Ctrl Pts',(6.62053656282354,49.7804138038033,-10.1286799125176));
#292702=CARTESIAN_POINT('Ctrl Pts',(8.98388750296656,49.6549790246415,-8.10595614246599));
#292703=CARTESIAN_POINT('Ctrl Pts',(9.95734378372957,49.5962785807417,-6.87518063584317));
#292704=CARTESIAN_POINT('Ctrl Pts',(11.3919731722414,49.4711479557705,-4.08872760854805));
#292705=CARTESIAN_POINT('Ctrl Pts',(11.8306707335156,49.406675621401,-2.5554025829876));
#292706=CARTESIAN_POINT('Ctrl Pts',(12.0863157245536,49.2836000769814,0.560706804715852));
#292707=CARTESIAN_POINT('Ctrl Pts',(11.9134519368995,49.2238937129125,2.11261320746752));
#292708=CARTESIAN_POINT('Ctrl Pts',(10.9806134950917,49.0977307783428,5.08894141443361));
#292709=CARTESIAN_POINT('Ctrl Pts',(10.2202603227565,49.0365917722932,6.48207908223318));
#292710=CARTESIAN_POINT('Ctrl Pts',(8.20972359130218,48.9135173804856,8.89113562490776));
#292711=CARTESIAN_POINT('Ctrl Pts',(6.98076465471862,48.8496597446431,9.88537443630402));
#292712=CARTESIAN_POINT('Ctrl Pts',(4.2262356362271,48.7249941615828,11.3373365458814));
#292713=CARTESIAN_POINT('Ctrl Pts',(2.7300589348449,48.6666832035132,11.7874093317986));
#292714=CARTESIAN_POINT('Ctrl Pts',(-0.392026331067906,48.5403922016132,
12.0984721210039));
#292715=CARTESIAN_POINT('Ctrl Pts',(-1.98946818663386,48.4757743211795,
11.9402272870843));
#292716=CARTESIAN_POINT('Ctrl Pts',(-4.99444789369535,48.3542203386418,
11.0211812157372));
#292717=CARTESIAN_POINT('Ctrl Pts',(-6.37721571212599,48.2920486779669,
10.2831227191624));
#292718=CARTESIAN_POINT('Ctrl Pts',(-8.78896645640985,48.1663900703293,
8.31760167700385));
#292719=CARTESIAN_POINT('Ctrl Pts',(-9.79368884331946,48.1072498720136,
7.1071890123526));
#292720=CARTESIAN_POINT('Ctrl Pts',(-11.292468355393,47.9826229572552,4.35467285326218));
#292721=CARTESIAN_POINT('Ctrl Pts',(-11.7661084694716,47.9182697115858,
2.83579689248597));
#292722=CARTESIAN_POINT('Ctrl Pts',(-11.9776268652391,47.8390998979341,
0.846616841177166));
#292723=CARTESIAN_POINT('Ctrl Pts',(-12.,47.8225261014706,0.423074080334272));
#292724=CARTESIAN_POINT('Ctrl Pts',(-12.,47.80624999982,1.73611125475759E-13));
#292725=CARTESIAN_POINT('Origin',(-8.79029313101884E-14,130.96875,0.));
#292726=CARTESIAN_POINT('',(-12.,44.431249999832,4.71435798574715E-14));
#292727=CARTESIAN_POINT('',(-12.,44.806249999832,4.32577992712834E-14));
#292728=CARTESIAN_POINT('',(-12.0000000000001,130.96875,-1.46957615897682E-15));
#292729=CARTESIAN_POINT('Ctrl Pts',(-12.,44.431249999832,2.12191375581483E-13));
#292730=CARTESIAN_POINT('Ctrl Pts',(-12.,44.4480633973018,0.437040319885026));
#292731=CARTESIAN_POINT('Ctrl Pts',(-11.9761253853199,44.4651936746564,
0.874560148487268));
#292732=CARTESIAN_POINT('Ctrl Pts',(-11.7561719971819,44.5449565599248,
2.87641555660222));
#292733=CARTESIAN_POINT('Ctrl Pts',(-11.2774887994135,44.6092895857453,
4.39312733398706));
#292734=CARTESIAN_POINT('Ctrl Pts',(-9.769422444749,44.7338401007517,7.14064011226523));
#292735=CARTESIAN_POINT('Ctrl Pts',(-8.76014300197083,44.7930576606372,
8.3480659234863));
#292736=CARTESIAN_POINT('Ctrl Pts',(-6.34137693634925,44.9187463133987,
10.3051948567027));
#292737=CARTESIAN_POINT('Ctrl Pts',(-4.95646526673096,44.9807567681892,
11.0382537859001));
#292738=CARTESIAN_POINT('Ctrl Pts',(-1.9493068899536,45.1023988797682,11.9467775902144));
#292739=CARTESIAN_POINT('Ctrl Pts',(-0.351898131209509,45.1670154214074,
12.0996351633707));
#292740=CARTESIAN_POINT('Ctrl Pts',(2.76884245591405,45.2932520299078,11.7783891778682));
#292741=CARTESIAN_POINT('Ctrl Pts',(4.26374680592003,45.3515551502874,11.323313415966));
#292742=CARTESIAN_POINT('Ctrl Pts',(7.01317923842076,45.4762685836509,9.86232394612193));
#292743=CARTESIAN_POINT('Ctrl Pts',(8.23848222451373,45.5400940614743,8.86440566825877));
#292744=CARTESIAN_POINT('Ctrl Pts',(10.2415028621997,45.6630813533292,6.44866740241013));
#292745=CARTESIAN_POINT('Ctrl Pts',(10.9976565736167,45.7243547713553,5.05226566134454));
#292746=CARTESIAN_POINT('Ctrl Pts',(11.92054272461,45.8505403224076,2.07211587581859));
#292747=CARTESIAN_POINT('Ctrl Pts',(12.0881258529366,45.9101517109846,0.519786142751066));
#292748=CARTESIAN_POINT('Ctrl Pts',(11.8220280136357,46.0332982737874,-2.59477293038869));
#292749=CARTESIAN_POINT('Ctrl Pts',(11.3784104957874,46.0977560372114,-4.12612061417768));
#292750=CARTESIAN_POINT('Ctrl Pts',(9.93476841314932,46.2228184111249,-6.90787115060338));
#292751=CARTESIAN_POINT('Ctrl Pts',(8.95694147161195,46.28157074466,-8.13581345040347));
#292752=CARTESIAN_POINT('Ctrl Pts',(6.58681770431223,46.4070375608798,-10.1505626538572));
#292753=CARTESIAN_POINT('Ctrl Pts',(5.21679342013365,46.4701221067991,-10.9181266772137));
#292754=CARTESIAN_POINT('Ctrl Pts',(2.22631721205064,46.5912979910622,-11.8985638824829));
#292755=CARTESIAN_POINT('Ctrl Pts',(0.63043916516099,46.6557481998966,-12.0886574981134));
#292756=CARTESIAN_POINT('Ctrl Pts',(-2.49806951449905,46.7822990343408,
-11.8386062570599));
#292757=CARTESIAN_POINT('Ctrl Pts',(-4.00176733541213,46.8407219916465,
-11.4183558921771));
#292758=CARTESIAN_POINT('Ctrl Pts',(-6.78627496913661,46.9650854684867,
-10.0203619377339));
#292759=CARTESIAN_POINT('Ctrl Pts',(-8.03677248548348,47.0291208981668,
-9.04829069795741));
#292760=CARTESIAN_POINT('Ctrl Pts',(-10.0917662518949,47.1526983168778,
-6.67926746296542));
#292761=CARTESIAN_POINT('Ctrl Pts',(-10.8769328846958,47.2131020949138,
-5.30553745375233));
#292762=CARTESIAN_POINT('Ctrl Pts',(-11.7897156391528,47.3290914917053,
-2.58713938330585));
#292763=CARTESIAN_POINT('Ctrl Pts',(-12.,47.3813523556844,-1.29701819002632));
#292764=CARTESIAN_POINT('Ctrl Pts',(-12.,47.43124999982,2.16771045558062E-13));
#292765=CARTESIAN_POINT('Ctrl Pts',(-12.,47.80624999982,2.04003480774873E-13));
#292766=CARTESIAN_POINT('Ctrl Pts',(-12.,47.7632541030443,-1.11761709757617));
#292767=CARTESIAN_POINT('Ctrl Pts',(-11.8438691418875,47.7184381854061,
-2.23181305421852));
#292768=CARTESIAN_POINT('Ctrl Pts',(-11.0991279573074,47.6092880553311,
-4.82703414338412));
#292769=CARTESIAN_POINT('Ctrl Pts',(-10.3687627631493,47.5471277954344,
-6.24334594351771));
#292770=CARTESIAN_POINT('Ctrl Pts',(-8.41183557330947,47.4246874049577,
-8.69952455205501));
#292771=CARTESIAN_POINT('Ctrl Pts',(-7.20903772274042,47.3610720405269,
-9.71958143976674));
#292772=CARTESIAN_POINT('Ctrl Pts',(-4.49103627275375,47.2360851638739,
-11.2353325572595));
#292773=CARTESIAN_POINT('Ctrl Pts',(-3.00394262343975,47.177762031447,-11.720854706413));
#292774=CARTESIAN_POINT('Ctrl Pts',(0.108228352968689,47.0518720709817,
-12.103841048153));
#292775=CARTESIAN_POINT('Ctrl Pts',(1.70506011519628,46.987278869342,-11.9836421050193));
#292776=CARTESIAN_POINT('Ctrl Pts',(4.72498218786174,46.8651204554188,-11.1389841017771));
#292777=CARTESIAN_POINT('Ctrl Pts',(6.12279678628232,46.804014061626,-10.436191065797));
#292778=CARTESIAN_POINT('Ctrl Pts',(8.58385739181458,46.678151220751,-8.52994948380035));
#292779=CARTESIAN_POINT('Ctrl Pts',(9.62066378834719,46.618395094874,-7.34067395799302));
#292780=CARTESIAN_POINT('Ctrl Pts',(11.1844836000381,46.4943220083027,-4.6236866482046));
#292781=CARTESIAN_POINT('Ctrl Pts',(11.6933529492508,46.430126384601,-3.12035451835472));
#292782=CARTESIAN_POINT('Ctrl Pts',(12.0991883805569,46.3061087047262,-0.0285554936068377));
#292783=CARTESIAN_POINT('Ctrl Pts',(12.0022010561016,46.2474495293521,1.52914964686318));
#292784=CARTESIAN_POINT('Ctrl Pts',(11.2126464649974,46.1209970957569,4.55955871390806));
#292785=CARTESIAN_POINT('Ctrl Pts',(10.5129341842395,46.0576501769004,5.99922541638793));
#292786=CARTESIAN_POINT('Ctrl Pts',(8.61062745985699,45.9358856515147,8.50215678159028));
#292787=CARTESIAN_POINT('Ctrl Pts',(7.43466838544492,45.8725470762023,9.54751274348946));
#292788=CARTESIAN_POINT('Ctrl Pts',(4.75429418025336,45.7472797427785,11.1268489084341));
#292789=CARTESIAN_POINT('Ctrl Pts',(3.27648282411912,45.688786514153,11.6479513487885));
#292790=CARTESIAN_POINT('Ctrl Pts',(0.175152526872331,45.5633350683713,
12.1025662801572));
#292791=CARTESIAN_POINT('Ctrl Pts',(-1.42019834163361,45.498801770141,12.0202321282542));
#292792=CARTESIAN_POINT('Ctrl Pts',(-4.45396624172863,45.3760832807332,
11.249820552242));
#292793=CARTESIAN_POINT('Ctrl Pts',(-5.86655654536747,45.315867792378,10.582056634735));
#292794=CARTESIAN_POINT('Ctrl Pts',(-8.37619037859286,45.1898200456127,
8.73489350280551));
#292795=CARTESIAN_POINT('Ctrl Pts',(-9.44472037212808,45.1292928650767,
7.56677849119635));
#292796=CARTESIAN_POINT('Ctrl Pts',(-11.0720581406693,45.0058035139223,
4.88560278740076));
#292797=CARTESIAN_POINT('Ctrl Pts',(-11.6151138397186,44.9417981794053,
3.39832477228253));
#292798=CARTESIAN_POINT('Ctrl Pts',(-11.9523124591163,44.8543875745271,
1.23577307049343));
#292799=CARTESIAN_POINT('Ctrl Pts',(-12.,44.8300125392067,0.617673366029319));
#292800=CARTESIAN_POINT('Ctrl Pts',(-12.,44.806249999832,-3.46944695195361E-15));
#292801=CARTESIAN_POINT('Origin',(-8.79029313101884E-14,130.96875,0.));
#292802=CARTESIAN_POINT('',(-12.,41.431249999844,-1.46125758873029E-14));
#292803=CARTESIAN_POINT('',(-12.,41.806249999844,-1.69717998146313E-14));
#292804=CARTESIAN_POINT('',(-12.0000000000001,130.96875,-1.46957615897682E-15));
#292805=CARTESIAN_POINT('Ctrl Pts',(-12.,41.431249999844,9.43689570931383E-15));
#292806=CARTESIAN_POINT('Ctrl Pts',(-12.,41.4555295818647,0.631113153188752));
#292807=CARTESIAN_POINT('Ctrl Pts',(-11.9502146704977,41.480447020204,1.26263023873752));
#292808=CARTESIAN_POINT('Ctrl Pts',(-11.6036949894875,41.5684241015784,
3.43687809370616));
#292809=CARTESIAN_POINT('Ctrl Pts',(-11.0559156247007,41.6324001760595,
4.92186072382863));
#292810=CARTESIAN_POINT('Ctrl Pts',(-9.41976702018347,41.7558051513705,
7.59798038360397));
#292811=CARTESIAN_POINT('Ctrl Pts',(-8.34680511181584,41.8164527518273,
8.76311730869326));
#292812=CARTESIAN_POINT('Ctrl Pts',(-5.83039947901914,41.9425249504412,
10.6019882659294));
#292813=CARTESIAN_POINT('Ctrl Pts',(-4.41575251688016,42.0026290583863,
11.2648449144665));
#292814=CARTESIAN_POINT('Ctrl Pts',(-1.38012561054793,42.1254227461761,
12.0248295578064));
#292815=CARTESIAN_POINT('Ctrl Pts',(0.214947713004328,42.1899448174772,
12.1018562767893));
#292816=CARTESIAN_POINT('Ctrl Pts',(3.31467996834863,42.315331621106,11.6371948376792));
#292817=CARTESIAN_POINT('Ctrl Pts',(4.79116959092115,42.3738614683273,11.1110785709522));
#292818=CARTESIAN_POINT('Ctrl Pts',(7.46616442758904,42.4991648908377,9.52282048797467));
#292819=CARTESIAN_POINT('Ctrl Pts',(8.63829657933997,42.5624617695215,8.47395091611032));
#292820=CARTESIAN_POINT('Ctrl Pts',(10.5328423833091,42.6841278665148,5.96447730981581));
#292821=CARTESIAN_POINT('Ctrl Pts',(11.2281896251307,42.7476550373785,4.52151316204852));
#292822=CARTESIAN_POINT('Ctrl Pts',(12.0074663393262,42.8741251897373,1.48730403633692));
#292823=CARTESIAN_POINT('Ctrl Pts',(12.0990229616799,42.9327356783733,-0.0707926080980731));
#292824=CARTESIAN_POINT('Ctrl Pts',(11.6824444101056,43.0568142310699,-3.16068328377196));
#292825=CARTESIAN_POINT('Ctrl Pts',(11.1686012325138,43.1209844862839,-4.66173990110958));
#292826=CARTESIAN_POINT('Ctrl Pts',(9.59556606119807,43.2449755342907,-7.37360048341212));
#292827=CARTESIAN_POINT('Ctrl Pts',(8.55418145173455,43.3048330375685,-8.55983872995765));
#292828=CARTESIAN_POINT('Ctrl Pts',(6.08609991188275,43.4307236214075,-10.4575836520369));
#292829=CARTESIAN_POINT('Ctrl Pts',(4.68614689785719,43.4916913759107,-11.1553316022767));
#292830=CARTESIAN_POINT('Ctrl Pts',(1.66416888938256,43.6139329541844,-11.9893170423389));
#292831=CARTESIAN_POINT('Ctrl Pts',(0.067496458510527,43.6785197107354,
-12.104065813472));
#292832=CARTESIAN_POINT('Ctrl Pts',(-3.04317437145658,43.8043489890024,
-11.7107734300768));
#292833=CARTESIAN_POINT('Ctrl Pts',(-4.52894729934066,43.8626868170876,
-11.2201494953272));
#292834=CARTESIAN_POINT('Ctrl Pts',(-7.24161258390349,43.9877165151098,
-9.69525277413838));
#292835=CARTESIAN_POINT('Ctrl Pts',(-8.4405970497795,44.0512942543223,-8.67152967250919));
#292836=CARTESIAN_POINT('Ctrl Pts',(-10.3897417120076,44.1736401674515,
-6.20861290814931));
#292837=CARTESIAN_POINT('Ctrl Pts',(-11.115746097572,44.2359606257585,-4.78895761877185));
#292838=CARTESIAN_POINT('Ctrl Pts',(-11.8477912822414,44.3445657147565,
-2.20377891566744));
#292839=CARTESIAN_POINT('Ctrl Pts',(-12.,44.3887975354914,-1.10349134543309));
#292840=CARTESIAN_POINT('Ctrl Pts',(-12.,44.431249999832,2.11775041947249E-13));
#292841=CARTESIAN_POINT('Ctrl Pts',(-12.,44.806249999832,1.2490009027033E-14));
#292842=CARTESIAN_POINT('Ctrl Pts',(-12.,44.7707571013409,-0.922587343696966));
#292843=CARTESIAN_POINT('Ctrl Pts',(-11.8936087828564,44.7339748643673,
-1.84412060288041));
#292844=CARTESIAN_POINT('Ctrl Pts',(-11.3171654079714,44.6324372407734,
-4.29614870177773));
#292845=CARTESIAN_POINT('Ctrl Pts',(-10.6479128705179,44.5678230724129,
-5.75824864709434));
#292846=CARTESIAN_POINT('Ctrl Pts',(-8.79958584391621,44.4467137796665,
-8.30575435989554));
#292847=CARTESIAN_POINT('Ctrl Pts',(-7.65025428745581,44.383701387247,-9.37510781353939));
#292848=CARTESIAN_POINT('Ctrl Pts',(-5.00717796024875,44.2581956490076,
-11.0158070497208));
#292849=CARTESIAN_POINT('Ctrl Pts',(-3.53854538320666,44.1993871673535,
-11.5714554134028));
#292850=CARTESIAN_POINT('Ctrl Pts',(-0.448572613682795,44.074395143219,
-12.0950485754387));
#292851=CARTESIAN_POINT('Ctrl Pts',(1.14452620374632,44.0099529423683,-12.0491312232276));
#292852=CARTESIAN_POINT('Ctrl Pts',(4.19064476565769,43.8867348581954,-11.3503763214298));
#292853=CARTESIAN_POINT('Ctrl Pts',(5.61728165907052,43.8272168385556,-10.716282921232));
#292854=CARTESIAN_POINT('Ctrl Pts',(8.17321331619008,43.7010086192829,-8.92609404588821));
#292855=CARTESIAN_POINT('Ctrl Pts',(9.27208779579082,43.6395952508958,-7.77848261244147));
#292856=CARTESIAN_POINT('Ctrl Pts',(10.9594430391363,43.5166973288171,-5.13218112477692));
#292857=CARTESIAN_POINT('Ctrl Pts',(11.5345800225846,43.4529052377067,-3.66086990947338));
#292858=CARTESIAN_POINT('Ctrl Pts',(12.084772499407,43.3281439874099,-0.59664727805155));
#292859=CARTESIAN_POINT('Ctrl Pts',(12.0608636000957,43.269845613111,0.966055964610005));
#292860=CARTESIAN_POINT('Ctrl Pts',(11.4122909633861,43.1436650635112,4.0352056082348));
#292861=CARTESIAN_POINT('Ctrl Pts',(10.7785087786671,43.0790506090707,5.50883800602957));
#292862=CARTESIAN_POINT('Ctrl Pts',(8.99467956134047,42.9573198358976,8.09345482594726));
#292863=CARTESIAN_POINT('Ctrl Pts',(7.87369414154674,42.895469631438,9.18769182077571));
#292864=CARTESIAN_POINT('Ctrl Pts',(5.27082318036897,42.7697508400841,10.8926896879356));
#292865=CARTESIAN_POINT('Ctrl Pts',(3.81206688801357,42.7104513446453,11.4847923470224));
#292866=CARTESIAN_POINT('Ctrl Pts',(0.734944359608439,42.5859791236831,
12.080540589554));
#292867=CARTESIAN_POINT('Ctrl Pts',(-0.854930055522513,42.5216673526452,
12.0726431855703));
#292868=CARTESIAN_POINT('Ctrl Pts',(-3.91292811989484,42.3979687325035,
11.4490135627046));
#292869=CARTESIAN_POINT('Ctrl Pts',(-5.35408061776081,42.3390119364223,
10.850101759793));
#292870=CARTESIAN_POINT('Ctrl Pts',(-7.95796292680611,42.2126546460276,
9.11964158869093));
#292871=CARTESIAN_POINT('Ctrl Pts',(-9.08837248934058,42.1501687604152,
7.99363321081445));
#292872=CARTESIAN_POINT('Ctrl Pts',(-10.837335509043,42.0279192380799,5.38420353094394));
#292873=CARTESIAN_POINT('Ctrl Pts',(-11.445157596175,41.9643802601783,3.93009166695208));
#292874=CARTESIAN_POINT('Ctrl Pts',(-11.9191153548007,41.8691479620093,
1.60866192649058));
#292875=CARTESIAN_POINT('Ctrl Pts',(-12.,41.8371973529385,0.804432365335873));
#292876=CARTESIAN_POINT('Ctrl Pts',(-12.,41.806249999844,-1.30451205393456E-14));
#292877=CARTESIAN_POINT('Origin',(-8.79029313101884E-14,130.96875,0.));
#292878=CARTESIAN_POINT('',(-12.,38.431249999856,1.32817776064042E-14));
#292879=CARTESIAN_POINT('',(-12.,38.806249999856,-4.22293736248536E-14));
#292880=CARTESIAN_POINT('',(-12.0000000000001,130.96875,-1.46957615897682E-15));
#292881=CARTESIAN_POINT('Ctrl Pts',(-12.,38.431249999856,3.19189119579733E-15));
#292882=CARTESIAN_POINT('Ctrl Pts',(-12.,38.4627470412595,0.818720730010485));
#292883=CARTESIAN_POINT('Ctrl Pts',(-11.9162164291614,38.4952804862953,
1.63715836389978));
#292884=CARTESIAN_POINT('Ctrl Pts',(-11.4311628703194,38.5911059325512,
3.97040090002212));
#292885=CARTESIAN_POINT('Ctrl Pts',(-10.8184656394873,38.6546039678113,
5.42186448815198));
#292886=CARTESIAN_POINT('Ctrl Pts',(-9.06027034794767,38.7767526520915,
8.02567327944428));
#292887=CARTESIAN_POINT('Ctrl Pts',(-7.92510055901498,38.8394136877261,
9.14839305516659));
#292888=CARTESIAN_POINT('Ctrl Pts',(-5.31399423879045,38.9657918611721,
10.8697885374707));
#292889=CARTESIAN_POINT('Ctrl Pts',(-3.87065742753112,39.0246786179399,
11.4633714113522));
#292890=CARTESIAN_POINT('Ctrl Pts',(-0.810952705910088,39.1484462738174,
12.0756027183795));
#292891=CARTESIAN_POINT('Ctrl Pts',(0.778355614096445,39.2127351458265,
12.077747465541));
#292892=CARTESIAN_POINT('Ctrl Pts',(3.85344412602932,39.3371250890941,11.4710661599005));
#292893=CARTESIAN_POINT('Ctrl Pts',(5.31067786234046,39.3965134969212,10.8734102690138));
#292894=CARTESIAN_POINT('Ctrl Pts',(7.90739026213174,39.5222632701861,9.15863281694728));
#292895=CARTESIAN_POINT('Ctrl Pts',(9.02404753124986,39.5839503239638,8.06061484314743));
#292896=CARTESIAN_POINT('Ctrl Pts',(10.7979807496565,39.7057725186941,5.47040624510141));
#292897=CARTESIAN_POINT('Ctrl Pts',(11.4263198233243,39.7703840195296,3.99508204807151));
#292898=CARTESIAN_POINT('Ctrl Pts',(12.0641932735035,39.8965053178702,0.923996180099739));
#292899=CARTESIAN_POINT('Ctrl Pts',(12.0826383631988,39.9548022036435,-0.63905682404472));
#292900=CARTESIAN_POINT('Ctrl Pts',(11.5216766930976,40.07961240592,-3.7010527694457));
#292901=CARTESIAN_POINT('Ctrl Pts',(10.9416475861037,40.1433689492677,-5.16985042399155));
#292902=CARTESIAN_POINT('Ctrl Pts',(9.24510211101141,40.2661728281079,-7.81072130431282));
#292903=CARTESIAN_POINT('Ctrl Pts',(8.14154860183542,40.3277356340467,-8.95514693641855));
#292904=CARTESIAN_POINT('Ctrl Pts',(5.57849184352484,40.4539671305243,-10.7365079553709));
#292905=CARTESIAN_POINT('Ctrl Pts',(4.14969608175823,40.5133912672661,-11.365394034471));
#292906=CARTESIAN_POINT('Ctrl Pts',(1.10175261287963,40.6366831704764,-12.0530444689562));
#292907=CARTESIAN_POINT('Ctrl Pts',(-0.490925135201216,40.7011083387142,
-12.0933310903339));
#292908=CARTESIAN_POINT('Ctrl Pts',(-3.57905925800803,40.8260259880267,
-11.5590620019779));
#292909=CARTESIAN_POINT('Ctrl Pts',(-5.04624884960544,40.8848966761853,
-10.9980408831662));
#292910=CARTESIAN_POINT('Ctrl Pts',(-7.68342360485882,41.0104348637905,
-9.34785405875282));
#292911=CARTESIAN_POINT('Ctrl Pts',(-8.82858459186161,41.0732661061744,
-8.27482610799069));
#292912=CARTESIAN_POINT('Ctrl Pts',(-10.6674568021903,41.194469297909,-5.72180756870018));
#292913=CARTESIAN_POINT('Ctrl Pts',(-11.3315107912658,41.2590856390456,
-4.25796203440441));
#292914=CARTESIAN_POINT('Ctrl Pts',(-11.896660693456,41.360034065031,-1.81757981643005));
#292915=CARTESIAN_POINT('Ctrl Pts',(-12.,41.3962698521127,-0.909259118006817));
#292916=CARTESIAN_POINT('Ctrl Pts',(-12.,41.431249999844,-2.692290834716E-14));
#292917=CARTESIAN_POINT('Ctrl Pts',(-12.,41.806249999844,-1.51267887105178E-14));
#292918=CARTESIAN_POINT('Ctrl Pts',(-12.,41.7778205860545,-0.738982119407512));
#292919=CARTESIAN_POINT('Ctrl Pts',(-11.9317419193925,41.7485339036576,
-1.47806932044144));
#292920=CARTESIAN_POINT('Ctrl Pts',(-11.5035983705324,41.655184985873,-3.76542920943106));
#292921=CARTESIAN_POINT('Ctrl Pts',(-10.9063587082155,41.5906054825755,
-5.25002648732262));
#292922=CARTESIAN_POINT('Ctrl Pts',(-9.18897205810974,41.4682807599009,
-7.87167067732582));
#292923=CARTESIAN_POINT('Ctrl Pts',(-8.09694473926842,41.407449509464,-8.99111433965235));
#292924=CARTESIAN_POINT('Ctrl Pts',(-5.5353796252676,41.281531283893,-10.7613527298956));
#292925=CARTESIAN_POINT('Ctrl Pts',(-4.08688731425502,41.2215680644128,
-11.3905441816188));
#292926=CARTESIAN_POINT('Ctrl Pts',(-1.02372569601573,41.0976605741296,
-12.0590118479223));
#292927=CARTESIAN_POINT('Ctrl Pts',(0.561999477521797,41.0335166434399,
-12.0893292334744));
#292928=CARTESIAN_POINT('Ctrl Pts',(3.63088463893472,40.909377630972,-11.5415894732783));
#292929=CARTESIAN_POINT('Ctrl Pts',(5.08649399878036,40.8508126621997,-10.9781210699601));
#292930=CARTESIAN_POINT('Ctrl Pts',(7.73822477815293,40.7243250672075,-9.30803825386205));
#292931=CARTESIAN_POINT('Ctrl Pts',(8.90020859356382,40.6606132834455,-8.20398555482632));
#292932=CARTESIAN_POINT('Ctrl Pts',(10.7100801257288,40.5390470177957,-5.63210653469817));
#292933=CARTESIAN_POINT('Ctrl Pts',(11.3499486695057,40.475792761556,-4.19580812973791));
#292934=CARTESIAN_POINT('Ctrl Pts',(12.0440596481023,40.3504538888403,-1.16333298212337));
#292935=CARTESIAN_POINT('Ctrl Pts',(12.0933754581578,40.2918840575548,0.403761734034306));
#292936=CARTESIAN_POINT('Ctrl Pts',(11.5875293687639,40.1665629969046,3.49694485298569));
#292937=CARTESIAN_POINT('Ctrl Pts',(11.0265311623774,40.1020529092557,4.99151333281217));
#292938=CARTESIAN_POINT('Ctrl Pts',(9.37508065496285,39.9791844834636,7.64871426241236));
#292939=CARTESIAN_POINT('Ctrl Pts',(8.31156816845547,39.9191889447782,8.79277523687751));
#292940=CARTESIAN_POINT('Ctrl Pts',(5.79091324092277,39.7930925420681,10.6268155293752));
#292941=CARTESIAN_POINT('Ctrl Pts',(4.35271268300412,39.7323209264614,11.2923734401967));
#292942=CARTESIAN_POINT('Ctrl Pts',(1.30408528138926,39.6090013575907,12.0314479104659));
#292943=CARTESIAN_POINT('Ctrl Pts',(-0.276747876045521,39.5450553131092,
12.0987463589307));
#292944=CARTESIAN_POINT('Ctrl Pts',(-3.35515052035818,39.4205313103708,
11.6248643914831));
#292945=CARTESIAN_POINT('Ctrl Pts',(-4.82464042947219,39.3621804905949,
11.095824236271));
#292946=CARTESIAN_POINT('Ctrl Pts',(-7.51915453353781,39.2357377403919,
9.48651371884892));
#292947=CARTESIAN_POINT('Ctrl Pts',(-8.7094080333007,39.1711199584178,8.40703084629784));
#292948=CARTESIAN_POINT('Ctrl Pts',(-10.5773933932437,39.0498235777697,
5.87654963587647));
#292949=CARTESIAN_POINT('Ctrl Pts',(-11.2488153785026,38.9871702481793,
4.45868949119449));
#292950=CARTESIAN_POINT('Ctrl Pts',(-11.8766392410368,38.8841629732154,
1.98515443060089));
#292951=CARTESIAN_POINT('Ctrl Pts',(-12.,38.8444686416769,0.993439159275016));
#292952=CARTESIAN_POINT('Ctrl Pts',(-12.,38.806249999856,1.66533453693773E-14));
#292953=CARTESIAN_POINT('Origin',(-8.79029313101884E-14,130.96875,0.));
#292954=CARTESIAN_POINT('',(-12.,35.431249999868,-5.15968803951284E-14));
#292955=CARTESIAN_POINT('',(-12.,35.806249999868,-1.33406439522195E-13));
#292956=CARTESIAN_POINT('',(-12.0000000000001,130.96875,-1.46957615897682E-15));
#292957=CARTESIAN_POINT('Ctrl Pts',(-12.,35.431249999868,-1.04360964314765E-13));
#292958=CARTESIAN_POINT('Ctrl Pts',(-12.,35.4700381716479,1.00824327937616));
#292959=CARTESIAN_POINT('Ctrl Pts',(-11.8729349682393,35.51034198472,2.01459756389213));
#292960=CARTESIAN_POINT('Ctrl Pts',(-11.2324217201602,35.6139509957666,
4.49965086560238));
#292961=CARTESIAN_POINT('Ctrl Pts',(-10.5560913389816,35.6764253426343,
5.91459768290572));
#292962=CARTESIAN_POINT('Ctrl Pts',(-8.67974020180297,35.7978165013443,
8.43755061085998));
#292963=CARTESIAN_POINT('Ctrl Pts',(-7.48615700668944,35.8624349960771,
9.51248052848435));
#292964=CARTESIAN_POINT('Ctrl Pts',(-4.78646793873384,35.9888231360038,
11.1123714934671));
#292965=CARTESIAN_POINT('Ctrl Pts',(-3.31497518795321,36.0471564367163,
11.6364104546645));
#292966=CARTESIAN_POINT('Ctrl Pts',(-0.235277726382621,36.171732815913,
12.099555273878));
#292967=CARTESIAN_POINT('Ctrl Pts',(1.34477456587885,36.2356472737348,12.0268993925935));
#292968=CARTESIAN_POINT('Ctrl Pts',(4.39121111942935,36.3588782209397,11.277574042516));
#292969=CARTESIAN_POINT('Ctrl Pts',(5.82788906599174,36.4197807200876,10.6067061703878));
#292970=CARTESIAN_POINT('Ctrl Pts',(8.34253553350199,36.5459016694114,8.76336354866154));
#292971=CARTESIAN_POINT('Ctrl Pts',(9.40187406344104,36.6057888893765,7.61571572231948));
#292972=CARTESIAN_POINT('Ctrl Pts',(11.0436327369964,36.7287334334172,4.9533871395502));
#292973=CARTESIAN_POINT('Ctrl Pts',(11.5993072771692,36.7932304407386,3.45742890019772));
#292974=CARTESIAN_POINT('Ctrl Pts',(12.0947375415577,36.9184829563752,0.362643204550438));
#292975=CARTESIAN_POINT('Ctrl Pts',(12.0400468780078,36.9770973226748,-1.20474787555495));
#292976=CARTESIAN_POINT('Ctrl Pts',(11.335412173293,37.1024718528658,-4.2347305225582));
#292977=CARTESIAN_POINT('Ctrl Pts',(10.6908673865189,37.1656814449742,-5.66834854358663));
#292978=CARTESIAN_POINT('Ctrl Pts',(8.87206294573137,37.2871439038344,-8.23462677611558));
#292979=CARTESIAN_POINT('Ctrl Pts',(7.70541453987611,37.3510495185937,-9.33540665419294));
#292980=CARTESIAN_POINT('Ctrl Pts',(5.04662834355365,37.4775546945405,-10.9965179503444));
#292981=CARTESIAN_POINT('Ctrl Pts',(3.58888934073206,37.5360763764805,-11.5547299900151));
#292982=CARTESIAN_POINT('Ctrl Pts',(0.518483215847364,37.6602769132132,
-12.0912010592991));
#292983=CARTESIAN_POINT('Ctrl Pts',(-1.0665498363905,37.7243928470083,-12.0552273362314));
#292984=CARTESIAN_POINT('Ctrl Pts',(-4.12755437962205,37.8482130817744,
-11.375976411187));
#292985=CARTESIAN_POINT('Ctrl Pts',(-5.57449640280557,37.9082892707063,
-10.7412540867963));
#292986=CARTESIAN_POINT('Ctrl Pts',(-8.1298661695661,38.0342357156939,-8.96130166659882));
#292987=CARTESIAN_POINT('Ctrl Pts',(-9.21756461347896,38.0949293589744,
-7.83810797722948));
#292988=CARTESIAN_POINT('Ctrl Pts',(-10.9249731035212,38.2173392686393,
-5.21100737200903));
#292989=CARTESIAN_POINT('Ctrl Pts',(-11.5167262601255,38.2819104729188,
-3.72484314150043));
#292990=CARTESIAN_POINT('Ctrl Pts',(-11.9342867633289,38.3746336494357,
-1.45030986554002));
#292991=CARTESIAN_POINT('Ctrl Pts',(-12.,38.4033555800282,-0.725075713364724));
#292992=CARTESIAN_POINT('Ctrl Pts',(-12.,38.431249999856,1.13797860024079E-14));
#292993=CARTESIAN_POINT('Ctrl Pts',(-12.,38.806249999856,1.95676808090184E-14));
#292994=CARTESIAN_POINT('Ctrl Pts',(-12.,38.7848368006228,-0.556605615219962));
#292995=CARTESIAN_POINT('Ctrl Pts',(-11.9612756878353,38.7629201691543,
-1.11371494261193));
#292996=CARTESIAN_POINT('Ctrl Pts',(-11.6644552582536,38.6778210346364,
-3.22930293378464));
#292997=CARTESIAN_POINT('Ctrl Pts',(-11.1394629688195,38.6134136771892,
-4.73290011993798));
#292998=CARTESIAN_POINT('Ctrl Pts',(-9.55360537494578,38.4900489314371,
-7.42431460952982));
#292999=CARTESIAN_POINT('Ctrl Pts',(-8.5182607742844,38.4307148678992,-8.59250029243608));
#293000=CARTESIAN_POINT('Ctrl Pts',(-6.03825498759269,38.3044605264228,
-10.4891319933311));
#293001=CARTESIAN_POINT('Ctrl Pts',(-4.61041277056975,38.242745113982,-11.1904554442826));
#293002=CARTESIAN_POINT('Ctrl Pts',(-1.57687408184143,38.1200358963687,
-11.9982836169922));
#293003=CARTESIAN_POINT('Ctrl Pts',(-0.00162053623311592,38.0563155519266,
-12.1014523639863));
#293004=CARTESIAN_POINT('Ctrl Pts',(3.08504138152381,37.9314574545594,-11.6996554205751));
#293005=CARTESIAN_POINT('Ctrl Pts',(4.56790597917435,37.8731585374633,-11.20417964339));
#293006=CARTESIAN_POINT('Ctrl Pts',(7.29667881694916,37.7470971393136,-9.65806131879168));
#293007=CARTESIAN_POINT('Ctrl Pts',(8.50889043244637,37.6824893721698,-8.60922240837434));
#293008=CARTESIAN_POINT('Ctrl Pts',(10.4324769840663,37.560577044529,-6.12936387313183));
#293009=CARTESIAN_POINT('Ctrl Pts',(11.1365970977192,37.4990487018181,-4.7309910451774));
#293010=CARTESIAN_POINT('Ctrl Pts',(11.9761702450188,37.373268480201,-1.73430718515646));
#293011=CARTESIAN_POINT('Ctrl Pts',(12.0999915756348,37.3137878947727,-0.163447609588439));
#293012=CARTESIAN_POINT('Ctrl Pts',(11.7376918656824,37.1894806492918,2.9500238740173));
#293013=CARTESIAN_POINT('Ctrl Pts',(11.2501446104752,37.1252153578106,4.46209488687447));
#293014=CARTESIAN_POINT('Ctrl Pts',(9.73263915500905,37.0013800721998,7.18794934595158));
#293015=CARTESIAN_POINT('Ctrl Pts',(8.72646017235344,36.9425590237925,8.38091488005002));
#293016=CARTESIAN_POINT('Ctrl Pts',(6.28879684496449,36.8161605437619,10.341888226191));
#293017=CARTESIAN_POINT('Ctrl Pts',(4.87189218036381,36.7533221782981,11.0800661200621));
#293018=CARTESIAN_POINT('Ctrl Pts',(1.85470485672127,36.6312743872966,11.9580191975185));
#293019=CARTESIAN_POINT('Ctrl Pts',(0.285969466989008,36.5678177077983,
12.097608011535));
#293020=CARTESIAN_POINT('Ctrl Pts',(-2.80808018452431,36.4426607703231,
11.7695039807635));
#293021=CARTESIAN_POINT('Ctrl Pts',(-4.30444491654658,36.3842567180682,
11.3083293063412));
#293022=CARTESIAN_POINT('Ctrl Pts',(-7.06708425206928,36.2586202861418,
9.82669765417226));
#293023=CARTESIAN_POINT('Ctrl Pts',(-8.30078803454533,36.1940580917055,
8.80935689303109));
#293024=CARTESIAN_POINT('Ctrl Pts',(-10.2798691440691,36.0715647349362,
6.38144285677968));
#293025=CARTESIAN_POINT('Ctrl Pts',(-11.016825756956,36.0110036067955,5.00282570486589));
#293026=CARTESIAN_POINT('Ctrl Pts',(-11.8224444004248,35.8999944688486,
2.37906263930499));
#293027=CARTESIAN_POINT('Ctrl Pts',(-12.0000000000001,35.8521007994926,
1.19182623088897));
#293028=CARTESIAN_POINT('Ctrl Pts',(-12.,35.806249999868,-2.27873275804313E-13));
#293029=CARTESIAN_POINT('Origin',(-8.79029313101884E-14,130.96875,0.));
#293030=CARTESIAN_POINT('',(-12.,32.43124999988,-1.15434704311075E-13));
#293031=CARTESIAN_POINT('',(-12.,32.80624999988,-5.31445805606718E-15));
#293032=CARTESIAN_POINT('',(-12.0000000000001,130.96875,-1.46957615897682E-15));
#293033=CARTESIAN_POINT('Ctrl Pts',(-12.,32.43124999988,-2.18158824338843E-13));
#293034=CARTESIAN_POINT('Ctrl Pts',(-12.0000000000001,32.4776762727195,
1.20678483746527));
#293035=CARTESIAN_POINT('Ctrl Pts',(-11.8179589645538,32.5261907975428,
2.40870209300642));
#293036=CARTESIAN_POINT('Ctrl Pts',(-10.9982644188703,32.6377969953442,
5.0434113412201));
#293037=CARTESIAN_POINT('Ctrl Pts',(-10.2563850742601,32.698227446797,6.41905095562799));
#293038=CARTESIAN_POINT('Ctrl Pts',(-8.26901764732399,32.8208045715522,
8.83908300931383));
#293039=CARTESIAN_POINT('Ctrl Pts',(-7.03214309924002,32.8853568146657,
9.85164104839903));
#293040=CARTESIAN_POINT('Ctrl Pts',(-4.26447583888615,33.0109258659356,
11.3235184271393));
#293041=CARTESIAN_POINT('Ctrl Pts',(-2.76608200565986,33.0693596323568,
11.7794987318951));
#293042=CARTESIAN_POINT('Ctrl Pts',(0.328992884834674,33.1945580416199,
12.0964443517389));
#293043=CARTESIAN_POINT('Ctrl Pts',(1.89667010069928,33.2579719170862,11.9513643438712));
#293044=CARTESIAN_POINT('Ctrl Pts',(4.91129963068495,33.3799162431608,11.0628074664535));
#293045=CARTESIAN_POINT('Ctrl Pts',(6.3265156265557,33.4429385666294,10.3190227205775));
#293046=CARTESIAN_POINT('Ctrl Pts',(8.75769482069915,33.5693572706409,8.34827414059132));
#293047=CARTESIAN_POINT('Ctrl Pts',(9.75942334147266,33.6281153813829,7.15154516538066));
#293048=CARTESIAN_POINT('Ctrl Pts',(11.2664628787054,33.7520185502841,4.42052559388299));
#293049=CARTESIAN_POINT('Ctrl Pts',(11.7482850488903,33.816258979221,2.90724065456717));
#293050=CARTESIAN_POINT('Ctrl Pts',(12.0994052463512,33.9404810327821,-0.207648830224786));
#293051=CARTESIAN_POINT('Ctrl Pts',(11.9697396871303,34.0000594305946,-1.77877097455616));
#293052=CARTESIAN_POINT('Ctrl Pts',(11.1187907608595,34.125870314321,-4.77255563778874));
#293053=CARTESIAN_POINT('Ctrl Pts',(10.4096637930931,34.1872405346318,-6.16792808916501));
#293054=CARTESIAN_POINT('Ctrl Pts',(8.47759190364955,34.3092439253597,-8.63993753467918));
#293055=CARTESIAN_POINT('Ctrl Pts',(7.26206580242804,34.3738470647927,-9.68401981234569));
#293056=CARTESIAN_POINT('Ctrl Pts',(4.52809320359843,34.499846399196,-11.2203709724452));
#293057=CARTESIAN_POINT('Ctrl Pts',(3.04317416810518,34.5581510189295,-11.7106554039441));
#293058=CARTESIAN_POINT('Ctrl Pts',(-0.0446744412204195,34.6830571189791,
-12.1012993876648));
#293059=CARTESIAN_POINT('Ctrl Pts',(-1.61899415642968,34.746739689188,-11.9926018972619));
#293060=CARTESIAN_POINT('Ctrl Pts',(-4.65011840450887,34.8693512406255,
-11.1741502096888));
#293061=CARTESIAN_POINT('Ctrl Pts',(-6.07632860852273,34.9312263422972,
-10.4672682898571));
#293062=CARTESIAN_POINT('Ctrl Pts',(-8.54997851100817,35.0575036507789,
-8.56092250731231));
#293063=CARTESIAN_POINT('Ctrl Pts',(-9.5809337182492,35.1167493351784,-7.38899455347827));
#293064=CARTESIAN_POINT('Ctrl Pts',(-11.1565315742162,35.2401877322821,
-4.69233201097822));
#293065=CARTESIAN_POINT('Ctrl Pts',(-11.675897777898,35.3045760268348,-3.18740231154562));
#293066=CARTESIAN_POINT('Ctrl Pts',(-11.9632185252926,35.3890323308912,
-1.08543714878296));
#293067=CARTESIAN_POINT('Ctrl Pts',(-12.,35.4103808839011,-0.542462945650476));
#293068=CARTESIAN_POINT('Ctrl Pts',(-12.,35.431249999868,-1.13103970633688E-13));
#293069=CARTESIAN_POINT('Ctrl Pts',(-12.,35.806249999868,-2.04627981226224E-13));
#293070=CARTESIAN_POINT('Ctrl Pts',(-12.,35.7920639646029,-0.368745781529345));
#293071=CARTESIAN_POINT('Ctrl Pts',(-11.9830038542012,35.7776492037367,
-0.737914576754738));
#293072=CARTESIAN_POINT('Ctrl Pts',(-11.8041633160057,35.7011049692098,
-2.66946411788623));
#293073=CARTESIAN_POINT('Ctrl Pts',(-11.354105989905,35.6370174959843,-4.18909421482921));
#293074=CARTESIAN_POINT('Ctrl Pts',(-9.90522339156164,35.5127571124111,
-6.94829540786313));
#293075=CARTESIAN_POINT('Ctrl Pts',(-8.92815820661399,35.4542744622871,
-8.1657947673545));
#293076=CARTESIAN_POINT('Ctrl Pts',(-6.53302381849094,35.3277523578375,
-10.1905036328583));
#293077=CARTESIAN_POINT('Ctrl Pts',(-5.12726325995961,35.2636521554673,
-10.9652742067382));
#293078=CARTESIAN_POINT('Ctrl Pts',(-2.12709803906788,35.1422929229861,
-11.912123170417));
#293079=CARTESIAN_POINT('Ctrl Pts',(-0.565577341076917,35.0791280839252,
-12.0873085786455));
#293080=CARTESIAN_POINT('Ctrl Pts',(2.52752654738964,34.9540094033686,-11.8323663023729));
#293081=CARTESIAN_POINT('Ctrl Pts',(4.03027763949432,34.8956068183643,-11.4083384908807));
#293082=CARTESIAN_POINT('Ctrl Pts',(6.81102621451258,34.7712034870444,-10.0034944167991));
#293083=CARTESIAN_POINT('Ctrl Pts',(8.05881998447991,34.7071892601766,-9.02859354763777));
#293084=CARTESIAN_POINT('Ctrl Pts',(10.1082156653494,34.5836740271163,-6.65448064341902));
#293085=CARTESIAN_POINT('Ctrl Pts',(10.8902599029851,34.5231833580987,-5.27829725337419));
#293086=CARTESIAN_POINT('Ctrl Pts',(11.8745727165592,34.3971432211835,-2.32188603377452));
#293087=CARTESIAN_POINT('Ctrl Pts',(12.0747742808167,34.3368927320492,-0.772218541801659));
#293088=CARTESIAN_POINT('Ctrl Pts',(11.873227379025,34.214197585593,2.35158047736658));
#293089=CARTESIAN_POINT('Ctrl Pts',(11.4600717986303,34.1496609674394,3.8948755610043));
#293090=CARTESIAN_POINT('Ctrl Pts',(10.0721373165819,34.024189754806,6.70535377430503));
#293091=CARTESIAN_POINT('Ctrl Pts',(9.12121355161991,33.9657071760561,7.95066998817524));
#293092=CARTESIAN_POINT('Ctrl Pts',(6.79299867096633,33.8404511283386,10.0142372207861));
#293093=CARTESIAN_POINT('Ctrl Pts',(5.43608279131537,33.7770998455958,10.8110619628864));
#293094=CARTESIAN_POINT('Ctrl Pts',(2.46898927635769,33.6553051667091,11.8497082510787));
#293095=CARTESIAN_POINT('Ctrl Pts',(0.884112711395966,33.5920131103,12.0718827108435));
#293096=CARTESIAN_POINT('Ctrl Pts',(-2.2418265845094,33.4655662096119,11.8897137412496));
#293097=CARTESIAN_POINT('Ctrl Pts',(-3.75366399717397,33.4068913516675,
11.5022228938451));
#293098=CARTESIAN_POINT('Ctrl Pts',(-6.57030474952821,33.2828925745752,
10.1637951032527));
#293099=CARTESIAN_POINT('Ctrl Pts',(-7.84394492687112,33.2186892972338,
9.21651758465373));
#293100=CARTESIAN_POINT('Ctrl Pts',(-9.94707858033792,33.0945911471668,
6.89185204586521));
#293101=CARTESIAN_POINT('Ctrl Pts',(-10.75907758468,33.0348655046159,5.53933429402285));
#293102=CARTESIAN_POINT('Ctrl Pts',(-11.7598464659617,32.915546560012,2.76297779607306));
#293103=CARTESIAN_POINT('Ctrl Pts',(-12.,32.8595735697097,1.38607024889398));
#293104=CARTESIAN_POINT('Ctrl Pts',(-12.,32.80624999988,3.88578058618805E-15));
#293105=CARTESIAN_POINT('Origin',(-8.79029313101884E-14,130.96875,0.));
#293106=CARTESIAN_POINT('',(-12.,29.431249999892,-5.31060898192282E-14));
#293107=CARTESIAN_POINT('',(-12.,29.806249999892,-2.57148061335544E-14));
#293108=CARTESIAN_POINT('',(-12.0000000000001,130.96875,-1.46957615897682E-15));
#293109=CARTESIAN_POINT('Ctrl Pts',(-12.,29.431249999892,-9.32587340685131E-14));
#293110=CARTESIAN_POINT('Ctrl Pts',(-12.,29.4851488241481,1.40102316837458));
#293111=CARTESIAN_POINT('Ctrl Pts',(-11.7546358261363,29.541753991599,2.79267022061044));
#293112=CARTESIAN_POINT('Ctrl Pts',(-10.7438889970809,29.6610106605539,
5.56416592000471));
#293113=CARTESIAN_POINT('Ctrl Pts',(-9.93826035902713,29.7200942929683,
6.90087635712038));
#293114=CARTESIAN_POINT('Ctrl Pts',(-7.8444929696234,29.8436744278595,9.2166465168711));
#293115=CARTESIAN_POINT('Ctrl Pts',(-6.56786190030818,29.9080228891066,
10.1659136415296));
#293116=CARTESIAN_POINT('Ctrl Pts',(-3.73633664274598,30.0326315459472,
11.5095052889258));
#293117=CARTESIAN_POINT('Ctrl Pts',(-2.21157294657299,30.0917899949855,
11.8969668898356));
#293118=CARTESIAN_POINT('Ctrl Pts',(0.895057612379632,30.2174558408568,
12.0668979865983));
#293119=CARTESIAN_POINT('Ctrl Pts',(2.4472716297175,30.2795885355239,11.8499569001875));
#293120=CARTESIAN_POINT('Ctrl Pts',(5.41749433871223,30.4011637263426,10.8248489145821));
#293121=CARTESIAN_POINT('Ctrl Pts',(6.80210151923264,30.4657813504751,10.0128775729825));
#293122=CARTESIAN_POINT('Ctrl Pts',(9.14338880188783,30.5920593815452,7.92431988258037));
#293123=CARTESIAN_POINT('Ctrl Pts',(10.0883236951527,30.6503681744823,6.67998170676279));
#293124=CARTESIAN_POINT('Ctrl Pts',(11.4610834689155,30.7750453012285,3.88521406347696));
#293125=CARTESIAN_POINT('Ctrl Pts',(11.8697061866883,30.8388952901868,2.35829411145753));
#293126=CARTESIAN_POINT('Ctrl Pts',(12.0778585345691,30.9619488763262,-0.772675797213721));
#293127=CARTESIAN_POINT('Ctrl Pts',(11.8728581235085,31.0231198087666,-2.34671393167774));
#293128=CARTESIAN_POINT('Ctrl Pts',(10.8756316476451,31.1492881933354,-5.30226286314234));
#293129=CARTESIAN_POINT('Ctrl Pts',(10.1022106565283,31.2089715090149,-6.65872709649208));
#293130=CARTESIAN_POINT('Ctrl Pts',(8.06197802432647,31.3320641370475,-9.02767772633765));
#293131=CARTESIAN_POINT('Ctrl Pts',(6.8051221704812,31.3965330449699,-10.0092289052083));
#293132=CARTESIAN_POINT('Ctrl Pts',(4.00556095415405,31.5216473949094,-11.4180839686849));
#293133=CARTESIAN_POINT('Ctrl Pts',(2.49413853287218,31.5803599769125,-11.840455574618));
#293134=CARTESIAN_POINT('Ctrl Pts',(-0.606971283075425,31.7058025040382,
-12.0852335809304));
#293135=CARTESIAN_POINT('Ctrl Pts',(-2.16735607895474,31.7689213949195,
-11.9047965025742));
#293136=CARTESIAN_POINT('Ctrl Pts',(-5.16492051548911,31.8901754234635,
-10.9477503712494));
#293137=CARTESIAN_POINT('Ctrl Pts',(-6.56899609687767,31.9544757824724,
-10.1675305909724));
#293138=CARTESIAN_POINT('Ctrl Pts',(-8.95775373601538,32.0810145793702,
-8.13334282430559));
#293139=CARTESIAN_POINT('Ctrl Pts',(-9.93046914074174,32.1394614895692,
-6.91219539265034));
#293140=CARTESIAN_POINT('Ctrl Pts',(-11.3690686936999,32.2637815229155,
-4.14810252474221));
#293141=CARTESIAN_POINT('Ctrl Pts',(-11.8135187518015,32.3278393648193,
-2.6274207399871));
#293142=CARTESIAN_POINT('Ctrl Pts',(-11.9842718072799,32.4037445737492,
-0.709853976657044));
#293143=CARTESIAN_POINT('Ctrl Pts',(-12.,32.4176033869892,-0.354724265208347));
#293144=CARTESIAN_POINT('Ctrl Pts',(-12.,32.43124999988,-2.08791317568569E-13));
#293145=CARTESIAN_POINT('Ctrl Pts',(-12.,32.80624999988,4.5102810375397E-16));
#293146=CARTESIAN_POINT('Ctrl Pts',(-12.,32.8000424641438,-0.161356050061035));
#293147=CARTESIAN_POINT('Ctrl Pts',(-11.9967455546346,32.7937895901545,
-0.322833170037546));
#293148=CARTESIAN_POINT('Ctrl Pts',(-11.9262084743953,32.7257288838371,
-2.06905540512378));
#293149=CARTESIAN_POINT('Ctrl Pts',(-11.5486544106732,32.6611338492227,
-3.62543657544074));
#293150=CARTESIAN_POINT('Ctrl Pts',(-10.2255683019167,32.535225413725,-6.4683502881123));
#293151=CARTESIAN_POINT('Ctrl Pts',(-9.30563617959406,32.4769061387655,
-7.73349450970906));
#293152=CARTESIAN_POINT('Ctrl Pts',(-7.02632893219277,32.3519325782973,
-9.85249633764293));
#293153=CARTESIAN_POINT('Ctrl Pts',(-5.685223823736,32.2883058052959,-10.6826694433699));
#293154=CARTESIAN_POINT('Ctrl Pts',(-2.74576725643883,32.1658365822708,
-11.7877250338585));
#293155=CARTESIAN_POINT('Ctrl Pts',(-1.17364211102602,32.1037248205395,
-12.0462668531426));
#293156=CARTESIAN_POINT('Ctrl Pts',(1.94890553891517,31.9774151148127,-11.941229191595));
#293157=CARTESIAN_POINT('Ctrl Pts',(3.46985003208625,31.9182901507538,-11.5910027489076));
#293158=CARTESIAN_POINT('Ctrl Pts',(6.32201899278502,31.7947470883891,-10.3206420147937));
#293159=CARTESIAN_POINT('Ctrl Pts',(7.62129871611257,31.7303877946302,-9.40209248895725));
#293160=CARTESIAN_POINT('Ctrl Pts',(9.77828338826287,31.6057376318048,-7.12832969617556));
#293161=CARTESIAN_POINT('Ctrl Pts',(10.6202783134745,31.5466204539994,-5.79978884346416));
#293162=CARTESIAN_POINT('Ctrl Pts',(11.7474348874117,31.4209711163855,-2.8999486463113));
#293163=CARTESIAN_POINT('Ctrl Pts',(12.0237302200211,31.3587494337806,-1.35693759319928));
#293164=CARTESIAN_POINT('Ctrl Pts',(11.972474690382,31.2372225916453,1.78532564615453));
#293165=CARTESIAN_POINT('Ctrl Pts',(11.63090385625,31.1726044433631,3.35399928337155));
#293166=CARTESIAN_POINT('Ctrl Pts',(10.3731262802374,31.0462969511876,6.22850593462641));
#293167=CARTESIAN_POINT('Ctrl Pts',(9.48407280831626,30.9879829679234,7.51321676272817));
#293168=CARTESIAN_POINT('Ctrl Pts',(7.2541253814875,30.8633321832837,9.68658109167525));
#293169=CARTESIAN_POINT('Ctrl Pts',(5.92950656980374,30.7994648455449,10.5495634275673));
#293170=CARTESIAN_POINT('Ctrl Pts',(3.01830377911047,30.6763639699012,11.7200733600513));
#293171=CARTESIAN_POINT('Ctrl Pts',(1.45894185072004,30.6152654374406,12.0142368666767));
#293172=CARTESIAN_POINT('Ctrl Pts',(-1.65980483796559,30.4891094838263,
11.9849352026845));
#293173=CARTESIAN_POINT('Ctrl Pts',(-3.18954833416544,30.4293734498415,
11.6713473717854));
#293174=CARTESIAN_POINT('Ctrl Pts',(-6.07557898484373,30.3063197608035,
10.4681755582203));
#293175=CARTESIAN_POINT('Ctrl Pts',(-7.39932882970642,30.2418431144289,
9.57837059156762));
#293176=CARTESIAN_POINT('Ctrl Pts',(-9.60829173472751,30.1166917984454,
7.35507195419466));
#293177=CARTESIAN_POINT('Ctrl Pts',(-10.4792481496153,30.0580065703022,
6.04993124133885));
#293178=CARTESIAN_POINT('Ctrl Pts',(-11.6756085493199,29.9325817407516,
3.17841249757036));
#293179=CARTESIAN_POINT('Ctrl Pts',(-11.9890112143639,29.869438496906,1.63892450753172));
#293180=CARTESIAN_POINT('Ctrl Pts',(-11.9999054182355,29.8083678250883,
0.0550191180779561));
#293181=CARTESIAN_POINT('Ctrl Pts',(-12.,29.807308236395,0.027507350646264));
#293182=CARTESIAN_POINT('Ctrl Pts',(-12.,29.806249999892,-1.04101115714572E-13));
#293183=CARTESIAN_POINT('Origin',(-8.79029313101884E-14,130.96875,0.));
#293184=CARTESIAN_POINT('',(-12.,26.4312499994205,-6.28404526952038E-9));
#293185=CARTESIAN_POINT('',(-12.,26.806249999904,3.01779842624183E-14));
#293186=CARTESIAN_POINT('',(-12.0000000000001,130.96875,-1.46957615897682E-15));
#293187=CARTESIAN_POINT('Ctrl Pts',(-12.,26.4312499994205,-1.25681301308442E-8));
#293188=CARTESIAN_POINT('Ctrl Pts',(-12.0000000000063,26.4314790020448,
0.005952584484202));
#293189=CARTESIAN_POINT('Ctrl Pts',(-11.9999955708361,26.4317080680303,
0.0119053893945655));
#293190=CARTESIAN_POINT('Ctrl Pts',(-11.9976172228562,26.4932197505189,
1.61004119241557));
#293191=CARTESIAN_POINT('Ctrl Pts',(-11.678391503657,26.5578345097249,3.18588710337945));
#293192=CARTESIAN_POINT('Ctrl Pts',(-10.4610723416985,26.6843687439975,
6.0794333281055));
#293193=CARTESIAN_POINT('Ctrl Pts',(-9.59098918588322,26.7427574557944,
7.37607697614277));
#293194=CARTESIAN_POINT('Ctrl Pts',(-7.39166162622063,26.8671898824307,
9.58240212898549));
#293195=CARTESIAN_POINT('Ctrl Pts',(-6.07752317006222,26.931188229299,10.4653194827716));
#293196=CARTESIAN_POINT('Ctrl Pts',(-3.18402088459822,27.0546573220819,
11.6756787271243));
#293197=CARTESIAN_POINT('Ctrl Pts',(-1.63251893587116,27.1152132217633,
11.9914301900934));
#293198=CARTESIAN_POINT('Ctrl Pts',(1.4836990924161,27.2412668889159,12.0081169930264));
#293199=CARTESIAN_POINT('Ctrl Pts',(3.01871679408634,27.3014552565358,11.716802448988));
#293200=CARTESIAN_POINT('Ctrl Pts',(5.92481138151768,27.4241919260214,10.5545796385704));
#293201=CARTESIAN_POINT('Ctrl Pts',(7.26306823652372,27.488722584878,9.6824701750163));
#293202=CARTESIAN_POINT('Ctrl Pts',(9.50314964785391,27.6141585383666,7.49003106375069));
#293203=CARTESIAN_POINT('Ctrl Pts',(10.3914615484667,27.6726602946857,6.1990252522971));
#293204=CARTESIAN_POINT('Ctrl Pts',(11.6293109061408,27.7979363907583,3.34485320306925));
#293205=CARTESIAN_POINT('Ctrl Pts',(11.9649950199946,27.8612649924479,1.80778678146149));
#293206=CARTESIAN_POINT('Ctrl Pts',(12.0303715249327,27.9830059032825,-1.33545268582758));
#293207=CARTESIAN_POINT('Ctrl Pts',(11.7489204696593,28.0463959052348,-2.91147312204396));
#293208=CARTESIAN_POINT('Ctrl Pts',(10.6039167708586,28.172852637454,-5.82650150959838));
#293209=CARTESIAN_POINT('Ctrl Pts',(9.76567299451591,28.2314997836282,-7.14302793176961));
#293210=CARTESIAN_POINT('Ctrl Pts',(7.61820968020575,28.3555321834124,-9.40391356928499));
#293211=CARTESIAN_POINT('Ctrl Pts',(6.32224180580404,28.4197217744015,-10.3198840220338));
#293212=CARTESIAN_POINT('Ctrl Pts',(3.45901026767688,28.5437752099896,-11.5964839511652));
#293213=CARTESIAN_POINT('Ctrl Pts',(1.92071620599176,28.6035553972944,-11.9479715018053));
#293214=CARTESIAN_POINT('Ctrl Pts',(-1.1909499873322,28.7294249388549,-12.040934522847));
#293215=CARTESIAN_POINT('Ctrl Pts',(-2.7346005176524,28.7904977009883,-11.7866081716702));
#293216=CARTESIAN_POINT('Ctrl Pts',(-5.67314045061089,28.9126761759063,
-10.6925193683012));
#293217=CARTESIAN_POINT('Ctrl Pts',(-7.03485626457987,28.9772678956048,
-9.85013026499296));
#293218=CARTESIAN_POINT('Ctrl Pts',(-9.32579612279864,29.1031433497616,
-7.70920706652483));
#293219=CARTESIAN_POINT('Ctrl Pts',(-10.2425208237552,29.1614697147043,
-6.4415146649703));
#293220=CARTESIAN_POINT('Ctrl Pts',(-11.5481671297799,29.2864669548987,
-3.61661964098504));
#293221=CARTESIAN_POINT('Ctrl Pts',(-11.9204183427465,29.3500733461147,
-2.08421384703015));
#293222=CARTESIAN_POINT('Ctrl Pts',(-11.9961974439967,29.4177771295152,
-0.348972550675605));
#293223=CARTESIAN_POINT('Ctrl Pts',(-12.,29.4245400561049,-0.174415431763315));
#293224=CARTESIAN_POINT('Ctrl Pts',(-12.,29.431249999892,-1.0842021724855E-13));
#293225=CARTESIAN_POINT('Ctrl Pts',(-12.,29.806249999892,-1.08801856413265E-13));
#293226=CARTESIAN_POINT('Ctrl Pts',(-12.,29.7461635566442,-1.56186151103106));
#293227=CARTESIAN_POINT('Ctrl Pts',(-11.6950686578715,29.6828245025684,
-3.1091918087787));
#293228=CARTESIAN_POINT('Ctrl Pts',(-10.5148572656756,29.5574045423193,
-5.98583111260254));
#293229=CARTESIAN_POINT('Ctrl Pts',(-9.65660561959846,29.4989392255624,
-7.28988416406018));
#293230=CARTESIAN_POINT('Ctrl Pts',(-7.47648354397054,29.3746505852464,
-9.51659596253284));
#293231=CARTESIAN_POINT('Ctrl Pts',(-6.16901356837322,29.3105769874857,
-10.4118566312308));
#293232=CARTESIAN_POINT('Ctrl Pts',(-3.28667891078174,29.1868858422458,
-11.6469259874971));
#293233=CARTESIAN_POINT('Ctrl Pts',(-1.74008355600073,29.1266378583166,
-11.9760291153752));
#293234=CARTESIAN_POINT('Ctrl Pts',(1.37448685209422,29.0006508388008,-12.0211925873615));
#293235=CARTESIAN_POINT('Ctrl Pts',(2.91274434176103,28.9401517936605,-11.743680215496));
#293236=CARTESIAN_POINT('Ctrl Pts',(5.83107365352603,28.8176188307369,-10.6068646486473));
#293237=CARTESIAN_POINT('Ctrl Pts',(7.17817733977478,28.7530612262002,-9.74579850908251));
#293238=CARTESIAN_POINT('Ctrl Pts',(9.43735700957167,28.6274564438988,-7.57254521072166));
#293239=CARTESIAN_POINT('Ctrl Pts',(10.3363302801933,28.5690388406801,-6.29026256566099));
#293240=CARTESIAN_POINT('Ctrl Pts',(11.5996396563453,28.4438622385919,-3.44694918231876));
#293241=CARTESIAN_POINT('Ctrl Pts',(11.9490339098776,28.3804256333046,-1.91153005543417));
#293242=CARTESIAN_POINT('Ctrl Pts',(12.0412893187095,28.2584264836826,1.22968847603223));
#293243=CARTESIAN_POINT('Ctrl Pts',(11.7743308323104,28.195501897565,2.80541482406902));
#293244=CARTESIAN_POINT('Ctrl Pts',(10.6572910223695,28.0690938346845,5.72826413975934));
#293245=CARTESIAN_POINT('Ctrl Pts',(9.83130606094285,28.0103029298356,7.05239846244492));
#293246=CARTESIAN_POINT('Ctrl Pts',(7.7039605726298,27.886435546933,9.33403355125254));
#293247=CARTESIAN_POINT('Ctrl Pts',(6.41517677553145,27.8221818590215,10.2625878578183));
#293248=CARTESIAN_POINT('Ctrl Pts',(3.56378173465436,27.6979146157577,11.5644717555374));
#293249=CARTESIAN_POINT('Ctrl Pts',(2.0305743381716,27.6383884572968,11.9295549490862));
#293250=CARTESIAN_POINT('Ctrl Pts',(-1.07924184233729,27.5125937503266,
12.0515849848931));
#293251=CARTESIAN_POINT('Ctrl Pts',(-2.62614400459274,27.4511403249807,
11.811369716088));
#293252=CARTESIAN_POINT('Ctrl Pts',(-5.57677391434579,27.3291850153474,
10.7433073328657));
#293253=CARTESIAN_POINT('Ctrl Pts',(-6.94722786573379,27.2645793236449,
9.91235760254589));
#293254=CARTESIAN_POINT('Ctrl Pts',(-9.25729741802083,27.1385470230812,
7.79116744626057));
#293255=CARTESIAN_POINT('Ctrl Pts',(-10.184729240557,27.0802458792577,6.53231540738293));
#293256=CARTESIAN_POINT('Ctrl Pts',(-11.5158750392046,26.9553650750171,
3.71873225757449));
#293257=CARTESIAN_POINT('Ctrl Pts',(-11.9019263496545,26.8916624070597,
2.18830781033492));
#293258=CARTESIAN_POINT('Ctrl Pts',(-11.9945473038564,26.8223955724385,
0.417909473500312));
#293259=CARTESIAN_POINT('Ctrl Pts',(-12.,26.8142850295081,0.208859150254401));
#293260=CARTESIAN_POINT('Ctrl Pts',(-12.,26.806249999904,1.13312137450805E-13));
#293261=CARTESIAN_POINT('Origin',(-8.79029313101884E-14,130.96875,0.));
#293262=CARTESIAN_POINT('',(-12.,23.431249999916,7.61134619062841E-14));
#293263=CARTESIAN_POINT('',(-12.,23.806249999916,1.38875757267125E-13));
#293264=CARTESIAN_POINT('',(-12.0000000000001,130.96875,-1.46957615897682E-15));
#293265=CARTESIAN_POINT('Ctrl Pts',(-12.,23.431249999916,1.11577413974828E-13));
#293266=CARTESIAN_POINT('Ctrl Pts',(-12.,23.4398130406759,0.22258404820464));
#293267=CARTESIAN_POINT('Ctrl Pts',(-11.9938071335293,23.4484616365627,
0.445379795782725));
#293268=CARTESIAN_POINT('Ctrl Pts',(-11.8943033853353,23.518351927683,2.22974764099004));
#293269=CARTESIAN_POINT('Ctrl Pts',(-11.5027536396383,23.5820916451671,
3.75934858799651));
#293270=CARTESIAN_POINT('Ctrl Pts',(-10.1614602463391,23.7069243478206,
6.56838425218786));
#293271=CARTESIAN_POINT('Ctrl Pts',(-9.22976384960113,23.7652217461412,
7.82370706132516));
#293272=CARTESIAN_POINT('Ctrl Pts',(-6.91208163660612,23.8913151486123,
9.93698914294296));
#293273=CARTESIAN_POINT('Ctrl Pts',(-5.53816396297601,23.9559250022048,
10.7633465114));
#293274=CARTESIAN_POINT('Ctrl Pts',(-2.58274047876639,24.0777894527795,
11.8209897106908));
#293275=CARTESIAN_POINT('Ctrl Pts',(-1.03454361812171,24.139401831489,12.0555579958973));
#293276=CARTESIAN_POINT('Ctrl Pts',(2.07451493030272,24.2651658915976,11.9219010856576));
#293277=CARTESIAN_POINT('Ctrl Pts',(3.60567970990701,24.3245969477269,11.5513830311112));
#293278=CARTESIAN_POINT('Ctrl Pts',(6.45229346006646,24.44894831872,10.2393799661171));
#293279=CARTESIAN_POINT('Ctrl Pts',(7.73816339564967,24.5132262620019,9.3057949290138));
#293280=CARTESIAN_POINT('Ctrl Pts',(9.85740713840747,24.6370256775676,7.01586734759232));
#293281=CARTESIAN_POINT('Ctrl Pts',(10.6784688336598,24.695881211199,5.68868492135024));
#293282=CARTESIAN_POINT('Ctrl Pts',(11.7842800249469,24.8222689400477,2.76271576049254));
#293283=CARTESIAN_POINT('Ctrl Pts',(12.045422510488,24.8850125296937,1.18711851387509));
#293284=CARTESIAN_POINT('Ctrl Pts',(11.9423554273777,25.0071140984816,-1.95324933201141));
#293285=CARTESIAN_POINT('Ctrl Pts',(11.5874432158204,25.0705928692317,-3.48797159679797));
#293286=CARTESIAN_POINT('Ctrl Pts',(10.3139009873652,25.1957277148076,-6.3268747238173));
#293287=CARTESIAN_POINT('Ctrl Pts',(9.41063996641178,25.2541176617196,-7.605640666435));
#293288=CARTESIAN_POINT('Ctrl Pts',(7.14378402625019,25.3797890270167,-9.77112886524276));
#293289=CARTESIAN_POINT('Ctrl Pts',(5.79313702996344,25.4443561104804,-10.6277167262761));
#293290=CARTESIAN_POINT('Ctrl Pts',(2.86990730503427,25.5668052080308,-11.7542602021739));
#293291=CARTESIAN_POINT('Ctrl Pts',(1.3303469679492,25.6274363345891,-12.0261957086734));
#293292=CARTESIAN_POINT('Ctrl Pts',(-1.76483950428071,25.7526392574292,
-11.9698710723832));
#293293=CARTESIAN_POINT('Ctrl Pts',(-3.29140693331789,25.8121342827434,
-11.6429845208071));
#293294=CARTESIAN_POINT('Ctrl Pts',(-6.16526988915022,25.9353702621123,
-10.4153984561717));
#293295=CARTESIAN_POINT('Ctrl Pts',(-7.48022415333472,25.9998084258097,
-9.51510593454787));
#293296=CARTESIAN_POINT('Ctrl Pts',(-9.67043315155746,26.1247825872557,
-7.27344561108007));
#293297=CARTESIAN_POINT('Ctrl Pts',(-10.5309372747227,26.1836057457594,
-5.95983225202021));
#293298=CARTESIAN_POINT('Ctrl Pts',(-11.7001145821,26.3088791217704,-3.08341800519752));
#293299=CARTESIAN_POINT('Ctrl Pts',(-11.9999999983778,26.3716626034119,
-1.54888950087861));
#293300=CARTESIAN_POINT('Ctrl Pts',(-12.,26.4312499994205,-1.25681384743892E-8));
#293301=CARTESIAN_POINT('Ctrl Pts',(-12.,26.806249999904,1.29896093881143E-13));
#293302=CARTESIAN_POINT('Ctrl Pts',(-12.,26.7537890016525,-1.36364892928156));
#293303=CARTESIAN_POINT('Ctrl Pts',(-11.7675527535486,26.6987444641245,
-2.71892659361115));
#293304=CARTESIAN_POINT('Ctrl Pts',(-10.7947443658577,26.5809437486461,
-5.46490380294277));
#293305=CARTESIAN_POINT('Ctrl Pts',(-10.0013609216683,26.5216517362606,
-6.80914524864304));
#293306=CARTESIAN_POINT('Ctrl Pts',(-7.92789050622467,26.398252233563,-9.14525467926901));
#293307=CARTESIAN_POINT('Ctrl Pts',(-6.65870048348816,26.3338537374135,
-10.1068679183002));
#293308=CARTESIAN_POINT('Ctrl Pts',(-3.83925340538554,26.2090478577536,
-11.4753786473057));
#293309=CARTESIAN_POINT('Ctrl Pts',(-2.31956538971854,26.1500783908989,
-11.8761840996725));
#293310=CARTESIAN_POINT('Ctrl Pts',(0.785082900623845,26.0244927294772,
-12.0747109172162));
#293311=CARTESIAN_POINT('Ctrl Pts',(2.34043984396086,25.9619239810052,-11.8716759525006));
#293312=CARTESIAN_POINT('Ctrl Pts',(5.32216235716819,25.8405829440187,-10.8722442458735));
#293313=CARTESIAN_POINT('Ctrl Pts',(6.71507066342784,25.7759647302934,-10.0716736262776));
#293314=CARTESIAN_POINT('Ctrl Pts',(9.0748101075305,25.6495475374532,-8.00266022351069));
#293315=CARTESIAN_POINT('Ctrl Pts',(10.0301109621315,25.5912053758984,-6.7669533887209));
#293316=CARTESIAN_POINT('Ctrl Pts',(11.4274700267537,25.4666566549912,-3.98351626644247));
#293317=CARTESIAN_POINT('Ctrl Pts',(11.8494629126326,25.4027253598738,-2.45882710758252));
#293318=CARTESIAN_POINT('Ctrl Pts',(12.0837415350844,25.2794473222752,0.66948815588767));
#293319=CARTESIAN_POINT('Ctrl Pts',(11.8925943782014,25.2186146452849,2.24305802232372));
#293320=CARTESIAN_POINT('Ctrl Pts',(10.9222168551947,25.0925066677988,5.20576051131627));
#293321=CARTESIAN_POINT('Ctrl Pts',(10.1605857816088,25.0325624351741,6.56941195749918));
#293322=CARTESIAN_POINT('Ctrl Pts',(8.14006577677286,24.909658157909,8.95757294257594));
#293323=CARTESIAN_POINT('Ctrl Pts',(6.89060965781988,24.8451541191261,9.95078653368017));
#293324=CARTESIAN_POINT('Ctrl Pts',(4.10290371893131,24.7198651398814,11.383303631392));
#293325=CARTESIAN_POINT('Ctrl Pts',(2.59635635370549,24.6612748205926,11.8183042639752));
#293326=CARTESIAN_POINT('Ctrl Pts',(-0.50260758961881,24.5359190958379,
12.0901927815865));
#293327=CARTESIAN_POINT('Ctrl Pts',(-2.06582271479834,24.4726857157314,
11.9230053433905));
#293328=CARTESIAN_POINT('Ctrl Pts',(-5.06990412957124,24.35116806988,10.9916693343548));
#293329=CARTESIAN_POINT('Ctrl Pts',(-6.47821009372995,24.2873657358891,
10.22517208831));
#293330=CARTESIAN_POINT('Ctrl Pts',(-8.8830041082046,24.1608698364378,8.21486070050412));
#293331=CARTESIAN_POINT('Ctrl Pts',(-9.86666611749828,24.1023256506135,
7.00290264189264));
#293332=CARTESIAN_POINT('Ctrl Pts',(-11.3311293953531,23.9781576531616,
4.25116536415171));
#293333=CARTESIAN_POINT('Ctrl Pts',(-11.7896882704929,23.9140267567717,
2.7331688646281));
#293334=CARTESIAN_POINT('Ctrl Pts',(-11.9809869533892,23.8365132364504,
0.780472016417012));
#293335=CARTESIAN_POINT('Ctrl Pts',(-12.,23.8212541772838,0.390012220207713));
#293336=CARTESIAN_POINT('Ctrl Pts',(-12.,23.806249999916,3.25017790459015E-13));
#293337=CARTESIAN_POINT('Origin',(-8.79029313101884E-14,130.96875,0.));
#293338=CARTESIAN_POINT('',(-12.,20.431249999928,1.34330781760066E-13));
#293339=CARTESIAN_POINT('',(-12.,20.806249999928,2.71595654142186E-14));
#293340=CARTESIAN_POINT('',(-12.0000000000001,130.96875,-1.46957615897682E-15));
#293341=CARTESIAN_POINT('Ctrl Pts',(-12.,20.431249999928,3.23074900165921E-13));
#293342=CARTESIAN_POINT('Ctrl Pts',(-12.,20.4467848257397,0.403805670704763));
#293343=CARTESIAN_POINT('Ctrl Pts',(-11.9796183449311,20.4625921950636,
0.808073320648967));
#293344=CARTESIAN_POINT('Ctrl Pts',(-11.7801159006779,20.5407344048709,
2.77444649295645));
#293345=CARTESIAN_POINT('Ctrl Pts',(-11.3160449848468,20.604892485555,4.29135863890174));
#293346=CARTESIAN_POINT('Ctrl Pts',(-9.84148614536275,20.7289993282602,
7.03822603928776));
#293347=CARTESIAN_POINT('Ctrl Pts',(-8.85354564014989,20.7875881579817,
8.24658460486558));
#293348=CARTESIAN_POINT('Ctrl Pts',(-6.44249394372589,20.9140664918751,
10.2475442515478));
#293349=CARTESIAN_POINT('Ctrl Pts',(-5.03254351667025,20.9776793384299,
11.0086698879463));
#293350=CARTESIAN_POINT('Ctrl Pts',(-2.02594049367394,21.0992989854766,
11.9299138331781));
#293351=CARTESIAN_POINT('Ctrl Pts',(-0.461644847179159,21.1625760735884,
12.0918926621046));
#293352=CARTESIAN_POINT('Ctrl Pts',(2.63643741123524,21.2878961334393,11.8093688217767));
#293353=CARTESIAN_POINT('Ctrl Pts',(4.14106597654989,21.3464442328503,11.3694152091123));
#293354=CARTESIAN_POINT('Ctrl Pts',(6.92407989691486,21.4718004693551,9.92761136320372));
#293355=CARTESIAN_POINT('Ctrl Pts',(8.17059822423941,21.5363170385871,8.92982723706064));
#293356=CARTESIAN_POINT('Ctrl Pts',(10.1833370256642,21.659145690427,6.53413703540161));
#293357=CARTESIAN_POINT('Ctrl Pts',(10.940323806214,21.719198738833,5.16766084013816));
#293358=CARTESIAN_POINT('Ctrl Pts',(11.9001278424061,21.8452822730432,2.20215818516315));
#293359=CARTESIAN_POINT('Ctrl Pts',(12.0858225482307,21.9059873448058,0.628781301812343));
#293360=CARTESIAN_POINT('Ctrl Pts',(11.8412402405099,22.0293525601758,-2.49845215337111));
#293361=CARTESIAN_POINT('Ctrl Pts',(11.4139731840186,22.0933147054619,-4.0222295365126));
#293362=CARTESIAN_POINT('Ctrl Pts',(10.0069201157794,22.2178111846298,-6.80115893647389));
#293363=CARTESIAN_POINT('Ctrl Pts',(9.04752999575144,22.2761724459011,-8.03345356440084));
#293364=CARTESIAN_POINT('Ctrl Pts',(6.68051948207383,22.4026432132964,-10.0947124632924));
#293365=CARTESIAN_POINT('Ctrl Pts',(5.28435371861963,22.4672603187263,-10.8907529644727));
#293366=CARTESIAN_POINT('Ctrl Pts',(2.29811650048091,22.588507122638,-11.8800074121184));
#293367=CARTESIAN_POINT('Ctrl Pts',(0.741520454552576,22.6512548674486,
-12.0775312505332));
#293368=CARTESIAN_POINT('Ctrl Pts',(-2.36232605474743,22.7768080961458,
-11.8676768837343));
#293369=CARTESIAN_POINT('Ctrl Pts',(-3.87999642471441,22.8357090654822,
-11.4615887160664));
#293370=CARTESIAN_POINT('Ctrl Pts',(-6.69461417398888,22.9605916894066,
-10.0832032383739));
#293371=CARTESIAN_POINT('Ctrl Pts',(-7.96081811139866,23.0250086359743,
-9.11670400877424));
#293372=CARTESIAN_POINT('Ctrl Pts',(-10.0261963824355,23.14833468153,-6.77254619328493));
#293373=CARTESIAN_POINT('Ctrl Pts',(-10.8147096955589,23.2077162761768,
-5.42531660356751));
#293374=CARTESIAN_POINT('Ctrl Pts',(-11.7725905894236,23.3249359390307,
-2.6895927928564));
#293375=CARTESIAN_POINT('Ctrl Pts',(-12.,23.3793605712179,-1.34879179282623));
#293376=CARTESIAN_POINT('Ctrl Pts',(-12.,23.431249999916,1.08246744900953E-13));
#293377=CARTESIAN_POINT('Ctrl Pts',(-12.,23.806249999916,3.29458682557515E-13));
#293378=CARTESIAN_POINT('Ctrl Pts',(-12.,23.761270474463,-1.16917869975571));
#293379=CARTESIAN_POINT('Ctrl Pts',(-11.8291289136152,23.7143161307078,
-2.33417060705515));
#293380=CARTESIAN_POINT('Ctrl Pts',(-11.0446447532021,23.6042128314296,
-4.94125469642478));
#293381=CARTESIAN_POINT('Ctrl Pts',(-10.3151456048164,23.5434465782065,
-6.32437469437398));
#293382=CARTESIAN_POINT('Ctrl Pts',(-8.34863463534201,23.4210817968168,
-8.76418235793767));
#293383=CARTESIAN_POINT('Ctrl Pts',(-7.11976024704336,23.3565060849324,
-9.78873873335731));
#293384=CARTESIAN_POINT('Ctrl Pts',(-4.36476270921836,23.2307694099466,
-11.2851044893288));
#293385=CARTESIAN_POINT('Ctrl Pts',(-2.87146936935017,23.17240337585,-11.7541221595676));
#293386=CARTESIAN_POINT('Ctrl Pts',(0.220985512029197,23.0473109481819,
-12.099075516286));
#293387=CARTESIAN_POINT('Ctrl Pts',(1.7912833647821,22.9837910657267,-11.9677904024354));
#293388=CARTESIAN_POINT('Ctrl Pts',(4.81229210353979,22.8615886952367,-11.1058563450733));
#293389=CARTESIAN_POINT('Ctrl Pts',(6.23173012211203,22.799021172219,-10.3761315516819));
#293390=CARTESIAN_POINT('Ctrl Pts',(8.67914767360568,22.6726540431373,-8.42990231678871));
#293391=CARTESIAN_POINT('Ctrl Pts',(9.69202949891002,22.6137305466513,-7.24261379317035));
#293392=CARTESIAN_POINT('Ctrl Pts',(11.2252803437536,22.4899994638192,-4.52458392404308));
#293393=CARTESIAN_POINT('Ctrl Pts',(11.721445154911,22.4256983166613,-3.0143809076004));
#293394=CARTESIAN_POINT('Ctrl Pts',(12.1005737742388,22.3012645216902,0.0969120056357209));
#293395=CARTESIAN_POINT('Ctrl Pts',(11.9855379923338,22.2419238543774,1.66736754248129));
#293396=CARTESIAN_POINT('Ctrl Pts',(11.1630735659662,22.1161905068203,4.66839193848627));
#293397=CARTESIAN_POINT('Ctrl Pts',(10.4664856162945,22.0544171592613,6.07127028798239));
#293398=CARTESIAN_POINT('Ctrl Pts',(8.55567909165914,21.9326434694289,8.56288812457291));
#293399=CARTESIAN_POINT('Ctrl Pts',(7.34847816608553,21.8680302986595,9.61885092633913));
#293400=CARTESIAN_POINT('Ctrl Pts',(4.62755125718015,21.7418773780287,11.1796175428449));
#293401=CARTESIAN_POINT('Ctrl Pts',(3.1477741743481,21.6835801399995,11.6828769675529));
#293402=CARTESIAN_POINT('Ctrl Pts',(0.0629372260864292,21.558795864199,
12.1013948602857));
#293403=CARTESIAN_POINT('Ctrl Pts',(-1.51368102089066,21.495020316427,12.0065258535606));
#293404=CARTESIAN_POINT('Ctrl Pts',(-4.55079936511367,21.3721662987073,
11.2146319147188));
#293405=CARTESIAN_POINT('Ctrl Pts',(-5.98107330162838,21.3106834381994,
10.5216293205749));
#293406=CARTESIAN_POINT('Ctrl Pts',(-8.47057404200132,21.1844642790414,
8.63954601741154));
#293407=CARTESIAN_POINT('Ctrl Pts',(-9.51248341293276,21.1249906405834,
7.47696583729867));
#293408=CARTESIAN_POINT('Ctrl Pts',(-11.1136666219519,21.0017379116272,
4.79344265898674));
#293409=CARTESIAN_POINT('Ctrl Pts',(-11.6470661436893,20.9373035795534,
3.29187598120315));
#293410=CARTESIAN_POINT('Ctrl Pts',(-11.9582772315793,20.8512438335824,
1.15599407183253));
#293411=CARTESIAN_POINT('Ctrl Pts',(-12.,20.8284767802287,0.577753496285518));
#293412=CARTESIAN_POINT('Ctrl Pts',(-12.,20.806249999928,9.57567358739198E-15));
#293413=CARTESIAN_POINT('Origin',(-8.79029313101884E-14,130.96875,0.));
#293414=CARTESIAN_POINT('',(-12.,17.43124999994,2.44533967916948E-14));
#293415=CARTESIAN_POINT('',(-12.,17.80624999994,-2.19195579930893E-15));
#293416=CARTESIAN_POINT('',(-12.0000000000001,130.96875,-1.46957615897682E-15));
#293417=CARTESIAN_POINT('Ctrl Pts',(-12.,17.43124999994,5.35682609381638E-14));
#293418=CARTESIAN_POINT('Ctrl Pts',(-12.,17.4539971128015,0.591278800092865));
#293419=CARTESIAN_POINT('Ctrl Pts',(-11.9563009265847,17.4773086571402,
1.18303050285719));
#293420=CARTESIAN_POINT('Ctrl Pts',(-11.6357699188653,17.5639823368467,
3.331842519734));
#293421=CARTESIAN_POINT('Ctrl Pts',(-11.0969971356305,17.6284329581875,
4.83208673531864));
#293422=CARTESIAN_POINT('Ctrl Pts',(-9.48602239365201,17.7516128629079,
7.51053548942931));
#293423=CARTESIAN_POINT('Ctrl Pts',(-8.43991362594118,17.8111804351853,
8.66952450881498));
#293424=CARTESIAN_POINT('Ctrl Pts',(-5.94434591436069,17.937376567561,10.5422888708228));
#293425=CARTESIAN_POINT('Ctrl Pts',(-4.5125221168834,17.9987146459351,11.2299639974067));
#293426=CARTESIAN_POINT('Ctrl Pts',(-1.47313381954063,18.1216604851874,
12.0116363905843));
#293427=CARTESIAN_POINT('Ctrl Pts',(0.104337134805024,18.185470525697,12.1011768361982));
#293428=CARTESIAN_POINT('Ctrl Pts',(3.18797499635399,18.3102062974211,11.6719373989125));
#293429=CARTESIAN_POINT('Ctrl Pts',(4.66576764457087,18.3685068068196,11.163686575192));
#293430=CARTESIAN_POINT('Ctrl Pts',(7.38163184806853,18.4947174440379,9.59352427003675));
#293431=CARTESIAN_POINT('Ctrl Pts',(8.58559365724217,18.5593331061441,8.53299842515826));
#293432=CARTESIAN_POINT('Ctrl Pts',(10.4881684878408,18.6810165610806,6.0338457770933));
#293433=CARTESIAN_POINT('Ctrl Pts',(11.179910341594,18.7429520460265,4.62807383611877));
#293434=CARTESIAN_POINT('Ctrl Pts',(11.9913702643163,18.8686547636934,1.62427004050253));
#293435=CARTESIAN_POINT('Ctrl Pts',(12.1007575921369,18.9279100116668,0.0540801116266604));
#293436=CARTESIAN_POINT('Ctrl Pts',(11.7107948809275,19.0524241989025,-3.05578227418279));
#293437=CARTESIAN_POINT('Ctrl Pts',(11.2090827886063,19.1167474287713,-4.56475687833112));
#293438=CARTESIAN_POINT('Ctrl Pts',(9.66570132517863,19.2404101454037,-7.27771802796008));
#293439=CARTESIAN_POINT('Ctrl Pts',(8.64850206774641,19.2994045093754,-8.46134422340063));
#293440=CARTESIAN_POINT('Ctrl Pts',(6.19480894882948,19.4257508803272,-10.3980628251768));
#293441=CARTESIAN_POINT('Ctrl Pts',(4.77374542976002,19.488147940957,-11.1223374114215));
#293442=CARTESIAN_POINT('Ctrl Pts',(1.75029509261386,19.6104490761765,-11.9739224784792));
#293443=CARTESIAN_POINT('Ctrl Pts',(0.179010938886157,19.6740088553441,
-12.0998378860898));
#293444=CARTESIAN_POINT('Ctrl Pts',(-2.91238430867471,19.7990584199239,
-11.7440039397611));
#293445=CARTESIAN_POINT('Ctrl Pts',(-4.40368952208624,19.8574042958986,
-11.2699218185076));
#293446=CARTESIAN_POINT('Ctrl Pts',(-7.15372046582846,19.9832047383442,
-9.7640381692274));
#293447=CARTESIAN_POINT('Ctrl Pts',(-8.37944964047272,20.047788209345,-8.73482644189239));
#293448=CARTESIAN_POINT('Ctrl Pts',(-10.3378062779058,20.1700686233113,
-6.28734366947722));
#293449=CARTESIAN_POINT('Ctrl Pts',(-11.062474098562,20.2309723528992,-4.90131154770073));
#293450=CARTESIAN_POINT('Ctrl Pts',(-11.8333884458573,20.3404879887831,
-2.30509383170136));
#293451=CARTESIAN_POINT('Ctrl Pts',(-12.,20.3868345884464,-1.15451536053513));
#293452=CARTESIAN_POINT('Ctrl Pts',(-12.,20.431249999928,3.34177130412172E-13));
#293453=CARTESIAN_POINT('Ctrl Pts',(-12.,20.806249999928,3.88578058618805E-15));
#293454=CARTESIAN_POINT('Ctrl Pts',(-12.,20.7688814633124,-0.971341885268998));
#293455=CARTESIAN_POINT('Ctrl Pts',(-11.8820664283109,20.7300961104164,
-1.94119295148273));
#293456=CARTESIAN_POINT('Ctrl Pts',(-11.2730074993954,20.6279881502184,
-4.39744870216082));
#293457=CARTESIAN_POINT('Ctrl Pts',(-10.6089181380125,20.5650608786088,
-5.81965308324059));
#293458=CARTESIAN_POINT('Ctrl Pts',(-8.75344208941597,20.4439075836876,
-8.36133391417179));
#293459=CARTESIAN_POINT('Ctrl Pts',(-7.56818400896899,20.3792923083396,
-9.44758696664805));
#293460=CARTESIAN_POINT('Ctrl Pts',(-4.88142122317779,20.2527696970531,
-11.070925094903));
#293461=CARTESIAN_POINT('Ctrl Pts',(-3.41491999798804,20.1943864155705,
-11.6074121784866));
#293462=CARTESIAN_POINT('Ctrl Pts',(-0.338486781005807,20.0699420778411,
-12.0972787778748));
#293463=CARTESIAN_POINT('Ctrl Pts',(1.24347617575282,20.0059503320169,-12.0379651060085));
#293464=CARTESIAN_POINT('Ctrl Pts',(4.29532847004766,19.8825003134971,-11.3141577789942));
#293465=CARTESIAN_POINT('Ctrl Pts',(5.7357830630127,19.8219172611387,-10.6564938888015));
#293466=CARTESIAN_POINT('Ctrl Pts',(8.26535369452417,19.6958580483938,-8.83628916380843));
#293467=CARTESIAN_POINT('Ctrl Pts',(9.3350663651124,19.6356949967075,-7.69756403507541));
#293468=CARTESIAN_POINT('Ctrl Pts',(11.0008950231688,19.512941282377,-5.04801661087702));
#293469=CARTESIAN_POINT('Ctrl Pts',(11.5697929225376,19.4484131411879,-3.55554562082969));
#293470=CARTESIAN_POINT('Ctrl Pts',(12.0910996598554,19.3229917907181,-0.464779079887096));
#293471=CARTESIAN_POINT('Ctrl Pts',(12.0497536139095,19.2644818519719,1.10186944496459));
#293472=CARTESIAN_POINT('Ctrl Pts',(11.3712584209357,19.1391975620908,4.13799966585378));
#293473=CARTESIAN_POINT('Ctrl Pts',(10.7383436427877,19.0758783728349,5.57824532750321));
#293474=CARTESIAN_POINT('Ctrl Pts',(8.94173389183376,18.9541597065169,8.15839479986107));
#293475=CARTESIAN_POINT('Ctrl Pts',(7.78665902721745,18.8907290269032,9.26728093053828));
#293476=CARTESIAN_POINT('Ctrl Pts',(5.14538467415531,18.7642682730146,10.9506268864999));
#293477=CARTESIAN_POINT('Ctrl Pts',(3.69293246893586,18.7056322562587,11.5218708993174));
#293478=CARTESIAN_POINT('Ctrl Pts',(0.626341788480967,18.5815860574952,
12.0862741549164));
#293479=CARTESIAN_POINT('Ctrl Pts',(-0.960370917922583,18.5174021802619,
12.0643298816322));
#293480=CARTESIAN_POINT('Ctrl Pts',(-4.02668243917191,18.3933672737255,
11.4118148451283));
#293481=CARTESIAN_POINT('Ctrl Pts',(-5.47745451590982,18.3335642700473,
10.7907907424887));
#293482=CARTESIAN_POINT('Ctrl Pts',(-8.0481511058204,18.2076884424295,9.03490394444749));
#293483=CARTESIAN_POINT('Ctrl Pts',(-9.14656576390013,18.146647146687,7.92100201639144));
#293484=CARTESIAN_POINT('Ctrl Pts',(-10.8786540110187,18.0244498374781,
5.30744659638946));
#293485=CARTESIAN_POINT('Ctrl Pts',(-11.48397828387,17.9598595509646,3.82519587335654));
#293486=CARTESIAN_POINT('Ctrl Pts',(-11.9279001944013,17.8655889419805,
1.51900463488298));
#293487=CARTESIAN_POINT('Ctrl Pts',(-12.,17.8354684935126,0.759493124481815));
#293488=CARTESIAN_POINT('Ctrl Pts',(-12.,17.80624999994,1.04083408558608E-14));
#293489=CARTESIAN_POINT('Origin',(-8.79029313101884E-14,130.96875,0.));
#293490=CARTESIAN_POINT('',(-12.,14.431249999952,-1.35928853084006E-15));
#293491=CARTESIAN_POINT('',(-12.,14.806249999952,-4.36865413446742E-14));
#293492=CARTESIAN_POINT('',(-12.0000000000001,130.96875,-1.46957615897682E-15));
#293493=CARTESIAN_POINT('Ctrl Pts',(-12.,14.431249999952,4.16333634234434E-16));
#293494=CARTESIAN_POINT('Ctrl Pts',(-12.,14.460987767858,0.772990921177218));
#293495=CARTESIAN_POINT('Ctrl Pts',(-11.9253146601718,14.4916574086311,
1.54593781233599));
#293496=CARTESIAN_POINT('Ctrl Pts',(-11.4708998428656,14.5865337222738,
3.86446412862074));
#293497=CARTESIAN_POINT('Ctrl Pts',(-10.8602603601541,14.6511301570846,
5.34514765151272));
#293498=CARTESIAN_POINT('Ctrl Pts',(-9.1185074465202,14.7732424691752,7.95335345197746));
#293499=CARTESIAN_POINT('Ctrl Pts',(-8.01588770460201,14.834426599361,9.06360143593913));
#293500=CARTESIAN_POINT('Ctrl Pts',(-5.43918583426702,14.9602740213547,
10.8100279769507));
#293501=CARTESIAN_POINT('Ctrl Pts',(-3.98691784246459,15.0199757854631,
11.4256709688868));
#293502=CARTESIAN_POINT('Ctrl Pts',(-0.918554175498763,15.1440937030375,
12.0676565860704));
#293503=CARTESIAN_POINT('Ctrl Pts',(0.66878655424738,15.2083029843487,12.0840709717991));
#293504=CARTESIAN_POINT('Ctrl Pts',(3.73383381415189,15.3322867504394,11.508673841105));
#293505=CARTESIAN_POINT('Ctrl Pts',(5.18419781753589,15.3909742483674,10.9322978502764));
#293506=CARTESIAN_POINT('Ctrl Pts',(7.81855818192678,15.5174167452044,9.24020346931188));
#293507=CARTESIAN_POINT('Ctrl Pts',(8.9690674588818,15.5806656015378,8.12813241825711));
#293508=CARTESIAN_POINT('Ctrl Pts',(10.7568932976436,15.702484090034,5.54253414447198));
#293509=CARTESIAN_POINT('Ctrl Pts',(11.3851948471033,15.765845384446,4.09969509039685));
#293510=CARTESIAN_POINT('Ctrl Pts',(12.0533520147543,15.8910924437712,1.0611735967341));
#293511=CARTESIAN_POINT('Ctrl Pts',(12.0894255701802,15.9495668040691,-0.505175363631084));
#293512=CARTESIAN_POINT('Ctrl Pts',(11.5578801980134,16.0750536126133,-3.59431665985857));
#293513=CARTESIAN_POINT('Ctrl Pts',(10.9837525372396,16.1395928120628,-5.08537584114874));
#293514=CARTESIAN_POINT('Ctrl Pts',(9.30840727074358,16.2622694239057,-7.72982696247656));
#293515=CARTESIAN_POINT('Ctrl Pts',(8.23458548037391,16.3225478455797,-8.86501066592352));
#293516=CARTESIAN_POINT('Ctrl Pts',(5.69911229414429,16.448581933702,-10.6760345176555));
#293517=CARTESIAN_POINT('Ctrl Pts',(4.25716889207649,16.5090439008629,-11.3284625629591));
#293518=CARTESIAN_POINT('Ctrl Pts',(1.20319891082697,16.6325795816195,-12.0421254554265));
#293519=CARTESIAN_POINT('Ctrl Pts',(-0.379492791011095,16.6966008058014,
-12.096129889922));
#293520=CARTESIAN_POINT('Ctrl Pts',(-3.45459032687708,16.8209911140947,
-11.5956465592013));
#293521=CARTESIAN_POINT('Ctrl Pts',(-4.91910185381263,16.8794001840513,
-11.0542122147388));
#293522=CARTESIAN_POINT('Ctrl Pts',(-7.60033579695139,17.005958400366,-9.42176679373339));
#293523=CARTESIAN_POINT('Ctrl Pts',(-8.78184023446649,17.0705029359655,
-8.3314626220704));
#293524=CARTESIAN_POINT('Ctrl Pts',(-10.6289833189954,17.1916298915339,
-5.78311310327076));
#293525=CARTESIAN_POINT('Ctrl Pts',(-11.2883210946912,17.2546928414801,
-4.35811336985312));
#293526=CARTESIAN_POINT('Ctrl Pts',(-11.8854674394808,17.3562186805609,
-1.91311839528264));
#293527=CARTESIAN_POINT('Ctrl Pts',(-12.,17.3944241966078,-0.957234306581829));
#293528=CARTESIAN_POINT('Ctrl Pts',(-12.,17.43124999994,5.60662627435704E-14));
#293529=CARTESIAN_POINT('Ctrl Pts',(-12.,17.80624999994,1.13797860024079E-14));
#293530=CARTESIAN_POINT('Ctrl Pts',(-12.,17.7761119753235,-0.783395024280319));
#293531=CARTESIAN_POINT('Ctrl Pts',(-11.9232906485854,17.7450186926119,
-1.56669624300091));
#293532=CARTESIAN_POINT('Ctrl Pts',(-11.465508196661,17.6506612618365,-3.87064072738115));
#293533=CARTESIAN_POINT('Ctrl Pts',(-10.8648852070875,17.5870633542603,
-5.32862351292106));
#293534=CARTESIAN_POINT('Ctrl Pts',(-9.12953434449562,17.4646669131686,
-7.94629499456211));
#293535=CARTESIAN_POINT('Ctrl Pts',(-8.0061267671257,17.4024323741593,-9.07712725864556));
#293536=CARTESIAN_POINT('Ctrl Pts',(-5.4128771983687,17.276106583186,-10.8208973231749));
#293537=CARTESIAN_POINT('Ctrl Pts',(-3.97494086041983,17.2170397353279,
-11.4276386605344));
#293538=CARTESIAN_POINT('Ctrl Pts',(-0.919494781300424,17.0934443451582,
-12.0680067393541));
#293539=CARTESIAN_POINT('Ctrl Pts',(0.671174299028302,17.0291004292379,
-12.0843598021253));
#293540=CARTESIAN_POINT('Ctrl Pts',(3.75124351266482,16.9045090123542,-11.5046737807013));
#293541=CARTESIAN_POINT('Ctrl Pts',(5.21222391654724,16.8453331927415,-10.9207152458411));
#293542=CARTESIAN_POINT('Ctrl Pts',(7.82411039744174,16.719660545862,-9.23006694389104));
#293543=CARTESIAN_POINT('Ctrl Pts',(8.95143845658941,16.6575643890469,-8.14137947652282));
#293544=CARTESIAN_POINT('Ctrl Pts',(10.7497470693045,16.535969257765,-5.56499311512457));
#293545=CARTESIAN_POINT('Ctrl Pts',(11.3914932367514,16.471351912502,-4.09387322936519));
#293546=CARTESIAN_POINT('Ctrl Pts',(12.0557290891391,16.3450861452902,-1.02759776257042));
#293547=CARTESIAN_POINT('Ctrl Pts',(12.087630137356,16.2867792276593,0.53458775095372));
#293548=CARTESIAN_POINT('Ctrl Pts',(11.5531974907912,16.1620912636547,3.60202608884916));
#293549=CARTESIAN_POINT('Ctrl Pts',(10.9852331632466,16.0982485173233,5.076984551652));
#293550=CARTESIAN_POINT('Ctrl Pts',(9.31133355087314,15.9752145821935,7.7311935043871));
#293551=CARTESIAN_POINT('Ctrl Pts',(8.21929404044133,15.9140133905269,8.8834467907717));
#293552=CARTESIAN_POINT('Ctrl Pts',(5.67377710036676,15.7878398859371,10.6865102472551));
#293553=CARTESIAN_POINT('Ctrl Pts',(4.2502971290847,15.7281781303768,11.3282027085803));
#293554=CARTESIAN_POINT('Ctrl Pts',(1.20688282896854,15.6050694358914,12.043152154094));
#293555=CARTESIAN_POINT('Ctrl Pts',(-0.386795444128867,15.5406037955665,
12.09728761924));
#293556=CARTESIAN_POINT('Ctrl Pts',(-3.47941185947045,15.4155048337123,
11.5892705222127));
#293557=CARTESIAN_POINT('Ctrl Pts',(-4.95013874828265,15.3567806387341,
11.0414482393785));
#293558=CARTESIAN_POINT('Ctrl Pts',(-7.60162688164875,15.231330848694,9.41467995783229));
#293559=CARTESIAN_POINT('Ctrl Pts',(-8.75706777119083,15.1682221135034,
8.35074986546862));
#293560=CARTESIAN_POINT('Ctrl Pts',(-10.6178353111347,15.046991234969,5.81308909801941));
#293561=CARTESIAN_POINT('Ctrl Pts',(-11.2941531048397,14.9826465868061,
4.35583447463269));
#293562=CARTESIAN_POINT('Ctrl Pts',(-11.8885694328649,14.8802421012849,
1.88711330108603));
#293563=CARTESIAN_POINT('Ctrl Pts',(-12.,14.8425737134021,0.944183195223962));
#293564=CARTESIAN_POINT('Ctrl Pts',(-12.,14.806249999952,-1.00475183728577E-13));
#293565=CARTESIAN_POINT('Origin',(-8.79029313101884E-14,130.96875,0.));
#293566=CARTESIAN_POINT('',(-12.,11.431249999964,-3.88293156119391E-14));
#293567=CARTESIAN_POINT('',(-12.,11.806249999964,-8.49382656034026E-14));
#293568=CARTESIAN_POINT('',(-12.0000000000001,130.96875,-1.46957615897682E-15));
#293569=CARTESIAN_POINT('Ctrl Pts',(-12.,11.431249999964,-5.07927033766009E-14));
#293570=CARTESIAN_POINT('Ctrl Pts',(-12.,11.468121395742,0.958419417275447));
#293571=CARTESIAN_POINT('Ctrl Pts',(-11.8851836503325,11.5063744328613,
1.91544653988381));
#293572=CARTESIAN_POINT('Ctrl Pts',(-11.2788881633895,11.6093366144611,
4.39480445595943));
#293573=CARTESIAN_POINT('Ctrl Pts',(-10.5980910112658,11.6734842595123,
5.84870775642085));
#293574=CARTESIAN_POINT('Ctrl Pts',(-8.72938078653482,11.7948184680951,
8.37978226182653));
#293575=CARTESIAN_POINT('Ctrl Pts',(-7.57001013475369,11.8579724084575,
9.44020476171866));
#293576=CARTESIAN_POINT('Ctrl Pts',(-4.91298096368815,11.9833893373363,
11.0579643683581));
#293577=CARTESIAN_POINT('Ctrl Pts',(-3.44089744373657,12.0420627745674,
11.6006993699913));
#293578=CARTESIAN_POINT('Ctrl Pts',(-0.34658463568243,12.1672303569483,
12.0985754145678));
#293579=CARTESIAN_POINT('Ctrl Pts',(1.24744865956387,12.2317103582207,12.0390876488422));
#293580=CARTESIAN_POINT('Ctrl Pts',(4.28907572010713,12.3547467573467,11.3135987775732));
#293581=CARTESIAN_POINT('Ctrl Pts',(5.71049570567009,12.4145064081564,10.6669576658726));
#293582=CARTESIAN_POINT('Ctrl Pts',(8.24921959246757,12.5406568322771,8.85551510332783));
#293583=CARTESIAN_POINT('Ctrl Pts',(9.33680374771899,12.6017236380238,7.70024351636594));
#293584=CARTESIAN_POINT('Ctrl Pts',(11.0019126150717,12.7248453601402,5.04089637975034));
#293585=CARTESIAN_POINT('Ctrl Pts',(11.5651846431726,12.78872030928,3.56357623029895));
#293586=CARTESIAN_POINT('Ctrl Pts',(12.0893260345269,12.913359362794,0.494065419426067));
#293587=CARTESIAN_POINT('Ctrl Pts',(12.0522083116166,12.9716759408897,-1.06777826455158));
#293588=CARTESIAN_POINT('Ctrl Pts',(11.3777405180559,13.0979963969138,-4.13215072990994));
#293589=CARTESIAN_POINT('Ctrl Pts',(10.7307949238898,13.162614709663,-5.60160636794518));
#293590=CARTESIAN_POINT('Ctrl Pts',(8.9230328122269,13.2841200741918,-8.17258774244646));
#293591=CARTESIAN_POINT('Ctrl Pts',(7.79155726353775,13.3463814656007,-9.25764068226929));
#293592=CARTESIAN_POINT('Ctrl Pts',(5.17378153763854,13.4720234616693,-10.9388940070764));
#293593=CARTESIAN_POINT('Ctrl Pts',(3.7113512800567,13.5311226870725,-11.517523069066));
#293594=CARTESIAN_POINT('Ctrl Pts',(0.629377258875286,13.6557911550399,
-12.0866799579317));
#293595=CARTESIAN_POINT('Ctrl Pts',(-0.961788845064329,13.7201551759877,
-12.064781443821));
#293596=CARTESIAN_POINT('Ctrl Pts',(-4.01553325036617,13.8436817320055,
-11.4134456384658));
#293597=CARTESIAN_POINT('Ctrl Pts',(-5.45135669482629,13.9028253429919,
-10.8015713665829));
#293598=CARTESIAN_POINT('Ctrl Pts',(-8.0376235095307,14.0291299589728,-9.0490809538014));
#293599=CARTESIAN_POINT('Ctrl Pts',(-9.15643559500131,14.0912036179821,
-7.91509128812461));
#293600=CARTESIAN_POINT('Ctrl Pts',(-10.8828318353858,14.2136955710466,
-5.29202757565925));
#293601=CARTESIAN_POINT('Ctrl Pts',(-11.4787118397578,14.2773313132461,
-3.83152024366495));
#293602=CARTESIAN_POINT('Ctrl Pts',(-11.9259733144817,14.3711130450116,
-1.53912176236354));
#293603=CARTESIAN_POINT('Ctrl Pts',(-12.,14.4016436505551,-0.769574884210652));
#293604=CARTESIAN_POINT('Ctrl Pts',(-12.,14.431249999952,8.46545056276682E-15));
#293605=CARTESIAN_POINT('Ctrl Pts',(-12.,14.806249999952,-1.08524300657109E-13));
#293606=CARTESIAN_POINT('Ctrl Pts',(-12.,14.7833237431069,-0.595935392792773));
#293607=CARTESIAN_POINT('Ctrl Pts',(-11.9556099107365,14.7598250575928,
-1.19232703919809));
#293608=CARTESIAN_POINT('Ctrl Pts',(-11.6333140357018,14.6733316268826,
-3.33588029999469));
#293609=CARTESIAN_POINT('Ctrl Pts',(-11.0979184575167,14.6092803890216,
-4.82684043130409));
#293610=CARTESIAN_POINT('Ctrl Pts',(-9.48485046374418,14.4856561552388,
-7.51615874779507));
#293611=CARTESIAN_POINT('Ctrl Pts',(-8.42348187457655,14.4253170025921,
-8.68907439094324));
#293612=CARTESIAN_POINT('Ctrl Pts',(-5.92479762126047,14.2993094887007,
-10.5496161928145));
#293613=CARTESIAN_POINT('Ctrl Pts',(-4.51553444132652,14.23890720504,-11.2253024111993));
#293614=CARTESIAN_POINT('Ctrl Pts',(-1.48480981289121,14.1163118185567,
-12.0125344581499));
#293615=CARTESIAN_POINT('Ctrl Pts',(0.110952708358791,14.0517618686231,
-12.1034359909647));
#293616=CARTESIAN_POINT('Ctrl Pts',(3.21482169659992,13.9262077306336,-11.6650344976422));
#293617=CARTESIAN_POINT('Ctrl Pts',(4.69475560629124,13.8677669508926,-11.1520111884328));
#293618=CARTESIAN_POINT('Ctrl Pts',(7.38375802076941,13.7425595614282,-9.58707188710994));
#293619=CARTESIAN_POINT('Ctrl Pts',(8.56586069103511,13.6791551935694,-8.54740472438333));
#293620=CARTESIAN_POINT('Ctrl Pts',(10.4806400999911,13.557233721765,-6.05503960750681));
#293621=CARTESIAN_POINT('Ctrl Pts',(11.1873622091499,13.494170481708,-4.62068324356806));
#293622=CARTESIAN_POINT('Ctrl Pts',(11.993432245557,13.3677473913579,-1.59640310585493));
#293623=CARTESIAN_POINT('Ctrl Pts',(12.0991493850008,13.3090025850949,-0.0393339420722724));
#293624=CARTESIAN_POINT('Ctrl Pts',(11.7105867762451,13.1850846193959,3.05548543495258));
#293625=CARTESIAN_POINT('Ctrl Pts',(11.2097277761212,13.1208497738241,4.56243980164547));
#293626=CARTESIAN_POINT('Ctrl Pts',(9.66073170363857,12.9966465906864,7.28762531122103));
#293627=CARTESIAN_POINT('Ctrl Pts',(8.6312727436616,12.9370461441711,8.48176401491606));
#293628=CARTESIAN_POINT('Ctrl Pts',(6.1814877412528,12.8112285633671,10.4016215629996));
#293629=CARTESIAN_POINT('Ctrl Pts',(4.78710944777118,12.749892644819,11.1125044187706));
#293630=CARTESIAN_POINT('Ctrl Pts',(1.7705270509074,12.6278693236197,11.9742604606147));
#293631=CARTESIAN_POINT('Ctrl Pts',(0.173477555825857,12.563267314501,12.1031955259798));
#293632=CARTESIAN_POINT('Ctrl Pts',(-2.94105624238201,12.4372817758863,
11.7367268103642));
#293633=CARTESIAN_POINT('Ctrl Pts',(-4.43025614388931,12.378975406019,11.2593695964559));
#293634=CARTESIAN_POINT('Ctrl Pts',(-7.15675630678309,12.2540588534684,
9.75827367924247));
#293635=CARTESIAN_POINT('Ctrl Pts',(-8.36563209591937,12.1903847159397,
8.74411044859983));
#293636=CARTESIAN_POINT('Ctrl Pts',(-10.3349794652727,12.0677948191106,
6.29873873932138));
#293637=CARTESIAN_POINT('Ctrl Pts',(-11.0722999088359,12.0058840092412,
4.88777370037917));
#293638=CARTESIAN_POINT('Ctrl Pts',(-11.8374969081264,11.8958645770464,
2.27660283786094));
#293639=CARTESIAN_POINT('Ctrl Pts',(-12.,11.8501144449795,1.14019377199156));
#293640=CARTESIAN_POINT('Ctrl Pts',(-12.,11.806249999964,-1.58206781009085E-13));
#293641=CARTESIAN_POINT('Origin',(-8.79029313101884E-14,130.96875,0.));
#293642=CARTESIAN_POINT('',(-12.,8.43124999997595,-1.13942842121735E-13));
#293643=CARTESIAN_POINT('',(-12.,8.80624999997602,-8.17810688771248E-14));
#293644=CARTESIAN_POINT('',(-12.0000000000001,130.96875,-1.46957615897682E-15));
#293645=CARTESIAN_POINT('Ctrl Pts',(-12.,8.43124999997595,-2.38142838782096E-13));
#293646=CARTESIAN_POINT('Ctrl Pts',(-12.,8.47567904276991,1.15486968708691));
#293647=CARTESIAN_POINT('Ctrl Pts',(-11.8332862861018,8.52203689564963,
2.30570747586626));
#293648=CARTESIAN_POINT('Ctrl Pts',(-11.0546840741179,8.63262018149063,
4.92717929318519));
#293649=CARTESIAN_POINT('Ctrl Pts',(-10.3128518110714,8.6943731952545,6.33466675125794));
#293650=CARTESIAN_POINT('Ctrl Pts',(-8.33544286534331,8.81705929161092,
8.772988659322));
#293651=CARTESIAN_POINT('Ctrl Pts',(-7.12262737739931,8.88077073210684,
9.78329826619002));
#293652=CARTESIAN_POINT('Ctrl Pts',(-4.39062248372888,9.00564032179357,
11.2748423843938));
#293653=CARTESIAN_POINT('Ctrl Pts',(-2.90005621554315,9.06394026182268,
11.7468847293909));
#293654=CARTESIAN_POINT('Ctrl Pts',(0.215990291541665,9.18998699079689,
12.1025858000625));
#293655=CARTESIAN_POINT('Ctrl Pts',(1.81315678618581,9.25459373264729,11.9679551876436));
#293656=CARTESIAN_POINT('Ctrl Pts',(4.82753254542353,9.37652779347956,11.0950577850757));
#293657=CARTESIAN_POINT('Ctrl Pts',(6.21966467391305,9.43801819258929,10.378898502507));
#293658=CARTESIAN_POINT('Ctrl Pts',(8.66208380791205,9.5638057413359,8.45016580927124));
#293659=CARTESIAN_POINT('Ctrl Pts',(9.68674645413114,9.62330923814904,7.25285986368789));
#293660=CARTESIAN_POINT('Ctrl Pts',(11.2260430133152,9.74759630337008,4.52234239591337));
#293661=CARTESIAN_POINT('Ctrl Pts',(11.7216544504217,9.81185575689031,3.01304334406987));
#293662=CARTESIAN_POINT('Ctrl Pts',(12.0989206745883,9.93570728451623,-0.0837194877233916));
#293663=CARTESIAN_POINT('Ctrl Pts',(11.9874952273135,9.99451299425393,-1.64036838390401));
#293664=CARTESIAN_POINT('Ctrl Pts',(11.1706301135791,10.1209163279355,-4.66062744191089));
#293665=CARTESIAN_POINT('Ctrl Pts',(10.4593290033012,10.1837981545383,-6.0915050773422));
#293666=CARTESIAN_POINT('Ctrl Pts',(8.53639605876238,10.3058213938744,-8.57692800386591));
#293667=CARTESIAN_POINT('Ctrl Pts',(7.35028185501117,10.3692679518947,-9.61284821886774));
#293668=CARTESIAN_POINT('Ctrl Pts',(4.6556505078725,10.4944348524845,-11.1683370581618));
#293669=CARTESIAN_POINT('Ctrl Pts',(3.1743300758674,10.5528456511109,-11.6760645492037));
#293670=CARTESIAN_POINT('Ctrl Pts',(0.0688214425628372,10.6784661141365,
-12.1038217757956));
#293671=CARTESIAN_POINT('Ctrl Pts',(-1.52718699512888,10.7430260115992,
-12.0072944293978));
#293672=CARTESIAN_POINT('Ctrl Pts',(-4.55588475974131,10.8655394097185,
-11.2090242181891));
#293673=CARTESIAN_POINT('Ctrl Pts',(-5.96295820240637,10.9260690566215,
-10.5281349593043));
#293674=CARTESIAN_POINT('Ctrl Pts',(-8.45443974112375,11.0520496403179,
-8.65881211458809));
#293675=CARTESIAN_POINT('Ctrl Pts',(-9.51110070527266,11.1122696139857,
-7.48274840654294));
#293676=CARTESIAN_POINT('Ctrl Pts',(-11.1147663784201,11.2359815304433,
-4.78809590464511));
#293677=CARTESIAN_POINT('Ctrl Pts',(-11.6451082116492,11.3000620123745,
-3.29473355410627));
#293678=CARTESIAN_POINT('Ctrl Pts',(-11.9577152330903,11.3859513408221,
-1.16373497183783));
#293679=CARTESIAN_POINT('Ctrl Pts',(-12.,11.4088740267595,-0.581631553322767));
#293680=CARTESIAN_POINT('Ctrl Pts',(-12.,11.431249999964,-4.94049245958195E-14));
#293681=CARTESIAN_POINT('Ctrl Pts',(-12.,11.806249999964,-1.61745616900077E-13));
#293682=CARTESIAN_POINT('Ctrl Pts',(-12.,11.7908310580493,-0.400793433853994));
#293683=CARTESIAN_POINT('Ctrl Pts',(-11.9799212696319,11.7751438853602,
-0.802035169667738));
#293684=CARTESIAN_POINT('Ctrl Pts',(-11.7816700157317,11.6969204614742,
-2.77092592266831));
#293685=CARTESIAN_POINT('Ctrl Pts',(-11.316093947334,11.6325364866386,-4.29322081162527));
#293686=CARTESIAN_POINT('Ctrl Pts',(-9.83214892128302,11.5077893688272,
-7.05368149456638));
#293687=CARTESIAN_POINT('Ctrl Pts',(-8.83468948695932,11.448765508599,-8.26884438344096));
#293688=CARTESIAN_POINT('Ctrl Pts',(-6.43412768719993,11.3231554888659,
-10.2477221527081));
#293689=CARTESIAN_POINT('Ctrl Pts',(-5.0547814365477,11.2607202042168,-10.9937426620182));
#293690=CARTESIAN_POINT('Ctrl Pts',(-2.05331204574442,11.1393082169545,
-11.9295289522943));
#293691=CARTESIAN_POINT('Ctrl Pts',(-0.455853701824085,11.0746896695529,
-12.0963479369981));
#293692=CARTESIAN_POINT('Ctrl Pts',(2.66833162018204,10.9483137185994,-11.8014923603382));
#293693=CARTESIAN_POINT('Ctrl Pts',(4.1665243434072,10.8899838299704,-11.3593715915035));
#293694=CARTESIAN_POINT('Ctrl Pts',(6.92911439357375,10.7653959840471,-9.92177404670185));
#293695=CARTESIAN_POINT('Ctrl Pts',(8.16385933511844,10.7014886122352,-8.93340716820374));
#293696=CARTESIAN_POINT('Ctrl Pts',(10.1863084718864,10.5782773839634,-6.53499150991227));
#293697=CARTESIAN_POINT('Ctrl Pts',(10.9533146286252,10.5173454636238,-5.14703722123551));
#293698=CARTESIAN_POINT('Ctrl Pts',(11.9019288490941,10.391219130035,-2.17678626584642));
#293699=CARTESIAN_POINT('Ctrl Pts',(12.0831664937677,10.3313554208171,-0.625557225353349));
#293700=CARTESIAN_POINT('Ctrl Pts',(11.8440955525672,10.2083941351607,2.49296740377523));
#293701=CARTESIAN_POINT('Ctrl Pts',(11.4132093961979,10.1439001263703,4.02939390434652));
#293702=CARTESIAN_POINT('Ctrl Pts',(9.99287701464981,10.0186629073762,6.82326307060616));
#293703=CARTESIAN_POINT('Ctrl Pts',(9.02633952552437,9.96003821567332,8.05851500568563));
#293704=CARTESIAN_POINT('Ctrl Pts',(6.67373853886068,9.83465590549268,10.0938280512869));
#293705=CARTESIAN_POINT('Ctrl Pts',(5.30914420066387,9.77145631141753,10.873704505715));
#293706=CARTESIAN_POINT('Ctrl Pts',(2.32841002448062,9.65001698073936,11.8786306257011));
#293707=CARTESIAN_POINT('Ctrl Pts',(0.737139668560564,9.58606792592722,
12.0822450578068));
#293708=CARTESIAN_POINT('Ctrl Pts',(-2.39033521655523,9.45955890935075,
11.8607856440462));
#293709=CARTESIAN_POINT('Ctrl Pts',(-3.89747585812195,9.40104631775012,
11.4543296406377));
#293710=CARTESIAN_POINT('Ctrl Pts',(-6.69561629539186,9.27683225742513,
10.0813838633756));
#293711=CARTESIAN_POINT('Ctrl Pts',(-7.95592592650306,9.21272264692234,
9.11969790764957));
#293712=CARTESIAN_POINT('Ctrl Pts',(-10.031280211762,9.08892190382184,6.76930583631912));
#293713=CARTESIAN_POINT('Ctrl Pts',(-10.8277989771356,9.02882012738768,
5.40452225488909));
#293714=CARTESIAN_POINT('Ctrl Pts',(-11.777351614017,8.91141976316705,2.66139535479353));
#293715=CARTESIAN_POINT('Ctrl Pts',(-12.,8.85759349064843,1.33460091143043));
#293716=CARTESIAN_POINT('Ctrl Pts',(-12.,8.80624999997602,-1.55708779203678E-13));
#293717=CARTESIAN_POINT('Origin',(-8.79029313101884E-14,130.96875,0.));
#293718=CARTESIAN_POINT('',(-12.,5.43124999998795,-4.9081531354962E-14));
#293719=CARTESIAN_POINT('',(-12.,5.80624999998803,-4.33395966494788E-14));
#293720=CARTESIAN_POINT('',(-12.0000000000001,130.96875,-1.46957615897682E-15));
#293721=CARTESIAN_POINT('Ctrl Pts',(-12.,5.43124999998796,-1.0547118733939E-13));
#293722=CARTESIAN_POINT('Ctrl Pts',(-12.,5.48316066100001,1.34934369658807));
#293723=CARTESIAN_POINT('Ctrl Pts',(-11.772405113539,5.53760150108826,2.69050573314737));
#293724=CARTESIAN_POINT('Ctrl Pts',(-10.808283298763,5.65555307592163,5.44322675517562));
#293725=CARTESIAN_POINT('Ctrl Pts',(-10.0073226821317,5.71554268054446,
6.80449854506295));
#293726=CARTESIAN_POINT('Ctrl Pts',(-7.92399898072301,5.83942961064025,
9.14754655087858));
#293727=CARTESIAN_POINT('Ctrl Pts',(-6.65985819086981,5.90356699044507,
10.1051273038608));
#293728=CARTESIAN_POINT('Ctrl Pts',(-3.85639847296629,6.0277206464562,11.4682112052612));
#293729=CARTESIAN_POINT('Ctrl Pts',(-2.34791038983903,6.08627502965305,
11.8692437344367));
#293730=CARTESIAN_POINT('Ctrl Pts',(0.779138761520414,6.21276682493733,
12.0794649387276));
#293731=CARTESIAN_POINT('Ctrl Pts',(2.36858754625643,6.27652418701721,11.8705394221944));
#293732=CARTESIAN_POINT('Ctrl Pts',(5.34545009884912,6.39806595211044,10.8559762327792));
#293733=CARTESIAN_POINT('Ctrl Pts',(6.70787386690365,6.46130969798621,10.0712552868311));
#293734=CARTESIAN_POINT('Ctrl Pts',(9.05353598797736,6.58665709630091,8.02786005241167));
#293735=CARTESIAN_POINT('Ctrl Pts',(10.0156193450479,6.64523716971519,6.78973179473641));
#293736=CARTESIAN_POINT('Ctrl Pts',(11.42672840657,6.77054206895559,3.99110653852963));
#293737=CARTESIAN_POINT('Ctrl Pts',(11.8525709468448,6.83504912565561,2.45270210592386));
#293738=CARTESIAN_POINT('Ctrl Pts',(12.08095445666,6.95793566212947,-0.667352081631377));
#293739=CARTESIAN_POINT('Ctrl Pts',(11.8943164326147,7.01790521951554,-2.21814033602071));
#293740=CARTESIAN_POINT('Ctrl Pts',(10.9355322908033,7.14400747227379,-5.18446093676301));
#293741=CARTESIAN_POINT('Ctrl Pts',(10.1642396821313,7.20480980455327,-6.56906772064067));
#293742=CARTESIAN_POINT('Ctrl Pts',(8.13411242723517,7.32810843972088,-8.96059155792173));
#293743=CARTESIAN_POINT('Ctrl Pts',(6.89564370264464,7.39204706166707,-9.94514742218858));
#293744=CARTESIAN_POINT('Ctrl Pts',(4.12786880580135,7.51658356185018,-11.3734491135158));
#293745=CARTESIAN_POINT('Ctrl Pts',(2.62837697546685,7.57492991794071,-11.8104294769704));
#293746=CARTESIAN_POINT('Ctrl Pts',(-0.497141444118381,7.70135979382401,
-12.0947944144799));
#293747=CARTESIAN_POINT('Ctrl Pts',(-2.09458678244572,7.76597781513833,
-11.9224256637474));
#293748=CARTESIAN_POINT('Ctrl Pts',(-5.09375598834702,7.88729675796684,
-10.9758080629586));
#293749=CARTESIAN_POINT('Ctrl Pts',(-6.47088121212119,7.94990729844587,
-10.2246305765451));
#293750=CARTESIAN_POINT('Ctrl Pts',(-8.86418498157722,8.07548536384248,
-8.23710693670026));
#293751=CARTESIAN_POINT('Ctrl Pts',(-9.85693654644579,8.13443839020935,
-7.01887152039891));
#293752=CARTESIAN_POINT('Ctrl Pts',(-11.3312440069665,8.25926239558325,
-4.25328081991911));
#293753=CARTESIAN_POINT('Ctrl Pts',(-11.7915756778617,8.32366530262542,
-2.72878980717319));
#293754=CARTESIAN_POINT('Ctrl Pts',(-11.9813435805726,8.40127455381076,
-0.773107190868359));
#293755=CARTESIAN_POINT('Ctrl Pts',(-12.,8.41638721319939,-0.386336973170943));
#293756=CARTESIAN_POINT('Ctrl Pts',(-12.,8.43124999997595,-2.37795894086901E-13));
#293757=CARTESIAN_POINT('Ctrl Pts',(-12.,8.80624999997602,-1.66255897937617E-13));
#293758=CARTESIAN_POINT('Ctrl Pts',(-12.,8.79813272939646,-0.21099688727731));
#293759=CARTESIAN_POINT('Ctrl Pts',(-11.9944351114046,8.7899385956393,-0.422183581457404));
#293760=CARTESIAN_POINT('Ctrl Pts',(-11.8996707215412,8.71977517169762,
-2.21519103619965));
#293761=CARTESIAN_POINT('Ctrl Pts',(-11.5036732986091,8.65520592074364,
-3.76490938631468));
#293762=CARTESIAN_POINT('Ctrl Pts',(-10.1470244217602,8.529518619843,-6.59116981568474));
#293763=CARTESIAN_POINT('Ctrl Pts',(-9.21109500593409,8.47113480593771,
-7.84610328964277));
#293764=CARTESIAN_POINT('Ctrl Pts',(-6.90646045764588,8.3460101749747,-9.93659887528159));
#293765=CARTESIAN_POINT('Ctrl Pts',(-5.55710042579121,8.28252135004021,
-10.7496081664373));
#293766=CARTESIAN_POINT('Ctrl Pts',(-2.60328607266364,8.16039521741785,
-11.8204720961739));
#293767=CARTESIAN_POINT('Ctrl Pts',(-1.02456992343103,8.09769472397751,
-12.0603195299831));
#293768=CARTESIAN_POINT('Ctrl Pts',(2.09978380262065,7.9713119609373,-11.9156091672496));
#293769=CARTESIAN_POINT('Ctrl Pts',(3.6160626052177,7.9124402673541,-11.5462098306494));
#293770=CARTESIAN_POINT('Ctrl Pts',(6.45008849028493,7.78865737076106,-10.2407902300069));
#293771=CARTESIAN_POINT('Ctrl Pts',(7.73626938443166,7.72437371151312,-9.30739278575468));
#293772=CARTESIAN_POINT('Ctrl Pts',(9.86566953124602,7.60000222059313,-7.00738367027481));
#293773=CARTESIAN_POINT('Ctrl Pts',(10.6923002669755,7.54059348651161,-5.66652775660526));
#293774=CARTESIAN_POINT('Ctrl Pts',(11.7827709730715,7.41483685997714,-2.75197877573901));
#293775=CARTESIAN_POINT('Ctrl Pts',(12.0394907776967,7.35318567197567,-1.20719461145544));
#293776=CARTESIAN_POINT('Ctrl Pts',(11.9496282804079,7.23134321534966,1.93072841285107));
#293777=CARTESIAN_POINT('Ctrl Pts',(11.5895883716215,7.16673248183404,3.49320834764535));
#293778=CARTESIAN_POINT('Ctrl Pts',(10.2983163653039,7.0406245189931,6.35164551791823));
#293779=CARTESIAN_POINT('Ctrl Pts',(9.39346694581025,6.98232748347902,7.6263696258289));
#293780=CARTESIAN_POINT('Ctrl Pts',(7.13819304752949,6.85750648206278,9.77203411777655));
#293781=CARTESIAN_POINT('Ctrl Pts',(5.8050507275199,6.79375797518282,10.6182870045464));
#293782=CARTESIAN_POINT('Ctrl Pts',(2.87930693272437,6.67097520571558,11.755403896766));
#293783=CARTESIAN_POINT('Ctrl Pts',(1.31341015214886,6.60937855666803,12.0314204579715));
#293784=CARTESIAN_POINT('Ctrl Pts',(-1.80733124687646,6.48314191532549,
11.963513117834));
#293785=CARTESIAN_POINT('Ctrl Pts',(-3.33260716233041,6.42373824615532,
11.6312428003402));
#293786=CARTESIAN_POINT('Ctrl Pts',(-6.20150430623542,6.30042997321308,
10.3937813234885));
#293787=CARTESIAN_POINT('Ctrl Pts',(-7.51286969343425,6.23600871932628,
9.489260337549));
#293788=CARTESIAN_POINT('Ctrl Pts',(-9.69544983274317,6.111107812912,7.24018078654216));
#293789=CARTESIAN_POINT('Ctrl Pts',(-10.5517032124387,6.05222272741964,
5.92313055806081));
#293790=CARTESIAN_POINT('Ctrl Pts',(-11.7056476605019,5.92746690877289,
3.0552200217429));
#293791=CARTESIAN_POINT('Ctrl Pts',(-12.,5.86528504658153,1.53453195250642));
#293792=CARTESIAN_POINT('Ctrl Pts',(-12.,5.80624999998803,-7.82707232360735E-14));
#293793=CARTESIAN_POINT('Origin',(-8.79029313101884E-14,130.96875,0.));
#293794=CARTESIAN_POINT('',(-12.,2.43125,1.10010189965134E-12));
#293795=CARTESIAN_POINT('',(-12.,2.80625000000003,2.67779262495037E-14));
#293796=CARTESIAN_POINT('',(-12.0000000000001,130.96875,-1.46957615897682E-15));
#293797=CARTESIAN_POINT('Ctrl Pts',(-12.,2.43125,9.00945984483315E-13));
#293798=CARTESIAN_POINT('Ctrl Pts',(-11.9999999999999,2.4911350116956,1.55662558473029));
#293799=CARTESIAN_POINT('Ctrl Pts',(-11.6971144483733,2.55424279958433,
3.09860916496787));
#293800=CARTESIAN_POINT('Ctrl Pts',(-10.5224531068447,2.67950010145453,
5.97282371668433));
#293801=CARTESIAN_POINT('Ctrl Pts',(-9.66497642460032,2.73802981152558,
7.27907409547783));
#293802=CARTESIAN_POINT('Ctrl Pts',(-7.48003477965859,2.86270132352826,
9.51525533049624));
#293803=CARTESIAN_POINT('Ctrl Pts',(-6.16505976325898,2.92713958298818,
10.4155233167743));
#293804=CARTESIAN_POINT('Ctrl Pts',(-3.29116809533114,3.05037514083823,
11.6430521341568));
#293805=CARTESIAN_POINT('Ctrl Pts',(-1.76459319119719,3.10987070600563,
11.9699074843356));
#293806=CARTESIAN_POINT('Ctrl Pts',(1.35558206429589,3.23608444636122,12.0266224287251));
#293807=CARTESIAN_POINT('Ctrl Pts',(2.91959038239198,3.29753272360557,11.7453424601158));
#293808=CARTESIAN_POINT('Ctrl Pts',(5.84114830094354,3.42040855260187,10.5985502603361));
#293809=CARTESIAN_POINT('Ctrl Pts',(7.17184521901149,3.48419233047212,9.74744812198967));
#293810=CARTESIAN_POINT('Ctrl Pts',(9.41981206730866,3.60896520534576,7.59375046821348));
#293811=CARTESIAN_POINT('Ctrl Pts',(10.3200940077531,3.66726291054294,6.31613384843947));
#293812=CARTESIAN_POINT('Ctrl Pts',(11.601699280568,3.79342956421014,3.453030181618));
#293813=CARTESIAN_POINT('Ctrl Pts',(11.9564118807405,3.85804339370619,1.88873882372495));
#293814=CARTESIAN_POINT('Ctrl Pts',(12.0351273056935,3.97979581503355,-1.25046576458793));
#293815=CARTESIAN_POINT('Ctrl Pts',(11.7727578542884,4.04160719230054,-2.7947425831598));
#293816=CARTESIAN_POINT('Ctrl Pts',(10.6716949431582,4.16733332880825,-5.70505740316497));
#293817=CARTESIAN_POINT('Ctrl Pts',(9.84062591668189,4.22665346776733,-7.0423630525007));
#293818=CARTESIAN_POINT('Ctrl Pts',(7.7032573569002,4.35110634929211,-9.33482775429073));
#293819=CARTESIAN_POINT('Ctrl Pts',(6.41328493131931,4.41541278903545,-10.2639647164412));
#293820=CARTESIAN_POINT('Ctrl Pts',(3.57400587694271,4.53912779617043,-11.5592986217982));
#293821=CARTESIAN_POINT('Ctrl Pts',(2.05637948023744,4.59806770267168,-11.9231780273746));
#293822=CARTESIAN_POINT('Ctrl Pts',(-1.06746740839951,4.7244299637078,-12.0564638092353));
#293823=CARTESIAN_POINT('Ctrl Pts',(-2.64429244292222,4.78695690058136,
-11.8112304892412));
#293824=CARTESIAN_POINT('Ctrl Pts',(-5.59400321749938,4.90918267913456,
-10.730527510895));
#293825=CARTESIAN_POINT('Ctrl Pts',(-6.94101277916468,4.9727120522437,-9.91257768011027));
#293826=CARTESIAN_POINT('Ctrl Pts',(-9.23839107840673,5.0977944387425,-7.81387146280667));
#293827=CARTESIAN_POINT('Ctrl Pts',(-10.1697260942533,5.15615539903364,
-6.55600029274628));
#293828=CARTESIAN_POINT('Ctrl Pts',(-11.5167551841335,5.28190720769102,
-3.72493741785824));
#293829=CARTESIAN_POINT('Ctrl Pts',(-11.9074700526976,5.34648482152274,
-2.17328528068706));
#293830=CARTESIAN_POINT('Ctrl Pts',(-11.9951611270702,5.4160444741397,-0.393673742057767));
#293831=CARTESIAN_POINT('Ctrl Pts',(-12.,5.42368073729527,-0.196752202786124));
#293832=CARTESIAN_POINT('Ctrl Pts',(-12.,5.43124999998796,-1.03528297046296E-13));
#293833=CARTESIAN_POINT('Ctrl Pts',(-12.,5.80624999998803,-7.73410487064402E-14));
#293834=CARTESIAN_POINT('Ctrl Pts',(-12.,5.80549759002151,-0.0195578254213006));
#293835=CARTESIAN_POINT('Ctrl Pts',(-11.9999521864408,5.80474449763365,
-0.0391178538336524));
#293836=CARTESIAN_POINT('Ctrl Pts',(-11.9920734110103,5.74266205787834,
-1.65030248185612));
#293837=CARTESIAN_POINT('Ctrl Pts',(-11.6677074305612,5.67804533094413,
-3.22452936898916));
#293838=CARTESIAN_POINT('Ctrl Pts',(-10.4410870423967,5.55156184943048,
-6.11373419643874));
#293839=CARTESIAN_POINT('Ctrl Pts',(-9.56665307445172,5.49319551600094,
-7.40764685647228));
#293840=CARTESIAN_POINT('Ctrl Pts',(-7.36028372895381,5.36871167674947,
-9.60644215951102));
#293841=CARTESIAN_POINT('Ctrl Pts',(-6.04371840307873,5.30474224885963,
-10.4848029251598));
#293842=CARTESIAN_POINT('Ctrl Pts',(-3.14613399240567,5.18135627761357,
-11.686047639939));
#293843=CARTESIAN_POINT('Ctrl Pts',(-1.59282846915494,5.12068126502382,
-11.9968676396392));
#293844=CARTESIAN_POINT('Ctrl Pts',(1.52398198989469,4.99460363354349,-12.0030430608051));
#293845=CARTESIAN_POINT('Ctrl Pts',(3.05779876832007,4.93452404342637,-11.7066358305338));
#293846=CARTESIAN_POINT('Ctrl Pts',(5.95934066276901,4.81171360655184,-10.5350442308914));
#293847=CARTESIAN_POINT('Ctrl Pts',(7.29430552357991,4.74719414830042,-9.65887480657748));
#293848=CARTESIAN_POINT('Ctrl Pts',(9.52730421974323,4.62182194640091,-7.4593684697147));
#293849=CARTESIAN_POINT('Ctrl Pts',(10.4116643536932,4.56328345421739,-6.16513701376164));
#293850=CARTESIAN_POINT('Ctrl Pts',(11.6400712060169,4.43797205030929,-3.30697913166894));
#293851=CARTESIAN_POINT('Ctrl Pts',(11.9706775872629,4.37468461963252,-1.76933303656079));
#293852=CARTESIAN_POINT('Ctrl Pts',(12.0260930463176,4.25304071884541,1.37462133271613));
#293853=CARTESIAN_POINT('Ctrl Pts',(11.7392589524117,4.18947265612799,2.95074082568823));
#293854=CARTESIAN_POINT('Ctrl Pts',(10.5838743001801,4.06299857987467,5.86284707047165));
#293855=CARTESIAN_POINT('Ctrl Pts',(9.74108044214217,4.00439854555643,7.17654303706032));
#293856=CARTESIAN_POINT('Ctrl Pts',(7.58617056509479,3.88030643972879,9.42969050622614));
#293857=CARTESIAN_POINT('Ctrl Pts',(6.28756241453168,3.81614198603421,10.340969693975));
#293858=CARTESIAN_POINT('Ctrl Pts',(3.41996284795624,3.69216948565523,11.608153535125));
#293859=CARTESIAN_POINT('Ctrl Pts',(1.8797807380391,3.63228872813482,11.9545718356335));
#293860=CARTESIAN_POINT('Ctrl Pts',(-1.23255864397486,3.50639195551972,
12.0367037164367));
#293861=CARTESIAN_POINT('Ctrl Pts',(-2.77499211667185,3.44545490694412,
11.7771214706575));
#293862=CARTESIAN_POINT('Ctrl Pts',(-5.70898826801489,3.32319473827851,
10.6733427728421));
#293863=CARTESIAN_POINT('Ctrl Pts',(-7.0674193640055,3.25860953229914,9.82670660028009));
#293864=CARTESIAN_POINT('Ctrl Pts',(-9.35119537620759,3.13279401741017,
7.67844416870611));
#293865=CARTESIAN_POINT('Ctrl Pts',(-10.2639133847422,3.07445243231789,
6.40745149139112));
#293866=CARTESIAN_POINT('Ctrl Pts',(-11.5600103262491,2.94941321380034,
3.57836252406713));
#293867=CARTESIAN_POINT('Ctrl Pts',(-11.9270998194105,2.88584404053605,
2.04524701332363));
#293868=CARTESIAN_POINT('Ctrl Pts',(-11.9967384171378,2.81872422872653,
0.323190056187629));
#293869=CARTESIAN_POINT('Ctrl Pts',(-12.,2.81246434007284,0.161532919100313));
#293870=CARTESIAN_POINT('Ctrl Pts',(-12.,2.80625000000003,5.24927323830582E-14));
#293871=CARTESIAN_POINT('Origin',(-8.79029313101884E-14,130.96875,0.));
#293872=CARTESIAN_POINT('',(-8.46872171229246,2.43125,-8.50180878165034));
#293873=CARTESIAN_POINT('Ctrl Pts',(-12.,2.80625000000003,5.77315972805081E-14));
#293874=CARTESIAN_POINT('Ctrl Pts',(-12.,2.75181214583704,-1.41503448306261));
#293875=CARTESIAN_POINT('Ctrl Pts',(-11.7497034409074,2.69462147714694,
-2.82029817695595));
#293876=CARTESIAN_POINT('Ctrl Pts',(-10.9573405555813,2.60202148529659,
-4.96984876681417));
#293877=CARTESIAN_POINT('Ctrl Pts',(-10.5667212506353,2.56697606517402,
-5.75388464177398));
#293878=CARTESIAN_POINT('Ctrl Pts',(-9.6267115219977,2.49896581374268,-7.21628658515935));
#293879=CARTESIAN_POINT('Ctrl Pts',(-9.08163925424091,2.46582425285662,
-7.89127657272241));
#293880=CARTESIAN_POINT('Ctrl Pts',(-8.4687217122924,2.43125000000001,-8.50180878165037));
#293881=CARTESIAN_POINT('Origin',(-1.38777878078145E-14,2.43125000000001,
0.));
#293882=CARTESIAN_POINT('Origin',(-4.54192801987171E-14,57.2,0.));
#293883=CARTESIAN_POINT('',(-11.251117508365,58.9988824916351,-9.57071644917375E-15));
#293884=CARTESIAN_POINT('Ctrl Pts',(9.41568944744522,58.25,-7.43940805637572));
#293885=CARTESIAN_POINT('Ctrl Pts',(8.79573603498597,58.2739415406423,-8.18543385222336));
#293886=CARTESIAN_POINT('Ctrl Pts',(8.08700707828182,58.2986811839343,-8.85294058875071));
#293887=CARTESIAN_POINT('Ctrl Pts',(6.53424618639461,58.348352376611,-9.99336249557727));
#293888=CARTESIAN_POINT('Ctrl Pts',(5.6978562173087,58.3730962739907,-10.4646913423123));
#293889=CARTESIAN_POINT('Ctrl Pts',(4.21229181931588,58.4139168883336,-11.0803254365483));
#293890=CARTESIAN_POINT('Ctrl Pts',(3.58715467640316,58.4299857748698,-11.281544084094));
#293891=CARTESIAN_POINT('Ctrl Pts',(1.45628305848908,58.4851817311957,-11.7744414883963));
#293892=CARTESIAN_POINT('Ctrl Pts',(-0.090158574616811,58.5256317479014,
-11.8236949834757));
#293893=CARTESIAN_POINT('Ctrl Pts',(-3.02394526826764,58.6031803869245,
-11.3392745716886));
#293894=CARTESIAN_POINT('Ctrl Pts',(-4.49506113981352,58.6411124276446,
-10.8282548234504));
#293895=CARTESIAN_POINT('Ctrl Pts',(-7.12494968894065,58.723324568187,-9.17826743218203));
#293896=CARTESIAN_POINT('Ctrl Pts',(-8.20553019239892,58.7626401442854,
-8.17129870321612));
#293897=CARTESIAN_POINT('Ctrl Pts',(-10.0520993471377,58.8433462973028,
-5.64304338821277));
#293898=CARTESIAN_POINT('Ctrl Pts',(-10.6336060765998,58.8835565622676,
-4.23613498781373));
#293899=CARTESIAN_POINT('Ctrl Pts',(-11.1741358391133,58.9468224589001,
-1.96620905423901));
#293900=CARTESIAN_POINT('Ctrl Pts',(-11.2766767876284,58.9733232123716,
-0.982555718105193));
#293901=CARTESIAN_POINT('Ctrl Pts',(-11.251117508365,58.9988824916351,1.77635683940025E-14));
#293902=CARTESIAN_POINT('',(-13.05,57.2,-1.59816407288729E-15));
#293903=CARTESIAN_POINT('',(-13.05,57.2,-1.59816407288729E-15));
#293904=CARTESIAN_POINT('Origin',(-4.54192801987171E-14,57.2,0.));
#293905=CARTESIAN_POINT('',(6.83270577527258,60.1985571585059,-7.37194919844001));
#293906=CARTESIAN_POINT('Ctrl Pts',(-11.251117508365,58.9988824916351,3.27515792264421E-14));
#293907=CARTESIAN_POINT('Ctrl Pts',(-11.2385726688954,59.0114273311046,
0.482251616975299));
#293908=CARTESIAN_POINT('Ctrl Pts',(-11.1947127197006,59.0242689258418,
0.964213182637807));
#293909=CARTESIAN_POINT('Ctrl Pts',(-10.895798509458,59.0761575489079,2.86503292607173));
#293910=CARTESIAN_POINT('Ctrl Pts',(-10.3986941703556,59.1162399397277,
4.23081678926045));
#293911=CARTESIAN_POINT('Ctrl Pts',(-9.28561894190705,59.1748510495143,
6.07866846337327));
#293912=CARTESIAN_POINT('Ctrl Pts',(-8.85456618599315,59.1937120748971,
6.66018982610041));
#293913=CARTESIAN_POINT('Ctrl Pts',(-7.40967389241113,59.2520150973381,
8.25170914496314));
#293914=CARTESIAN_POINT('Ctrl Pts',(-6.25222753197104,59.2923785121678,
9.11138079427429));
#293915=CARTESIAN_POINT('Ctrl Pts',(-3.74760729768966,59.369570655975,10.3028052876729));
#293916=CARTESIAN_POINT('Ctrl Pts',(-2.34928610066821,59.4075104184351,
10.6948750747753));
#293917=CARTESIAN_POINT('Ctrl Pts',(0.779711812100376,59.4964841752171,
10.8441374514475));
#293918=CARTESIAN_POINT('Ctrl Pts',(2.19507014871295,59.5372684261364,10.5537953412713));
#293919=CARTESIAN_POINT('Ctrl Pts',(4.5699429723945,59.6064277448452,9.70309149882849));
#293920=CARTESIAN_POINT('Ctrl Pts',(5.72066828246454,59.6447411400348,9.02739600905606));
#293921=CARTESIAN_POINT('Ctrl Pts',(7.76853464378474,59.7237483857297,7.23875024917893));
#293922=CARTESIAN_POINT('Ctrl Pts',(8.63524372650229,59.7622453507951,6.1148459525091));
#293923=CARTESIAN_POINT('Ctrl Pts',(9.83658164315294,59.8417129538795,3.65453270819226));
#293924=CARTESIAN_POINT('Ctrl Pts',(10.1857205813106,59.8816061800705,2.35290905826649));
#293925=CARTESIAN_POINT('Ctrl Pts',(10.3729006217155,59.9595796521074,-0.320720838433725));
#293926=CARTESIAN_POINT('Ctrl Pts',(10.205314917492,59.9976670280176,-1.66555307451394));
#293927=CARTESIAN_POINT('Ctrl Pts',(9.49559971070312,60.0651115369737,-3.78971049737241));
#293928=CARTESIAN_POINT('Ctrl Pts',(9.1027240403221,60.0920685051517,-4.59569513239433));
#293929=CARTESIAN_POINT('Ctrl Pts',(8.11140739263744,60.1450250918943,-6.09351276754362));
#293930=CARTESIAN_POINT('Ctrl Pts',(7.51526380442641,60.1710414084933,-6.77683587343302));
#293931=CARTESIAN_POINT('Ctrl Pts',(6.83270577527257,60.1985571585058,-7.37194919844003));
#293932=CARTESIAN_POINT('',(-0.358381257737887,60.1985571585059,-10.0450518201713));
#293933=CARTESIAN_POINT('Origin',(-8.10462807976364E-14,60.1985571585057,
6.21724893790088E-14));
#293934=CARTESIAN_POINT('Ctrl Pts',(-0.358381257737859,60.1985571585059,
-10.0450518201713));
#293935=CARTESIAN_POINT('Ctrl Pts',(0.569600497855516,60.0920908389641,
-10.1846938468385));
#293936=CARTESIAN_POINT('Ctrl Pts',(1.86768826672467,59.9489768555399,-10.2622313963477));
#293937=CARTESIAN_POINT('Ctrl Pts',(4.82229184539531,59.6316500051715,-9.5602844533037));
#293938=CARTESIAN_POINT('Ctrl Pts',(6.09703360509207,59.4828126471393,-8.98125348648291));
#293939=CARTESIAN_POINT('Ctrl Pts',(8.64359555920175,59.1568934783279,-7.16524174281715));
#293940=CARTESIAN_POINT('Ctrl Pts',(9.58558008715325,59.0150265477672,-5.97673601271509));
#293941=CARTESIAN_POINT('Ctrl Pts',(10.7798566334032,58.7884331321821,-4.04272726160383));
#293942=CARTESIAN_POINT('Ctrl Pts',(11.2179091250566,58.6795346125953,-3.03593820382734));
#293943=CARTESIAN_POINT('Ctrl Pts',(11.8513180753988,58.4474576877315,-0.725960973686208));
#293944=CARTESIAN_POINT('Ctrl Pts',(11.9400790733319,58.3432212931802,0.43745433545044));
#293945=CARTESIAN_POINT('Ctrl Pts',(11.9139873655789,58.25,1.43419142823615));
#293946=CARTESIAN_POINT('Origin',(-8.79029313101884E-14,130.96875,0.));
#293947=CARTESIAN_POINT('',(-4.83831102398129,130.817307158506,8.81034900733485));
#293948=CARTESIAN_POINT('',(-10.3754400975249,130.493309902475,-3.34148109778276E-15));
#293949=CARTESIAN_POINT('Ctrl Pts',(-10.3754400975249,130.493309902475,
-4.85722573273506E-15));
#293950=CARTESIAN_POINT('Ctrl Pts',(-10.3638450429889,130.504904957011,
0.411047722935234));
#293951=CARTESIAN_POINT('Ctrl Pts',(-10.3275450278176,130.516761565068,
0.822042306381597));
#293952=CARTESIAN_POINT('Ctrl Pts',(-10.0721499446089,130.567155272434,
2.52967838917212));
#293953=CARTESIAN_POINT('Ctrl Pts',(-9.63043563877547,130.606815619881,
3.77975573956643));
#293954=CARTESIAN_POINT('Ctrl Pts',(-8.47232889963708,130.674443677503,
5.75246532316119));
#293955=CARTESIAN_POINT('Ctrl Pts',(-7.85961320778648,130.702096724505,
6.52278639205452));
#293956=CARTESIAN_POINT('Ctrl Pts',(-6.45488736456084,130.759774236249,
7.83679328916589));
#293957=CARTESIAN_POINT('Ctrl Pts',(-5.67876562648238,130.788661778153,
8.38148366250018));
#293958=CARTESIAN_POINT('Ctrl Pts',(-4.83831102398136,130.817307158506,
8.81034900733487));
#293959=CARTESIAN_POINT('',(2.81735069959344,130.817307158506,9.64852518426128));
#293960=CARTESIAN_POINT('Origin',(1.77635683940025E-14,130.817307158505,
-7.7715611723761E-13));
#293961=CARTESIAN_POINT('Ctrl Pts',(-11.894167785564,128.86875,1.59021152330507));
#293962=CARTESIAN_POINT('Ctrl Pts',(-11.6160944182043,128.984669600074,
2.79534433683652));
#293963=CARTESIAN_POINT('Ctrl Pts',(-11.1495590589446,129.104808940769,
3.9486436044955));
#293964=CARTESIAN_POINT('Ctrl Pts',(-9.99474123522102,129.322681085237,
5.86611791592308));
#293965=CARTESIAN_POINT('Ctrl Pts',(-9.24106914132451,129.438710702818,
6.87629466505421));
#293966=CARTESIAN_POINT('Ctrl Pts',(-7.60212862518274,129.653506500676,
8.27681501381399));
#293967=CARTESIAN_POINT('Ctrl Pts',(-7.00852279237346,129.727188567012,
8.69083371192293));
#293968=CARTESIAN_POINT('Ctrl Pts',(-5.75231106181202,129.87582352063,9.39498084136462));
#293969=CARTESIAN_POINT('Ctrl Pts',(-5.09304579581803,129.9504191299,9.68406859338561));
#293970=CARTESIAN_POINT('Ctrl Pts',(-3.1915580491957,130.156529510499,10.3049448070743));
#293971=CARTESIAN_POINT('Ctrl Pts',(-1.94706281547003,130.282347955964,
10.4821475592344));
#293972=CARTESIAN_POINT('Ctrl Pts',(0.523645534039794,130.552019108861,
10.3725726766803));
#293973=CARTESIAN_POINT('Ctrl Pts',(1.70640129850129,130.686168481297,10.1095352252478));
#293974=CARTESIAN_POINT('Ctrl Pts',(2.8173506995935,130.817307158506,9.64852518426143));
#293975=CARTESIAN_POINT('Ctrl Pts',(-7.30108394240721,128.868749999999,
9.52334884722601));
#293976=CARTESIAN_POINT('Ctrl Pts',(-6.30302171533989,128.90036926442,10.248671949143));
#293977=CARTESIAN_POINT('Ctrl Pts',(-5.19895338212386,128.932055884534,
10.8155858694633));
#293978=CARTESIAN_POINT('Ctrl Pts',(-2.84939595618331,128.993471671357,
11.5949956950555));
#293979=CARTESIAN_POINT('Ctrl Pts',(-1.6294605374271,129.024443351536,11.7964401725797));
#293980=CARTESIAN_POINT('Ctrl Pts',(1.19446780691268,129.097950041924,11.8173195636497));
#293981=CARTESIAN_POINT('Ctrl Pts',(2.66422769795,129.136066177321,11.508354646803));
#293982=CARTESIAN_POINT('Ctrl Pts',(5.36881592504784,129.209269604011,10.4617874232397));
#293983=CARTESIAN_POINT('Ctrl Pts',(6.67010341062351,129.249841492879,9.63525664930798));
#293984=CARTESIAN_POINT('Ctrl Pts',(8.80069211440203,129.327673228521,7.59990649152918));
#293985=CARTESIAN_POINT('Ctrl Pts',(9.71750054011973,129.365467783131,6.36547005128502));
#293986=CARTESIAN_POINT('Ctrl Pts',(10.6671105988966,129.428419178648,4.20075858084496));
#293987=CARTESIAN_POINT('Ctrl Pts',(10.8985785326509,129.448468661738,3.49231250117377));
#293988=CARTESIAN_POINT('Ctrl Pts',(11.3798900320565,129.50832678461,1.32145897720948));
#293989=CARTESIAN_POINT('Ctrl Pts',(11.4183347881864,129.546093788355,-0.181457365732128));
#293990=CARTESIAN_POINT('Ctrl Pts',(11.035404631011,129.605797053053,-2.36908459971864));
#293991=CARTESIAN_POINT('Ctrl Pts',(10.838193172437,129.625864165925,-3.07808845028999));
#293992=CARTESIAN_POINT('Ctrl Pts',(10.0527919462299,129.685481946684,-5.10722353689452));
#293993=CARTESIAN_POINT('Ctrl Pts',(9.27574806257917,129.723282730156,-6.34546975494142));
#293994=CARTESIAN_POINT('Ctrl Pts',(7.30265479182673,129.801149008045,-8.43888275379305));
#293995=CARTESIAN_POINT('Ctrl Pts',(6.12615848216244,129.84141096262,-9.28030131521465));
#293996=CARTESIAN_POINT('Ctrl Pts',(3.51132031891206,129.92061366261,-10.4691433409554));
#293997=CARTESIAN_POINT('Ctrl Pts',(2.09323021142943,129.958633060114,-10.8045158956757));
#293998=CARTESIAN_POINT('Ctrl Pts',(-0.910552320525702,130.043534699612,
-10.898914083415));
#293999=CARTESIAN_POINT('Ctrl Pts',(-2.33181430589621,130.083835312678,
-10.6070904248003));
#294000=CARTESIAN_POINT('Ctrl Pts',(-4.77795410356712,130.155467557091,
-9.68150441188508));
#294001=CARTESIAN_POINT('Ctrl Pts',(-5.92816571815587,130.194022804729,
-8.97732226984948));
#294002=CARTESIAN_POINT('Ctrl Pts',(-7.89717510050072,130.270679844274,
-7.19030195250223));
#294003=CARTESIAN_POINT('Ctrl Pts',(-8.77341371877538,130.308974063784,
-6.06403251894919));
#294004=CARTESIAN_POINT('Ctrl Pts',(-9.9732821988043,130.391291620567,-3.48310903998621));
#294005=CARTESIAN_POINT('Ctrl Pts',(-10.300207709712,130.431340575298,-2.16021817703969));
#294006=CARTESIAN_POINT('Ctrl Pts',(-10.3801921577127,130.477950105763,
-0.541661562394141));
#294007=CARTESIAN_POINT('Ctrl Pts',(-10.383079668429,130.485670331571,-0.270824791260495));
#294008=CARTESIAN_POINT('Ctrl Pts',(-10.3754400975249,130.493309902475,
4.42701431069281E-14));
#294009=CARTESIAN_POINT('',(-9.9000000000001,130.96875,-1.21240033115588E-15));
#294010=CARTESIAN_POINT('',(-9.9000000000001,130.96875,-1.21240033115588E-15));
#294011=CARTESIAN_POINT('Origin',(-8.79029313101884E-14,130.96875,0.));
#294012=CARTESIAN_POINT('Origin',(-8.79029313101884E-14,130.96875,0.));
#294013=CARTESIAN_POINT('',(11.6184932898974,91.186,3.00176842421407));
#294014=CARTESIAN_POINT('Ctrl Pts',(-12.0000000000001,92.80624999964,-3.4555691641458E-14));
#294015=CARTESIAN_POINT('Ctrl Pts',(-12.0000000000001,92.7882122178229,
-0.468866447099216));
#294016=CARTESIAN_POINT('Ctrl Pts',(-11.972521673645,92.769811805124,-0.938230718020533));
#294017=CARTESIAN_POINT('Ctrl Pts',(-11.733006065977,92.6886980402866,-2.96884416604449));
#294018=CARTESIAN_POINT('Ctrl Pts',(-11.2428649939964,92.6244138443026,
-4.48056379236747));
#294019=CARTESIAN_POINT('Ctrl Pts',(-9.71367031873571,92.5000404579741,
-7.21660735543917));
#294020=CARTESIAN_POINT('Ctrl Pts',(-8.69399354379183,92.440633818221,-8.41719962742405));
#294021=CARTESIAN_POINT('Ctrl Pts',(-6.25923585411257,92.3148778940627,
-10.3551473117068));
#294022=CARTESIAN_POINT('Ctrl Pts',(-4.8694412051415,92.2532230340454,-11.0767878398891));
#294023=CARTESIAN_POINT('Ctrl Pts',(-1.85738137910691,92.1313826546791,
-11.9612501088246));
#294024=CARTESIAN_POINT('Ctrl Pts',(-0.260114213238191,92.0667718405922,
-12.1017951164519));
#294025=CARTESIAN_POINT('Ctrl Pts',(2.85747996146335,91.9406625071477,-11.7572747332122));
#294026=CARTESIAN_POINT('Ctrl Pts',(4.34945959390987,91.8823654951006,-11.2907447234468));
#294027=CARTESIAN_POINT('Ctrl Pts',(7.08715085155504,91.7575455999654,-9.80911729155921));
#294028=CARTESIAN_POINT('Ctrl Pts',(8.30403841759875,91.6937962665103,-8.80281869876389));
#294029=CARTESIAN_POINT('Ctrl Pts',(10.289789073564,91.5710113283916,-6.37182103468252));
#294030=CARTESIAN_POINT('Ctrl Pts',(11.0362878674002,91.5094181611936,-4.96793793338489));
#294031=CARTESIAN_POINT('Ctrl Pts',(11.8058222286519,91.4014840499907,-2.41238131425744));
#294032=CARTESIAN_POINT('Ctrl Pts',(11.976544227546,91.3575745868965,-1.32648830144042));
#294033=CARTESIAN_POINT('Ctrl Pts',(12.0188779046423,91.2730160899065,0.85773434553886));
#294034=CARTESIAN_POINT('Ctrl Pts',(11.8913002682865,91.2300321596809,1.94585550891945));
#294035=CARTESIAN_POINT('Ctrl Pts',(11.6184932898973,91.186,3.00176842421425));
#294036=CARTESIAN_POINT('',(10.3435570531169,91.185999999999,-6.08365247930179));
#294037=CARTESIAN_POINT('Origin',(-6.49919226343618E-14,91.186,0.));
#294038=CARTESIAN_POINT('Ctrl Pts',(10.343557053117,91.185999999999,-6.08365247930161));
#294039=CARTESIAN_POINT('Ctrl Pts',(9.55890855690799,91.2471314138738,-7.41772876238869));
#294040=CARTESIAN_POINT('Ctrl Pts',(8.52353606068608,91.3064930697652,-8.58747742168945));
#294041=CARTESIAN_POINT('Ctrl Pts',(6.06330327988208,91.4317877484173,-10.4709623620909));
#294042=CARTESIAN_POINT('Ctrl Pts',(4.66089813768456,91.4927127095218,-11.1660411123352));
#294043=CARTESIAN_POINT('Ctrl Pts',(1.65780900183523,91.6141902168476,-11.9872326559139));
#294044=CARTESIAN_POINT('Ctrl Pts',(0.0843670061797239,91.6778372825548,
-12.101022716674));
#294045=CARTESIAN_POINT('Ctrl Pts',(-3.00455409179326,91.8027867656814,
-11.7206623108048));
#294046=CARTESIAN_POINT('Ctrl Pts',(-4.49136392438059,91.8610998850578,
-11.2351643727108));
#294047=CARTESIAN_POINT('Ctrl Pts',(-7.23010729887462,91.9870412753891,
-9.70781666209722));
#294048=CARTESIAN_POINT('Ctrl Pts',(-8.44866993703788,92.0516394256888,
-8.66812365438208));
#294049=CARTESIAN_POINT('Ctrl Pts',(-10.3885381900297,92.1737257864082,
-6.20335539022936));
#294050=CARTESIAN_POINT('Ctrl Pts',(-11.1022697317196,92.2349539470959,
-4.8107460550984));
#294051=CARTESIAN_POINT('Ctrl Pts',(-11.8428241618736,92.343137182588,-2.23929765448896));
#294052=CARTESIAN_POINT('Ctrl Pts',(-12.0000000000001,92.3881104835417,
-1.1213502773074));
#294053=CARTESIAN_POINT('Ctrl Pts',(-12.0000000000001,92.43124999964,1.0547118733939E-14));
#294054=CARTESIAN_POINT('Ctrl Pts',(-10.0514428414942,-1.69374999998275,
2.46189346052968E-15));
#294055=CARTESIAN_POINT('Ctrl Pts',(-10.0514428414942,-1.54374999998335,
3.26591175476071));
#294056=CARTESIAN_POINT('Ctrl Pts',(-8.1317880767572,-1.39374999998395,
5.90808986649102));
#294057=CARTESIAN_POINT('Ctrl Pts',(-6.21213331202023,-1.24374999998455,
8.55026797822134));
#294058=CARTESIAN_POINT('Ctrl Pts',(-3.10606665601012,-1.09374999998515,
9.5594902125713));
#294059=CARTESIAN_POINT('Ctrl Pts',(-9.99267389681068E-15,-0.943749999985747,
10.5687124469213));
#294060=CARTESIAN_POINT('Ctrl Pts',(3.1060666560101,-0.793749999986346,
9.5594902125713));
#294061=CARTESIAN_POINT('Ctrl Pts',(6.21213331202021,-0.643749999986944,
8.55026797822134));
#294062=CARTESIAN_POINT('Ctrl Pts',(8.13178807675718,-0.493749999987543,
5.90808986649102));
#294063=CARTESIAN_POINT('Ctrl Pts',(10.0514428414942,-0.343749999988142,
3.2659117547607));
#294064=CARTESIAN_POINT('Ctrl Pts',(10.0514428414942,-0.193749999988742,
-1.23094673026484E-15));
#294065=CARTESIAN_POINT('Ctrl Pts',(10.0514428414942,-0.0437499999893418,
-3.26591175476071));
#294066=CARTESIAN_POINT('Ctrl Pts',(8.13178807675718,0.106250000010057,
-5.90808986649102));
#294067=CARTESIAN_POINT('Ctrl Pts',(6.2121333120202,0.256250000009456,-8.55026797822134));
#294068=CARTESIAN_POINT('Ctrl Pts',(3.10606665601009,0.406250000008854,
-9.5594902125713));
#294069=CARTESIAN_POINT('Ctrl Pts',(-1.34451165064878E-14,0.556250000008252,
-10.5687124469213));
#294070=CARTESIAN_POINT('Ctrl Pts',(-3.10606665601012,0.70625000000765,
-9.5594902125713));
#294071=CARTESIAN_POINT('Ctrl Pts',(-6.21213331202023,0.856250000007049,
-8.55026797822134));
#294072=CARTESIAN_POINT('Ctrl Pts',(-8.1317880767572,1.00625000000645,-5.90808986649102));
#294073=CARTESIAN_POINT('Ctrl Pts',(-10.0514428414942,1.15625000000585,
-3.2659117547607));
#294074=CARTESIAN_POINT('Ctrl Pts',(-10.0514428414942,1.30625000000525,
2.46189346052968E-15));
#294075=CARTESIAN_POINT('Ctrl Pts',(-10.0514428414942,1.45625000000465,
3.26591175476071));
#294076=CARTESIAN_POINT('Ctrl Pts',(-8.1317880767572,1.60625000000405,5.90808986649102));
#294077=CARTESIAN_POINT('Ctrl Pts',(-6.21213331202023,1.75625000000345,
8.55026797822134));
#294078=CARTESIAN_POINT('Ctrl Pts',(-3.10606665601012,1.90625000000285,
9.5594902125713));
#294079=CARTESIAN_POINT('Ctrl Pts',(-1.17203831684725E-14,2.05625000000225,
10.5687124469213));
#294080=CARTESIAN_POINT('Ctrl Pts',(3.1060666560101,2.20625000000165,9.5594902125713));
#294081=CARTESIAN_POINT('Ctrl Pts',(6.2121333120202,2.35625000000106,8.55026797822134));
#294082=CARTESIAN_POINT('Ctrl Pts',(8.13178807675718,2.50625000000046,5.90808986649102));
#294083=CARTESIAN_POINT('Ctrl Pts',(10.0514428414942,2.65624999999986,3.2659117547607));
#294084=CARTESIAN_POINT('Ctrl Pts',(10.0514428414942,2.80624999999926,-1.23094673026484E-15));
#294085=CARTESIAN_POINT('Ctrl Pts',(10.0514428414942,2.95624999999866,-3.26591175476071));
#294086=CARTESIAN_POINT('Ctrl Pts',(8.13178807675718,3.10624999999806,-5.90808986649102));
#294087=CARTESIAN_POINT('Ctrl Pts',(6.2121333120202,3.25624999999746,-8.55026797822134));
#294088=CARTESIAN_POINT('Ctrl Pts',(3.10606665601009,3.40624999999685,-9.5594902125713));
#294089=CARTESIAN_POINT('Ctrl Pts',(-1.51728257781496E-14,3.55624999999625,
-10.5687124469213));
#294090=CARTESIAN_POINT('Ctrl Pts',(-3.10606665601012,3.70624999999565,
-9.5594902125713));
#294091=CARTESIAN_POINT('Ctrl Pts',(-6.21213331202023,3.85624999999505,
-8.55026797822134));
#294092=CARTESIAN_POINT('Ctrl Pts',(-8.13178807675721,4.00624999999445,
-5.90808986649102));
#294093=CARTESIAN_POINT('Ctrl Pts',(-10.0514428414942,4.15624999999385,
-3.2659117547607));
#294094=CARTESIAN_POINT('Ctrl Pts',(-10.0514428414942,4.30624999999325,
2.46189346052968E-15));
#294095=CARTESIAN_POINT('Ctrl Pts',(-10.0514428414942,4.45624999999265,
3.26591175476071));
#294096=CARTESIAN_POINT('Ctrl Pts',(-8.13178807675721,4.60624999999205,
5.90808986649102));
#294097=CARTESIAN_POINT('Ctrl Pts',(-6.21213331202023,4.75624999999145,
8.55026797822134));
#294098=CARTESIAN_POINT('Ctrl Pts',(-3.10606665601012,4.90624999999085,
9.5594902125713));
#294099=CARTESIAN_POINT('Ctrl Pts',(-1.34480924401344E-14,5.05624999999025,
10.5687124469213));
#294100=CARTESIAN_POINT('Ctrl Pts',(3.10606665601009,5.20624999998966,9.5594902125713));
#294101=CARTESIAN_POINT('Ctrl Pts',(6.2121333120202,5.35624999998906,8.55026797822134));
#294102=CARTESIAN_POINT('Ctrl Pts',(8.13178807675718,5.50624999998846,5.90808986649102));
#294103=CARTESIAN_POINT('Ctrl Pts',(10.0514428414942,5.65624999998786,3.2659117547607));
#294104=CARTESIAN_POINT('Ctrl Pts',(10.0514428414941,5.80624999998726,-1.23094673026484E-15));
#294105=CARTESIAN_POINT('Ctrl Pts',(10.0514428414941,5.95624999998666,-3.26591175476071));
#294106=CARTESIAN_POINT('Ctrl Pts',(8.13178807675717,6.10624999998606,-5.90808986649102));
#294107=CARTESIAN_POINT('Ctrl Pts',(6.2121333120202,6.25624999998545,-8.55026797822134));
#294108=CARTESIAN_POINT('Ctrl Pts',(3.10606665601009,6.40624999998485,-9.5594902125713));
#294109=CARTESIAN_POINT('Ctrl Pts',(-1.69005350498115E-14,6.55624999998425,
-10.5687124469213));
#294110=CARTESIAN_POINT('Ctrl Pts',(-3.10606665601013,6.70624999998365,
-9.5594902125713));
#294111=CARTESIAN_POINT('Ctrl Pts',(-6.21213331202023,6.85624999998305,
-8.55026797822134));
#294112=CARTESIAN_POINT('Ctrl Pts',(-8.13178807675721,7.00624999998245,
-5.90808986649102));
#294113=CARTESIAN_POINT('Ctrl Pts',(-10.0514428414942,7.15624999998184,
-3.2659117547607));
#294114=CARTESIAN_POINT('Ctrl Pts',(-10.0514428414942,7.30624999998125,
2.46189346052968E-15));
#294115=CARTESIAN_POINT('Ctrl Pts',(-10.0514428414942,7.45624999998065,
3.26591175476071));
#294116=CARTESIAN_POINT('Ctrl Pts',(-8.13178807675721,7.60624999998005,
5.90808986649102));
#294117=CARTESIAN_POINT('Ctrl Pts',(-6.21213331202023,7.75624999997945,
8.55026797822134));
#294118=CARTESIAN_POINT('Ctrl Pts',(-3.10606665601012,7.90624999997885,
9.5594902125713));
#294119=CARTESIAN_POINT('Ctrl Pts',(-1.51758017117962E-14,8.05624999997825,
10.5687124469213));
#294120=CARTESIAN_POINT('Ctrl Pts',(3.10606665601009,8.20624999997765,9.5594902125713));
#294121=CARTESIAN_POINT('Ctrl Pts',(6.2121333120202,8.35624999997706,8.55026797822134));
#294122=CARTESIAN_POINT('Ctrl Pts',(8.13178807675717,8.50624999997646,5.90808986649102));
#294123=CARTESIAN_POINT('Ctrl Pts',(10.0514428414942,8.65624999997586,3.2659117547607));
#294124=CARTESIAN_POINT('Ctrl Pts',(10.0514428414941,8.80624999997526,-1.23094673026484E-15));
#294125=CARTESIAN_POINT('Ctrl Pts',(10.0514428414941,8.95624999997466,-3.26591175476071));
#294126=CARTESIAN_POINT('Ctrl Pts',(8.13178807675717,9.10624999997406,-5.90808986649102));
#294127=CARTESIAN_POINT('Ctrl Pts',(6.2121333120202,9.25624999997346,-8.55026797822134));
#294128=CARTESIAN_POINT('Ctrl Pts',(3.10606665601009,9.40624999997286,-9.5594902125713));
#294129=CARTESIAN_POINT('Ctrl Pts',(-1.86282443214733E-14,9.55624999997225,
-10.5687124469213));
#294130=CARTESIAN_POINT('Ctrl Pts',(-3.10606665601013,9.70624999997165,
-9.5594902125713));
#294131=CARTESIAN_POINT('Ctrl Pts',(-6.21213331202023,9.85624999997105,
-8.55026797822134));
#294132=CARTESIAN_POINT('Ctrl Pts',(-8.13178807675721,10.0062499999704,
-5.90808986649102));
#294133=CARTESIAN_POINT('Ctrl Pts',(-10.0514428414942,10.1562499999698,
-3.2659117547607));
#294134=CARTESIAN_POINT('Ctrl Pts',(-10.0514428414942,10.3062499999692,
2.46189346052968E-15));
#294135=CARTESIAN_POINT('Ctrl Pts',(-10.0514428414942,10.4562499999686,
3.26591175476071));
#294136=CARTESIAN_POINT('Ctrl Pts',(-8.13178807675721,10.606249999968,5.90808986649102));
#294137=CARTESIAN_POINT('Ctrl Pts',(-6.21213331202023,10.7562499999674,
8.55026797822134));
#294138=CARTESIAN_POINT('Ctrl Pts',(-3.10606665601013,10.9062499999668,
9.5594902125713));
#294139=CARTESIAN_POINT('Ctrl Pts',(-1.6903510983458E-14,11.0562499999663,
10.5687124469213));
#294140=CARTESIAN_POINT('Ctrl Pts',(3.10606665601009,11.2062499999657,9.5594902125713));
#294141=CARTESIAN_POINT('Ctrl Pts',(6.2121333120202,11.3562499999651,8.55026797822134));
#294142=CARTESIAN_POINT('Ctrl Pts',(8.13178807675717,11.5062499999645,5.90808986649102));
#294143=CARTESIAN_POINT('Ctrl Pts',(10.0514428414941,11.6562499999639,3.2659117547607));
#294144=CARTESIAN_POINT('Ctrl Pts',(10.0514428414941,11.8062499999633,-1.23094673026484E-15));
#294145=CARTESIAN_POINT('Ctrl Pts',(10.0514428414941,11.9562499999627,-3.26591175476071));
#294146=CARTESIAN_POINT('Ctrl Pts',(8.13178807675717,12.1062499999621,-5.90808986649102));
#294147=CARTESIAN_POINT('Ctrl Pts',(6.2121333120202,12.2562499999615,-8.55026797822134));
#294148=CARTESIAN_POINT('Ctrl Pts',(3.10606665601009,12.4062499999609,-9.5594902125713));
#294149=CARTESIAN_POINT('Ctrl Pts',(-2.03559535931351E-14,12.5562499999603,
-10.5687124469213));
#294150=CARTESIAN_POINT('Ctrl Pts',(-3.10606665601013,12.7062499999597,
-9.5594902125713));
#294151=CARTESIAN_POINT('Ctrl Pts',(-6.21213331202024,12.856249999959,-8.55026797822134));
#294152=CARTESIAN_POINT('Ctrl Pts',(-8.13178807675721,13.0062499999584,
-5.90808986649102));
#294153=CARTESIAN_POINT('Ctrl Pts',(-10.0514428414942,13.1562499999578,
-3.2659117547607));
#294154=CARTESIAN_POINT('Ctrl Pts',(-10.0514428414942,13.3062499999572,
2.46189346052968E-15));
#294155=CARTESIAN_POINT('Ctrl Pts',(-10.0514428414942,13.4562499999566,
3.26591175476071));
#294156=CARTESIAN_POINT('Ctrl Pts',(-8.13178807675721,13.606249999956,5.90808986649102));
#294157=CARTESIAN_POINT('Ctrl Pts',(-6.21213331202023,13.7562499999554,
8.55026797822134));
#294158=CARTESIAN_POINT('Ctrl Pts',(-3.10606665601013,13.9062499999549,
9.5594902125713));
#294159=CARTESIAN_POINT('Ctrl Pts',(-1.86312202551199E-14,14.0562499999543,
10.5687124469213));
#294160=CARTESIAN_POINT('Ctrl Pts',(3.10606665601009,14.2062499999537,9.5594902125713));
#294161=CARTESIAN_POINT('Ctrl Pts',(6.2121333120202,14.3562499999531,8.55026797822134));
#294162=CARTESIAN_POINT('Ctrl Pts',(8.13178807675717,14.5062499999525,5.90808986649102));
#294163=CARTESIAN_POINT('Ctrl Pts',(10.0514428414941,14.6562499999519,3.2659117547607));
#294164=CARTESIAN_POINT('Ctrl Pts',(10.0514428414941,14.8062499999513,-1.23094673026484E-15));
#294165=CARTESIAN_POINT('Ctrl Pts',(10.0514428414941,14.9562499999507,-3.26591175476071));
#294166=CARTESIAN_POINT('Ctrl Pts',(8.13178807675717,15.1062499999501,-5.90808986649102));
#294167=CARTESIAN_POINT('Ctrl Pts',(6.21213331202019,15.2562499999495,-8.55026797822134));
#294168=CARTESIAN_POINT('Ctrl Pts',(3.10606665601009,15.4062499999489,-9.5594902125713));
#294169=CARTESIAN_POINT('Ctrl Pts',(-2.2083662864797E-14,15.5562499999482,
-10.5687124469213));
#294170=CARTESIAN_POINT('Ctrl Pts',(-3.10606665601013,15.7062499999477,
-9.5594902125713));
#294171=CARTESIAN_POINT('Ctrl Pts',(-6.21213331202024,15.856249999947,-8.55026797822134));
#294172=CARTESIAN_POINT('Ctrl Pts',(-8.13178807675721,16.0062499999464,
-5.90808986649102));
#294173=CARTESIAN_POINT('Ctrl Pts',(-10.0514428414942,16.1562499999458,
-3.2659117547607));
#294174=CARTESIAN_POINT('Ctrl Pts',(-10.0514428414942,16.3062499999452,
2.46189346052968E-15));
#294175=CARTESIAN_POINT('Ctrl Pts',(-10.0514428414942,16.4562499999446,
3.26591175476071));
#294176=CARTESIAN_POINT('Ctrl Pts',(-8.13178807675721,16.606249999944,5.90808986649102));
#294177=CARTESIAN_POINT('Ctrl Pts',(-6.21213331202024,16.7562499999434,
8.55026797822134));
#294178=CARTESIAN_POINT('Ctrl Pts',(-3.10606665601013,16.9062499999428,
9.5594902125713));
#294179=CARTESIAN_POINT('Ctrl Pts',(-2.03589295267817E-14,17.0562499999422,
10.5687124469213));
#294180=CARTESIAN_POINT('Ctrl Pts',(3.10606665601009,17.2062499999417,9.5594902125713));
#294181=CARTESIAN_POINT('Ctrl Pts',(6.21213331202019,17.3562499999411,8.55026797822134));
#294182=CARTESIAN_POINT('Ctrl Pts',(8.13178807675717,17.5062499999405,5.90808986649102));
#294183=CARTESIAN_POINT('Ctrl Pts',(10.0514428414941,17.6562499999399,3.2659117547607));
#294184=CARTESIAN_POINT('Ctrl Pts',(10.0514428414941,17.8062499999393,-1.23094673026484E-15));
#294185=CARTESIAN_POINT('Ctrl Pts',(10.0514428414941,17.9562499999387,-3.26591175476071));
#294186=CARTESIAN_POINT('Ctrl Pts',(8.13178807675717,18.1062499999381,-5.90808986649102));
#294187=CARTESIAN_POINT('Ctrl Pts',(6.21213331202019,18.2562499999375,-8.55026797822134));
#294188=CARTESIAN_POINT('Ctrl Pts',(3.10606665601008,18.4062499999369,-9.5594902125713));
#294189=CARTESIAN_POINT('Ctrl Pts',(-2.38113721364588E-14,18.5562499999362,
-10.5687124469213));
#294190=CARTESIAN_POINT('Ctrl Pts',(-3.10606665601013,18.7062499999357,
-9.5594902125713));
#294191=CARTESIAN_POINT('Ctrl Pts',(-6.21213331202024,18.856249999935,-8.55026797822134));
#294192=CARTESIAN_POINT('Ctrl Pts',(-8.13178807675721,19.0062499999344,
-5.90808986649102));
#294193=CARTESIAN_POINT('Ctrl Pts',(-10.0514428414942,19.1562499999338,
-3.2659117547607));
#294194=CARTESIAN_POINT('Ctrl Pts',(-10.0514428414942,19.3062499999332,
2.46189346052968E-15));
#294195=CARTESIAN_POINT('Ctrl Pts',(-10.0514428414942,19.4562499999326,
3.26591175476071));
#294196=CARTESIAN_POINT('Ctrl Pts',(-8.13178807675721,19.606249999932,5.90808986649102));
#294197=CARTESIAN_POINT('Ctrl Pts',(-6.21213331202024,19.7562499999314,
8.55026797822134));
#294198=CARTESIAN_POINT('Ctrl Pts',(-3.10606665601013,19.9062499999308,
9.5594902125713));
#294199=CARTESIAN_POINT('Ctrl Pts',(-2.20866387984435E-14,20.0562499999302,
10.5687124469213));
#294200=CARTESIAN_POINT('Ctrl Pts',(3.10606665601009,20.2062499999297,9.5594902125713));
#294201=CARTESIAN_POINT('Ctrl Pts',(6.21213331202019,20.356249999929,8.55026797822134));
#294202=CARTESIAN_POINT('Ctrl Pts',(8.13178807675717,20.5062499999285,5.90808986649102));
#294203=CARTESIAN_POINT('Ctrl Pts',(10.0514428414941,20.6562499999279,3.2659117547607));
#294204=CARTESIAN_POINT('Ctrl Pts',(10.0514428414941,20.8062499999273,-1.23094673026484E-15));
#294205=CARTESIAN_POINT('Ctrl Pts',(10.0514428414941,20.9562499999267,-3.26591175476071));
#294206=CARTESIAN_POINT('Ctrl Pts',(8.13178807675716,21.1062499999261,-5.90808986649102));
#294207=CARTESIAN_POINT('Ctrl Pts',(6.21213331202019,21.2562499999255,-8.55026797822134));
#294208=CARTESIAN_POINT('Ctrl Pts',(3.10606665601008,21.4062499999249,-9.5594902125713));
#294209=CARTESIAN_POINT('Ctrl Pts',(-2.55390814081207E-14,21.5562499999242,
-10.5687124469213));
#294210=CARTESIAN_POINT('Ctrl Pts',(-3.10606665601013,21.7062499999237,
-9.5594902125713));
#294211=CARTESIAN_POINT('Ctrl Pts',(-6.21213331202024,21.856249999923,-8.55026797822134));
#294212=CARTESIAN_POINT('Ctrl Pts',(-8.13178807675722,22.0062499999224,
-5.90808986649102));
#294213=CARTESIAN_POINT('Ctrl Pts',(-10.0514428414942,22.1562499999218,
-3.2659117547607));
#294214=CARTESIAN_POINT('Ctrl Pts',(-10.0514428414942,22.3062499999212,
2.46189346052968E-15));
#294215=CARTESIAN_POINT('Ctrl Pts',(-10.0514428414942,22.4562499999206,
3.26591175476071));
#294216=CARTESIAN_POINT('Ctrl Pts',(-8.13178807675722,22.60624999992,5.90808986649102));
#294217=CARTESIAN_POINT('Ctrl Pts',(-6.21213331202024,22.7562499999194,
8.55026797822134));
#294218=CARTESIAN_POINT('Ctrl Pts',(-3.10606665601013,22.9062499999188,
9.5594902125713));
#294219=CARTESIAN_POINT('Ctrl Pts',(-2.38143480701054E-14,23.0562499999182,
10.5687124469213));
#294220=CARTESIAN_POINT('Ctrl Pts',(3.10606665601008,23.2062499999177,9.5594902125713));
#294221=CARTESIAN_POINT('Ctrl Pts',(6.21213331202019,23.3562499999171,8.55026797822134));
#294222=CARTESIAN_POINT('Ctrl Pts',(8.13178807675716,23.5062499999165,5.90808986649102));
#294223=CARTESIAN_POINT('Ctrl Pts',(10.0514428414941,23.6562499999159,3.2659117547607));
#294224=CARTESIAN_POINT('Ctrl Pts',(10.0514428414941,23.8062499999153,-1.23094673026484E-15));
#294225=CARTESIAN_POINT('Ctrl Pts',(10.0514428414941,23.9562499999147,-3.26591175476071));
#294226=CARTESIAN_POINT('Ctrl Pts',(8.13178807675716,24.1062499999141,-5.90808986649102));
#294227=CARTESIAN_POINT('Ctrl Pts',(6.21213331202019,24.2562499999135,-8.55026797822134));
#294228=CARTESIAN_POINT('Ctrl Pts',(3.10606665601008,24.4062499999129,-9.5594902125713));
#294229=CARTESIAN_POINT('Ctrl Pts',(-2.72667906797825E-14,24.5562499999122,
-10.5687124469213));
#294230=CARTESIAN_POINT('Ctrl Pts',(-3.10606665601014,24.7062499999116,
-9.5594902125713));
#294231=CARTESIAN_POINT('Ctrl Pts',(-6.21213331202024,24.856249999911,-8.55026797822134));
#294232=CARTESIAN_POINT('Ctrl Pts',(-8.13178807675722,25.0062499999104,
-5.90808986649102));
#294233=CARTESIAN_POINT('Ctrl Pts',(-10.0514428414942,25.1562499999098,
-3.2659117547607));
#294234=CARTESIAN_POINT('Ctrl Pts',(-10.0514428414942,25.3062499999092,
2.46189346052968E-15));
#294235=CARTESIAN_POINT('Ctrl Pts',(-10.0514428414942,25.4562499999086,
3.26591175476071));
#294236=CARTESIAN_POINT('Ctrl Pts',(-8.13178807675722,25.6062499999081,
5.90808986649102));
#294237=CARTESIAN_POINT('Ctrl Pts',(-6.21213331202024,25.7562499999074,
8.55026797822134));
#294238=CARTESIAN_POINT('Ctrl Pts',(-3.10606665601013,25.9062499999069,
9.5594902125713));
#294239=CARTESIAN_POINT('Ctrl Pts',(-2.55420573417672E-14,26.0562499999062,
10.5687124469213));
#294240=CARTESIAN_POINT('Ctrl Pts',(3.10606665601008,26.2062499999057,9.5594902125713));
#294241=CARTESIAN_POINT('Ctrl Pts',(6.21213331202019,26.356249999905,8.55026797822134));
#294242=CARTESIAN_POINT('Ctrl Pts',(8.13178807675716,26.5062499999045,5.90808986649102));
#294243=CARTESIAN_POINT('Ctrl Pts',(10.0514428414941,26.6562499999039,3.2659117547607));
#294244=CARTESIAN_POINT('Ctrl Pts',(10.0514428414941,26.8062499999033,-1.23094673026484E-15));
#294245=CARTESIAN_POINT('Ctrl Pts',(10.0514428414941,26.9562499999027,-3.26591175476071));
#294246=CARTESIAN_POINT('Ctrl Pts',(8.13178807675716,27.1062499999021,-5.90808986649102));
#294247=CARTESIAN_POINT('Ctrl Pts',(6.21213331202019,27.2562499999015,-8.55026797822134));
#294248=CARTESIAN_POINT('Ctrl Pts',(3.10606665601008,27.4062499999009,-9.5594902125713));
#294249=CARTESIAN_POINT('Ctrl Pts',(-2.89944999514443E-14,27.5562499999002,
-10.5687124469213));
#294250=CARTESIAN_POINT('Ctrl Pts',(-3.10606665601014,27.7062499998996,
-9.5594902125713));
#294251=CARTESIAN_POINT('Ctrl Pts',(-6.21213331202024,27.856249999899,-8.55026797822134));
#294252=CARTESIAN_POINT('Ctrl Pts',(-8.13178807675722,28.0062499998984,
-5.90808986649102));
#294253=CARTESIAN_POINT('Ctrl Pts',(-10.0514428414942,28.1562499998978,
-3.2659117547607));
#294254=CARTESIAN_POINT('Ctrl Pts',(-10.0514428414942,28.3062499998973,
2.46189346052968E-15));
#294255=CARTESIAN_POINT('Ctrl Pts',(-10.0514428414942,28.4562499998966,
3.26591175476071));
#294256=CARTESIAN_POINT('Ctrl Pts',(-8.13178807675722,28.606249999896,5.90808986649102));
#294257=CARTESIAN_POINT('Ctrl Pts',(-6.21213331202024,28.7562499998954,
8.55026797822134));
#294258=CARTESIAN_POINT('Ctrl Pts',(-3.10606665601014,28.9062499998949,
9.5594902125713));
#294259=CARTESIAN_POINT('Ctrl Pts',(-2.72697666134291E-14,29.0562499998942,
10.5687124469213));
#294260=CARTESIAN_POINT('Ctrl Pts',(3.10606665601008,29.2062499998937,9.5594902125713));
#294261=CARTESIAN_POINT('Ctrl Pts',(6.21213331202019,29.356249999893,8.55026797822134));
#294262=CARTESIAN_POINT('Ctrl Pts',(8.13178807675716,29.5062499998925,5.90808986649102));
#294263=CARTESIAN_POINT('Ctrl Pts',(10.0514428414941,29.6562499998919,3.2659117547607));
#294264=CARTESIAN_POINT('Ctrl Pts',(10.0514428414941,29.8062499998913,-1.23094673026484E-15));
#294265=CARTESIAN_POINT('Ctrl Pts',(10.0514428414941,29.9562499998907,-3.26591175476071));
#294266=CARTESIAN_POINT('Ctrl Pts',(8.13178807675716,30.1062499998901,-5.90808986649102));
#294267=CARTESIAN_POINT('Ctrl Pts',(6.21213331202019,30.2562499998895,-8.55026797822134));
#294268=CARTESIAN_POINT('Ctrl Pts',(3.10606665601008,30.4062499998889,-9.5594902125713));
#294269=CARTESIAN_POINT('Ctrl Pts',(-3.07222092231062E-14,30.5562499998883,
-10.5687124469213));
#294270=CARTESIAN_POINT('Ctrl Pts',(-3.10606665601014,30.7062499998877,
-9.5594902125713));
#294271=CARTESIAN_POINT('Ctrl Pts',(-6.21213331202025,30.8562499998871,
-8.55026797822134));
#294272=CARTESIAN_POINT('Ctrl Pts',(-8.13178807675722,31.0062499998864,
-5.90808986649102));
#294273=CARTESIAN_POINT('Ctrl Pts',(-10.0514428414942,31.1562499998858,
-3.2659117547607));
#294274=CARTESIAN_POINT('Ctrl Pts',(-10.0514428414942,31.3062499998852,
2.46189346052968E-15));
#294275=CARTESIAN_POINT('Ctrl Pts',(-10.0514428414942,31.4562499998847,
3.26591175476071));
#294276=CARTESIAN_POINT('Ctrl Pts',(-8.13178807675722,31.606249999884,5.90808986649102));
#294277=CARTESIAN_POINT('Ctrl Pts',(-6.21213331202024,31.7562499998835,
8.55026797822134));
#294278=CARTESIAN_POINT('Ctrl Pts',(-3.10606665601014,31.9062499998829,
9.5594902125713));
#294279=CARTESIAN_POINT('Ctrl Pts',(-2.89974758850909E-14,32.0562499998822,
10.5687124469213));
#294280=CARTESIAN_POINT('Ctrl Pts',(3.10606665601008,32.2062499998816,9.5594902125713));
#294281=CARTESIAN_POINT('Ctrl Pts',(6.21213331202019,32.3562499998811,8.55026797822134));
#294282=CARTESIAN_POINT('Ctrl Pts',(8.13178807675716,32.5062499998805,5.90808986649102));
#294283=CARTESIAN_POINT('Ctrl Pts',(10.0514428414941,32.6562499998798,3.2659117547607));
#294284=CARTESIAN_POINT('Ctrl Pts',(10.0514428414941,32.8062499998793,-1.23094673026484E-15));
#294285=CARTESIAN_POINT('Ctrl Pts',(10.0514428414941,32.9562499998787,-3.26591175476071));
#294286=CARTESIAN_POINT('Ctrl Pts',(8.13178807675716,33.1062499998781,-5.90808986649102));
#294287=CARTESIAN_POINT('Ctrl Pts',(6.21213331202019,33.2562499998775,-8.55026797822134));
#294288=CARTESIAN_POINT('Ctrl Pts',(3.10606665601008,33.4062499998769,-9.5594902125713));
#294289=CARTESIAN_POINT('Ctrl Pts',(-3.2449918494768E-14,33.5562499998763,
-10.5687124469213));
#294290=CARTESIAN_POINT('Ctrl Pts',(-3.10606665601014,33.7062499998756,
-9.5594902125713));
#294291=CARTESIAN_POINT('Ctrl Pts',(-6.21213331202025,33.8562499998751,
-8.55026797822134));
#294292=CARTESIAN_POINT('Ctrl Pts',(-8.13178807675722,34.0062499998744,
-5.90808986649102));
#294293=CARTESIAN_POINT('Ctrl Pts',(-10.0514428414942,34.1562499998739,
-3.2659117547607));
#294294=CARTESIAN_POINT('Ctrl Pts',(-10.0514428414942,34.3062499998732,
2.46189346052968E-15));
#294295=CARTESIAN_POINT('Ctrl Pts',(-10.0514428414942,34.4562499998727,
3.26591175476071));
#294296=CARTESIAN_POINT('Ctrl Pts',(-8.13178807675722,34.606249999872,5.90808986649102));
#294297=CARTESIAN_POINT('Ctrl Pts',(-6.21213331202024,34.7562499998715,
8.55026797822134));
#294298=CARTESIAN_POINT('Ctrl Pts',(-3.10606665601014,34.9062499998708,
9.5594902125713));
#294299=CARTESIAN_POINT('Ctrl Pts',(-3.07251851567527E-14,35.0562499998703,
10.5687124469213));
#294300=CARTESIAN_POINT('Ctrl Pts',(3.10606665601008,35.2062499998697,9.5594902125713));
#294301=CARTESIAN_POINT('Ctrl Pts',(6.21213331202019,35.3562499998691,8.55026797822134));
#294302=CARTESIAN_POINT('Ctrl Pts',(8.13178807675716,35.5062499998685,5.90808986649102));
#294303=CARTESIAN_POINT('Ctrl Pts',(10.0514428414941,35.6562499998679,3.2659117547607));
#294304=CARTESIAN_POINT('Ctrl Pts',(10.0514428414941,35.8062499998673,-1.23094673026484E-15));
#294305=CARTESIAN_POINT('Ctrl Pts',(10.0514428414941,35.9562499998667,-3.26591175476071));
#294306=CARTESIAN_POINT('Ctrl Pts',(8.13178807675716,36.1062499998661,-5.90808986649102));
#294307=CARTESIAN_POINT('Ctrl Pts',(6.21213331202018,36.2562499998655,-8.55026797822134));
#294308=CARTESIAN_POINT('Ctrl Pts',(3.10606665601007,36.4062499998649,-9.5594902125713));
#294309=CARTESIAN_POINT('Ctrl Pts',(-3.41776277664299E-14,36.5562499998642,
-10.5687124469213));
#294310=CARTESIAN_POINT('Ctrl Pts',(-3.10606665601014,36.7062499998636,
-9.5594902125713));
#294311=CARTESIAN_POINT('Ctrl Pts',(-6.21213331202025,36.856249999863,-8.55026797822134));
#294312=CARTESIAN_POINT('Ctrl Pts',(-8.13178807675722,37.0062499998624,
-5.90808986649102));
#294313=CARTESIAN_POINT('Ctrl Pts',(-10.0514428414942,37.1562499998618,
-3.2659117547607));
#294314=CARTESIAN_POINT('Ctrl Pts',(-10.0514428414942,37.3062499998613,
2.46189346052968E-15));
#294315=CARTESIAN_POINT('Ctrl Pts',(-10.0514428414942,37.4562499998606,
3.26591175476071));
#294316=CARTESIAN_POINT('Ctrl Pts',(-8.13178807675722,37.60624999986,5.90808986649102));
#294317=CARTESIAN_POINT('Ctrl Pts',(-6.21213331202025,37.7562499998594,
8.55026797822134));
#294318=CARTESIAN_POINT('Ctrl Pts',(-3.10606665601014,37.9062499998588,
9.5594902125713));
#294319=CARTESIAN_POINT('Ctrl Pts',(-3.24528944284146E-14,38.0562499998583,
10.5687124469213));
#294320=CARTESIAN_POINT('Ctrl Pts',(3.10606665601007,38.2062499998577,9.5594902125713));
#294321=CARTESIAN_POINT('Ctrl Pts',(6.21213331202018,38.3562499998571,8.55026797822134));
#294322=CARTESIAN_POINT('Ctrl Pts',(8.13178807675716,38.5062499998565,5.90808986649102));
#294323=CARTESIAN_POINT('Ctrl Pts',(10.0514428414941,38.6562499998559,3.2659117547607));
#294324=CARTESIAN_POINT('Ctrl Pts',(10.0514428414941,38.8062499998553,-1.23094673026484E-15));
#294325=CARTESIAN_POINT('Ctrl Pts',(10.0514428414941,38.9562499998547,-3.26591175476071));
#294326=CARTESIAN_POINT('Ctrl Pts',(8.13178807675715,39.1062499998541,-5.90808986649102));
#294327=CARTESIAN_POINT('Ctrl Pts',(6.21213331202018,39.2562499998535,-8.55026797822134));
#294328=CARTESIAN_POINT('Ctrl Pts',(3.10606665601007,39.4062499998529,-9.5594902125713));
#294329=CARTESIAN_POINT('Ctrl Pts',(-3.59053370380917E-14,39.5562499998523,
-10.5687124469213));
#294330=CARTESIAN_POINT('Ctrl Pts',(-3.10606665601014,39.7062499998516,
-9.5594902125713));
#294331=CARTESIAN_POINT('Ctrl Pts',(-6.21213331202025,39.856249999851,-8.55026797822134));
#294332=CARTESIAN_POINT('Ctrl Pts',(-8.13178807675723,40.0062499998505,
-5.90808986649102));
#294333=CARTESIAN_POINT('Ctrl Pts',(-10.0514428414942,40.1562499998499,
-3.2659117547607));
#294334=CARTESIAN_POINT('Ctrl Pts',(-10.0514428414942,40.3062499998493,
2.46189346052968E-15));
#294335=CARTESIAN_POINT('Ctrl Pts',(-10.0514428414942,40.4562499998487,
3.26591175476071));
#294336=CARTESIAN_POINT('Ctrl Pts',(-8.13178807675723,40.606249999848,5.90808986649102));
#294337=CARTESIAN_POINT('Ctrl Pts',(-6.21213331202025,40.7562499998475,
8.55026797822134));
#294338=CARTESIAN_POINT('Ctrl Pts',(-3.10606665601014,40.9062499998468,
9.5594902125713));
#294339=CARTESIAN_POINT('Ctrl Pts',(-3.41806037000764E-14,41.0562499998463,
10.5687124469213));
#294340=CARTESIAN_POINT('Ctrl Pts',(3.10606665601007,41.2062499998457,9.5594902125713));
#294341=CARTESIAN_POINT('Ctrl Pts',(6.21213331202018,41.3562499998451,8.55026797822134));
#294342=CARTESIAN_POINT('Ctrl Pts',(8.13178807675715,41.5062499998444,5.90808986649102));
#294343=CARTESIAN_POINT('Ctrl Pts',(10.0514428414941,41.6562499998439,3.2659117547607));
#294344=CARTESIAN_POINT('Ctrl Pts',(10.0514428414941,41.8062499998433,-1.23094673026484E-15));
#294345=CARTESIAN_POINT('Ctrl Pts',(10.0514428414941,41.9562499998427,-3.26591175476071));
#294346=CARTESIAN_POINT('Ctrl Pts',(8.13178807675715,42.1062499998421,-5.90808986649102));
#294347=CARTESIAN_POINT('Ctrl Pts',(6.21213331202018,42.2562499998414,-8.55026797822134));
#294348=CARTESIAN_POINT('Ctrl Pts',(3.10606665601007,42.4062499998408,-9.5594902125713));
#294349=CARTESIAN_POINT('Ctrl Pts',(-3.76330463097535E-14,42.5562499998402,
-10.5687124469213));
#294350=CARTESIAN_POINT('Ctrl Pts',(-3.10606665601015,42.7062499998396,
-9.5594902125713));
#294351=CARTESIAN_POINT('Ctrl Pts',(-6.21213331202025,42.8562499998391,
-8.55026797822134));
#294352=CARTESIAN_POINT('Ctrl Pts',(-8.13178807675723,43.0062499998385,
-5.90808986649102));
#294353=CARTESIAN_POINT('Ctrl Pts',(-10.0514428414942,43.1562499998379,
-3.2659117547607));
#294354=CARTESIAN_POINT('Ctrl Pts',(-10.0514428414942,43.3062499998373,
2.46189346052968E-15));
#294355=CARTESIAN_POINT('Ctrl Pts',(-10.0514428414942,43.4562499998366,
3.26591175476071));
#294356=CARTESIAN_POINT('Ctrl Pts',(-8.13178807675723,43.6062499998361,
5.90808986649102));
#294357=CARTESIAN_POINT('Ctrl Pts',(-6.21213331202025,43.7562499998354,
8.55026797822134));
#294358=CARTESIAN_POINT('Ctrl Pts',(-3.10606665601014,43.9062499998348,
9.5594902125713));
#294359=CARTESIAN_POINT('Ctrl Pts',(-3.59083129717383E-14,44.0562499998343,
10.5687124469213));
#294360=CARTESIAN_POINT('Ctrl Pts',(3.10606665601007,44.2062499998337,9.5594902125713));
#294361=CARTESIAN_POINT('Ctrl Pts',(6.21213331202018,44.3562499998331,8.55026797822134));
#294362=CARTESIAN_POINT('Ctrl Pts',(8.13178807675715,44.5062499998324,5.90808986649102));
#294363=CARTESIAN_POINT('Ctrl Pts',(10.0514428414941,44.6562499998319,3.2659117547607));
#294364=CARTESIAN_POINT('Ctrl Pts',(10.0514428414941,44.8062499998313,-1.23094673026484E-15));
#294365=CARTESIAN_POINT('Ctrl Pts',(10.0514428414941,44.9562499998307,-3.26591175476071));
#294366=CARTESIAN_POINT('Ctrl Pts',(8.13178807675715,45.1062499998301,-5.90808986649102));
#294367=CARTESIAN_POINT('Ctrl Pts',(6.21213331202018,45.2562499998295,-8.55026797822134));
#294368=CARTESIAN_POINT('Ctrl Pts',(3.10606665601007,45.4062499998289,-9.5594902125713));
#294369=CARTESIAN_POINT('Ctrl Pts',(-3.93607555814154E-14,45.5562499998283,
-10.5687124469213));
#294370=CARTESIAN_POINT('Ctrl Pts',(-3.10606665601015,45.7062499998276,
-9.5594902125713));
#294371=CARTESIAN_POINT('Ctrl Pts',(-6.21213331202026,45.856249999827,-8.55026797822134));
#294372=CARTESIAN_POINT('Ctrl Pts',(-8.13178807675723,46.0062499998265,
-5.90808986649102));
#294373=CARTESIAN_POINT('Ctrl Pts',(-10.0514428414942,46.1562499998259,
-3.2659117547607));
#294374=CARTESIAN_POINT('Ctrl Pts',(-10.0514428414942,46.3062499998252,
2.46189346052968E-15));
#294375=CARTESIAN_POINT('Ctrl Pts',(-10.0514428414942,46.4562499998247,
3.26591175476071));
#294376=CARTESIAN_POINT('Ctrl Pts',(-8.13178807675723,46.606249999824,5.90808986649102));
#294377=CARTESIAN_POINT('Ctrl Pts',(-6.21213331202025,46.7562499998235,
8.55026797822134));
#294378=CARTESIAN_POINT('Ctrl Pts',(-3.10606665601015,46.9062499998228,
9.5594902125713));
#294379=CARTESIAN_POINT('Ctrl Pts',(-3.76360222434001E-14,47.0562499998223,
10.5687124469213));
#294380=CARTESIAN_POINT('Ctrl Pts',(3.10606665601007,47.2062499998217,9.5594902125713));
#294381=CARTESIAN_POINT('Ctrl Pts',(6.21213331202018,47.3562499998211,8.55026797822134));
#294382=CARTESIAN_POINT('Ctrl Pts',(8.13178807675715,47.5062499998204,5.90808986649102));
#294383=CARTESIAN_POINT('Ctrl Pts',(10.0514428414941,47.6562499998198,3.2659117547607));
#294384=CARTESIAN_POINT('Ctrl Pts',(10.0514428414941,47.8062499998193,-1.23094673026484E-15));
#294385=CARTESIAN_POINT('Ctrl Pts',(10.0514428414941,47.9562499998186,-3.26591175476071));
#294386=CARTESIAN_POINT('Ctrl Pts',(8.13178807675715,48.1062499998181,-5.90808986649102));
#294387=CARTESIAN_POINT('Ctrl Pts',(6.21213331202017,48.2562499998174,-8.55026797822134));
#294388=CARTESIAN_POINT('Ctrl Pts',(3.10606665601007,48.4062499998169,-9.5594902125713));
#294389=CARTESIAN_POINT('Ctrl Pts',(-4.10884648530772E-14,48.5562499998163,
-10.5687124469213));
#294390=CARTESIAN_POINT('Ctrl Pts',(-3.10606665601015,48.7062499998157,
-9.5594902125713));
#294391=CARTESIAN_POINT('Ctrl Pts',(-6.21213331202026,48.8562499998151,
-8.55026797822134));
#294392=CARTESIAN_POINT('Ctrl Pts',(-8.13178807675723,49.0062499998145,
-5.90808986649102));
#294393=CARTESIAN_POINT('Ctrl Pts',(-10.0514428414942,49.1562499998138,
-3.2659117547607));
#294394=CARTESIAN_POINT('Ctrl Pts',(-10.0514428414942,49.3062499998132,
2.46189346052968E-15));
#294395=CARTESIAN_POINT('Ctrl Pts',(-10.0514428414942,49.4562499998126,
3.26591175476071));
#294396=CARTESIAN_POINT('Ctrl Pts',(-8.13178807675723,49.6062499998121,
5.90808986649102));
#294397=CARTESIAN_POINT('Ctrl Pts',(-6.21213331202026,49.7562499998114,
8.55026797822134));
#294398=CARTESIAN_POINT('Ctrl Pts',(-3.10606665601015,49.9062499998109,
9.5594902125713));
#294399=CARTESIAN_POINT('Ctrl Pts',(-3.9363731515062E-14,50.0562499998103,
10.5687124469213));
#294400=CARTESIAN_POINT('Ctrl Pts',(3.10606665601007,50.2062499998097,9.5594902125713));
#294401=CARTESIAN_POINT('Ctrl Pts',(6.21213331202017,50.3562499998091,8.55026797822134));
#294402=CARTESIAN_POINT('Ctrl Pts',(8.13178807675715,50.5062499998085,5.90808986649102));
#294403=CARTESIAN_POINT('Ctrl Pts',(10.0514428414941,50.6562499998078,3.2659117547607));
#294404=CARTESIAN_POINT('Ctrl Pts',(10.0514428414941,50.8062499998072,-1.23094673026484E-15));
#294405=CARTESIAN_POINT('Ctrl Pts',(10.0514428414941,50.9562499998067,-3.26591175476071));
#294406=CARTESIAN_POINT('Ctrl Pts',(8.13178807675715,51.1062499998061,-5.90808986649102));
#294407=CARTESIAN_POINT('Ctrl Pts',(6.21213331202017,51.2562499998055,-8.55026797822134));
#294408=CARTESIAN_POINT('Ctrl Pts',(3.10606665601006,51.4062499998048,-9.5594902125713));
#294409=CARTESIAN_POINT('Ctrl Pts',(-4.2816174124739E-14,51.5562499998043,
-10.5687124469213));
#294410=CARTESIAN_POINT('Ctrl Pts',(-3.10606665601015,51.7062499998037,
-9.5594902125713));
#294411=CARTESIAN_POINT('Ctrl Pts',(-6.21213331202026,51.856249999803,-8.55026797822134));
#294412=CARTESIAN_POINT('Ctrl Pts',(-8.13178807675723,52.0062499998025,
-5.90808986649102));
#294413=CARTESIAN_POINT('Ctrl Pts',(-10.0514428414942,52.1562499998019,
-3.2659117547607));
#294414=CARTESIAN_POINT('Ctrl Pts',(-10.0514428414942,52.3062499998012,
2.46189346052968E-15));
#294415=CARTESIAN_POINT('Ctrl Pts',(-10.0514428414942,52.4562499998006,
3.26591175476071));
#294416=CARTESIAN_POINT('Ctrl Pts',(-8.13178807675723,52.6062499998,5.90808986649102));
#294417=CARTESIAN_POINT('Ctrl Pts',(-6.21213331202026,52.7562499997994,
8.55026797822134));
#294418=CARTESIAN_POINT('Ctrl Pts',(-3.10606665601015,52.9062499997988,
9.5594902125713));
#294419=CARTESIAN_POINT('Ctrl Pts',(-4.10914407867238E-14,53.0562499997983,
10.5687124469213));
#294420=CARTESIAN_POINT('Ctrl Pts',(3.10606665601007,53.2062499997976,9.5594902125713));
#294421=CARTESIAN_POINT('Ctrl Pts',(6.21213331202017,53.3562499997971,8.55026797822134));
#294422=CARTESIAN_POINT('Ctrl Pts',(8.13178807675715,53.5062499997965,5.90808986649102));
#294423=CARTESIAN_POINT('Ctrl Pts',(10.0514428414941,53.6562499997959,3.2659117547607));
#294424=CARTESIAN_POINT('Ctrl Pts',(10.0514428414941,53.8062499997953,-1.23094673026484E-15));
#294425=CARTESIAN_POINT('Ctrl Pts',(10.0514428414941,53.9562499997946,-3.26591175476071));
#294426=CARTESIAN_POINT('Ctrl Pts',(8.13178807675714,54.106249999794,-5.90808986649102));
#294427=CARTESIAN_POINT('Ctrl Pts',(6.21213331202017,54.2562499997934,-8.55026797822134));
#294428=CARTESIAN_POINT('Ctrl Pts',(3.10606665601006,54.4062499997928,-9.5594902125713));
#294429=CARTESIAN_POINT('Ctrl Pts',(-4.45438833964009E-14,54.5562499997923,
-10.5687124469213));
#294430=CARTESIAN_POINT('Ctrl Pts',(-3.10606665601015,54.7062499997917,
-9.5594902125713));
#294431=CARTESIAN_POINT('Ctrl Pts',(-6.21213331202026,54.856249999791,-8.55026797822134));
#294432=CARTESIAN_POINT('Ctrl Pts',(-8.13178807675724,55.0062499997905,
-5.90808986649102));
#294433=CARTESIAN_POINT('Ctrl Pts',(-10.0514428414942,55.1562499997898,
-3.2659117547607));
#294434=CARTESIAN_POINT('Ctrl Pts',(-10.0514428414942,55.3062499997893,
2.46189346052968E-15));
#294435=CARTESIAN_POINT('Ctrl Pts',(-10.0514428414942,55.4562499997886,
3.26591175476071));
#294436=CARTESIAN_POINT('Ctrl Pts',(-8.13178807675724,55.606249999788,5.90808986649102));
#294437=CARTESIAN_POINT('Ctrl Pts',(-6.21213331202026,55.7562499997874,
8.55026797822134));
#294438=CARTESIAN_POINT('Ctrl Pts',(-3.10606665601015,55.9062499997869,
9.5594902125713));
#294439=CARTESIAN_POINT('Ctrl Pts',(-4.28191500583856E-14,56.0562499997862,
10.5687124469213));
#294440=CARTESIAN_POINT('Ctrl Pts',(3.10606665601006,56.2062499997857,9.5594902125713));
#294441=CARTESIAN_POINT('Ctrl Pts',(6.21213331202017,56.356249999785,8.55026797822134));
#294442=CARTESIAN_POINT('Ctrl Pts',(8.13178807675714,56.5062499997845,5.90808986649102));
#294443=CARTESIAN_POINT('Ctrl Pts',(10.0514428414941,56.6562499997839,3.2659117547607));
#294444=CARTESIAN_POINT('Ctrl Pts',(10.0514428414941,56.8062499997833,-1.23094673026484E-15));
#294445=CARTESIAN_POINT('Ctrl Pts',(10.0514428414941,56.9562499997827,-3.26591175476071));
#294446=CARTESIAN_POINT('Ctrl Pts',(8.13178807675714,57.1062499997821,-5.90808986649102));
#294447=CARTESIAN_POINT('Ctrl Pts',(6.21213331202017,57.2562499997814,-8.55026797822134));
#294448=CARTESIAN_POINT('Ctrl Pts',(3.10606665601006,57.4062499997808,-9.5594902125713));
#294449=CARTESIAN_POINT('Ctrl Pts',(-4.62715926680627E-14,57.5562499997802,
-10.5687124469213));
#294450=CARTESIAN_POINT('Ctrl Pts',(-3.10606665601015,57.7062499997797,
-9.5594902125713));
#294451=CARTESIAN_POINT('Ctrl Pts',(-6.21213331202026,57.856249999779,-8.55026797822134));
#294452=CARTESIAN_POINT('Ctrl Pts',(-8.13178807675724,58.0062499997784,
-5.90808986649102));
#294453=CARTESIAN_POINT('Ctrl Pts',(-10.0514428414942,58.1562499997778,
-3.2659117547607));
#294454=CARTESIAN_POINT('Ctrl Pts',(-10.0514428414942,58.3062499997773,
2.46189346052968E-15));
#294455=CARTESIAN_POINT('Ctrl Pts',(-10.0514428414942,58.4562499997766,
3.26591175476071));
#294456=CARTESIAN_POINT('Ctrl Pts',(-8.13178807675724,58.6062499997761,
5.90808986649102));
#294457=CARTESIAN_POINT('Ctrl Pts',(-6.21213331202026,58.7562499997754,
8.55026797822134));
#294458=CARTESIAN_POINT('Ctrl Pts',(-3.10606665601015,58.9062499997749,
9.5594902125713));
#294459=CARTESIAN_POINT('Ctrl Pts',(-4.45468593300475E-14,59.0562499997743,
10.5687124469213));
#294460=CARTESIAN_POINT('Ctrl Pts',(3.10606665601006,59.2062499997736,9.5594902125713));
#294461=CARTESIAN_POINT('Ctrl Pts',(6.21213331202017,59.356249999773,8.55026797822134));
#294462=CARTESIAN_POINT('Ctrl Pts',(8.13178807675714,59.5062499997725,5.90808986649102));
#294463=CARTESIAN_POINT('Ctrl Pts',(10.0514428414941,59.6562499997718,3.2659117547607));
#294464=CARTESIAN_POINT('Ctrl Pts',(10.0514428414941,59.8062499997713,-1.23094673026484E-15));
#294465=CARTESIAN_POINT('Ctrl Pts',(10.0514428414941,59.9562499997706,-3.26591175476071));
#294466=CARTESIAN_POINT('Ctrl Pts',(8.13178807675714,60.10624999977,-5.90808986649102));
#294467=CARTESIAN_POINT('Ctrl Pts',(6.21213331202017,60.2562499997694,-8.55026797822134));
#294468=CARTESIAN_POINT('Ctrl Pts',(3.10606665601006,60.4062499997689,-9.5594902125713));
#294469=CARTESIAN_POINT('Ctrl Pts',(-4.79993019397246E-14,60.5562499997682,
-10.5687124469213));
#294470=CARTESIAN_POINT('Ctrl Pts',(-3.10606665601016,60.7062499997676,
-9.5594902125713));
#294471=CARTESIAN_POINT('Ctrl Pts',(-6.21213331202026,60.856249999767,-8.55026797822134));
#294472=CARTESIAN_POINT('Ctrl Pts',(-8.13178807675724,61.0062499997664,
-5.90808986649102));
#294473=CARTESIAN_POINT('Ctrl Pts',(-10.0514428414942,61.1562499997658,
-3.2659117547607));
#294474=CARTESIAN_POINT('Ctrl Pts',(-10.0514428414942,61.3062499997652,
2.46189346052968E-15));
#294475=CARTESIAN_POINT('Ctrl Pts',(-10.0514428414942,61.4562499997646,
3.26591175476071));
#294476=CARTESIAN_POINT('Ctrl Pts',(-8.13178807675724,61.6062499997641,
5.90808986649102));
#294477=CARTESIAN_POINT('Ctrl Pts',(-6.21213331202026,61.7562499997634,
8.55026797822134));
#294478=CARTESIAN_POINT('Ctrl Pts',(-3.10606665601015,61.9062499997628,
9.5594902125713));
#294479=CARTESIAN_POINT('Ctrl Pts',(-4.62745686017093E-14,62.0562499997622,
10.5687124469213));
#294480=CARTESIAN_POINT('Ctrl Pts',(3.10606665601006,62.2062499997617,9.5594902125713));
#294481=CARTESIAN_POINT('Ctrl Pts',(6.21213331202017,62.356249999761,8.55026797822134));
#294482=CARTESIAN_POINT('Ctrl Pts',(8.13178807675714,62.5062499997605,5.90808986649102));
#294483=CARTESIAN_POINT('Ctrl Pts',(10.0514428414941,62.6562499997599,3.2659117547607));
#294484=CARTESIAN_POINT('Ctrl Pts',(10.0514428414941,62.8062499997593,-1.23094673026484E-15));
#294485=CARTESIAN_POINT('Ctrl Pts',(10.0514428414941,62.9562499997587,-3.26591175476071));
#294486=CARTESIAN_POINT('Ctrl Pts',(8.13178807675714,63.1062499997581,-5.90808986649102));
#294487=CARTESIAN_POINT('Ctrl Pts',(6.21213331202017,63.2562499997575,-8.55026797822134));
#294488=CARTESIAN_POINT('Ctrl Pts',(3.10606665601006,63.4062499997568,-9.5594902125713));
#294489=CARTESIAN_POINT('Ctrl Pts',(-4.97270112113864E-14,63.5562499997562,
-10.5687124469213));
#294490=CARTESIAN_POINT('Ctrl Pts',(-3.10606665601016,63.7062499997556,
-9.5594902125713));
#294491=CARTESIAN_POINT('Ctrl Pts',(-6.21213331202027,63.8562499997551,
-8.55026797822134));
#294492=CARTESIAN_POINT('Ctrl Pts',(-8.13178807675724,64.0062499997544,
-5.90808986649102));
#294493=CARTESIAN_POINT('Ctrl Pts',(-10.0514428414942,64.1562499997538,
-3.2659117547607));
#294494=CARTESIAN_POINT('Ctrl Pts',(-10.0514428414942,64.3062499997532,
2.46189346052968E-15));
#294495=CARTESIAN_POINT('Ctrl Pts',(-10.0514428414942,64.4562499997526,
3.26591175476071));
#294496=CARTESIAN_POINT('Ctrl Pts',(-8.13178807675724,64.606249999752,5.90808986649102));
#294497=CARTESIAN_POINT('Ctrl Pts',(-6.21213331202026,64.7562499997514,
8.55026797822134));
#294498=CARTESIAN_POINT('Ctrl Pts',(-3.10606665601016,64.9062499997509,
9.5594902125713));
#294499=CARTESIAN_POINT('Ctrl Pts',(-4.80022778733711E-14,65.0562499997502,
10.5687124469213));
#294500=CARTESIAN_POINT('Ctrl Pts',(3.10606665601006,65.2062499997497,9.5594902125713));
#294501=CARTESIAN_POINT('Ctrl Pts',(6.21213331202017,65.3562499997491,8.55026797822134));
#294502=CARTESIAN_POINT('Ctrl Pts',(8.13178807675714,65.5062499997484,5.90808986649102));
#294503=CARTESIAN_POINT('Ctrl Pts',(10.0514428414941,65.6562499997479,3.2659117547607));
#294504=CARTESIAN_POINT('Ctrl Pts',(10.0514428414941,65.8062499997473,-1.23094673026484E-15));
#294505=CARTESIAN_POINT('Ctrl Pts',(10.0514428414941,65.9562499997467,-3.26591175476071));
#294506=CARTESIAN_POINT('Ctrl Pts',(8.13178807675714,66.1062499997461,-5.90808986649102));
#294507=CARTESIAN_POINT('Ctrl Pts',(6.21213331202016,66.2562499997454,-8.55026797822134));
#294508=CARTESIAN_POINT('Ctrl Pts',(3.10606665601006,66.4062499997449,-9.5594902125713));
#294509=CARTESIAN_POINT('Ctrl Pts',(-5.14547204830482E-14,66.5562499997443,
-10.5687124469213));
#294510=CARTESIAN_POINT('Ctrl Pts',(-3.10606665601016,66.7062499997436,
-9.5594902125713));
#294511=CARTESIAN_POINT('Ctrl Pts',(-6.21213331202027,66.8562499997431,
-8.55026797822134));
#294512=CARTESIAN_POINT('Ctrl Pts',(-8.13178807675724,67.0062499997424,
-5.90808986649102));
#294513=CARTESIAN_POINT('Ctrl Pts',(-10.0514428414942,67.1562499997418,
-3.2659117547607));
#294514=CARTESIAN_POINT('Ctrl Pts',(-10.0514428414942,67.3062499997412,
2.46189346052968E-15));
#294515=CARTESIAN_POINT('Ctrl Pts',(-10.0514428414942,67.4562499997406,
3.26591175476071));
#294516=CARTESIAN_POINT('Ctrl Pts',(-8.13178807675724,67.60624999974,5.90808986649102));
#294517=CARTESIAN_POINT('Ctrl Pts',(-6.21213331202027,67.7562499997395,
8.55026797822134));
#294518=CARTESIAN_POINT('Ctrl Pts',(-3.10606665601016,67.9062499997388,
9.5594902125713));
#294519=CARTESIAN_POINT('Ctrl Pts',(-4.9729987145033E-14,68.0562499997382,
10.5687124469213));
#294520=CARTESIAN_POINT('Ctrl Pts',(3.10606665601006,68.2062499997377,9.5594902125713));
#294521=CARTESIAN_POINT('Ctrl Pts',(6.21213331202017,68.356249999737,8.55026797822134));
#294522=CARTESIAN_POINT('Ctrl Pts',(8.13178807675714,68.5062499997365,5.90808986649102));
#294523=CARTESIAN_POINT('Ctrl Pts',(10.0514428414941,68.6562499997358,3.2659117547607));
#294524=CARTESIAN_POINT('Ctrl Pts',(10.0514428414941,68.8062499997353,-1.23094673026484E-15));
#294525=CARTESIAN_POINT('Ctrl Pts',(10.0514428414941,68.9562499997347,-3.26591175476071));
#294526=CARTESIAN_POINT('Ctrl Pts',(8.13178807675714,69.1062499997341,-5.90808986649102));
#294527=CARTESIAN_POINT('Ctrl Pts',(6.21213331202016,69.2562499997335,-8.55026797822134));
#294528=CARTESIAN_POINT('Ctrl Pts',(3.10606665601005,69.4062499997329,-9.5594902125713));
#294529=CARTESIAN_POINT('Ctrl Pts',(-5.31824297547101E-14,69.5562499997323,
-10.5687124469213));
#294530=CARTESIAN_POINT('Ctrl Pts',(-3.10606665601016,69.7062499997317,
-9.5594902125713));
#294531=CARTESIAN_POINT('Ctrl Pts',(-6.21213331202027,69.856249999731,-8.55026797822134));
#294532=CARTESIAN_POINT('Ctrl Pts',(-8.13178807675724,70.0062499997304,
-5.90808986649102));
#294533=CARTESIAN_POINT('Ctrl Pts',(-10.0514428414942,70.1562499997298,
-3.2659117547607));
#294534=CARTESIAN_POINT('Ctrl Pts',(-10.0514428414942,70.3062499997292,
2.46189346052968E-15));
#294535=CARTESIAN_POINT('Ctrl Pts',(-10.0514428414942,70.4562499997286,
3.26591175476071));
#294536=CARTESIAN_POINT('Ctrl Pts',(-8.13178807675724,70.606249999728,5.90808986649102));
#294537=CARTESIAN_POINT('Ctrl Pts',(-6.21213331202027,70.7562499997274,
8.55026797822134));
#294538=CARTESIAN_POINT('Ctrl Pts',(-3.10606665601016,70.9062499997269,
9.5594902125713));
#294539=CARTESIAN_POINT('Ctrl Pts',(-5.14576964166948E-14,71.0562499997262,
10.5687124469213));
#294540=CARTESIAN_POINT('Ctrl Pts',(3.10606665601006,71.2062499997256,9.5594902125713));
#294541=CARTESIAN_POINT('Ctrl Pts',(6.21213331202016,71.3562499997251,8.55026797822134));
#294542=CARTESIAN_POINT('Ctrl Pts',(8.13178807675714,71.5062499997244,5.90808986649102));
#294543=CARTESIAN_POINT('Ctrl Pts',(10.0514428414941,71.6562499997239,3.2659117547607));
#294544=CARTESIAN_POINT('Ctrl Pts',(10.0514428414941,71.8062499997232,-1.23094673026484E-15));
#294545=CARTESIAN_POINT('Ctrl Pts',(10.0514428414941,71.9562499997227,-3.26591175476071));
#294546=CARTESIAN_POINT('Ctrl Pts',(8.13178807675713,72.1062499997221,-5.90808986649102));
#294547=CARTESIAN_POINT('Ctrl Pts',(6.21213331202016,72.2562499997215,-8.55026797822134));
#294548=CARTESIAN_POINT('Ctrl Pts',(3.10606665601005,72.4062499997209,-9.5594902125713));
#294549=CARTESIAN_POINT('Ctrl Pts',(-5.49101390263719E-14,72.5562499997203,
-10.5687124469213));
#294550=CARTESIAN_POINT('Ctrl Pts',(-3.10606665601016,72.7062499997197,
-9.5594902125713));
#294551=CARTESIAN_POINT('Ctrl Pts',(-6.21213331202027,72.8562499997191,
-8.55026797822134));
#294552=CARTESIAN_POINT('Ctrl Pts',(-8.13178807675725,73.0062499997184,
-5.90808986649102));
#294553=CARTESIAN_POINT('Ctrl Pts',(-10.0514428414942,73.1562499997178,
-3.2659117547607));
#294554=CARTESIAN_POINT('Ctrl Pts',(-10.0514428414942,73.3062499997172,
2.46189346052968E-15));
#294555=CARTESIAN_POINT('Ctrl Pts',(-10.0514428414942,73.4562499997166,
3.26591175476071));
#294556=CARTESIAN_POINT('Ctrl Pts',(-8.13178807675725,73.606249999716,5.90808986649102));
#294557=CARTESIAN_POINT('Ctrl Pts',(-6.21213331202027,73.7562499997155,
8.55026797822134));
#294558=CARTESIAN_POINT('Ctrl Pts',(-3.10606665601016,73.9062499997148,
9.5594902125713));
#294559=CARTESIAN_POINT('Ctrl Pts',(-5.31854056883567E-14,74.0562499997143,
10.5687124469213));
#294560=CARTESIAN_POINT('Ctrl Pts',(3.10606665601005,74.2062499997136,9.5594902125713));
#294561=CARTESIAN_POINT('Ctrl Pts',(6.21213331202016,74.3562499997131,8.55026797822134));
#294562=CARTESIAN_POINT('Ctrl Pts',(8.13178807675713,74.5062499997125,5.90808986649102));
#294563=CARTESIAN_POINT('Ctrl Pts',(10.0514428414941,74.6562499997118,3.2659117547607));
#294564=CARTESIAN_POINT('Ctrl Pts',(10.0514428414941,74.8062499997113,-1.23094673026484E-15));
#294565=CARTESIAN_POINT('Ctrl Pts',(10.0514428414941,74.9562499997106,-3.26591175476071));
#294566=CARTESIAN_POINT('Ctrl Pts',(8.13178807675713,75.10624999971,-5.90808986649102));
#294567=CARTESIAN_POINT('Ctrl Pts',(6.21213331202016,75.2562499997094,-8.55026797822134));
#294568=CARTESIAN_POINT('Ctrl Pts',(3.10606665601005,75.4062499997088,-9.5594902125713));
#294569=CARTESIAN_POINT('Ctrl Pts',(-5.66378482980338E-14,75.5562499997083,
-10.5687124469213));
#294570=CARTESIAN_POINT('Ctrl Pts',(-3.10606665601016,75.7062499997077,
-9.5594902125713));
#294571=CARTESIAN_POINT('Ctrl Pts',(-6.21213331202027,75.856249999707,-8.55026797822134));
#294572=CARTESIAN_POINT('Ctrl Pts',(-8.13178807675725,76.0062499997065,
-5.90808986649102));
#294573=CARTESIAN_POINT('Ctrl Pts',(-10.0514428414942,76.1562499997058,
-3.2659117547607));
#294574=CARTESIAN_POINT('Ctrl Pts',(-10.0514428414942,76.3062499997052,
2.46189346052968E-15));
#294575=CARTESIAN_POINT('Ctrl Pts',(-10.0514428414942,76.4562499997046,
3.26591175476071));
#294576=CARTESIAN_POINT('Ctrl Pts',(-8.13178807675725,76.606249999704,5.90808986649102));
#294577=CARTESIAN_POINT('Ctrl Pts',(-6.21213331202027,76.7562499997035,
8.55026797822134));
#294578=CARTESIAN_POINT('Ctrl Pts',(-3.10606665601016,76.9062499997029,
9.5594902125713));
#294579=CARTESIAN_POINT('Ctrl Pts',(-5.49131149600185E-14,77.0562499997022,
10.5687124469213));
#294580=CARTESIAN_POINT('Ctrl Pts',(3.10606665601005,77.2062499997016,9.5594902125713));
#294581=CARTESIAN_POINT('Ctrl Pts',(6.21213331202016,77.356249999701,8.55026797822134));
#294582=CARTESIAN_POINT('Ctrl Pts',(8.13178807675713,77.5062499997004,5.90808986649102));
#294583=CARTESIAN_POINT('Ctrl Pts',(10.0514428414941,77.6562499996998,3.2659117547607));
#294584=CARTESIAN_POINT('Ctrl Pts',(10.0514428414941,77.8062499996992,-1.23094673026484E-15));
#294585=CARTESIAN_POINT('Ctrl Pts',(10.0514428414941,77.9562499996987,-3.26591175476071));
#294586=CARTESIAN_POINT('Ctrl Pts',(8.13178807675713,78.1062499996981,-5.90808986649102));
#294587=CARTESIAN_POINT('Ctrl Pts',(6.21213331202016,78.2562499996974,-8.55026797822134));
#294588=CARTESIAN_POINT('Ctrl Pts',(3.10606665601005,78.4062499996969,-9.5594902125713));
#294589=CARTESIAN_POINT('Ctrl Pts',(-5.83655575696956E-14,78.5562499996963,
-10.5687124469213));
#294590=CARTESIAN_POINT('Ctrl Pts',(-3.10606665601017,78.7062499996957,
-9.5594902125713));
#294591=CARTESIAN_POINT('Ctrl Pts',(-6.21213331202028,78.8562499996951,
-8.55026797822134));
#294592=CARTESIAN_POINT('Ctrl Pts',(-8.13178807675725,79.0062499996944,
-5.90808986649102));
#294593=CARTESIAN_POINT('Ctrl Pts',(-10.0514428414942,79.1562499996939,
-3.2659117547607));
#294594=CARTESIAN_POINT('Ctrl Pts',(-10.0514428414942,79.3062499996932,
2.46189346052968E-15));
#294595=CARTESIAN_POINT('Ctrl Pts',(-10.0514428414942,79.4562499996926,
3.26591175476071));
#294596=CARTESIAN_POINT('Ctrl Pts',(-8.13178807675725,79.606249999692,5.90808986649102));
#294597=CARTESIAN_POINT('Ctrl Pts',(-6.21213331202027,79.7562499996915,
8.55026797822134));
#294598=CARTESIAN_POINT('Ctrl Pts',(-3.10606665601016,79.9062499996908,
9.5594902125713));
#294599=CARTESIAN_POINT('Ctrl Pts',(-5.66408242316803E-14,80.0562499996902,
10.5687124469213));
#294600=CARTESIAN_POINT('Ctrl Pts',(3.10606665601005,80.2062499996896,9.5594902125713));
#294601=CARTESIAN_POINT('Ctrl Pts',(6.21213331202016,80.356249999689,8.55026797822134));
#294602=CARTESIAN_POINT('Ctrl Pts',(8.13178807675713,80.5062499996884,5.90808986649102));
#294603=CARTESIAN_POINT('Ctrl Pts',(10.0514428414941,80.6562499996878,3.2659117547607));
#294604=CARTESIAN_POINT('Ctrl Pts',(10.0514428414941,80.8062499996873,-1.23094673026484E-15));
#294605=CARTESIAN_POINT('Ctrl Pts',(10.0514428414941,80.9562499996866,-3.26591175476071));
#294606=CARTESIAN_POINT('Ctrl Pts',(8.13178807675713,81.1062499996861,-5.90808986649102));
#294607=CARTESIAN_POINT('Ctrl Pts',(6.21213331202016,81.2562499996854,-8.55026797822134));
#294608=CARTESIAN_POINT('Ctrl Pts',(3.10606665601005,81.4062499996849,-9.5594902125713));
#294609=CARTESIAN_POINT('Ctrl Pts',(-6.00932668413574E-14,81.5562499996843,
-10.5687124469213));
#294610=CARTESIAN_POINT('Ctrl Pts',(-3.10606665601017,81.7062499996837,
-9.5594902125713));
#294611=CARTESIAN_POINT('Ctrl Pts',(-6.21213331202028,81.856249999683,-8.55026797822134));
#294612=CARTESIAN_POINT('Ctrl Pts',(-8.13178807675725,82.0062499996824,
-5.90808986649102));
#294613=CARTESIAN_POINT('Ctrl Pts',(-10.0514428414942,82.1562499996818,
-3.2659117547607));
#294614=CARTESIAN_POINT('Ctrl Pts',(-10.0514428414942,82.3062499996813,
2.46189346052968E-15));
#294615=CARTESIAN_POINT('Ctrl Pts',(-10.0514428414942,82.4562499996806,
3.26591175476071));
#294616=CARTESIAN_POINT('Ctrl Pts',(-8.13178807675725,82.60624999968,5.90808986649102));
#294617=CARTESIAN_POINT('Ctrl Pts',(-6.21213331202028,82.7562499996795,
8.55026797822134));
#294618=CARTESIAN_POINT('Ctrl Pts',(-3.10606665601017,82.9062499996789,
9.5594902125713));
#294619=CARTESIAN_POINT('Ctrl Pts',(-5.83685335033422E-14,83.0562499996782,
10.5687124469213));
#294620=CARTESIAN_POINT('Ctrl Pts',(3.10606665601005,83.2062499996776,9.5594902125713));
#294621=CARTESIAN_POINT('Ctrl Pts',(6.21213331202016,83.356249999677,8.55026797822134));
#294622=CARTESIAN_POINT('Ctrl Pts',(8.13178807675713,83.5062499996764,5.90808986649102));
#294623=CARTESIAN_POINT('Ctrl Pts',(10.0514428414941,83.6562499996759,3.2659117547607));
#294624=CARTESIAN_POINT('Ctrl Pts',(10.0514428414941,83.8062499996752,-1.23094673026484E-15));
#294625=CARTESIAN_POINT('Ctrl Pts',(10.0514428414941,83.9562499996747,-3.26591175476071));
#294626=CARTESIAN_POINT('Ctrl Pts',(8.13178807675713,84.106249999674,-5.90808986649102));
#294627=CARTESIAN_POINT('Ctrl Pts',(6.21213331202016,84.2562499996734,-8.55026797822134));
#294628=CARTESIAN_POINT('Ctrl Pts',(3.10606665601005,84.4062499996729,-9.5594902125713));
#294629=CARTESIAN_POINT('Ctrl Pts',(-6.18209761130193E-14,84.5562499996723,
-10.5687124469213));
#294630=CARTESIAN_POINT('Ctrl Pts',(-3.10606665601017,84.7062499996717,
-9.5594902125713));
#294631=CARTESIAN_POINT('Ctrl Pts',(-6.21213331202028,84.856249999671,-8.55026797822134));
#294632=CARTESIAN_POINT('Ctrl Pts',(-8.13178807675725,85.0062499996704,
-5.90808986649102));
#294633=CARTESIAN_POINT('Ctrl Pts',(-10.0514428414942,85.1562499996699,
-3.2659117547607));
#294634=CARTESIAN_POINT('Ctrl Pts',(-10.0514428414942,85.3062499996692,
2.46189346052968E-15));
#294635=CARTESIAN_POINT('Ctrl Pts',(-10.0514428414942,85.4562499996686,
3.26591175476071));
#294636=CARTESIAN_POINT('Ctrl Pts',(-8.13178807675725,85.606249999668,5.90808986649102));
#294637=CARTESIAN_POINT('Ctrl Pts',(-6.21213331202028,85.7562499996675,
8.55026797822134));
#294638=CARTESIAN_POINT('Ctrl Pts',(-3.10606665601017,85.9062499996669,
9.5594902125713));
#294639=CARTESIAN_POINT('Ctrl Pts',(-6.0096242775004E-14,86.0562499996662,
10.5687124469213));
#294640=CARTESIAN_POINT('Ctrl Pts',(3.10606665601005,86.2062499996657,9.5594902125713));
#294641=CARTESIAN_POINT('Ctrl Pts',(6.21213331202016,86.3562499996651,8.55026797822134));
#294642=CARTESIAN_POINT('Ctrl Pts',(8.13178807675713,86.5062499996644,5.90808986649102));
#294643=CARTESIAN_POINT('Ctrl Pts',(10.0514428414941,86.6562499996638,3.2659117547607));
#294644=CARTESIAN_POINT('Ctrl Pts',(10.0514428414941,86.8062499996633,-1.23094673026484E-15));
#294645=CARTESIAN_POINT('Ctrl Pts',(10.0514428414941,86.9562499996626,-3.26591175476071));
#294646=CARTESIAN_POINT('Ctrl Pts',(8.13178807675713,87.1062499996621,-5.90808986649102));
#294647=CARTESIAN_POINT('Ctrl Pts',(6.21213331202015,87.2562499996614,-8.55026797822134));
#294648=CARTESIAN_POINT('Ctrl Pts',(3.10606665601004,87.4062499996609,-9.5594902125713));
#294649=CARTESIAN_POINT('Ctrl Pts',(-6.35486853846811E-14,87.5562499996603,
-10.5687124469213));
#294650=CARTESIAN_POINT('Ctrl Pts',(-3.10606665601017,87.7062499996597,
-9.5594902125713));
#294651=CARTESIAN_POINT('Ctrl Pts',(-6.21213331202028,87.856249999659,-8.55026797822134));
#294652=CARTESIAN_POINT('Ctrl Pts',(-8.13178807675726,88.0062499996585,
-5.90808986649102));
#294653=CARTESIAN_POINT('Ctrl Pts',(-10.0514428414942,88.1562499996578,
-3.2659117547607));
#294654=CARTESIAN_POINT('Ctrl Pts',(-10.0514428414942,88.3062499996572,
2.46189346052968E-15));
#294655=CARTESIAN_POINT('Ctrl Pts',(-10.0514428414942,88.4562499996566,
3.26591175476071));
#294656=CARTESIAN_POINT('Ctrl Pts',(-8.13178807675726,88.6062499996561,
5.90808986649102));
#294657=CARTESIAN_POINT('Ctrl Pts',(-6.21213331202028,88.7562499996555,
8.55026797822134));
#294658=CARTESIAN_POINT('Ctrl Pts',(-3.10606665601017,88.9062499996548,
9.5594902125713));
#294659=CARTESIAN_POINT('Ctrl Pts',(-6.18239520466659E-14,89.0562499996542,
10.5687124469213));
#294660=CARTESIAN_POINT('Ctrl Pts',(3.10606665601005,89.2062499996537,9.5594902125713));
#294661=CARTESIAN_POINT('Ctrl Pts',(6.21213331202016,89.3562499996531,8.55026797822134));
#294662=CARTESIAN_POINT('Ctrl Pts',(8.13178807675713,89.5062499996525,5.90808986649102));
#294663=CARTESIAN_POINT('Ctrl Pts',(10.0514428414941,89.6562499996518,3.2659117547607));
#294664=CARTESIAN_POINT('Ctrl Pts',(10.0514428414941,89.8062499996512,-1.23094673026484E-15));
#294665=CARTESIAN_POINT('Ctrl Pts',(10.0514428414941,89.9562499996507,-3.26591175476071));
#294666=CARTESIAN_POINT('Ctrl Pts',(8.13178807675713,90.10624999965,-5.90808986649102));
#294667=CARTESIAN_POINT('Ctrl Pts',(6.21213331202015,90.2562499996494,-8.55026797822134));
#294668=CARTESIAN_POINT('Ctrl Pts',(3.10606665601004,90.4062499996488,-9.5594902125713));
#294669=CARTESIAN_POINT('Ctrl Pts',(-6.52763946563429E-14,90.5562499996483,
-10.5687124469213));
#294670=CARTESIAN_POINT('Ctrl Pts',(-3.10606665601017,90.7062499996476,
-9.5594902125713));
#294671=CARTESIAN_POINT('Ctrl Pts',(-6.21213331202028,90.856249999647,-8.55026797822134));
#294672=CARTESIAN_POINT('Ctrl Pts',(-8.13178807675726,91.0062499996464,
-5.90808986649102));
#294673=CARTESIAN_POINT('Ctrl Pts',(-10.0514428414942,91.1562499996458,
-3.2659117547607));
#294674=CARTESIAN_POINT('Ctrl Pts',(-10.0514428414942,91.3062499996452,
2.46189346052968E-15));
#294675=CARTESIAN_POINT('Ctrl Pts',(-10.0514428414942,91.4562499996446,
3.26591175476071));
#294676=CARTESIAN_POINT('Ctrl Pts',(-8.13178807675726,91.606249999644,5.90808986649102));
#294677=CARTESIAN_POINT('Ctrl Pts',(-6.21213331202028,91.7562499996434,
8.55026797822134));
#294678=CARTESIAN_POINT('Ctrl Pts',(-3.10606665601017,91.9062499996429,
9.5594902125713));
#294679=CARTESIAN_POINT('Ctrl Pts',(-6.35516613183277E-14,92.0562499996422,
10.5687124469213));
#294680=CARTESIAN_POINT('Ctrl Pts',(3.10606665601004,92.2062499996417,9.5594902125713));
#294681=CARTESIAN_POINT('Ctrl Pts',(6.21213331202015,92.3562499996411,8.55026797822134));
#294682=CARTESIAN_POINT('Ctrl Pts',(8.13178807675712,92.5062499996404,5.90808986649102));
#294683=CARTESIAN_POINT('Ctrl Pts',(10.0514428414941,92.6562499996398,3.2659117547607));
#294684=CARTESIAN_POINT('Ctrl Pts',(10.0514428414941,92.8062499996392,-1.23094673026484E-15));
#294685=CARTESIAN_POINT('Ctrl Pts',(10.0514428414941,92.9562499996387,-3.26591175476071));
#294686=CARTESIAN_POINT('Ctrl Pts',(8.13178807675712,93.1062499996381,-5.90808986649102));
#294687=CARTESIAN_POINT('Ctrl Pts',(6.21213331202015,93.2562499996374,-8.55026797822134));
#294688=CARTESIAN_POINT('Ctrl Pts',(3.10606665601004,93.4062499996369,-9.5594902125713));
#294689=CARTESIAN_POINT('Ctrl Pts',(-6.70041039280048E-14,93.5562499996362,
-10.5687124469213));
#294690=CARTESIAN_POINT('Ctrl Pts',(-3.10606665601018,93.7062499996357,
-9.5594902125713));
#294691=CARTESIAN_POINT('Ctrl Pts',(-6.21213331202028,93.856249999635,-8.55026797822134));
#294692=CARTESIAN_POINT('Ctrl Pts',(-8.13178807675726,94.0062499996344,
-5.90808986649102));
#294693=CARTESIAN_POINT('Ctrl Pts',(-10.0514428414942,94.1562499996338,
-3.2659117547607));
#294694=CARTESIAN_POINT('Ctrl Pts',(-10.0514428414942,94.3062499996333,
2.46189346052968E-15));
#294695=CARTESIAN_POINT('Ctrl Pts',(-10.0514428414942,94.4562499996326,
3.26591175476071));
#294696=CARTESIAN_POINT('Ctrl Pts',(-8.13178807675726,94.606249999632,5.90808986649102));
#294697=CARTESIAN_POINT('Ctrl Pts',(-6.21213331202028,94.7562499996315,
8.55026797822134));
#294698=CARTESIAN_POINT('Ctrl Pts',(-3.10606665601017,94.9062499996309,
9.5594902125713));
#294699=CARTESIAN_POINT('Ctrl Pts',(-6.52793705899895E-14,95.0562499996302,
10.5687124469213));
#294700=CARTESIAN_POINT('Ctrl Pts',(3.10606665601004,95.2062499996296,9.5594902125713));
#294701=CARTESIAN_POINT('Ctrl Pts',(6.21213331202015,95.3562499996291,8.55026797822134));
#294702=CARTESIAN_POINT('Ctrl Pts',(8.13178807675712,95.5062499996285,5.90808986649102));
#294703=CARTESIAN_POINT('Ctrl Pts',(10.0514428414941,95.6562499996278,3.2659117547607));
#294704=CARTESIAN_POINT('Ctrl Pts',(10.0514428414941,95.8062499996273,-1.23094673026484E-15));
#294705=CARTESIAN_POINT('Ctrl Pts',(10.0514428414941,95.9562499996266,-3.26591175476071));
#294706=CARTESIAN_POINT('Ctrl Pts',(8.13178807675712,96.1062499996261,-5.90808986649102));
#294707=CARTESIAN_POINT('Ctrl Pts',(6.21213331202015,96.2562499996255,-8.55026797822134));
#294708=CARTESIAN_POINT('Ctrl Pts',(3.10606665601004,96.4062499996248,-9.5594902125713));
#294709=CARTESIAN_POINT('Ctrl Pts',(-6.87318131996666E-14,96.5562499996243,
-10.5687124469213));
#294710=CARTESIAN_POINT('Ctrl Pts',(-3.10606665601018,96.7062499996236,
-9.5594902125713));
#294711=CARTESIAN_POINT('Ctrl Pts',(-6.21213331202028,96.856249999623,-8.55026797822134));
#294712=CARTESIAN_POINT('Ctrl Pts',(-8.13178807675726,97.0062499996224,
-5.90808986649102));
#294713=CARTESIAN_POINT('Ctrl Pts',(-10.0514428414942,97.1562499996218,
-3.2659117547607));
#294714=CARTESIAN_POINT('Ctrl Pts',(-10.0514428414942,97.3062499996212,
2.46189346052968E-15));
#294715=CARTESIAN_POINT('Ctrl Pts',(-10.0514428414942,97.4562499996206,
3.26591175476071));
#294716=CARTESIAN_POINT('Ctrl Pts',(-8.13178807675726,97.60624999962,5.90808986649102));
#294717=CARTESIAN_POINT('Ctrl Pts',(-6.21213331202028,97.7562499996195,
8.55026797822134));
#294718=CARTESIAN_POINT('Ctrl Pts',(-3.10606665601018,97.9062499996189,
9.5594902125713));
#294719=CARTESIAN_POINT('Ctrl Pts',(-6.70070798616514E-14,98.0562499996182,
10.5687124469213));
#294720=CARTESIAN_POINT('Ctrl Pts',(3.10606665601004,98.2062499996177,9.5594902125713));
#294721=CARTESIAN_POINT('Ctrl Pts',(6.21213331202015,98.3562499996171,8.55026797822134));
#294722=CARTESIAN_POINT('Ctrl Pts',(8.13178807675712,98.5062499996165,5.90808986649102));
#294723=CARTESIAN_POINT('Ctrl Pts',(10.0514428414941,98.6562499996158,3.2659117547607));
#294724=CARTESIAN_POINT('Ctrl Pts',(10.0514428414941,98.8062499996153,-1.23094673026484E-15));
#294725=CARTESIAN_POINT('Ctrl Pts',(10.0514428414941,98.9562499996147,-3.26591175476071));
#294726=CARTESIAN_POINT('Ctrl Pts',(8.13178807675712,99.1062499996141,-5.90808986649102));
#294727=CARTESIAN_POINT('Ctrl Pts',(6.21213331202015,99.2562499996134,-8.55026797822134));
#294728=CARTESIAN_POINT('Ctrl Pts',(3.10606665601004,99.4062499996129,-9.5594902125713));
#294729=CARTESIAN_POINT('Ctrl Pts',(-7.04595224713284E-14,99.5562499996123,
-10.5687124469213));
#294730=CARTESIAN_POINT('Ctrl Pts',(-3.10606665601018,99.7062499996117,
-9.5594902125713));
#294731=CARTESIAN_POINT('Ctrl Pts',(-6.21213331202028,99.856249999611,-8.55026797822134));
#294732=CARTESIAN_POINT('Ctrl Pts',(-8.13178807675726,100.00624999961,-5.90808986649102));
#294733=CARTESIAN_POINT('Ctrl Pts',(-10.0514428414942,100.15624999961,-3.2659117547607));
#294734=CARTESIAN_POINT('Ctrl Pts',(-10.0514428414942,100.306249999609,
2.46189346052968E-15));
#294735=CARTESIAN_POINT('Ctrl Pts',(-10.0514428414942,100.456249999609,
3.26591175476071));
#294736=CARTESIAN_POINT('Ctrl Pts',(-8.13178807675726,100.606249999608,
5.90808986649102));
#294737=CARTESIAN_POINT('Ctrl Pts',(-6.21213331202028,100.756249999607,
8.55026797822134));
#294738=CARTESIAN_POINT('Ctrl Pts',(-3.10606665601018,100.906249999607,
9.5594902125713));
#294739=CARTESIAN_POINT('Ctrl Pts',(-6.87347891333132E-14,101.056249999606,
10.5687124469213));
#294740=CARTESIAN_POINT('Ctrl Pts',(3.10606665601004,101.206249999606,9.5594902125713));
#294741=CARTESIAN_POINT('Ctrl Pts',(6.21213331202015,101.356249999605,8.55026797822134));
#294742=CARTESIAN_POINT('Ctrl Pts',(8.13178807675712,101.506249999604,5.90808986649102));
#294743=CARTESIAN_POINT('Ctrl Pts',(10.0514428414941,101.656249999604,3.2659117547607));
#294744=CARTESIAN_POINT('Ctrl Pts',(10.0514428414941,101.806249999603,-1.23094673026484E-15));
#294745=CARTESIAN_POINT('Ctrl Pts',(10.0514428414941,101.956249999603,-3.26591175476071));
#294746=CARTESIAN_POINT('Ctrl Pts',(8.13178807675712,102.106249999602,-5.90808986649102));
#294747=CARTESIAN_POINT('Ctrl Pts',(6.21213331202014,102.256249999601,-8.55026797822134));
#294748=CARTESIAN_POINT('Ctrl Pts',(3.10606665601004,102.406249999601,-9.5594902125713));
#294749=CARTESIAN_POINT('Ctrl Pts',(-7.21872317429903E-14,102.5562499996,
-10.5687124469213));
#294750=CARTESIAN_POINT('Ctrl Pts',(-3.10606665601018,102.7062499996,-9.5594902125713));
#294751=CARTESIAN_POINT('Ctrl Pts',(-6.21213331202029,102.856249999599,
-8.55026797822134));
#294752=CARTESIAN_POINT('Ctrl Pts',(-8.13178807675726,103.006249999598,
-5.90808986649102));
#294753=CARTESIAN_POINT('Ctrl Pts',(-10.0514428414942,103.156249999598,
-3.2659117547607));
#294754=CARTESIAN_POINT('Ctrl Pts',(-10.0514428414942,103.306249999597,
2.46189346052968E-15));
#294755=CARTESIAN_POINT('Ctrl Pts',(-10.0514428414942,103.456249999597,
3.26591175476071));
#294756=CARTESIAN_POINT('Ctrl Pts',(-8.13178807675726,103.606249999596,
5.90808986649102));
#294757=CARTESIAN_POINT('Ctrl Pts',(-6.21213331202028,103.756249999595,
8.55026797822134));
#294758=CARTESIAN_POINT('Ctrl Pts',(-3.10606665601018,103.906249999595,
9.5594902125713));
#294759=CARTESIAN_POINT('Ctrl Pts',(-7.04624984049751E-14,104.056249999594,
10.5687124469213));
#294760=CARTESIAN_POINT('Ctrl Pts',(3.10606665601004,104.206249999594,9.5594902125713));
#294761=CARTESIAN_POINT('Ctrl Pts',(6.21213331202015,104.356249999593,8.55026797822134));
#294762=CARTESIAN_POINT('Ctrl Pts',(8.13178807675712,104.506249999592,5.90808986649102));
#294763=CARTESIAN_POINT('Ctrl Pts',(10.0514428414941,104.656249999592,3.2659117547607));
#294764=CARTESIAN_POINT('Ctrl Pts',(10.0514428414941,104.806249999591,-1.23094673026484E-15));
#294765=CARTESIAN_POINT('Ctrl Pts',(10.0514428414941,104.956249999591,-3.26591175476071));
#294766=CARTESIAN_POINT('Ctrl Pts',(8.13178807675712,105.10624999959,-5.90808986649102));
#294767=CARTESIAN_POINT('Ctrl Pts',(6.21213331202014,105.256249999589,-8.55026797822134));
#294768=CARTESIAN_POINT('Ctrl Pts',(3.10606665601003,105.406249999589,-9.5594902125713));
#294769=CARTESIAN_POINT('Ctrl Pts',(-7.39149410146522E-14,105.556249999588,
-10.5687124469213));
#294770=CARTESIAN_POINT('Ctrl Pts',(-3.10606665601018,105.706249999588,
-9.5594902125713));
#294771=CARTESIAN_POINT('Ctrl Pts',(-6.21213331202029,105.856249999587,
-8.55026797822134));
#294772=CARTESIAN_POINT('Ctrl Pts',(-8.13178807675726,106.006249999586,
-5.90808986649102));
#294773=CARTESIAN_POINT('Ctrl Pts',(-10.0514428414942,106.156249999586,
-3.2659117547607));
#294774=CARTESIAN_POINT('Ctrl Pts',(-10.0514428414942,106.306249999585,
2.46189346052968E-15));
#294775=CARTESIAN_POINT('Ctrl Pts',(-10.0514428414942,106.456249999585,
3.26591175476071));
#294776=CARTESIAN_POINT('Ctrl Pts',(-8.13178807675726,106.606249999584,
5.90808986649102));
#294777=CARTESIAN_POINT('Ctrl Pts',(-6.21213331202029,106.756249999583,
8.55026797822134));
#294778=CARTESIAN_POINT('Ctrl Pts',(-3.10606665601018,106.906249999583,
9.5594902125713));
#294779=CARTESIAN_POINT('Ctrl Pts',(-7.21902076766369E-14,107.056249999582,
10.5687124469213));
#294780=CARTESIAN_POINT('Ctrl Pts',(3.10606665601003,107.206249999582,9.5594902125713));
#294781=CARTESIAN_POINT('Ctrl Pts',(6.21213331202014,107.356249999581,8.55026797822134));
#294782=CARTESIAN_POINT('Ctrl Pts',(8.13178807675711,107.50624999958,5.90808986649102));
#294783=CARTESIAN_POINT('Ctrl Pts',(10.0514428414941,107.65624999958,3.2659117547607));
#294784=CARTESIAN_POINT('Ctrl Pts',(10.0514428414941,107.806249999579,-1.23094673026484E-15));
#294785=CARTESIAN_POINT('Ctrl Pts',(10.0514428414941,107.956249999579,-3.26591175476071));
#294786=CARTESIAN_POINT('Ctrl Pts',(8.13178807675711,108.106249999578,-5.90808986649102));
#294787=CARTESIAN_POINT('Ctrl Pts',(6.21213331202014,108.256249999577,-8.55026797822134));
#294788=CARTESIAN_POINT('Ctrl Pts',(3.10606665601003,108.406249999577,-9.5594902125713));
#294789=CARTESIAN_POINT('Ctrl Pts',(-7.5642650286314E-14,108.556249999576,
-10.5687124469213));
#294790=CARTESIAN_POINT('Ctrl Pts',(-3.10606665601018,108.706249999576,
-9.5594902125713));
#294791=CARTESIAN_POINT('Ctrl Pts',(-6.21213331202029,108.856249999575,
-8.55026797822134));
#294792=CARTESIAN_POINT('Ctrl Pts',(-8.13178807675727,109.006249999574,
-5.90808986649102));
#294793=CARTESIAN_POINT('Ctrl Pts',(-10.0514428414942,109.156249999574,
-3.2659117547607));
#294794=CARTESIAN_POINT('Ctrl Pts',(-10.0514428414942,109.306249999573,
2.46189346052968E-15));
#294795=CARTESIAN_POINT('Ctrl Pts',(-10.0514428414942,109.456249999573,
3.26591175476071));
#294796=CARTESIAN_POINT('Ctrl Pts',(-8.13178807675727,109.606249999572,
5.90808986649102));
#294797=CARTESIAN_POINT('Ctrl Pts',(-6.21213331202029,109.756249999571,
8.55026797822134));
#294798=CARTESIAN_POINT('Ctrl Pts',(-3.10606665601018,109.906249999571,
9.5594902125713));
#294799=CARTESIAN_POINT('Ctrl Pts',(-7.39179169482987E-14,110.05624999957,
10.5687124469213));
#294800=CARTESIAN_POINT('Ctrl Pts',(3.10606665601003,110.20624999957,9.5594902125713));
#294801=CARTESIAN_POINT('Ctrl Pts',(6.21213331202014,110.356249999569,8.55026797822134));
#294802=CARTESIAN_POINT('Ctrl Pts',(8.13178807675711,110.506249999568,5.90808986649102));
#294803=CARTESIAN_POINT('Ctrl Pts',(10.0514428414941,110.656249999568,3.2659117547607));
#294804=CARTESIAN_POINT('Ctrl Pts',(10.0514428414941,110.806249999567,-1.23094673026484E-15));
#294805=CARTESIAN_POINT('Ctrl Pts',(10.0514428414941,110.956249999567,-3.26591175476071));
#294806=CARTESIAN_POINT('Ctrl Pts',(8.13178807675711,111.106249999566,-5.90808986649102));
#294807=CARTESIAN_POINT('Ctrl Pts',(6.21213331202014,111.256249999565,-8.55026797822134));
#294808=CARTESIAN_POINT('Ctrl Pts',(3.10606665601003,111.406249999565,-9.5594902125713));
#294809=CARTESIAN_POINT('Ctrl Pts',(-7.73703595579758E-14,111.556249999564,
-10.5687124469213));
#294810=CARTESIAN_POINT('Ctrl Pts',(-3.10606665601019,111.706249999564,
-9.5594902125713));
#294811=CARTESIAN_POINT('Ctrl Pts',(-6.21213331202029,111.856249999563,
-8.55026797822134));
#294812=CARTESIAN_POINT('Ctrl Pts',(-8.13178807675727,112.006249999562,
-5.90808986649102));
#294813=CARTESIAN_POINT('Ctrl Pts',(-10.0514428414942,112.156249999562,
-3.2659117547607));
#294814=CARTESIAN_POINT('Ctrl Pts',(-10.0514428414942,112.306249999561,
2.46189346052968E-15));
#294815=CARTESIAN_POINT('Ctrl Pts',(-10.0514428414942,112.456249999561,
3.26591175476071));
#294816=CARTESIAN_POINT('Ctrl Pts',(-8.13178807675727,112.60624999956,5.90808986649102));
#294817=CARTESIAN_POINT('Ctrl Pts',(-6.21213331202029,112.756249999559,
8.55026797822134));
#294818=CARTESIAN_POINT('Ctrl Pts',(-3.10606665601018,112.906249999559,
9.5594902125713));
#294819=CARTESIAN_POINT('Ctrl Pts',(-7.56456262199606E-14,113.056249999558,
10.5687124469213));
#294820=CARTESIAN_POINT('Ctrl Pts',(3.10606665601003,113.206249999558,9.5594902125713));
#294821=CARTESIAN_POINT('Ctrl Pts',(6.21213331202014,113.356249999557,8.55026797822134));
#294822=CARTESIAN_POINT('Ctrl Pts',(8.13178807675711,113.506249999556,5.90808986649102));
#294823=CARTESIAN_POINT('Ctrl Pts',(10.0514428414941,113.656249999556,3.2659117547607));
#294824=CARTESIAN_POINT('Ctrl Pts',(10.0514428414941,113.806249999555,-1.23094673026484E-15));
#294825=CARTESIAN_POINT('Ctrl Pts',(10.0514428414941,113.956249999555,-3.26591175476071));
#294826=CARTESIAN_POINT('Ctrl Pts',(8.13178807675711,114.106249999554,-5.90808986649102));
#294827=CARTESIAN_POINT('Ctrl Pts',(6.21213331202014,114.256249999553,-8.55026797822134));
#294828=CARTESIAN_POINT('Ctrl Pts',(3.10606665601003,114.406249999553,-9.5594902125713));
#294829=CARTESIAN_POINT('Ctrl Pts',(-7.90980688296377E-14,114.556249999552,
-10.5687124469213));
#294830=CARTESIAN_POINT('Ctrl Pts',(-3.10606665601019,114.706249999552,
-9.5594902125713));
#294831=CARTESIAN_POINT('Ctrl Pts',(-6.2121333120203,114.856249999551,-8.55026797822134));
#294832=CARTESIAN_POINT('Ctrl Pts',(-8.13178807675727,115.00624999955,-5.90808986649102));
#294833=CARTESIAN_POINT('Ctrl Pts',(-10.0514428414942,115.15624999955,-3.2659117547607));
#294834=CARTESIAN_POINT('Ctrl Pts',(-10.0514428414942,115.306249999549,
2.46189346052968E-15));
#294835=CARTESIAN_POINT('Ctrl Pts',(-10.0514428414942,115.456249999549,
3.26591175476071));
#294836=CARTESIAN_POINT('Ctrl Pts',(-8.13178807675727,115.606249999548,
5.90808986649102));
#294837=CARTESIAN_POINT('Ctrl Pts',(-6.21213331202029,115.756249999547,
8.55026797822134));
#294838=CARTESIAN_POINT('Ctrl Pts',(-3.10606665601019,115.906249999547,
9.5594902125713));
#294839=CARTESIAN_POINT('Ctrl Pts',(-7.73733354916224E-14,116.056249999546,
10.5687124469213));
#294840=CARTESIAN_POINT('Ctrl Pts',(3.10606665601003,116.206249999546,9.5594902125713));
#294841=CARTESIAN_POINT('Ctrl Pts',(6.21213331202014,116.356249999545,8.55026797822134));
#294842=CARTESIAN_POINT('Ctrl Pts',(8.13178807675711,116.506249999544,5.90808986649102));
#294843=CARTESIAN_POINT('Ctrl Pts',(10.0514428414941,116.656249999544,3.2659117547607));
#294844=CARTESIAN_POINT('Ctrl Pts',(10.0514428414941,116.806249999543,-1.23094673026484E-15));
#294845=CARTESIAN_POINT('Ctrl Pts',(10.0514428414941,116.956249999543,-3.26591175476071));
#294846=CARTESIAN_POINT('Ctrl Pts',(8.13178807675711,117.106249999542,-5.90808986649102));
#294847=CARTESIAN_POINT('Ctrl Pts',(6.21213331202014,117.256249999541,-8.55026797822134));
#294848=CARTESIAN_POINT('Ctrl Pts',(3.10606665601003,117.406249999541,-9.5594902125713));
#294849=CARTESIAN_POINT('Ctrl Pts',(-8.08257781012995E-14,117.55624999954,
-10.5687124469213));
#294850=CARTESIAN_POINT('Ctrl Pts',(-3.10606665601019,117.70624999954,-9.5594902125713));
#294851=CARTESIAN_POINT('Ctrl Pts',(-6.2121333120203,117.856249999539,-8.55026797822134));
#294852=CARTESIAN_POINT('Ctrl Pts',(-8.13178807675727,118.006249999538,
-5.90808986649102));
#294853=CARTESIAN_POINT('Ctrl Pts',(-10.0514428414942,118.156249999538,
-3.2659117547607));
#294854=CARTESIAN_POINT('Ctrl Pts',(-10.0514428414942,118.306249999537,
2.46189346052968E-15));
#294855=CARTESIAN_POINT('Ctrl Pts',(-10.0514428414942,118.456249999537,
3.26591175476071));
#294856=CARTESIAN_POINT('Ctrl Pts',(-8.13178807675727,118.606249999536,
5.90808986649102));
#294857=CARTESIAN_POINT('Ctrl Pts',(-6.2121333120203,118.756249999535,8.55026797822134));
#294858=CARTESIAN_POINT('Ctrl Pts',(-3.10606665601019,118.906249999535,
9.5594902125713));
#294859=CARTESIAN_POINT('Ctrl Pts',(-7.91010447632842E-14,119.056249999534,
10.5687124469213));
#294860=CARTESIAN_POINT('Ctrl Pts',(3.10606665601003,119.206249999534,9.5594902125713));
#294861=CARTESIAN_POINT('Ctrl Pts',(6.21213331202014,119.356249999533,8.55026797822134));
#294862=CARTESIAN_POINT('Ctrl Pts',(8.13178807675711,119.506249999532,5.90808986649102));
#294863=CARTESIAN_POINT('Ctrl Pts',(10.0514428414941,119.656249999532,3.2659117547607));
#294864=CARTESIAN_POINT('Ctrl Pts',(10.0514428414941,119.806249999531,-1.23094673026484E-15));
#294865=CARTESIAN_POINT('Ctrl Pts',(10.0514428414941,119.956249999531,-3.26591175476071));
#294866=CARTESIAN_POINT('Ctrl Pts',(8.13178807675711,120.10624999953,-5.90808986649102));
#294867=CARTESIAN_POINT('Ctrl Pts',(6.21213331202013,120.256249999529,-8.55026797822134));
#294868=CARTESIAN_POINT('Ctrl Pts',(3.10606665601003,120.406249999529,-9.5594902125713));
#294869=CARTESIAN_POINT('Ctrl Pts',(-8.25534873729613E-14,120.556249999528,
-10.5687124469213));
#294870=CARTESIAN_POINT('Ctrl Pts',(-3.10606665601019,120.706249999528,
-9.5594902125713));
#294871=CARTESIAN_POINT('Ctrl Pts',(-6.2121333120203,120.856249999527,-8.55026797822134));
#294872=CARTESIAN_POINT('Ctrl Pts',(-8.13178807675727,121.006249999526,
-5.90808986649102));
#294873=CARTESIAN_POINT('Ctrl Pts',(-10.0514428414943,121.156249999526,
-3.2659117547607));
#294874=CARTESIAN_POINT('Ctrl Pts',(-10.0514428414943,121.306249999525,
2.46189346052968E-15));
#294875=CARTESIAN_POINT('Ctrl Pts',(-10.0514428414943,121.456249999525,
3.26591175476071));
#294876=CARTESIAN_POINT('Ctrl Pts',(-8.13178807675727,121.606249999524,
5.90808986649102));
#294877=CARTESIAN_POINT('Ctrl Pts',(-6.2121333120203,121.756249999523,8.55026797822134));
#294878=CARTESIAN_POINT('Ctrl Pts',(-3.10606665601019,121.906249999523,
9.5594902125713));
#294879=CARTESIAN_POINT('Ctrl Pts',(-8.08287540349461E-14,122.056249999522,
10.5687124469213));
#294880=CARTESIAN_POINT('Ctrl Pts',(3.10606665601003,122.206249999522,9.5594902125713));
#294881=CARTESIAN_POINT('Ctrl Pts',(6.21213331202014,122.356249999521,8.55026797822134));
#294882=CARTESIAN_POINT('Ctrl Pts',(8.13178807675711,122.50624999952,5.90808986649102));
#294883=CARTESIAN_POINT('Ctrl Pts',(10.0514428414941,122.65624999952,3.2659117547607));
#294884=CARTESIAN_POINT('Ctrl Pts',(10.0514428414941,122.806249999519,-1.23094673026484E-15));
#294885=CARTESIAN_POINT('Ctrl Pts',(10.0514428414941,122.956249999519,-3.26591175476071));
#294886=CARTESIAN_POINT('Ctrl Pts',(8.13178807675711,123.106249999518,-5.90808986649102));
#294887=CARTESIAN_POINT('Ctrl Pts',(6.21213331202013,123.256249999517,-8.55026797822134));
#294888=CARTESIAN_POINT('Ctrl Pts',(3.10606665601002,123.406249999517,-9.5594902125713));
#294889=CARTESIAN_POINT('Ctrl Pts',(-8.42811966446232E-14,123.556249999516,
-10.5687124469213));
#294890=CARTESIAN_POINT('Ctrl Pts',(-3.10606665601019,123.706249999516,
-9.5594902125713));
#294891=CARTESIAN_POINT('Ctrl Pts',(-6.2121333120203,123.856249999515,-8.55026797822134));
#294892=CARTESIAN_POINT('Ctrl Pts',(-8.13178807675727,124.006249999514,
-5.90808986649102));
#294893=CARTESIAN_POINT('Ctrl Pts',(-10.0514428414943,124.156249999514,
-3.2659117547607));
#294894=CARTESIAN_POINT('Ctrl Pts',(-10.0514428414943,124.306249999513,
2.46189346052968E-15));
#294895=CARTESIAN_POINT('Ctrl Pts',(-10.0514428414943,124.456249999513,
3.26591175476071));
#294896=CARTESIAN_POINT('Ctrl Pts',(-8.13178807675727,124.606249999512,
5.90808986649102));
#294897=CARTESIAN_POINT('Ctrl Pts',(-6.2121333120203,124.756249999511,8.55026797822134));
#294898=CARTESIAN_POINT('Ctrl Pts',(-3.10606665601019,124.906249999511,
9.5594902125713));
#294899=CARTESIAN_POINT('Ctrl Pts',(-8.25564633066079E-14,125.05624999951,
10.5687124469213));
#294900=CARTESIAN_POINT('Ctrl Pts',(3.10606665601002,125.20624999951,9.5594902125713));
#294901=CARTESIAN_POINT('Ctrl Pts',(6.21213331202013,125.356249999509,8.55026797822134));
#294902=CARTESIAN_POINT('Ctrl Pts',(8.13178807675711,125.506249999508,5.90808986649102));
#294903=CARTESIAN_POINT('Ctrl Pts',(10.0514428414941,125.656249999508,3.2659117547607));
#294904=CARTESIAN_POINT('Ctrl Pts',(10.0514428414941,125.806249999507,-1.23094673026484E-15));
#294905=CARTESIAN_POINT('Ctrl Pts',(10.0514428414941,125.956249999507,-3.26591175476071));
#294906=CARTESIAN_POINT('Ctrl Pts',(8.13178807675711,126.106249999506,-5.90808986649102));
#294907=CARTESIAN_POINT('Ctrl Pts',(6.21213331202013,126.256249999505,-8.55026797822134));
#294908=CARTESIAN_POINT('Ctrl Pts',(3.10606665601002,126.406249999505,-9.5594902125713));
#294909=CARTESIAN_POINT('Ctrl Pts',(-8.6008905916285E-14,126.556249999504,
-10.5687124469213));
#294910=CARTESIAN_POINT('Ctrl Pts',(-3.10606665601019,126.706249999504,
-9.5594902125713));
#294911=CARTESIAN_POINT('Ctrl Pts',(-6.2121333120203,126.856249999503,-8.55026797822134));
#294912=CARTESIAN_POINT('Ctrl Pts',(-8.13178807675728,127.006249999502,
-5.90808986649102));
#294913=CARTESIAN_POINT('Ctrl Pts',(-10.0514428414943,127.156249999502,
-3.2659117547607));
#294914=CARTESIAN_POINT('Ctrl Pts',(-10.0514428414943,127.306249999501,
2.46189346052968E-15));
#294915=CARTESIAN_POINT('Ctrl Pts',(-10.0514428414943,127.456249999501,
3.26591175476071));
#294916=CARTESIAN_POINT('Ctrl Pts',(-8.13178807675728,127.6062499995,5.90808986649102));
#294917=CARTESIAN_POINT('Ctrl Pts',(-6.2121333120203,127.756249999499,8.55026797822134));
#294918=CARTESIAN_POINT('Ctrl Pts',(-3.10606665601019,127.906249999499,
9.5594902125713));
#294919=CARTESIAN_POINT('Ctrl Pts',(-8.42841725782698E-14,128.056249999498,
10.5687124469213));
#294920=CARTESIAN_POINT('Ctrl Pts',(3.10606665601002,128.206249999498,9.5594902125713));
#294921=CARTESIAN_POINT('Ctrl Pts',(6.21213331202013,128.356249999497,8.55026797822134));
#294922=CARTESIAN_POINT('Ctrl Pts',(8.1317880767571,128.506249999496,5.90808986649102));
#294923=CARTESIAN_POINT('Ctrl Pts',(10.0514428414941,128.656249999496,3.2659117547607));
#294924=CARTESIAN_POINT('Ctrl Pts',(10.0514428414941,128.806249999495,-1.23094673026484E-15));
#294925=CARTESIAN_POINT('Ctrl Pts',(10.0514428414941,128.956249999495,-3.26591175476071));
#294926=CARTESIAN_POINT('Ctrl Pts',(8.1317880767571,129.106249999494,-5.90808986649102));
#294927=CARTESIAN_POINT('Ctrl Pts',(6.21213331202013,129.256249999493,-8.55026797822134));
#294928=CARTESIAN_POINT('Ctrl Pts',(3.10606665601002,129.406249999493,-9.5594902125713));
#294929=CARTESIAN_POINT('Ctrl Pts',(-8.77366151879469E-14,129.556249999492,
-10.5687124469213));
#294930=CARTESIAN_POINT('Ctrl Pts',(-3.1060666560102,129.706249999492,-9.5594902125713));
#294931=CARTESIAN_POINT('Ctrl Pts',(-6.2121333120203,129.856249999491,-8.55026797822134));
#294932=CARTESIAN_POINT('Ctrl Pts',(-8.13178807675728,130.00624999949,-5.90808986649102));
#294933=CARTESIAN_POINT('Ctrl Pts',(-10.0514428414943,130.15624999949,-3.2659117547607));
#294934=CARTESIAN_POINT('Ctrl Pts',(-10.0514428414943,130.306249999489,
2.46189346052968E-15));
#294935=CARTESIAN_POINT('Ctrl Pts',(-10.0514428414943,130.456249999489,
3.26591175476071));
#294936=CARTESIAN_POINT('Ctrl Pts',(-8.13178807675728,130.606249999488,
5.90808986649102));
#294937=CARTESIAN_POINT('Ctrl Pts',(-6.2121333120203,130.756249999487,8.55026797822134));
#294938=CARTESIAN_POINT('Ctrl Pts',(-3.10606665601019,130.906249999487,
9.5594902125713));
#294939=CARTESIAN_POINT('Ctrl Pts',(-8.60118818499316E-14,131.056249999486,
10.5687124469213));
#294940=CARTESIAN_POINT('Ctrl Pts',(3.10606665601002,131.206249999486,9.5594902125713));
#294941=CARTESIAN_POINT('Ctrl Pts',(6.21213331202013,131.356249999485,8.55026797822134));
#294942=CARTESIAN_POINT('Ctrl Pts',(8.1317880767571,131.506249999484,5.90808986649102));
#294943=CARTESIAN_POINT('Ctrl Pts',(10.0514428414941,131.656249999484,3.2659117547607));
#294944=CARTESIAN_POINT('Ctrl Pts',(10.0514428414941,131.806249999483,-1.23094673026484E-15));
#294945=CARTESIAN_POINT('Ctrl Pts',(10.0514428414941,131.956249999483,-3.26591175476071));
#294946=CARTESIAN_POINT('Ctrl Pts',(8.1317880767571,132.106249999482,-5.90808986649102));
#294947=CARTESIAN_POINT('Ctrl Pts',(6.21213331202012,132.256249999481,-8.55026797822134));
#294948=CARTESIAN_POINT('Ctrl Pts',(3.10606665601002,132.406249999481,-9.5594902125713));
#294949=CARTESIAN_POINT('Ctrl Pts',(-8.94643244596087E-14,132.55624999948,
-10.5687124469213));
#294950=CARTESIAN_POINT('Ctrl Pts',(-3.1060666560102,132.70624999948,-9.5594902125713));
#294951=CARTESIAN_POINT('Ctrl Pts',(-6.2121333120203,132.856249999479,-8.55026797822134));
#294952=CARTESIAN_POINT('Ctrl Pts',(-8.13178807675728,133.006249999478,
-5.90808986649102));
#294953=CARTESIAN_POINT('Ctrl Pts',(-10.0514428414943,133.156249999478,
-3.2659117547607));
#294954=CARTESIAN_POINT('Ctrl Pts',(-10.0514428414943,133.306249999477,
2.46189346052968E-15));
#294955=CARTESIAN_POINT('Ctrl Pts',(-10.0514428414943,133.456249999477,
3.26591175476071));
#294956=CARTESIAN_POINT('Ctrl Pts',(-8.13178807675728,133.606249999476,
5.90808986649102));
#294957=CARTESIAN_POINT('Ctrl Pts',(-6.2121333120203,133.756249999475,8.55026797822134));
#294958=CARTESIAN_POINT('Ctrl Pts',(-3.1060666560102,133.906249999475,9.5594902125713));
#294959=CARTESIAN_POINT('Ctrl Pts',(-8.77395911215934E-14,134.056249999474,
10.5687124469213));
#294960=CARTESIAN_POINT('Ctrl Pts',(3.10606665601002,134.206249999474,9.5594902125713));
#294961=CARTESIAN_POINT('Ctrl Pts',(6.21213331202013,134.356249999473,8.55026797822134));
#294962=CARTESIAN_POINT('Ctrl Pts',(8.1317880767571,134.506249999472,5.90808986649102));
#294963=CARTESIAN_POINT('Ctrl Pts',(10.0514428414941,134.656249999472,3.2659117547607));
#294964=CARTESIAN_POINT('Ctrl Pts',(10.0514428414941,134.806249999471,-1.23094673026484E-15));
#294965=CARTESIAN_POINT('Ctrl Pts',(10.0514428414941,134.956249999471,-3.26591175476071));
#294966=CARTESIAN_POINT('Ctrl Pts',(8.1317880767571,135.10624999947,-5.90808986649102));
#294967=CARTESIAN_POINT('Ctrl Pts',(6.21213331202012,135.256249999469,-8.55026797822134));
#294968=CARTESIAN_POINT('Ctrl Pts',(3.10606665601002,135.406249999469,-9.5594902125713));
#294969=CARTESIAN_POINT('Ctrl Pts',(-9.11920337312706E-14,135.556249999468,
-10.5687124469213));
#294970=CARTESIAN_POINT('Ctrl Pts',(-3.1060666560102,135.706249999468,-9.5594902125713));
#294971=CARTESIAN_POINT('Ctrl Pts',(-6.21213331202031,135.856249999467,
-8.55026797822134));
#294972=CARTESIAN_POINT('Ctrl Pts',(-8.13178807675728,136.006249999466,
-5.90808986649102));
#294973=CARTESIAN_POINT('Ctrl Pts',(-10.0514428414943,136.156249999466,
-3.2659117547607));
#294974=CARTESIAN_POINT('Ctrl Pts',(-10.0514428414943,136.306249999465,
2.46189346052968E-15));
#294975=CARTESIAN_POINT('Ctrl Pts',(-10.0514428414943,136.456249999465,
3.26591175476071));
#294976=CARTESIAN_POINT('Ctrl Pts',(-8.13178807675728,136.606249999464,
5.90808986649102));
#294977=CARTESIAN_POINT('Ctrl Pts',(-6.2121333120203,136.756249999463,8.55026797822134));
#294978=CARTESIAN_POINT('Ctrl Pts',(-3.1060666560102,136.906249999463,9.5594902125713));
#294979=CARTESIAN_POINT('Ctrl Pts',(-8.94673003932553E-14,137.056249999462,
10.5687124469213));
#294980=CARTESIAN_POINT('Ctrl Pts',(3.10606665601002,137.206249999462,9.5594902125713));
#294981=CARTESIAN_POINT('Ctrl Pts',(6.21213331202012,137.356249999461,8.55026797822134));
#294982=CARTESIAN_POINT('Ctrl Pts',(8.1317880767571,137.50624999946,5.90808986649102));
#294983=CARTESIAN_POINT('Ctrl Pts',(10.0514428414941,137.65624999946,3.2659117547607));
#294984=CARTESIAN_POINT('Ctrl Pts',(10.0514428414941,137.806249999459,-1.23094673026484E-15));
#294985=CARTESIAN_POINT('Ctrl Pts',(10.0514428414941,137.956249999459,-3.26591175476071));
#294986=CARTESIAN_POINT('Ctrl Pts',(8.1317880767571,138.106249999458,-5.90808986649102));
#294987=CARTESIAN_POINT('Ctrl Pts',(6.21213331202012,138.256249999457,-8.55026797822134));
#294988=CARTESIAN_POINT('Ctrl Pts',(3.10606665601001,138.406249999457,-9.5594902125713));
#294989=CARTESIAN_POINT('Ctrl Pts',(-9.29197430029324E-14,138.556249999456,
-10.5687124469213));
#294990=CARTESIAN_POINT('Ctrl Pts',(-3.1060666560102,138.706249999456,-9.5594902125713));
#294991=CARTESIAN_POINT('Ctrl Pts',(-6.21213331202031,138.856249999455,
-8.55026797822134));
#294992=CARTESIAN_POINT('Ctrl Pts',(-8.13178807675728,139.006249999454,
-5.90808986649102));
#294993=CARTESIAN_POINT('Ctrl Pts',(-10.0514428414943,139.156249999454,
-3.2659117547607));
#294994=CARTESIAN_POINT('Ctrl Pts',(-10.0514428414943,139.306249999453,
2.46189346052968E-15));
#294995=CARTESIAN_POINT('Ctrl Pts',(-10.0514428414943,139.456249999453,
3.26591175476071));
#294996=CARTESIAN_POINT('Ctrl Pts',(-8.13178807675728,139.606249999452,
5.90808986649102));
#294997=CARTESIAN_POINT('Ctrl Pts',(-6.21213331202031,139.756249999451,
8.55026797822134));
#294998=CARTESIAN_POINT('Ctrl Pts',(-3.1060666560102,139.906249999451,9.5594902125713));
#294999=CARTESIAN_POINT('Ctrl Pts',(-9.11950096649171E-14,140.05624999945,
10.5687124469213));
#295000=CARTESIAN_POINT('Ctrl Pts',(3.10606665601002,140.20624999945,9.5594902125713));
#295001=CARTESIAN_POINT('Ctrl Pts',(6.21213331202012,140.356249999449,8.55026797822134));
#295002=CARTESIAN_POINT('Ctrl Pts',(8.1317880767571,140.506249999448,5.90808986649102));
#295003=CARTESIAN_POINT('Ctrl Pts',(10.0514428414941,140.656249999448,3.2659117547607));
#295004=CARTESIAN_POINT('Ctrl Pts',(10.0514428414941,140.806249999447,-1.23094673026484E-15));
#295005=CARTESIAN_POINT('Ctrl Pts',(10.0514428414941,140.956249999447,-3.26591175476071));
#295006=CARTESIAN_POINT('Ctrl Pts',(8.1317880767571,141.106249999446,-5.90808986649102));
#295007=CARTESIAN_POINT('Ctrl Pts',(6.21213331202012,141.256249999445,-8.55026797822134));
#295008=CARTESIAN_POINT('Ctrl Pts',(3.10606665601001,141.406249999445,-9.5594902125713));
#295009=CARTESIAN_POINT('Ctrl Pts',(-9.46474522745942E-14,141.556249999444,
-10.5687124469213));
#295010=CARTESIAN_POINT('Ctrl Pts',(-3.1060666560102,141.706249999444,-9.5594902125713));
#295011=CARTESIAN_POINT('Ctrl Pts',(-6.21213331202031,141.856249999443,
-8.55026797822134));
#295012=CARTESIAN_POINT('Ctrl Pts',(-8.13178807675729,142.006249999442,
-5.90808986649102));
#295013=CARTESIAN_POINT('Ctrl Pts',(-10.0514428414943,142.156249999442,
-3.2659117547607));
#295014=CARTESIAN_POINT('Ctrl Pts',(-10.0514428414943,142.306249999441,
2.46189346052968E-15));
#295015=CARTESIAN_POINT('Ctrl Pts',(-10.0514428414943,142.456249999441,
3.26591175476071));
#295016=CARTESIAN_POINT('Ctrl Pts',(-8.13178807675729,142.60624999944,5.90808986649102));
#295017=CARTESIAN_POINT('Ctrl Pts',(-6.21213331202031,142.756249999439,
8.55026797822134));
#295018=CARTESIAN_POINT('Ctrl Pts',(-3.1060666560102,142.906249999439,9.5594902125713));
#295019=CARTESIAN_POINT('Ctrl Pts',(-9.29227189365789E-14,143.056249999438,
10.5687124469213));
#295020=CARTESIAN_POINT('Ctrl Pts',(3.10606665601001,143.206249999438,9.5594902125713));
#295021=CARTESIAN_POINT('Ctrl Pts',(6.21213331202012,143.356249999437,8.55026797822134));
#295022=CARTESIAN_POINT('Ctrl Pts',(8.1317880767571,143.506249999436,5.90808986649102));
#295023=CARTESIAN_POINT('Ctrl Pts',(10.0514428414941,143.656249999436,3.2659117547607));
#295024=CARTESIAN_POINT('Ctrl Pts',(10.0514428414941,143.806249999435,-1.23094673026484E-15));
#295025=CARTESIAN_POINT('Ctrl Pts',(10.0514428414941,143.956249999435,-3.26591175476071));
#295026=CARTESIAN_POINT('Ctrl Pts',(8.1317880767571,144.106249999434,-5.90808986649102));
#295027=CARTESIAN_POINT('Ctrl Pts',(6.21213331202012,144.256249999433,-8.55026797822134));
#295028=CARTESIAN_POINT('Ctrl Pts',(3.10606665601001,144.406249999433,-9.5594902125713));
#295029=CARTESIAN_POINT('Ctrl Pts',(-9.63751615462561E-14,144.556249999432,
-10.5687124469213));
#295030=CARTESIAN_POINT('Ctrl Pts',(-3.1060666560102,144.706249999432,-9.5594902125713));
#295031=CARTESIAN_POINT('Ctrl Pts',(-6.21213331202031,144.856249999431,
-8.55026797822134));
#295032=CARTESIAN_POINT('Ctrl Pts',(-8.13178807675729,145.00624999943,-5.90808986649102));
#295033=CARTESIAN_POINT('Ctrl Pts',(-10.0514428414943,145.15624999943,-3.2659117547607));
#295034=CARTESIAN_POINT('Ctrl Pts',(-10.0514428414943,145.306249999429,
2.46189346052968E-15));
#295035=CARTESIAN_POINT('Ctrl Pts',(-10.0514428414943,145.456249999429,
3.26591175476071));
#295036=CARTESIAN_POINT('Ctrl Pts',(-8.13178807675729,145.606249999428,
5.90808986649102));
#295037=CARTESIAN_POINT('Ctrl Pts',(-6.21213331202031,145.756249999427,
8.55026797822134));
#295038=CARTESIAN_POINT('Ctrl Pts',(-3.1060666560102,145.906249999427,9.5594902125713));
#295039=CARTESIAN_POINT('Ctrl Pts',(-9.46504282082408E-14,146.056249999426,
10.5687124469213));
#295040=CARTESIAN_POINT('Ctrl Pts',(3.10606665601001,146.206249999426,9.5594902125713));
#295041=CARTESIAN_POINT('Ctrl Pts',(6.21213331202012,146.356249999425,8.55026797822134));
#295042=CARTESIAN_POINT('Ctrl Pts',(8.13178807675709,146.506249999424,5.90808986649102));
#295043=CARTESIAN_POINT('Ctrl Pts',(10.0514428414941,146.656249999424,3.2659117547607));
#295044=CARTESIAN_POINT('Ctrl Pts',(10.0514428414941,146.806249999423,-1.23094673026484E-15));
#295045=CARTESIAN_POINT('Ctrl Pts',(10.0514428414941,146.956249999423,-3.26591175476071));
#295046=CARTESIAN_POINT('Ctrl Pts',(8.13178807675709,147.106249999422,-5.90808986649102));
#295047=CARTESIAN_POINT('Ctrl Pts',(6.21213331202012,147.256249999421,-8.55026797822134));
#295048=CARTESIAN_POINT('Ctrl Pts',(3.10606665601001,147.406249999421,-9.5594902125713));
#295049=CARTESIAN_POINT('Ctrl Pts',(-9.81028708179179E-14,147.55624999942,
-10.5687124469213));
#295050=CARTESIAN_POINT('Ctrl Pts',(-3.10606665601021,147.70624999942,-9.5594902125713));
#295051=CARTESIAN_POINT('Ctrl Pts',(-6.21213331202032,147.856249999419,
-8.55026797822134));
#295052=CARTESIAN_POINT('Ctrl Pts',(-8.13178807675729,148.006249999418,
-5.90808986649102));
#295053=CARTESIAN_POINT('Ctrl Pts',(-10.0514428414943,148.156249999418,
-3.2659117547607));
#295054=CARTESIAN_POINT('Ctrl Pts',(-10.0514428414943,148.306249999417,
2.46189346052968E-15));
#295055=CARTESIAN_POINT('Ctrl Pts',(-10.0514428414943,148.456249999417,
3.26591175476071));
#295056=CARTESIAN_POINT('Ctrl Pts',(-8.13178807675729,148.606249999416,
5.90808986649102));
#295057=CARTESIAN_POINT('Ctrl Pts',(-6.21213331202031,148.756249999415,
8.55026797822134));
#295058=CARTESIAN_POINT('Ctrl Pts',(-3.1060666560102,148.906249999415,9.5594902125713));
#295059=CARTESIAN_POINT('Ctrl Pts',(-9.63781374799026E-14,149.056249999414,
10.5687124469213));
#295060=CARTESIAN_POINT('Ctrl Pts',(3.10606665601001,149.206249999414,9.5594902125713));
#295061=CARTESIAN_POINT('Ctrl Pts',(6.21213331202012,149.356249999413,8.55026797822134));
#295062=CARTESIAN_POINT('Ctrl Pts',(8.13178807675709,149.506249999412,5.90808986649102));
#295063=CARTESIAN_POINT('Ctrl Pts',(10.0514428414941,149.656249999412,3.2659117547607));
#295064=CARTESIAN_POINT('Ctrl Pts',(10.0514428414941,149.806249999411,-1.23094673026484E-15));
#295065=CARTESIAN_POINT('Ctrl Pts',(10.0514428414941,149.956249999411,-3.26591175476071));
#295066=CARTESIAN_POINT('Ctrl Pts',(8.13178807675709,150.10624999941,-5.90808986649102));
#295067=CARTESIAN_POINT('Ctrl Pts',(6.21213331202012,150.256249999409,-8.55026797822134));
#295068=CARTESIAN_POINT('Ctrl Pts',(3.10606665601001,150.406249999409,-9.5594902125713));
#295069=CARTESIAN_POINT('Ctrl Pts',(-9.98305800895797E-14,150.556249999408,
-10.5687124469213));
#295070=CARTESIAN_POINT('Ctrl Pts',(-3.10606665601021,150.706249999408,
-9.5594902125713));
#295071=CARTESIAN_POINT('Ctrl Pts',(-6.21213331202032,150.856249999407,
-8.55026797822134));
#295072=CARTESIAN_POINT('Ctrl Pts',(-8.13178807675729,151.006249999406,
-5.90808986649102));
#295073=CARTESIAN_POINT('Ctrl Pts',(-10.0514428414943,151.156249999406,
-3.2659117547607));
#295074=CARTESIAN_POINT('Ctrl Pts',(-10.0514428414943,151.306249999405,
2.46189346052968E-15));
#295075=CARTESIAN_POINT('Ctrl Pts',(-10.0514428414943,151.456249999405,
3.26591175476071));
#295076=CARTESIAN_POINT('Ctrl Pts',(-8.13178807675729,151.606249999404,
5.90808986649102));
#295077=CARTESIAN_POINT('Ctrl Pts',(-6.21213331202032,151.756249999403,
8.55026797822134));
#295078=CARTESIAN_POINT('Ctrl Pts',(-3.10606665601021,151.906249999403,
9.5594902125713));
#295079=CARTESIAN_POINT('Ctrl Pts',(-9.81058467515645E-14,152.056249999402,
10.5687124469213));
#295080=CARTESIAN_POINT('Ctrl Pts',(3.10606665601001,152.206249999402,9.5594902125713));
#295081=CARTESIAN_POINT('Ctrl Pts',(6.21213331202012,152.356249999401,8.55026797822134));
#295082=CARTESIAN_POINT('Ctrl Pts',(8.13178807675709,152.5062499994,5.90808986649102));
#295083=CARTESIAN_POINT('Ctrl Pts',(10.0514428414941,152.6562499994,3.2659117547607));
#295084=CARTESIAN_POINT('Ctrl Pts',(10.0514428414941,152.806249999399,-1.23094673026484E-15));
#295085=CARTESIAN_POINT('Ctrl Pts',(10.0514428414941,152.956249999399,-3.26591175476071));
#295086=CARTESIAN_POINT('Ctrl Pts',(8.13178807675709,153.106249999398,-5.90808986649102));
#295087=CARTESIAN_POINT('Ctrl Pts',(6.21213331202012,153.256249999397,-8.55026797822134));
#295088=CARTESIAN_POINT('Ctrl Pts',(3.10606665601001,153.406249999397,-9.5594902125713));
#295089=CARTESIAN_POINT('Ctrl Pts',(-1.01558289361242E-13,153.556249999396,
-10.5687124469213));
#295090=CARTESIAN_POINT('Ctrl Pts',(-3.10606665601021,153.706249999396,
-9.5594902125713));
#295091=CARTESIAN_POINT('Ctrl Pts',(-12.1623797632097,-0.474999999988005,
2.97892388940585E-15));
#295092=CARTESIAN_POINT('Ctrl Pts',(-12.1623797632096,-0.324999999988605,
3.95179673813133));
#295093=CARTESIAN_POINT('Ctrl Pts',(-9.83957192047856,-0.174999999989203,
7.14886745759505));
#295094=CARTESIAN_POINT('Ctrl Pts',(-7.51676407774747,-0.0249999999898023,
10.3459381770588));
#295095=CARTESIAN_POINT('Ctrl Pts',(-3.75838203887374,0.1250000000096,11.5671105274568));
#295096=CARTESIAN_POINT('Ctrl Pts',(-1.02868273148643E-14,0.275000000009002,
12.7882828778549));
#295097=CARTESIAN_POINT('Ctrl Pts',(3.75838203887372,0.425000000008404,
11.5671105274568));
#295098=CARTESIAN_POINT('Ctrl Pts',(7.51676407774745,0.575000000007806,
10.3459381770588));
#295099=CARTESIAN_POINT('Ctrl Pts',(9.83957192047854,0.725000000007208,
7.14886745759505));
#295100=CARTESIAN_POINT('Ctrl Pts',(12.1623797632096,0.875000000006609,
3.95179673813132));
#295101=CARTESIAN_POINT('Ctrl Pts',(12.1623797632096,1.02500000000601,-1.48946194470292E-15));
#295102=CARTESIAN_POINT('Ctrl Pts',(12.1623797632096,1.17500000000541,-3.95179673813132));
#295103=CARTESIAN_POINT('Ctrl Pts',(9.83957192047853,1.32500000000481,-7.14886745759505));
#295104=CARTESIAN_POINT('Ctrl Pts',(7.51676407774744,1.47500000000421,-10.3459381770588));
#295105=CARTESIAN_POINT('Ctrl Pts',(3.75838203887371,1.6250000000036,-11.5671105274568));
#295106=CARTESIAN_POINT('Ctrl Pts',(-1.42829078892864E-14,1.775000000003,
-12.7882828778549));
#295107=CARTESIAN_POINT('Ctrl Pts',(-3.75838203887374,1.9250000000024,-11.5671105274568));
#295108=CARTESIAN_POINT('Ctrl Pts',(-7.51676407774747,2.0750000000018,-10.3459381770588));
#295109=CARTESIAN_POINT('Ctrl Pts',(-9.83957192047856,2.2250000000012,-7.14886745759505));
#295110=CARTESIAN_POINT('Ctrl Pts',(-12.1623797632097,2.37500000000059,
-3.95179673813132));
#295111=CARTESIAN_POINT('Ctrl Pts',(-12.1623797632097,2.525,2.97892388940585E-15));
#295112=CARTESIAN_POINT('Ctrl Pts',(-12.1623797632097,2.6749999999994,3.95179673813133));
#295113=CARTESIAN_POINT('Ctrl Pts',(-9.83957192047856,2.8249999999988,7.14886745759505));
#295114=CARTESIAN_POINT('Ctrl Pts',(-7.51676407774747,2.9749999999982,10.3459381770588));
#295115=CARTESIAN_POINT('Ctrl Pts',(-3.75838203887374,3.1249999999976,11.5671105274568));
#295116=CARTESIAN_POINT('Ctrl Pts',(-1.20145365865262E-14,3.274999999997,
12.7882828778549));
#295117=CARTESIAN_POINT('Ctrl Pts',(3.75838203887372,3.4249999999964,11.5671105274568));
#295118=CARTESIAN_POINT('Ctrl Pts',(7.51676407774744,3.57499999999581,10.3459381770588));
#295119=CARTESIAN_POINT('Ctrl Pts',(9.83957192047853,3.72499999999521,7.14886745759505));
#295120=CARTESIAN_POINT('Ctrl Pts',(12.1623797632096,3.87499999999461,3.95179673813132));
#295121=CARTESIAN_POINT('Ctrl Pts',(12.1623797632096,4.02499999999401,-1.48946194470292E-15));
#295122=CARTESIAN_POINT('Ctrl Pts',(12.1623797632096,4.17499999999341,-3.95179673813132));
#295123=CARTESIAN_POINT('Ctrl Pts',(9.83957192047853,4.32499999999281,-7.14886745759505));
#295124=CARTESIAN_POINT('Ctrl Pts',(7.51676407774744,4.47499999999221,-10.3459381770588));
#295125=CARTESIAN_POINT('Ctrl Pts',(3.75838203887371,4.6249999999916,-11.5671105274568));
#295126=CARTESIAN_POINT('Ctrl Pts',(-1.60106171609483E-14,4.774999999991,
-12.7882828778549));
#295127=CARTESIAN_POINT('Ctrl Pts',(-3.75838203887374,4.9249999999904,-11.5671105274568));
#295128=CARTESIAN_POINT('Ctrl Pts',(-7.51676407774747,5.0749999999898,-10.3459381770588));
#295129=CARTESIAN_POINT('Ctrl Pts',(-9.83957192047857,5.2249999999892,-7.14886745759505));
#295130=CARTESIAN_POINT('Ctrl Pts',(-12.1623797632097,5.3749999999886,-3.95179673813132));
#295131=CARTESIAN_POINT('Ctrl Pts',(-12.1623797632097,5.52499999998799,
2.97892388940585E-15));
#295132=CARTESIAN_POINT('Ctrl Pts',(-12.1623797632097,5.6749999999874,3.95179673813133));
#295133=CARTESIAN_POINT('Ctrl Pts',(-9.83957192047857,5.8249999999868,7.14886745759505));
#295134=CARTESIAN_POINT('Ctrl Pts',(-7.51676407774747,5.9749999999862,10.3459381770588));
#295135=CARTESIAN_POINT('Ctrl Pts',(-3.75838203887374,6.1249999999856,11.5671105274568));
#295136=CARTESIAN_POINT('Ctrl Pts',(-1.3742245858188E-14,6.274999999985,
12.7882828778549));
#295137=CARTESIAN_POINT('Ctrl Pts',(3.75838203887371,6.4249999999844,11.5671105274568));
#295138=CARTESIAN_POINT('Ctrl Pts',(7.51676407774744,6.57499999998381,10.3459381770588));
#295139=CARTESIAN_POINT('Ctrl Pts',(9.83957192047853,6.72499999998321,7.14886745759505));
#295140=CARTESIAN_POINT('Ctrl Pts',(12.1623797632096,6.87499999998261,3.95179673813132));
#295141=CARTESIAN_POINT('Ctrl Pts',(12.1623797632096,7.02499999998201,-1.48946194470292E-15));
#295142=CARTESIAN_POINT('Ctrl Pts',(12.1623797632096,7.17499999998141,-3.95179673813132));
#295143=CARTESIAN_POINT('Ctrl Pts',(9.83957192047853,7.32499999998081,-7.14886745759505));
#295144=CARTESIAN_POINT('Ctrl Pts',(7.51676407774744,7.47499999998021,-10.3459381770588));
#295145=CARTESIAN_POINT('Ctrl Pts',(3.75838203887371,7.6249999999796,-11.5671105274568));
#295146=CARTESIAN_POINT('Ctrl Pts',(-1.77383264326101E-14,7.774999999979,
-12.7882828778549));
#295147=CARTESIAN_POINT('Ctrl Pts',(-3.75838203887375,7.9249999999784,-11.5671105274568));
#295148=CARTESIAN_POINT('Ctrl Pts',(-7.51676407774747,8.0749999999778,-10.3459381770588));
#295149=CARTESIAN_POINT('Ctrl Pts',(-9.83957192047857,8.2249999999772,-7.14886745759505));
#295150=CARTESIAN_POINT('Ctrl Pts',(-12.1623797632097,8.3749999999766,-3.95179673813132));
#295151=CARTESIAN_POINT('Ctrl Pts',(-12.1623797632097,8.52499999997599,
2.97892388940585E-15));
#295152=CARTESIAN_POINT('Ctrl Pts',(-12.1623797632097,8.6749999999754,3.95179673813133));
#295153=CARTESIAN_POINT('Ctrl Pts',(-9.83957192047857,8.8249999999748,7.14886745759505));
#295154=CARTESIAN_POINT('Ctrl Pts',(-7.51676407774747,8.9749999999742,10.3459381770588));
#295155=CARTESIAN_POINT('Ctrl Pts',(-3.75838203887374,9.1249999999736,11.5671105274568));
#295156=CARTESIAN_POINT('Ctrl Pts',(-1.54699551298498E-14,9.274999999973,
12.7882828778549));
#295157=CARTESIAN_POINT('Ctrl Pts',(3.75838203887371,9.4249999999724,11.5671105274568));
#295158=CARTESIAN_POINT('Ctrl Pts',(7.51676407774744,9.57499999997181,10.3459381770588));
#295159=CARTESIAN_POINT('Ctrl Pts',(9.83957192047853,9.72499999997121,7.14886745759505));
#295160=CARTESIAN_POINT('Ctrl Pts',(12.1623797632096,9.87499999997061,3.95179673813132));
#295161=CARTESIAN_POINT('Ctrl Pts',(12.1623797632096,10.02499999997,-1.48946194470292E-15));
#295162=CARTESIAN_POINT('Ctrl Pts',(12.1623797632096,10.1749999999694,-3.95179673813132));
#295163=CARTESIAN_POINT('Ctrl Pts',(9.83957192047853,10.3249999999688,-7.14886745759505));
#295164=CARTESIAN_POINT('Ctrl Pts',(7.51676407774744,10.4749999999682,-10.3459381770588));
#295165=CARTESIAN_POINT('Ctrl Pts',(3.75838203887371,10.6249999999676,-11.5671105274568));
#295166=CARTESIAN_POINT('Ctrl Pts',(-1.9466035704272E-14,10.774999999967,
-12.7882828778549));
#295167=CARTESIAN_POINT('Ctrl Pts',(-3.75838203887375,10.9249999999664,
-11.5671105274568));
#295168=CARTESIAN_POINT('Ctrl Pts',(-7.51676407774748,11.0749999999658,
-10.3459381770588));
#295169=CARTESIAN_POINT('Ctrl Pts',(-9.83957192047857,11.2249999999652,
-7.14886745759505));
#295170=CARTESIAN_POINT('Ctrl Pts',(-12.1623797632097,11.3749999999646,
-3.95179673813132));
#295171=CARTESIAN_POINT('Ctrl Pts',(-12.1623797632097,11.524999999964,2.97892388940585E-15));
#295172=CARTESIAN_POINT('Ctrl Pts',(-12.1623797632097,11.6749999999634,
3.95179673813133));
#295173=CARTESIAN_POINT('Ctrl Pts',(-9.83957192047857,11.8249999999628,
7.14886745759505));
#295174=CARTESIAN_POINT('Ctrl Pts',(-7.51676407774747,11.9749999999622,
10.3459381770588));
#295175=CARTESIAN_POINT('Ctrl Pts',(-3.75838203887375,12.1249999999616,
11.5671105274568));
#295176=CARTESIAN_POINT('Ctrl Pts',(-1.71976644015117E-14,12.274999999961,
12.7882828778549));
#295177=CARTESIAN_POINT('Ctrl Pts',(3.75838203887371,12.4249999999604,11.5671105274568));
#295178=CARTESIAN_POINT('Ctrl Pts',(7.51676407774744,12.5749999999598,10.3459381770588));
#295179=CARTESIAN_POINT('Ctrl Pts',(9.83957192047853,12.7249999999592,7.14886745759505));
#295180=CARTESIAN_POINT('Ctrl Pts',(12.1623797632096,12.8749999999586,3.95179673813132));
#295181=CARTESIAN_POINT('Ctrl Pts',(12.1623797632096,13.024999999958,-1.48946194470292E-15));
#295182=CARTESIAN_POINT('Ctrl Pts',(12.1623797632096,13.1749999999574,-3.95179673813132));
#295183=CARTESIAN_POINT('Ctrl Pts',(9.83957192047853,13.3249999999568,-7.14886745759505));
#295184=CARTESIAN_POINT('Ctrl Pts',(7.51676407774743,13.4749999999562,-10.3459381770588));
#295185=CARTESIAN_POINT('Ctrl Pts',(3.75838203887371,13.6249999999556,-11.5671105274568));
#295186=CARTESIAN_POINT('Ctrl Pts',(-2.11937449759338E-14,13.774999999955,
-12.7882828778549));
#295187=CARTESIAN_POINT('Ctrl Pts',(-3.75838203887375,13.9249999999544,
-11.5671105274568));
#295188=CARTESIAN_POINT('Ctrl Pts',(-7.51676407774748,14.0749999999538,
-10.3459381770588));
#295189=CARTESIAN_POINT('Ctrl Pts',(-9.83957192047857,14.2249999999532,
-7.14886745759505));
#295190=CARTESIAN_POINT('Ctrl Pts',(-12.1623797632097,14.3749999999526,
-3.95179673813132));
#295191=CARTESIAN_POINT('Ctrl Pts',(-12.1623797632097,14.524999999952,2.97892388940585E-15));
#295192=CARTESIAN_POINT('Ctrl Pts',(-12.1623797632097,14.6749999999514,
3.95179673813133));
#295193=CARTESIAN_POINT('Ctrl Pts',(-9.83957192047857,14.8249999999508,
7.14886745759505));
#295194=CARTESIAN_POINT('Ctrl Pts',(-7.51676407774747,14.9749999999502,
10.3459381770588));
#295195=CARTESIAN_POINT('Ctrl Pts',(-3.75838203887375,15.1249999999496,
11.5671105274568));
#295196=CARTESIAN_POINT('Ctrl Pts',(-1.89253736731735E-14,15.274999999949,
12.7882828778549));
#295197=CARTESIAN_POINT('Ctrl Pts',(3.75838203887371,15.4249999999484,11.5671105274568));
#295198=CARTESIAN_POINT('Ctrl Pts',(7.51676407774744,15.5749999999478,10.3459381770588));
#295199=CARTESIAN_POINT('Ctrl Pts',(9.83957192047853,15.7249999999472,7.14886745759505));
#295200=CARTESIAN_POINT('Ctrl Pts',(12.1623797632096,15.8749999999466,3.95179673813132));
#295201=CARTESIAN_POINT('Ctrl Pts',(12.1623797632096,16.024999999946,-1.48946194470292E-15));
#295202=CARTESIAN_POINT('Ctrl Pts',(12.1623797632096,16.1749999999454,-3.95179673813132));
#295203=CARTESIAN_POINT('Ctrl Pts',(9.83957192047852,16.3249999999448,-7.14886745759505));
#295204=CARTESIAN_POINT('Ctrl Pts',(7.51676407774743,16.4749999999442,-10.3459381770588));
#295205=CARTESIAN_POINT('Ctrl Pts',(3.7583820388737,16.6249999999436,-11.5671105274568));
#295206=CARTESIAN_POINT('Ctrl Pts',(-2.29214542475956E-14,16.774999999943,
-12.7882828778549));
#295207=CARTESIAN_POINT('Ctrl Pts',(-3.75838203887375,16.9249999999424,
-11.5671105274568));
#295208=CARTESIAN_POINT('Ctrl Pts',(-7.51676407774748,17.0749999999418,
-10.3459381770588));
#295209=CARTESIAN_POINT('Ctrl Pts',(-9.83957192047857,17.2249999999412,
-7.14886745759505));
#295210=CARTESIAN_POINT('Ctrl Pts',(-12.1623797632097,17.3749999999406,
-3.95179673813132));
#295211=CARTESIAN_POINT('Ctrl Pts',(-12.1623797632097,17.52499999994,2.97892388940585E-15));
#295212=CARTESIAN_POINT('Ctrl Pts',(-12.1623797632097,17.6749999999394,
3.95179673813133));
#295213=CARTESIAN_POINT('Ctrl Pts',(-9.83957192047857,17.8249999999388,
7.14886745759505));
#295214=CARTESIAN_POINT('Ctrl Pts',(-7.51676407774748,17.9749999999382,
10.3459381770588));
#295215=CARTESIAN_POINT('Ctrl Pts',(-3.75838203887375,18.1249999999376,
11.5671105274568));
#295216=CARTESIAN_POINT('Ctrl Pts',(-2.06530829448354E-14,18.274999999937,
12.7882828778549));
#295217=CARTESIAN_POINT('Ctrl Pts',(3.75838203887371,18.4249999999364,11.5671105274568));
#295218=CARTESIAN_POINT('Ctrl Pts',(7.51676407774743,18.5749999999358,10.3459381770588));
#295219=CARTESIAN_POINT('Ctrl Pts',(9.83957192047852,18.7249999999352,7.14886745759505));
#295220=CARTESIAN_POINT('Ctrl Pts',(12.1623797632096,18.8749999999346,3.95179673813132));
#295221=CARTESIAN_POINT('Ctrl Pts',(12.1623797632096,19.024999999934,-1.48946194470292E-15));
#295222=CARTESIAN_POINT('Ctrl Pts',(12.1623797632096,19.1749999999334,-3.95179673813132));
#295223=CARTESIAN_POINT('Ctrl Pts',(9.83957192047852,19.3249999999328,-7.14886745759505));
#295224=CARTESIAN_POINT('Ctrl Pts',(7.51676407774743,19.4749999999322,-10.3459381770588));
#295225=CARTESIAN_POINT('Ctrl Pts',(3.7583820388737,19.6249999999316,-11.5671105274568));
#295226=CARTESIAN_POINT('Ctrl Pts',(-2.46491635192575E-14,19.774999999931,
-12.7882828778549));
#295227=CARTESIAN_POINT('Ctrl Pts',(-3.75838203887375,19.9249999999304,
-11.5671105274568));
#295228=CARTESIAN_POINT('Ctrl Pts',(-7.51676407774748,20.0749999999298,
-10.3459381770588));
#295229=CARTESIAN_POINT('Ctrl Pts',(-9.83957192047857,20.2249999999292,
-7.14886745759505));
#295230=CARTESIAN_POINT('Ctrl Pts',(-12.1623797632097,20.3749999999286,
-3.95179673813132));
#295231=CARTESIAN_POINT('Ctrl Pts',(-12.1623797632097,20.524999999928,2.97892388940585E-15));
#295232=CARTESIAN_POINT('Ctrl Pts',(-12.1623797632097,20.6749999999274,
3.95179673813133));
#295233=CARTESIAN_POINT('Ctrl Pts',(-9.83957192047857,20.8249999999268,
7.14886745759505));
#295234=CARTESIAN_POINT('Ctrl Pts',(-7.51676407774748,20.9749999999262,
10.3459381770588));
#295235=CARTESIAN_POINT('Ctrl Pts',(-3.75838203887375,21.1249999999256,
11.5671105274568));
#295236=CARTESIAN_POINT('Ctrl Pts',(-2.23807922164972E-14,21.274999999925,
12.7882828778549));
#295237=CARTESIAN_POINT('Ctrl Pts',(3.7583820388737,21.4249999999244,11.5671105274568));
#295238=CARTESIAN_POINT('Ctrl Pts',(7.51676407774743,21.5749999999238,10.3459381770588));
#295239=CARTESIAN_POINT('Ctrl Pts',(9.83957192047852,21.7249999999232,7.14886745759505));
#295240=CARTESIAN_POINT('Ctrl Pts',(12.1623797632096,21.8749999999226,3.95179673813132));
#295241=CARTESIAN_POINT('Ctrl Pts',(12.1623797632096,22.024999999922,-1.48946194470292E-15));
#295242=CARTESIAN_POINT('Ctrl Pts',(12.1623797632096,22.1749999999214,-3.95179673813132));
#295243=CARTESIAN_POINT('Ctrl Pts',(9.83957192047852,22.3249999999208,-7.14886745759505));
#295244=CARTESIAN_POINT('Ctrl Pts',(7.51676407774743,22.4749999999202,-10.3459381770588));
#295245=CARTESIAN_POINT('Ctrl Pts',(3.7583820388737,22.6249999999196,-11.5671105274568));
#295246=CARTESIAN_POINT('Ctrl Pts',(-2.63768727909193E-14,22.774999999919,
-12.7882828778549));
#295247=CARTESIAN_POINT('Ctrl Pts',(-3.75838203887375,22.9249999999184,
-11.5671105274568));
#295248=CARTESIAN_POINT('Ctrl Pts',(-7.51676407774748,23.0749999999178,
-10.3459381770588));
#295249=CARTESIAN_POINT('Ctrl Pts',(-9.83957192047857,23.2249999999172,
-7.14886745759505));
#295250=CARTESIAN_POINT('Ctrl Pts',(-12.1623797632097,23.3749999999166,
-3.95179673813132));
#295251=CARTESIAN_POINT('Ctrl Pts',(-12.1623797632097,23.524999999916,2.97892388940585E-15));
#295252=CARTESIAN_POINT('Ctrl Pts',(-12.1623797632097,23.6749999999154,
3.95179673813133));
#295253=CARTESIAN_POINT('Ctrl Pts',(-9.83957192047857,23.8249999999148,
7.14886745759505));
#295254=CARTESIAN_POINT('Ctrl Pts',(-7.51676407774748,23.9749999999142,
10.3459381770588));
#295255=CARTESIAN_POINT('Ctrl Pts',(-3.75838203887375,24.1249999999136,
11.5671105274568));
#295256=CARTESIAN_POINT('Ctrl Pts',(-2.4108501488159E-14,24.274999999913,
12.7882828778549));
#295257=CARTESIAN_POINT('Ctrl Pts',(3.7583820388737,24.4249999999124,11.5671105274568));
#295258=CARTESIAN_POINT('Ctrl Pts',(7.51676407774743,24.5749999999118,10.3459381770588));
#295259=CARTESIAN_POINT('Ctrl Pts',(9.83957192047852,24.7249999999112,7.14886745759505));
#295260=CARTESIAN_POINT('Ctrl Pts',(12.1623797632096,24.8749999999106,3.95179673813132));
#295261=CARTESIAN_POINT('Ctrl Pts',(12.1623797632096,25.02499999991,-1.48946194470292E-15));
#295262=CARTESIAN_POINT('Ctrl Pts',(12.1623797632096,25.1749999999094,-3.95179673813132));
#295263=CARTESIAN_POINT('Ctrl Pts',(9.83957192047852,25.3249999999088,-7.14886745759505));
#295264=CARTESIAN_POINT('Ctrl Pts',(7.51676407774743,25.4749999999082,-10.3459381770588));
#295265=CARTESIAN_POINT('Ctrl Pts',(3.7583820388737,25.6249999999076,-11.5671105274568));
#295266=CARTESIAN_POINT('Ctrl Pts',(-2.81045820625811E-14,25.774999999907,
-12.7882828778549));
#295267=CARTESIAN_POINT('Ctrl Pts',(-3.75838203887376,25.9249999999064,
-11.5671105274568));
#295268=CARTESIAN_POINT('Ctrl Pts',(-7.51676407774749,26.0749999999058,
-10.3459381770588));
#295269=CARTESIAN_POINT('Ctrl Pts',(-9.83957192047857,26.2249999999052,
-7.14886745759505));
#295270=CARTESIAN_POINT('Ctrl Pts',(-12.1623797632097,26.3749999999046,
-3.95179673813132));
#295271=CARTESIAN_POINT('Ctrl Pts',(-12.1623797632097,26.524999999904,2.97892388940585E-15));
#295272=CARTESIAN_POINT('Ctrl Pts',(-12.1623797632097,26.6749999999034,
3.95179673813133));
#295273=CARTESIAN_POINT('Ctrl Pts',(-9.83957192047857,26.8249999999028,
7.14886745759505));
#295274=CARTESIAN_POINT('Ctrl Pts',(-7.51676407774748,26.9749999999022,
10.3459381770588));
#295275=CARTESIAN_POINT('Ctrl Pts',(-3.75838203887375,27.1249999999016,
11.5671105274568));
#295276=CARTESIAN_POINT('Ctrl Pts',(-2.58362107598209E-14,27.274999999901,
12.7882828778549));
#295277=CARTESIAN_POINT('Ctrl Pts',(3.7583820388737,27.4249999999004,11.5671105274568));
#295278=CARTESIAN_POINT('Ctrl Pts',(7.51676407774743,27.5749999998998,10.3459381770588));
#295279=CARTESIAN_POINT('Ctrl Pts',(9.83957192047852,27.7249999998992,7.14886745759505));
#295280=CARTESIAN_POINT('Ctrl Pts',(12.1623797632096,27.8749999998986,3.95179673813132));
#295281=CARTESIAN_POINT('Ctrl Pts',(12.1623797632096,28.024999999898,-1.48946194470292E-15));
#295282=CARTESIAN_POINT('Ctrl Pts',(12.1623797632096,28.1749999998974,-3.95179673813132));
#295283=CARTESIAN_POINT('Ctrl Pts',(9.83957192047852,28.3249999998968,-7.14886745759505));
#295284=CARTESIAN_POINT('Ctrl Pts',(7.51676407774743,28.4749999998962,-10.3459381770588));
#295285=CARTESIAN_POINT('Ctrl Pts',(3.7583820388737,28.6249999998956,-11.5671105274568));
#295286=CARTESIAN_POINT('Ctrl Pts',(-2.9832291334243E-14,28.774999999895,
-12.7882828778549));
#295287=CARTESIAN_POINT('Ctrl Pts',(-3.75838203887376,28.9249999998944,
-11.5671105274568));
#295288=CARTESIAN_POINT('Ctrl Pts',(-7.51676407774749,29.0749999998938,
-10.3459381770588));
#295289=CARTESIAN_POINT('Ctrl Pts',(-9.83957192047858,29.2249999998932,
-7.14886745759505));
#295290=CARTESIAN_POINT('Ctrl Pts',(-12.1623797632097,29.3749999998926,
-3.95179673813132));
#295291=CARTESIAN_POINT('Ctrl Pts',(-12.1623797632097,29.524999999892,2.97892388940585E-15));
#295292=CARTESIAN_POINT('Ctrl Pts',(-12.1623797632097,29.6749999998914,
3.95179673813133));
#295293=CARTESIAN_POINT('Ctrl Pts',(-9.83957192047858,29.8249999998908,
7.14886745759505));
#295294=CARTESIAN_POINT('Ctrl Pts',(-7.51676407774748,29.9749999998902,
10.3459381770588));
#295295=CARTESIAN_POINT('Ctrl Pts',(-3.75838203887376,30.1249999998896,
11.5671105274568));
#295296=CARTESIAN_POINT('Ctrl Pts',(-2.75639200314827E-14,30.274999999889,
12.7882828778549));
#295297=CARTESIAN_POINT('Ctrl Pts',(3.7583820388737,30.4249999998884,11.5671105274568));
#295298=CARTESIAN_POINT('Ctrl Pts',(7.51676407774743,30.5749999998878,10.3459381770588));
#295299=CARTESIAN_POINT('Ctrl Pts',(9.83957192047852,30.7249999998872,7.14886745759505));
#295300=CARTESIAN_POINT('Ctrl Pts',(12.1623797632096,30.8749999998866,3.95179673813132));
#295301=CARTESIAN_POINT('Ctrl Pts',(12.1623797632096,31.024999999886,-1.48946194470292E-15));
#295302=CARTESIAN_POINT('Ctrl Pts',(12.1623797632096,31.1749999998854,-3.95179673813132));
#295303=CARTESIAN_POINT('Ctrl Pts',(9.83957192047852,31.3249999998848,-7.14886745759505));
#295304=CARTESIAN_POINT('Ctrl Pts',(7.51676407774742,31.4749999998842,-10.3459381770588));
#295305=CARTESIAN_POINT('Ctrl Pts',(3.7583820388737,31.6249999998836,-11.5671105274568));
#295306=CARTESIAN_POINT('Ctrl Pts',(-3.15600006059048E-14,31.774999999883,
-12.7882828778549));
#295307=CARTESIAN_POINT('Ctrl Pts',(-3.75838203887376,31.9249999998824,
-11.5671105274568));
#295308=CARTESIAN_POINT('Ctrl Pts',(-7.51676407774749,32.0749999998818,
-10.3459381770588));
#295309=CARTESIAN_POINT('Ctrl Pts',(-9.83957192047858,32.2249999998812,
-7.14886745759505));
#295310=CARTESIAN_POINT('Ctrl Pts',(-12.1623797632097,32.3749999998806,
-3.95179673813132));
#295311=CARTESIAN_POINT('Ctrl Pts',(-12.1623797632097,32.52499999988,2.97892388940585E-15));
#295312=CARTESIAN_POINT('Ctrl Pts',(-12.1623797632097,32.6749999998794,
3.95179673813133));
#295313=CARTESIAN_POINT('Ctrl Pts',(-9.83957192047858,32.8249999998788,
7.14886745759505));
#295314=CARTESIAN_POINT('Ctrl Pts',(-7.51676407774749,32.9749999998782,
10.3459381770588));
#295315=CARTESIAN_POINT('Ctrl Pts',(-3.75838203887376,33.1249999998776,
11.5671105274568));
#295316=CARTESIAN_POINT('Ctrl Pts',(-2.92916293031446E-14,33.274999999877,
12.7882828778549));
#295317=CARTESIAN_POINT('Ctrl Pts',(3.7583820388737,33.4249999998764,11.5671105274568));
#295318=CARTESIAN_POINT('Ctrl Pts',(7.51676407774743,33.5749999998758,10.3459381770588));
#295319=CARTESIAN_POINT('Ctrl Pts',(9.83957192047852,33.7249999998752,7.14886745759505));
#295320=CARTESIAN_POINT('Ctrl Pts',(12.1623797632096,33.8749999998746,3.95179673813132));
#295321=CARTESIAN_POINT('Ctrl Pts',(12.1623797632096,34.024999999874,-1.48946194470292E-15));
#295322=CARTESIAN_POINT('Ctrl Pts',(12.1623797632096,34.1749999998734,-3.95179673813132));
#295323=CARTESIAN_POINT('Ctrl Pts',(9.83957192047851,34.3249999998728,-7.14886745759505));
#295324=CARTESIAN_POINT('Ctrl Pts',(7.51676407774742,34.4749999998722,-10.3459381770588));
#295325=CARTESIAN_POINT('Ctrl Pts',(3.7583820388737,34.6249999998716,-11.5671105274568));
#295326=CARTESIAN_POINT('Ctrl Pts',(-3.32877098775667E-14,34.774999999871,
-12.7882828778549));
#295327=CARTESIAN_POINT('Ctrl Pts',(-3.75838203887376,34.9249999998704,
-11.5671105274568));
#295328=CARTESIAN_POINT('Ctrl Pts',(-7.51676407774749,35.0749999998698,
-10.3459381770588));
#295329=CARTESIAN_POINT('Ctrl Pts',(-9.83957192047858,35.2249999998692,
-7.14886745759505));
#295330=CARTESIAN_POINT('Ctrl Pts',(-12.1623797632097,35.3749999998686,
-3.95179673813132));
#295331=CARTESIAN_POINT('Ctrl Pts',(-12.1623797632097,35.524999999868,2.97892388940585E-15));
#295332=CARTESIAN_POINT('Ctrl Pts',(-12.1623797632097,35.6749999998674,
3.95179673813133));
#295333=CARTESIAN_POINT('Ctrl Pts',(-9.83957192047858,35.8249999998668,
7.14886745759505));
#295334=CARTESIAN_POINT('Ctrl Pts',(-7.51676407774749,35.9749999998662,
10.3459381770588));
#295335=CARTESIAN_POINT('Ctrl Pts',(-3.75838203887376,36.1249999998656,
11.5671105274568));
#295336=CARTESIAN_POINT('Ctrl Pts',(-3.10193385748064E-14,36.274999999865,
12.7882828778549));
#295337=CARTESIAN_POINT('Ctrl Pts',(3.7583820388737,36.4249999998644,11.5671105274568));
#295338=CARTESIAN_POINT('Ctrl Pts',(7.51676407774742,36.5749999998638,10.3459381770588));
#295339=CARTESIAN_POINT('Ctrl Pts',(9.83957192047851,36.7249999998632,7.14886745759505));
#295340=CARTESIAN_POINT('Ctrl Pts',(12.1623797632096,36.8749999998626,3.95179673813132));
#295341=CARTESIAN_POINT('Ctrl Pts',(12.1623797632096,37.024999999862,-1.48946194470292E-15));
#295342=CARTESIAN_POINT('Ctrl Pts',(12.1623797632096,37.1749999998614,-3.95179673813132));
#295343=CARTESIAN_POINT('Ctrl Pts',(9.83957192047851,37.3249999998608,-7.14886745759505));
#295344=CARTESIAN_POINT('Ctrl Pts',(7.51676407774742,37.4749999998602,-10.3459381770588));
#295345=CARTESIAN_POINT('Ctrl Pts',(3.75838203887369,37.6249999998596,-11.5671105274568));
#295346=CARTESIAN_POINT('Ctrl Pts',(-3.50154191492285E-14,37.774999999859,
-12.7882828778549));
#295347=CARTESIAN_POINT('Ctrl Pts',(-3.75838203887376,37.9249999998584,
-11.5671105274568));
#295348=CARTESIAN_POINT('Ctrl Pts',(-7.51676407774749,38.0749999998578,
-10.3459381770588));
#295349=CARTESIAN_POINT('Ctrl Pts',(-9.83957192047858,38.2249999998572,
-7.14886745759505));
#295350=CARTESIAN_POINT('Ctrl Pts',(-12.1623797632097,38.3749999998566,
-3.95179673813132));
#295351=CARTESIAN_POINT('Ctrl Pts',(-12.1623797632097,38.524999999856,2.97892388940585E-15));
#295352=CARTESIAN_POINT('Ctrl Pts',(-12.1623797632097,38.6749999998554,
3.95179673813133));
#295353=CARTESIAN_POINT('Ctrl Pts',(-9.83957192047858,38.8249999998548,
7.14886745759505));
#295354=CARTESIAN_POINT('Ctrl Pts',(-7.51676407774749,38.9749999998542,
10.3459381770588));
#295355=CARTESIAN_POINT('Ctrl Pts',(-3.75838203887376,39.1249999998536,
11.5671105274568));
#295356=CARTESIAN_POINT('Ctrl Pts',(-3.27470478464682E-14,39.274999999853,
12.7882828778549));
#295357=CARTESIAN_POINT('Ctrl Pts',(3.7583820388737,39.4249999998524,11.5671105274568));
#295358=CARTESIAN_POINT('Ctrl Pts',(7.51676407774742,39.5749999998518,10.3459381770588));
#295359=CARTESIAN_POINT('Ctrl Pts',(9.83957192047851,39.7249999998512,7.14886745759505));
#295360=CARTESIAN_POINT('Ctrl Pts',(12.1623797632096,39.8749999998506,3.95179673813132));
#295361=CARTESIAN_POINT('Ctrl Pts',(12.1623797632096,40.02499999985,-1.48946194470292E-15));
#295362=CARTESIAN_POINT('Ctrl Pts',(12.1623797632096,40.1749999998494,-3.95179673813132));
#295363=CARTESIAN_POINT('Ctrl Pts',(9.83957192047851,40.3249999998488,-7.14886745759505));
#295364=CARTESIAN_POINT('Ctrl Pts',(7.51676407774742,40.4749999998482,-10.3459381770588));
#295365=CARTESIAN_POINT('Ctrl Pts',(3.75838203887369,40.6249999998476,-11.5671105274568));
#295366=CARTESIAN_POINT('Ctrl Pts',(-3.67431284208903E-14,40.774999999847,
-12.7882828778549));
#295367=CARTESIAN_POINT('Ctrl Pts',(-3.75838203887376,40.9249999998464,
-11.5671105274568));
#295368=CARTESIAN_POINT('Ctrl Pts',(-7.51676407774749,41.0749999998458,
-10.3459381770588));
#295369=CARTESIAN_POINT('Ctrl Pts',(-9.83957192047858,41.2249999998452,
-7.14886745759505));
#295370=CARTESIAN_POINT('Ctrl Pts',(-12.1623797632097,41.3749999998446,
-3.95179673813132));
#295371=CARTESIAN_POINT('Ctrl Pts',(-12.1623797632097,41.524999999844,2.97892388940585E-15));
#295372=CARTESIAN_POINT('Ctrl Pts',(-12.1623797632097,41.6749999998434,
3.95179673813133));
#295373=CARTESIAN_POINT('Ctrl Pts',(-9.83957192047858,41.8249999998428,
7.14886745759505));
#295374=CARTESIAN_POINT('Ctrl Pts',(-7.51676407774749,41.9749999998422,
10.3459381770588));
#295375=CARTESIAN_POINT('Ctrl Pts',(-3.75838203887376,42.1249999998416,
11.5671105274568));
#295376=CARTESIAN_POINT('Ctrl Pts',(-3.44747571181301E-14,42.274999999841,
12.7882828778549));
#295377=CARTESIAN_POINT('Ctrl Pts',(3.75838203887369,42.4249999998404,11.5671105274568));
#295378=CARTESIAN_POINT('Ctrl Pts',(7.51676407774742,42.5749999998398,10.3459381770588));
#295379=CARTESIAN_POINT('Ctrl Pts',(9.83957192047851,42.7249999998392,7.14886745759505));
#295380=CARTESIAN_POINT('Ctrl Pts',(12.1623797632096,42.8749999998386,3.95179673813132));
#295381=CARTESIAN_POINT('Ctrl Pts',(12.1623797632096,43.024999999838,-1.48946194470292E-15));
#295382=CARTESIAN_POINT('Ctrl Pts',(12.1623797632096,43.1749999998374,-3.95179673813132));
#295383=CARTESIAN_POINT('Ctrl Pts',(9.83957192047851,43.3249999998368,-7.14886745759505));
#295384=CARTESIAN_POINT('Ctrl Pts',(7.51676407774742,43.4749999998362,-10.3459381770588));
#295385=CARTESIAN_POINT('Ctrl Pts',(3.75838203887369,43.6249999998356,-11.5671105274568));
#295386=CARTESIAN_POINT('Ctrl Pts',(-3.84708376925522E-14,43.774999999835,
-12.7882828778549));
#295387=CARTESIAN_POINT('Ctrl Pts',(-3.75838203887377,43.9249999998344,
-11.5671105274568));
#295388=CARTESIAN_POINT('Ctrl Pts',(-7.51676407774749,44.0749999998338,
-10.3459381770588));
#295389=CARTESIAN_POINT('Ctrl Pts',(-9.83957192047859,44.2249999998332,
-7.14886745759505));
#295390=CARTESIAN_POINT('Ctrl Pts',(-12.1623797632097,44.3749999998326,
-3.95179673813132));
#295391=CARTESIAN_POINT('Ctrl Pts',(-12.1623797632097,44.524999999832,2.97892388940585E-15));
#295392=CARTESIAN_POINT('Ctrl Pts',(-12.1623797632097,44.6749999998314,
3.95179673813133));
#295393=CARTESIAN_POINT('Ctrl Pts',(-9.83957192047859,44.8249999998308,
7.14886745759505));
#295394=CARTESIAN_POINT('Ctrl Pts',(-7.51676407774749,44.9749999998302,
10.3459381770588));
#295395=CARTESIAN_POINT('Ctrl Pts',(-3.75838203887376,45.1249999998296,
11.5671105274568));
#295396=CARTESIAN_POINT('Ctrl Pts',(-3.62024663897919E-14,45.274999999829,
12.7882828778549));
#295397=CARTESIAN_POINT('Ctrl Pts',(3.75838203887369,45.4249999998284,11.5671105274568));
#295398=CARTESIAN_POINT('Ctrl Pts',(7.51676407774742,45.5749999998278,10.3459381770588));
#295399=CARTESIAN_POINT('Ctrl Pts',(9.83957192047851,45.7249999998272,7.14886745759505));
#295400=CARTESIAN_POINT('Ctrl Pts',(12.1623797632096,45.8749999998266,3.95179673813132));
#295401=CARTESIAN_POINT('Ctrl Pts',(12.1623797632096,46.024999999826,-1.48946194470292E-15));
#295402=CARTESIAN_POINT('Ctrl Pts',(12.1623797632096,46.1749999998254,-3.95179673813132));
#295403=CARTESIAN_POINT('Ctrl Pts',(9.83957192047851,46.3249999998248,-7.14886745759505));
#295404=CARTESIAN_POINT('Ctrl Pts',(7.51676407774742,46.4749999998242,-10.3459381770588));
#295405=CARTESIAN_POINT('Ctrl Pts',(3.75838203887369,46.6249999998236,-11.5671105274568));
#295406=CARTESIAN_POINT('Ctrl Pts',(-4.0198546964214E-14,46.774999999823,
-12.7882828778549));
#295407=CARTESIAN_POINT('Ctrl Pts',(-3.75838203887377,46.9249999998224,
-11.5671105274568));
#295408=CARTESIAN_POINT('Ctrl Pts',(-7.5167640777475,47.0749999998218,-10.3459381770588));
#295409=CARTESIAN_POINT('Ctrl Pts',(-9.83957192047859,47.2249999998212,
-7.14886745759505));
#295410=CARTESIAN_POINT('Ctrl Pts',(-12.1623797632097,47.3749999998206,
-3.95179673813132));
#295411=CARTESIAN_POINT('Ctrl Pts',(-12.1623797632097,47.52499999982,2.97892388940585E-15));
#295412=CARTESIAN_POINT('Ctrl Pts',(-12.1623797632097,47.6749999998194,
3.95179673813133));
#295413=CARTESIAN_POINT('Ctrl Pts',(-9.83957192047859,47.8249999998188,
7.14886745759505));
#295414=CARTESIAN_POINT('Ctrl Pts',(-7.51676407774749,47.9749999998182,
10.3459381770588));
#295415=CARTESIAN_POINT('Ctrl Pts',(-3.75838203887377,48.1249999998176,
11.5671105274568));
#295416=CARTESIAN_POINT('Ctrl Pts',(-3.79301756614538E-14,48.274999999817,
12.7882828778549));
#295417=CARTESIAN_POINT('Ctrl Pts',(3.75838203887369,48.4249999998164,11.5671105274568));
#295418=CARTESIAN_POINT('Ctrl Pts',(7.51676407774742,48.5749999998158,10.3459381770588));
#295419=CARTESIAN_POINT('Ctrl Pts',(9.83957192047851,48.7249999998152,7.14886745759505));
#295420=CARTESIAN_POINT('Ctrl Pts',(12.1623797632096,48.8749999998146,3.95179673813132));
#295421=CARTESIAN_POINT('Ctrl Pts',(12.1623797632096,49.024999999814,-1.48946194470292E-15));
#295422=CARTESIAN_POINT('Ctrl Pts',(12.1623797632096,49.1749999998134,-3.95179673813132));
#295423=CARTESIAN_POINT('Ctrl Pts',(9.83957192047851,49.3249999998128,-7.14886745759505));
#295424=CARTESIAN_POINT('Ctrl Pts',(7.51676407774741,49.4749999998122,-10.3459381770588));
#295425=CARTESIAN_POINT('Ctrl Pts',(3.75838203887369,49.6249999998116,-11.5671105274568));
#295426=CARTESIAN_POINT('Ctrl Pts',(-4.19262562358759E-14,49.774999999811,
-12.7882828778549));
#295427=CARTESIAN_POINT('Ctrl Pts',(-3.75838203887377,49.9249999998104,
-11.5671105274568));
#295428=CARTESIAN_POINT('Ctrl Pts',(-7.5167640777475,50.0749999998098,-10.3459381770588));
#295429=CARTESIAN_POINT('Ctrl Pts',(-9.83957192047859,50.2249999998092,
-7.14886745759505));
#295430=CARTESIAN_POINT('Ctrl Pts',(-12.1623797632097,50.3749999998086,
-3.95179673813132));
#295431=CARTESIAN_POINT('Ctrl Pts',(-12.1623797632097,50.524999999808,2.97892388940585E-15));
#295432=CARTESIAN_POINT('Ctrl Pts',(-12.1623797632097,50.6749999998074,
3.95179673813133));
#295433=CARTESIAN_POINT('Ctrl Pts',(-9.83957192047859,50.8249999998068,
7.14886745759505));
#295434=CARTESIAN_POINT('Ctrl Pts',(-7.51676407774749,50.9749999998062,
10.3459381770588));
#295435=CARTESIAN_POINT('Ctrl Pts',(-3.75838203887377,51.1249999998056,
11.5671105274568));
#295436=CARTESIAN_POINT('Ctrl Pts',(-3.96578849331156E-14,51.274999999805,
12.7882828778549));
#295437=CARTESIAN_POINT('Ctrl Pts',(3.75838203887369,51.4249999998044,11.5671105274568));
#295438=CARTESIAN_POINT('Ctrl Pts',(7.51676407774742,51.5749999998038,10.3459381770588));
#295439=CARTESIAN_POINT('Ctrl Pts',(9.83957192047851,51.7249999998032,7.14886745759505));
#295440=CARTESIAN_POINT('Ctrl Pts',(12.1623797632096,51.8749999998026,3.95179673813132));
#295441=CARTESIAN_POINT('Ctrl Pts',(12.1623797632096,52.024999999802,-1.48946194470292E-15));
#295442=CARTESIAN_POINT('Ctrl Pts',(12.1623797632096,52.1749999998014,-3.95179673813132));
#295443=CARTESIAN_POINT('Ctrl Pts',(9.8395719204785,52.3249999998008,-7.14886745759505));
#295444=CARTESIAN_POINT('Ctrl Pts',(7.51676407774741,52.4749999998002,-10.3459381770588));
#295445=CARTESIAN_POINT('Ctrl Pts',(3.75838203887368,52.6249999997996,-11.5671105274568));
#295446=CARTESIAN_POINT('Ctrl Pts',(-4.36539655075377E-14,52.774999999799,
-12.7882828778549));
#295447=CARTESIAN_POINT('Ctrl Pts',(-3.75838203887377,52.9249999997984,
-11.5671105274568));
#295448=CARTESIAN_POINT('Ctrl Pts',(-7.5167640777475,53.0749999997978,-10.3459381770588));
#295449=CARTESIAN_POINT('Ctrl Pts',(-9.83957192047859,53.2249999997972,
-7.14886745759505));
#295450=CARTESIAN_POINT('Ctrl Pts',(-12.1623797632097,53.3749999997966,
-3.95179673813132));
#295451=CARTESIAN_POINT('Ctrl Pts',(-12.1623797632097,53.524999999796,2.97892388940585E-15));
#295452=CARTESIAN_POINT('Ctrl Pts',(-12.1623797632097,53.6749999997954,
3.95179673813133));
#295453=CARTESIAN_POINT('Ctrl Pts',(-9.83957192047859,53.8249999997948,
7.14886745759505));
#295454=CARTESIAN_POINT('Ctrl Pts',(-7.5167640777475,53.9749999997942,10.3459381770588));
#295455=CARTESIAN_POINT('Ctrl Pts',(-3.75838203887377,54.1249999997936,
11.5671105274568));
#295456=CARTESIAN_POINT('Ctrl Pts',(-4.13855942047774E-14,54.274999999793,
12.7882828778549));
#295457=CARTESIAN_POINT('Ctrl Pts',(3.75838203887369,54.4249999997924,11.5671105274568));
#295458=CARTESIAN_POINT('Ctrl Pts',(7.51676407774741,54.5749999997918,10.3459381770588));
#295459=CARTESIAN_POINT('Ctrl Pts',(9.8395719204785,54.7249999997912,7.14886745759505));
#295460=CARTESIAN_POINT('Ctrl Pts',(12.1623797632096,54.8749999997906,3.95179673813132));
#295461=CARTESIAN_POINT('Ctrl Pts',(12.1623797632096,55.02499999979,-1.48946194470292E-15));
#295462=CARTESIAN_POINT('Ctrl Pts',(12.1623797632096,55.1749999997894,-3.95179673813132));
#295463=CARTESIAN_POINT('Ctrl Pts',(9.8395719204785,55.3249999997888,-7.14886745759505));
#295464=CARTESIAN_POINT('Ctrl Pts',(7.51676407774741,55.4749999997882,-10.3459381770588));
#295465=CARTESIAN_POINT('Ctrl Pts',(3.75838203887368,55.6249999997876,-11.5671105274568));
#295466=CARTESIAN_POINT('Ctrl Pts',(-4.53816747791995E-14,55.774999999787,
-12.7882828778549));
#295467=CARTESIAN_POINT('Ctrl Pts',(-3.75838203887377,55.9249999997864,
-11.5671105274568));
#295468=CARTESIAN_POINT('Ctrl Pts',(-7.5167640777475,56.0749999997858,-10.3459381770588));
#295469=CARTESIAN_POINT('Ctrl Pts',(-9.83957192047859,56.2249999997852,
-7.14886745759505));
#295470=CARTESIAN_POINT('Ctrl Pts',(-12.1623797632097,56.3749999997846,
-3.95179673813132));
#295471=CARTESIAN_POINT('Ctrl Pts',(-12.1623797632097,56.524999999784,2.97892388940585E-15));
#295472=CARTESIAN_POINT('Ctrl Pts',(-12.1623797632097,56.6749999997834,
3.95179673813133));
#295473=CARTESIAN_POINT('Ctrl Pts',(-9.83957192047859,56.8249999997828,
7.14886745759505));
#295474=CARTESIAN_POINT('Ctrl Pts',(-7.5167640777475,56.9749999997822,10.3459381770588));
#295475=CARTESIAN_POINT('Ctrl Pts',(-3.75838203887377,57.1249999997816,
11.5671105274568));
#295476=CARTESIAN_POINT('Ctrl Pts',(-4.31133034764393E-14,57.274999999781,
12.7882828778549));
#295477=CARTESIAN_POINT('Ctrl Pts',(3.75838203887368,57.4249999997804,11.5671105274568));
#295478=CARTESIAN_POINT('Ctrl Pts',(7.51676407774741,57.5749999997798,10.3459381770588));
#295479=CARTESIAN_POINT('Ctrl Pts',(9.8395719204785,57.7249999997792,7.14886745759505));
#295480=CARTESIAN_POINT('Ctrl Pts',(12.1623797632096,57.8749999997786,3.95179673813132));
#295481=CARTESIAN_POINT('Ctrl Pts',(12.1623797632096,58.024999999778,-1.48946194470292E-15));
#295482=CARTESIAN_POINT('Ctrl Pts',(12.1623797632096,58.1749999997774,-3.95179673813132));
#295483=CARTESIAN_POINT('Ctrl Pts',(9.8395719204785,58.3249999997768,-7.14886745759505));
#295484=CARTESIAN_POINT('Ctrl Pts',(7.51676407774741,58.4749999997762,-10.3459381770588));
#295485=CARTESIAN_POINT('Ctrl Pts',(3.75838203887368,58.6249999997756,-11.5671105274568));
#295486=CARTESIAN_POINT('Ctrl Pts',(-4.71093840508614E-14,58.774999999775,
-12.7882828778549));
#295487=CARTESIAN_POINT('Ctrl Pts',(-3.75838203887377,58.9249999997744,
-11.5671105274568));
#295488=CARTESIAN_POINT('Ctrl Pts',(-7.5167640777475,59.0749999997738,-10.3459381770588));
#295489=CARTESIAN_POINT('Ctrl Pts',(-9.83957192047859,59.2249999997732,
-7.14886745759505));
#295490=CARTESIAN_POINT('Ctrl Pts',(-12.1623797632097,59.3749999997726,
-3.95179673813132));
#295491=CARTESIAN_POINT('Ctrl Pts',(-12.1623797632097,59.524999999772,2.97892388940585E-15));
#295492=CARTESIAN_POINT('Ctrl Pts',(-12.1623797632097,59.6749999997714,
3.95179673813133));
#295493=CARTESIAN_POINT('Ctrl Pts',(-9.83957192047859,59.8249999997708,
7.14886745759505));
#295494=CARTESIAN_POINT('Ctrl Pts',(-7.5167640777475,59.9749999997702,10.3459381770588));
#295495=CARTESIAN_POINT('Ctrl Pts',(-3.75838203887377,60.1249999997696,
11.5671105274568));
#295496=CARTESIAN_POINT('Ctrl Pts',(-4.48410127481011E-14,60.274999999769,
12.7882828778549));
#295497=CARTESIAN_POINT('Ctrl Pts',(3.75838203887368,60.4249999997684,11.5671105274568));
#295498=CARTESIAN_POINT('Ctrl Pts',(7.51676407774741,60.5749999997678,10.3459381770588));
#295499=CARTESIAN_POINT('Ctrl Pts',(9.8395719204785,60.7249999997672,7.14886745759505));
#295500=CARTESIAN_POINT('Ctrl Pts',(12.1623797632096,60.8749999997666,3.95179673813132));
#295501=CARTESIAN_POINT('Ctrl Pts',(12.1623797632096,61.024999999766,-1.48946194470292E-15));
#295502=CARTESIAN_POINT('Ctrl Pts',(12.1623797632096,61.1749999997654,-3.95179673813132));
#295503=CARTESIAN_POINT('Ctrl Pts',(9.8395719204785,61.3249999997648,-7.14886745759505));
#295504=CARTESIAN_POINT('Ctrl Pts',(7.51676407774741,61.4749999997642,-10.3459381770588));
#295505=CARTESIAN_POINT('Ctrl Pts',(3.75838203887368,61.6249999997636,-11.5671105274568));
#295506=CARTESIAN_POINT('Ctrl Pts',(-4.88370933225232E-14,61.774999999763,
-12.7882828778549));
#295507=CARTESIAN_POINT('Ctrl Pts',(-3.75838203887378,61.9249999997624,
-11.5671105274568));
#295508=CARTESIAN_POINT('Ctrl Pts',(-7.5167640777475,62.0749999997618,-10.3459381770588));
#295509=CARTESIAN_POINT('Ctrl Pts',(-9.8395719204786,62.2249999997612,-7.14886745759505));
#295510=CARTESIAN_POINT('Ctrl Pts',(-12.1623797632097,62.3749999997606,
-3.95179673813132));
#295511=CARTESIAN_POINT('Ctrl Pts',(-12.1623797632097,62.52499999976,2.97892388940585E-15));
#295512=CARTESIAN_POINT('Ctrl Pts',(-12.1623797632097,62.6749999997594,
3.95179673813133));
#295513=CARTESIAN_POINT('Ctrl Pts',(-9.8395719204786,62.8249999997588,7.14886745759505));
#295514=CARTESIAN_POINT('Ctrl Pts',(-7.5167640777475,62.9749999997582,10.3459381770588));
#295515=CARTESIAN_POINT('Ctrl Pts',(-3.75838203887377,63.1249999997576,
11.5671105274568));
#295516=CARTESIAN_POINT('Ctrl Pts',(-4.6568722019763E-14,63.274999999757,
12.7882828778549));
#295517=CARTESIAN_POINT('Ctrl Pts',(3.75838203887368,63.4249999997564,11.5671105274568));
#295518=CARTESIAN_POINT('Ctrl Pts',(7.51676407774741,63.5749999997558,10.3459381770588));
#295519=CARTESIAN_POINT('Ctrl Pts',(9.8395719204785,63.7249999997552,7.14886745759505));
#295520=CARTESIAN_POINT('Ctrl Pts',(12.1623797632096,63.8749999997546,3.95179673813132));
#295521=CARTESIAN_POINT('Ctrl Pts',(12.1623797632096,64.024999999754,-1.48946194470292E-15));
#295522=CARTESIAN_POINT('Ctrl Pts',(12.1623797632096,64.1749999997534,-3.95179673813132));
#295523=CARTESIAN_POINT('Ctrl Pts',(9.8395719204785,64.3249999997528,-7.14886745759505));
#295524=CARTESIAN_POINT('Ctrl Pts',(7.5167640777474,64.4749999997522,-10.3459381770588));
#295525=CARTESIAN_POINT('Ctrl Pts',(3.75838203887368,64.6249999997516,-11.5671105274568));
#295526=CARTESIAN_POINT('Ctrl Pts',(-5.05648025941851E-14,64.774999999751,
-12.7882828778549));
#295527=CARTESIAN_POINT('Ctrl Pts',(-3.75838203887378,64.9249999997504,
-11.5671105274568));
#295528=CARTESIAN_POINT('Ctrl Pts',(-7.51676407774751,65.0749999997498,
-10.3459381770588));
#295529=CARTESIAN_POINT('Ctrl Pts',(-9.8395719204786,65.2249999997492,-7.14886745759505));
#295530=CARTESIAN_POINT('Ctrl Pts',(-12.1623797632097,65.3749999997486,
-3.95179673813132));
#295531=CARTESIAN_POINT('Ctrl Pts',(-12.1623797632097,65.524999999748,2.97892388940585E-15));
#295532=CARTESIAN_POINT('Ctrl Pts',(-12.1623797632097,65.6749999997474,
3.95179673813133));
#295533=CARTESIAN_POINT('Ctrl Pts',(-9.8395719204786,65.8249999997468,7.14886745759505));
#295534=CARTESIAN_POINT('Ctrl Pts',(-7.5167640777475,65.9749999997462,10.3459381770588));
#295535=CARTESIAN_POINT('Ctrl Pts',(-3.75838203887378,66.1249999997456,
11.5671105274568));
#295536=CARTESIAN_POINT('Ctrl Pts',(-4.82964312914248E-14,66.274999999745,
12.7882828778549));
#295537=CARTESIAN_POINT('Ctrl Pts',(3.75838203887368,66.4249999997444,11.5671105274568));
#295538=CARTESIAN_POINT('Ctrl Pts',(7.51676407774741,66.5749999997438,10.3459381770588));
#295539=CARTESIAN_POINT('Ctrl Pts',(9.8395719204785,66.7249999997432,7.14886745759505));
#295540=CARTESIAN_POINT('Ctrl Pts',(12.1623797632096,66.8749999997426,3.95179673813132));
#295541=CARTESIAN_POINT('Ctrl Pts',(12.1623797632096,67.024999999742,-1.48946194470292E-15));
#295542=CARTESIAN_POINT('Ctrl Pts',(12.1623797632096,67.1749999997414,-3.95179673813132));
#295543=CARTESIAN_POINT('Ctrl Pts',(9.8395719204785,67.3249999997408,-7.14886745759505));
#295544=CARTESIAN_POINT('Ctrl Pts',(7.5167640777474,67.4749999997402,-10.3459381770588));
#295545=CARTESIAN_POINT('Ctrl Pts',(3.75838203887368,67.6249999997396,-11.5671105274568));
#295546=CARTESIAN_POINT('Ctrl Pts',(-5.22925118658469E-14,67.774999999739,
-12.7882828778549));
#295547=CARTESIAN_POINT('Ctrl Pts',(-3.75838203887378,67.9249999997384,
-11.5671105274568));
#295548=CARTESIAN_POINT('Ctrl Pts',(-7.51676407774751,68.0749999997378,
-10.3459381770588));
#295549=CARTESIAN_POINT('Ctrl Pts',(-9.8395719204786,68.2249999997372,-7.14886745759505));
#295550=CARTESIAN_POINT('Ctrl Pts',(-12.1623797632097,68.3749999997366,
-3.95179673813132));
#295551=CARTESIAN_POINT('Ctrl Pts',(-12.1623797632097,68.524999999736,2.97892388940585E-15));
#295552=CARTESIAN_POINT('Ctrl Pts',(-12.1623797632097,68.6749999997354,
3.95179673813133));
#295553=CARTESIAN_POINT('Ctrl Pts',(-9.8395719204786,68.8249999997348,7.14886745759505));
#295554=CARTESIAN_POINT('Ctrl Pts',(-7.51676407774751,68.9749999997342,
10.3459381770588));
#295555=CARTESIAN_POINT('Ctrl Pts',(-3.75838203887378,69.1249999997336,
11.5671105274568));
#295556=CARTESIAN_POINT('Ctrl Pts',(-5.00241405630866E-14,69.274999999733,
12.7882828778549));
#295557=CARTESIAN_POINT('Ctrl Pts',(3.75838203887368,69.4249999997324,11.5671105274568));
#295558=CARTESIAN_POINT('Ctrl Pts',(7.5167640777474,69.5749999997318,10.3459381770588));
#295559=CARTESIAN_POINT('Ctrl Pts',(9.8395719204785,69.7249999997312,7.14886745759505));
#295560=CARTESIAN_POINT('Ctrl Pts',(12.1623797632096,69.8749999997306,3.95179673813132));
#295561=CARTESIAN_POINT('Ctrl Pts',(12.1623797632096,70.02499999973,-1.48946194470292E-15));
#295562=CARTESIAN_POINT('Ctrl Pts',(12.1623797632096,70.1749999997294,-3.95179673813132));
#295563=CARTESIAN_POINT('Ctrl Pts',(9.83957192047849,70.3249999997288,-7.14886745759505));
#295564=CARTESIAN_POINT('Ctrl Pts',(7.5167640777474,70.4749999997282,-10.3459381770588));
#295565=CARTESIAN_POINT('Ctrl Pts',(3.75838203887367,70.6249999997276,-11.5671105274568));
#295566=CARTESIAN_POINT('Ctrl Pts',(-5.40202211375087E-14,70.774999999727,
-12.7882828778549));
#295567=CARTESIAN_POINT('Ctrl Pts',(-3.75838203887378,70.9249999997264,
-11.5671105274568));
#295568=CARTESIAN_POINT('Ctrl Pts',(-7.51676407774751,71.0749999997258,
-10.3459381770588));
#295569=CARTESIAN_POINT('Ctrl Pts',(-9.8395719204786,71.2249999997252,-7.14886745759505));
#295570=CARTESIAN_POINT('Ctrl Pts',(-12.1623797632097,71.3749999997246,
-3.95179673813132));
#295571=CARTESIAN_POINT('Ctrl Pts',(-12.1623797632097,71.524999999724,2.97892388940585E-15));
#295572=CARTESIAN_POINT('Ctrl Pts',(-12.1623797632097,71.6749999997234,
3.95179673813133));
#295573=CARTESIAN_POINT('Ctrl Pts',(-9.8395719204786,71.8249999997228,7.14886745759505));
#295574=CARTESIAN_POINT('Ctrl Pts',(-7.51676407774751,71.9749999997222,
10.3459381770588));
#295575=CARTESIAN_POINT('Ctrl Pts',(-3.75838203887378,72.1249999997216,
11.5671105274568));
#295576=CARTESIAN_POINT('Ctrl Pts',(-5.17518498347485E-14,72.274999999721,
12.7882828778549));
#295577=CARTESIAN_POINT('Ctrl Pts',(3.75838203887368,72.4249999997204,11.5671105274568));
#295578=CARTESIAN_POINT('Ctrl Pts',(7.5167640777474,72.5749999997198,10.3459381770588));
#295579=CARTESIAN_POINT('Ctrl Pts',(9.83957192047849,72.7249999997192,7.14886745759505));
#295580=CARTESIAN_POINT('Ctrl Pts',(12.1623797632096,72.8749999997186,3.95179673813132));
#295581=CARTESIAN_POINT('Ctrl Pts',(12.1623797632096,73.024999999718,-1.48946194470292E-15));
#295582=CARTESIAN_POINT('Ctrl Pts',(12.1623797632096,73.1749999997174,-3.95179673813132));
#295583=CARTESIAN_POINT('Ctrl Pts',(9.83957192047849,73.3249999997168,-7.14886745759505));
#295584=CARTESIAN_POINT('Ctrl Pts',(7.5167640777474,73.4749999997162,-10.3459381770588));
#295585=CARTESIAN_POINT('Ctrl Pts',(3.75838203887367,73.6249999997156,-11.5671105274568));
#295586=CARTESIAN_POINT('Ctrl Pts',(-5.57479304091706E-14,73.774999999715,
-12.7882828778549));
#295587=CARTESIAN_POINT('Ctrl Pts',(-3.75838203887378,73.9249999997144,
-11.5671105274568));
#295588=CARTESIAN_POINT('Ctrl Pts',(-7.51676407774751,74.0749999997138,
-10.3459381770588));
#295589=CARTESIAN_POINT('Ctrl Pts',(-9.8395719204786,74.2249999997132,-7.14886745759505));
#295590=CARTESIAN_POINT('Ctrl Pts',(-12.1623797632097,74.3749999997126,
-3.95179673813132));
#295591=CARTESIAN_POINT('Ctrl Pts',(-12.1623797632097,74.524999999712,2.97892388940585E-15));
#295592=CARTESIAN_POINT('Ctrl Pts',(-12.1623797632097,74.6749999997114,
3.95179673813133));
#295593=CARTESIAN_POINT('Ctrl Pts',(-9.8395719204786,74.8249999997108,7.14886745759505));
#295594=CARTESIAN_POINT('Ctrl Pts',(-7.51676407774751,74.9749999997102,
10.3459381770588));
#295595=CARTESIAN_POINT('Ctrl Pts',(-3.75838203887378,75.1249999997096,
11.5671105274568));
#295596=CARTESIAN_POINT('Ctrl Pts',(-5.34795591064103E-14,75.274999999709,
12.7882828778549));
#295597=CARTESIAN_POINT('Ctrl Pts',(3.75838203887367,75.4249999997084,11.5671105274568));
#295598=CARTESIAN_POINT('Ctrl Pts',(7.5167640777474,75.5749999997078,10.3459381770588));
#295599=CARTESIAN_POINT('Ctrl Pts',(9.83957192047849,75.7249999997072,7.14886745759505));
#295600=CARTESIAN_POINT('Ctrl Pts',(12.1623797632096,75.8749999997066,3.95179673813132));
#295601=CARTESIAN_POINT('Ctrl Pts',(12.1623797632096,76.024999999706,-1.48946194470292E-15));
#295602=CARTESIAN_POINT('Ctrl Pts',(12.1623797632096,76.1749999997054,-3.95179673813132));
#295603=CARTESIAN_POINT('Ctrl Pts',(9.83957192047849,76.3249999997048,-7.14886745759505));
#295604=CARTESIAN_POINT('Ctrl Pts',(7.5167640777474,76.4749999997042,-10.3459381770588));
#295605=CARTESIAN_POINT('Ctrl Pts',(3.75838203887367,76.6249999997036,-11.5671105274568));
#295606=CARTESIAN_POINT('Ctrl Pts',(-5.74756396808324E-14,76.774999999703,
-12.7882828778549));
#295607=CARTESIAN_POINT('Ctrl Pts',(-3.75838203887379,76.9249999997024,
-11.5671105274568));
#295608=CARTESIAN_POINT('Ctrl Pts',(-7.51676407774751,77.0749999997018,
-10.3459381770588));
#295609=CARTESIAN_POINT('Ctrl Pts',(-9.8395719204786,77.2249999997012,-7.14886745759505));
#295610=CARTESIAN_POINT('Ctrl Pts',(-12.1623797632097,77.3749999997006,
-3.95179673813132));
#295611=CARTESIAN_POINT('Ctrl Pts',(-12.1623797632097,77.5249999997,2.97892388940585E-15));
#295612=CARTESIAN_POINT('Ctrl Pts',(-12.1623797632097,77.6749999996994,
3.95179673813133));
#295613=CARTESIAN_POINT('Ctrl Pts',(-9.8395719204786,77.8249999996988,7.14886745759505));
#295614=CARTESIAN_POINT('Ctrl Pts',(-7.51676407774751,77.9749999996982,
10.3459381770588));
#295615=CARTESIAN_POINT('Ctrl Pts',(-3.75838203887378,78.1249999996976,
11.5671105274568));
#295616=CARTESIAN_POINT('Ctrl Pts',(-5.52072683780721E-14,78.274999999697,
12.7882828778549));
#295617=CARTESIAN_POINT('Ctrl Pts',(3.75838203887367,78.4249999996964,11.5671105274568));
#295618=CARTESIAN_POINT('Ctrl Pts',(7.5167640777474,78.5749999996958,10.3459381770588));
#295619=CARTESIAN_POINT('Ctrl Pts',(9.83957192047849,78.7249999996952,7.14886745759505));
#295620=CARTESIAN_POINT('Ctrl Pts',(12.1623797632096,78.8749999996946,3.95179673813132));
#295621=CARTESIAN_POINT('Ctrl Pts',(12.1623797632096,79.024999999694,-1.48946194470292E-15));
#295622=CARTESIAN_POINT('Ctrl Pts',(12.1623797632096,79.1749999996934,-3.95179673813132));
#295623=CARTESIAN_POINT('Ctrl Pts',(9.83957192047849,79.3249999996928,-7.14886745759505));
#295624=CARTESIAN_POINT('Ctrl Pts',(7.5167640777474,79.4749999996922,-10.3459381770588));
#295625=CARTESIAN_POINT('Ctrl Pts',(3.75838203887367,79.6249999996916,-11.5671105274568));
#295626=CARTESIAN_POINT('Ctrl Pts',(-5.92033489524943E-14,79.774999999691,
-12.7882828778549));
#295627=CARTESIAN_POINT('Ctrl Pts',(-3.75838203887379,79.9249999996904,
-11.5671105274568));
#295628=CARTESIAN_POINT('Ctrl Pts',(-7.51676407774751,80.0749999996898,
-10.3459381770588));
#295629=CARTESIAN_POINT('Ctrl Pts',(-9.83957192047861,80.2249999996892,
-7.14886745759505));
#295630=CARTESIAN_POINT('Ctrl Pts',(-12.1623797632097,80.3749999996886,
-3.95179673813132));
#295631=CARTESIAN_POINT('Ctrl Pts',(-12.1623797632097,80.524999999688,2.97892388940585E-15));
#295632=CARTESIAN_POINT('Ctrl Pts',(-12.1623797632097,80.6749999996874,
3.95179673813133));
#295633=CARTESIAN_POINT('Ctrl Pts',(-9.83957192047861,80.8249999996868,
7.14886745759505));
#295634=CARTESIAN_POINT('Ctrl Pts',(-7.51676407774751,80.9749999996862,
10.3459381770588));
#295635=CARTESIAN_POINT('Ctrl Pts',(-3.75838203887378,81.1249999996856,
11.5671105274568));
#295636=CARTESIAN_POINT('Ctrl Pts',(-5.6934977649734E-14,81.274999999685,
12.7882828778549));
#295637=CARTESIAN_POINT('Ctrl Pts',(3.75838203887367,81.4249999996844,11.5671105274568));
#295638=CARTESIAN_POINT('Ctrl Pts',(7.5167640777474,81.5749999996838,10.3459381770588));
#295639=CARTESIAN_POINT('Ctrl Pts',(9.83957192047849,81.7249999996832,7.14886745759505));
#295640=CARTESIAN_POINT('Ctrl Pts',(12.1623797632096,81.8749999996826,3.95179673813132));
#295641=CARTESIAN_POINT('Ctrl Pts',(12.1623797632096,82.024999999682,-1.48946194470292E-15));
#295642=CARTESIAN_POINT('Ctrl Pts',(12.1623797632096,82.1749999996814,-3.95179673813132));
#295643=CARTESIAN_POINT('Ctrl Pts',(9.83957192047849,82.3249999996808,-7.14886745759505));
#295644=CARTESIAN_POINT('Ctrl Pts',(7.5167640777474,82.4749999996802,-10.3459381770588));
#295645=CARTESIAN_POINT('Ctrl Pts',(3.75838203887367,82.6249999996796,-11.5671105274568));
#295646=CARTESIAN_POINT('Ctrl Pts',(-6.09310582241561E-14,82.774999999679,
-12.7882828778549));
#295647=CARTESIAN_POINT('Ctrl Pts',(-3.75838203887379,82.9249999996784,
-11.5671105274568));
#295648=CARTESIAN_POINT('Ctrl Pts',(-7.51676407774752,83.0749999996778,
-10.3459381770588));
#295649=CARTESIAN_POINT('Ctrl Pts',(-9.83957192047861,83.2249999996772,
-7.14886745759505));
#295650=CARTESIAN_POINT('Ctrl Pts',(-12.1623797632097,83.3749999996766,
-3.95179673813132));
#295651=CARTESIAN_POINT('Ctrl Pts',(-12.1623797632097,83.524999999676,2.97892388940585E-15));
#295652=CARTESIAN_POINT('Ctrl Pts',(-12.1623797632097,83.6749999996754,
3.95179673813133));
#295653=CARTESIAN_POINT('Ctrl Pts',(-9.83957192047861,83.8249999996748,
7.14886745759505));
#295654=CARTESIAN_POINT('Ctrl Pts',(-7.51676407774751,83.9749999996742,
10.3459381770588));
#295655=CARTESIAN_POINT('Ctrl Pts',(-3.75838203887379,84.1249999996736,
11.5671105274568));
#295656=CARTESIAN_POINT('Ctrl Pts',(-5.86626869213958E-14,84.274999999673,
12.7882828778549));
#295657=CARTESIAN_POINT('Ctrl Pts',(3.75838203887367,84.4249999996724,11.5671105274568));
#295658=CARTESIAN_POINT('Ctrl Pts',(7.5167640777474,84.5749999996718,10.3459381770588));
#295659=CARTESIAN_POINT('Ctrl Pts',(9.83957192047849,84.7249999996712,7.14886745759505));
#295660=CARTESIAN_POINT('Ctrl Pts',(12.1623797632096,84.8749999996706,3.95179673813132));
#295661=CARTESIAN_POINT('Ctrl Pts',(12.1623797632096,85.02499999967,-1.48946194470292E-15));
#295662=CARTESIAN_POINT('Ctrl Pts',(12.1623797632096,85.1749999996694,-3.95179673813132));
#295663=CARTESIAN_POINT('Ctrl Pts',(9.83957192047849,85.3249999996688,-7.14886745759505));
#295664=CARTESIAN_POINT('Ctrl Pts',(7.51676407774739,85.4749999996682,-10.3459381770588));
#295665=CARTESIAN_POINT('Ctrl Pts',(3.75838203887367,85.6249999996676,-11.5671105274568));
#295666=CARTESIAN_POINT('Ctrl Pts',(-6.26587674958179E-14,85.774999999667,
-12.7882828778549));
#295667=CARTESIAN_POINT('Ctrl Pts',(-3.75838203887379,85.9249999996664,
-11.5671105274568));
#295668=CARTESIAN_POINT('Ctrl Pts',(-7.51676407774752,86.0749999996658,
-10.3459381770588));
#295669=CARTESIAN_POINT('Ctrl Pts',(-9.83957192047861,86.2249999996652,
-7.14886745759505));
#295670=CARTESIAN_POINT('Ctrl Pts',(-12.1623797632097,86.3749999996646,
-3.95179673813132));
#295671=CARTESIAN_POINT('Ctrl Pts',(-12.1623797632097,86.524999999664,2.97892388940585E-15));
#295672=CARTESIAN_POINT('Ctrl Pts',(-12.1623797632097,86.6749999996634,
3.95179673813133));
#295673=CARTESIAN_POINT('Ctrl Pts',(-9.83957192047861,86.8249999996628,
7.14886745759505));
#295674=CARTESIAN_POINT('Ctrl Pts',(-7.51676407774752,86.9749999996622,
10.3459381770588));
#295675=CARTESIAN_POINT('Ctrl Pts',(-3.75838203887379,87.1249999996616,
11.5671105274568));
#295676=CARTESIAN_POINT('Ctrl Pts',(-6.03903961930577E-14,87.274999999661,
12.7882828778549));
#295677=CARTESIAN_POINT('Ctrl Pts',(3.75838203887367,87.4249999996604,11.5671105274568));
#295678=CARTESIAN_POINT('Ctrl Pts',(7.5167640777474,87.5749999996598,10.3459381770588));
#295679=CARTESIAN_POINT('Ctrl Pts',(9.83957192047849,87.7249999996592,7.14886745759505));
#295680=CARTESIAN_POINT('Ctrl Pts',(12.1623797632096,87.8749999996586,3.95179673813132));
#295681=CARTESIAN_POINT('Ctrl Pts',(12.1623797632096,88.024999999658,-1.48946194470292E-15));
#295682=CARTESIAN_POINT('Ctrl Pts',(12.1623797632096,88.1749999996574,-3.95179673813132));
#295683=CARTESIAN_POINT('Ctrl Pts',(9.83957192047849,88.3249999996568,-7.14886745759505));
#295684=CARTESIAN_POINT('Ctrl Pts',(7.51676407774739,88.4749999996562,-10.3459381770588));
#295685=CARTESIAN_POINT('Ctrl Pts',(3.75838203887366,88.6249999996556,-11.5671105274568));
#295686=CARTESIAN_POINT('Ctrl Pts',(-6.43864767674798E-14,88.774999999655,
-12.7882828778549));
#295687=CARTESIAN_POINT('Ctrl Pts',(-3.75838203887379,88.9249999996544,
-11.5671105274568));
#295688=CARTESIAN_POINT('Ctrl Pts',(-7.51676407774752,89.0749999996538,
-10.3459381770588));
#295689=CARTESIAN_POINT('Ctrl Pts',(-9.83957192047861,89.2249999996532,
-7.14886745759505));
#295690=CARTESIAN_POINT('Ctrl Pts',(-12.1623797632097,89.3749999996526,
-3.95179673813132));
#295691=CARTESIAN_POINT('Ctrl Pts',(-12.1623797632097,89.524999999652,2.97892388940585E-15));
#295692=CARTESIAN_POINT('Ctrl Pts',(-12.1623797632097,89.6749999996514,
3.95179673813133));
#295693=CARTESIAN_POINT('Ctrl Pts',(-9.83957192047861,89.8249999996508,
7.14886745759505));
#295694=CARTESIAN_POINT('Ctrl Pts',(-7.51676407774752,89.9749999996502,
10.3459381770588));
#295695=CARTESIAN_POINT('Ctrl Pts',(-3.75838203887379,90.1249999996496,
11.5671105274568));
#295696=CARTESIAN_POINT('Ctrl Pts',(-6.21181054647195E-14,90.274999999649,
12.7882828778549));
#295697=CARTESIAN_POINT('Ctrl Pts',(3.75838203887366,90.4249999996484,11.5671105274568));
#295698=CARTESIAN_POINT('Ctrl Pts',(7.51676407774739,90.5749999996478,10.3459381770588));
#295699=CARTESIAN_POINT('Ctrl Pts',(9.83957192047848,90.7249999996472,7.14886745759505));
#295700=CARTESIAN_POINT('Ctrl Pts',(12.1623797632096,90.8749999996466,3.95179673813132));
#295701=CARTESIAN_POINT('Ctrl Pts',(12.1623797632096,91.024999999646,-1.48946194470292E-15));
#295702=CARTESIAN_POINT('Ctrl Pts',(12.1623797632096,91.1749999996454,-3.95179673813132));
#295703=CARTESIAN_POINT('Ctrl Pts',(9.83957192047848,91.3249999996448,-7.14886745759505));
#295704=CARTESIAN_POINT('Ctrl Pts',(7.51676407774739,91.4749999996442,-10.3459381770588));
#295705=CARTESIAN_POINT('Ctrl Pts',(3.75838203887366,91.6249999996436,-11.5671105274568));
#295706=CARTESIAN_POINT('Ctrl Pts',(-6.61141860391416E-14,91.774999999643,
-12.7882828778549));
#295707=CARTESIAN_POINT('Ctrl Pts',(-3.75838203887379,91.9249999996424,
-11.5671105274568));
#295708=CARTESIAN_POINT('Ctrl Pts',(-7.51676407774752,92.0749999996418,
-10.3459381770588));
#295709=CARTESIAN_POINT('Ctrl Pts',(-9.83957192047861,92.2249999996412,
-7.14886745759505));
#295710=CARTESIAN_POINT('Ctrl Pts',(-12.1623797632097,92.3749999996406,
-3.95179673813132));
#295711=CARTESIAN_POINT('Ctrl Pts',(-12.1623797632097,92.52499999964,2.97892388940585E-15));
#295712=CARTESIAN_POINT('Ctrl Pts',(-12.1623797632097,92.6749999996394,
3.95179673813133));
#295713=CARTESIAN_POINT('Ctrl Pts',(-9.83957192047861,92.8249999996388,
7.14886745759505));
#295714=CARTESIAN_POINT('Ctrl Pts',(-7.51676407774752,92.9749999996382,
10.3459381770588));
#295715=CARTESIAN_POINT('Ctrl Pts',(-3.75838203887379,93.1249999996376,
11.5671105274568));
#295716=CARTESIAN_POINT('Ctrl Pts',(-6.38458147363813E-14,93.274999999637,
12.7882828778549));
#295717=CARTESIAN_POINT('Ctrl Pts',(3.75838203887366,93.4249999996364,11.5671105274568));
#295718=CARTESIAN_POINT('Ctrl Pts',(7.51676407774739,93.5749999996358,10.3459381770588));
#295719=CARTESIAN_POINT('Ctrl Pts',(9.83957192047848,93.7249999996352,7.14886745759505));
#295720=CARTESIAN_POINT('Ctrl Pts',(12.1623797632096,93.8749999996346,3.95179673813132));
#295721=CARTESIAN_POINT('Ctrl Pts',(12.1623797632096,94.024999999634,-1.48946194470292E-15));
#295722=CARTESIAN_POINT('Ctrl Pts',(12.1623797632096,94.1749999996334,-3.95179673813132));
#295723=CARTESIAN_POINT('Ctrl Pts',(9.83957192047848,94.3249999996328,-7.14886745759505));
#295724=CARTESIAN_POINT('Ctrl Pts',(7.51676407774739,94.4749999996322,-10.3459381770588));
#295725=CARTESIAN_POINT('Ctrl Pts',(3.75838203887366,94.6249999996316,-11.5671105274568));
#295726=CARTESIAN_POINT('Ctrl Pts',(-6.78418953108034E-14,94.774999999631,
-12.7882828778549));
#295727=CARTESIAN_POINT('Ctrl Pts',(-3.7583820388738,94.9249999996304,-11.5671105274568));
#295728=CARTESIAN_POINT('Ctrl Pts',(-7.51676407774752,95.0749999996298,
-10.3459381770588));
#295729=CARTESIAN_POINT('Ctrl Pts',(-9.83957192047862,95.2249999996292,
-7.14886745759505));
#295730=CARTESIAN_POINT('Ctrl Pts',(-12.1623797632097,95.3749999996286,
-3.95179673813132));
#295731=CARTESIAN_POINT('Ctrl Pts',(-12.1623797632097,95.524999999628,2.97892388940585E-15));
#295732=CARTESIAN_POINT('Ctrl Pts',(-12.1623797632097,95.6749999996274,
3.95179673813133));
#295733=CARTESIAN_POINT('Ctrl Pts',(-9.83957192047862,95.8249999996268,
7.14886745759505));
#295734=CARTESIAN_POINT('Ctrl Pts',(-7.51676407774752,95.9749999996262,
10.3459381770588));
#295735=CARTESIAN_POINT('Ctrl Pts',(-3.75838203887379,96.1249999996256,
11.5671105274568));
#295736=CARTESIAN_POINT('Ctrl Pts',(-6.55735240080432E-14,96.274999999625,
12.7882828778549));
#295737=CARTESIAN_POINT('Ctrl Pts',(3.75838203887366,96.4249999996244,11.5671105274568));
#295738=CARTESIAN_POINT('Ctrl Pts',(7.51676407774739,96.5749999996238,10.3459381770588));
#295739=CARTESIAN_POINT('Ctrl Pts',(9.83957192047848,96.7249999996232,7.14886745759505));
#295740=CARTESIAN_POINT('Ctrl Pts',(12.1623797632096,96.8749999996226,3.95179673813132));
#295741=CARTESIAN_POINT('Ctrl Pts',(12.1623797632096,97.024999999622,-1.48946194470292E-15));
#295742=CARTESIAN_POINT('Ctrl Pts',(12.1623797632096,97.1749999996214,-3.95179673813132));
#295743=CARTESIAN_POINT('Ctrl Pts',(9.83957192047848,97.3249999996208,-7.14886745759505));
#295744=CARTESIAN_POINT('Ctrl Pts',(7.51676407774739,97.4749999996202,-10.3459381770588));
#295745=CARTESIAN_POINT('Ctrl Pts',(3.75838203887366,97.6249999996196,-11.5671105274568));
#295746=CARTESIAN_POINT('Ctrl Pts',(-6.95696045824653E-14,97.774999999619,
-12.7882828778549));
#295747=CARTESIAN_POINT('Ctrl Pts',(-3.7583820388738,97.9249999996184,-11.5671105274568));
#295748=CARTESIAN_POINT('Ctrl Pts',(-7.51676407774752,98.0749999996178,
-10.3459381770588));
#295749=CARTESIAN_POINT('Ctrl Pts',(-9.83957192047862,98.2249999996172,
-7.14886745759505));
#295750=CARTESIAN_POINT('Ctrl Pts',(-12.1623797632097,98.3749999996166,
-3.95179673813132));
#295751=CARTESIAN_POINT('Ctrl Pts',(-12.1623797632097,98.524999999616,2.97892388940585E-15));
#295752=CARTESIAN_POINT('Ctrl Pts',(-12.1623797632097,98.6749999996154,
3.95179673813133));
#295753=CARTESIAN_POINT('Ctrl Pts',(-9.83957192047862,98.8249999996148,
7.14886745759505));
#295754=CARTESIAN_POINT('Ctrl Pts',(-7.51676407774752,98.9749999996142,
10.3459381770588));
#295755=CARTESIAN_POINT('Ctrl Pts',(-3.7583820388738,99.1249999996136,11.5671105274568));
#295756=CARTESIAN_POINT('Ctrl Pts',(-6.7301233279705E-14,99.274999999613,
12.7882828778549));
#295757=CARTESIAN_POINT('Ctrl Pts',(3.75838203887366,99.4249999996124,11.5671105274568));
#295758=CARTESIAN_POINT('Ctrl Pts',(7.51676407774739,99.5749999996118,10.3459381770588));
#295759=CARTESIAN_POINT('Ctrl Pts',(9.83957192047848,99.7249999996112,7.14886745759505));
#295760=CARTESIAN_POINT('Ctrl Pts',(12.1623797632096,99.8749999996106,3.95179673813132));
#295761=CARTESIAN_POINT('Ctrl Pts',(12.1623797632096,100.02499999961,-1.48946194470292E-15));
#295762=CARTESIAN_POINT('Ctrl Pts',(12.1623797632096,100.174999999609,-3.95179673813132));
#295763=CARTESIAN_POINT('Ctrl Pts',(9.83957192047848,100.324999999609,-7.14886745759505));
#295764=CARTESIAN_POINT('Ctrl Pts',(7.51676407774738,100.474999999608,-10.3459381770588));
#295765=CARTESIAN_POINT('Ctrl Pts',(3.75838203887366,100.624999999608,-11.5671105274568));
#295766=CARTESIAN_POINT('Ctrl Pts',(-7.12973138541271E-14,100.774999999607,
-12.7882828778549));
#295767=CARTESIAN_POINT('Ctrl Pts',(-3.7583820388738,100.924999999606,-11.5671105274568));
#295768=CARTESIAN_POINT('Ctrl Pts',(-7.51676407774753,101.074999999606,
-10.3459381770588));
#295769=CARTESIAN_POINT('Ctrl Pts',(-9.83957192047862,101.224999999605,
-7.14886745759505));
#295770=CARTESIAN_POINT('Ctrl Pts',(-12.1623797632097,101.374999999605,
-3.95179673813132));
#295771=CARTESIAN_POINT('Ctrl Pts',(-12.1623797632097,101.524999999604,
2.97892388940585E-15));
#295772=CARTESIAN_POINT('Ctrl Pts',(-12.1623797632097,101.674999999603,
3.95179673813133));
#295773=CARTESIAN_POINT('Ctrl Pts',(-9.83957192047862,101.824999999603,
7.14886745759505));
#295774=CARTESIAN_POINT('Ctrl Pts',(-7.51676407774752,101.974999999602,
10.3459381770588));
#295775=CARTESIAN_POINT('Ctrl Pts',(-3.7583820388738,102.124999999602,11.5671105274568));
#295776=CARTESIAN_POINT('Ctrl Pts',(-6.90289425513669E-14,102.274999999601,
12.7882828778549));
#295777=CARTESIAN_POINT('Ctrl Pts',(3.75838203887366,102.4249999996,11.5671105274568));
#295778=CARTESIAN_POINT('Ctrl Pts',(7.51676407774739,102.5749999996,10.3459381770588));
#295779=CARTESIAN_POINT('Ctrl Pts',(9.83957192047848,102.724999999599,7.14886745759505));
#295780=CARTESIAN_POINT('Ctrl Pts',(12.1623797632096,102.874999999599,3.95179673813132));
#295781=CARTESIAN_POINT('Ctrl Pts',(12.1623797632096,103.024999999598,-1.48946194470292E-15));
#295782=CARTESIAN_POINT('Ctrl Pts',(12.1623797632096,103.174999999597,-3.95179673813132));
#295783=CARTESIAN_POINT('Ctrl Pts',(9.83957192047848,103.324999999597,-7.14886745759505));
#295784=CARTESIAN_POINT('Ctrl Pts',(7.51676407774738,103.474999999596,-10.3459381770588));
#295785=CARTESIAN_POINT('Ctrl Pts',(3.75838203887366,103.624999999596,-11.5671105274568));
#295786=CARTESIAN_POINT('Ctrl Pts',(-7.3025023125789E-14,103.774999999595,
-12.7882828778549));
#295787=CARTESIAN_POINT('Ctrl Pts',(-3.7583820388738,103.924999999594,-11.5671105274568));
#295788=CARTESIAN_POINT('Ctrl Pts',(-7.51676407774753,104.074999999594,
-10.3459381770588));
#295789=CARTESIAN_POINT('Ctrl Pts',(-9.83957192047862,104.224999999593,
-7.14886745759505));
#295790=CARTESIAN_POINT('Ctrl Pts',(-12.1623797632097,104.374999999593,
-3.95179673813132));
#295791=CARTESIAN_POINT('Ctrl Pts',(-12.1623797632097,104.524999999592,
2.97892388940585E-15));
#295792=CARTESIAN_POINT('Ctrl Pts',(-12.1623797632097,104.674999999591,
3.95179673813133));
#295793=CARTESIAN_POINT('Ctrl Pts',(-9.83957192047862,104.824999999591,
7.14886745759505));
#295794=CARTESIAN_POINT('Ctrl Pts',(-7.51676407774753,104.97499999959,10.3459381770588));
#295795=CARTESIAN_POINT('Ctrl Pts',(-3.7583820388738,105.12499999959,11.5671105274568));
#295796=CARTESIAN_POINT('Ctrl Pts',(-7.07566518230287E-14,105.274999999589,
12.7882828778549));
#295797=CARTESIAN_POINT('Ctrl Pts',(3.75838203887366,105.424999999588,11.5671105274568));
#295798=CARTESIAN_POINT('Ctrl Pts',(7.51676407774738,105.574999999588,10.3459381770588));
#295799=CARTESIAN_POINT('Ctrl Pts',(9.83957192047848,105.724999999587,7.14886745759505));
#295800=CARTESIAN_POINT('Ctrl Pts',(12.1623797632096,105.874999999587,3.95179673813132));
#295801=CARTESIAN_POINT('Ctrl Pts',(12.1623797632096,106.024999999586,-1.48946194470292E-15));
#295802=CARTESIAN_POINT('Ctrl Pts',(12.1623797632096,106.174999999585,-3.95179673813132));
#295803=CARTESIAN_POINT('Ctrl Pts',(9.83957192047848,106.324999999585,-7.14886745759505));
#295804=CARTESIAN_POINT('Ctrl Pts',(7.51676407774738,106.474999999584,-10.3459381770588));
#295805=CARTESIAN_POINT('Ctrl Pts',(3.75838203887365,106.624999999584,-11.5671105274568));
#295806=CARTESIAN_POINT('Ctrl Pts',(-7.47527323974508E-14,106.774999999583,
-12.7882828778549));
#295807=CARTESIAN_POINT('Ctrl Pts',(-3.7583820388738,106.924999999582,-11.5671105274568));
#295808=CARTESIAN_POINT('Ctrl Pts',(-7.51676407774753,107.074999999582,
-10.3459381770588));
#295809=CARTESIAN_POINT('Ctrl Pts',(-9.83957192047862,107.224999999581,
-7.14886745759505));
#295810=CARTESIAN_POINT('Ctrl Pts',(-12.1623797632097,107.374999999581,
-3.95179673813132));
#295811=CARTESIAN_POINT('Ctrl Pts',(-12.1623797632097,107.52499999958,2.97892388940585E-15));
#295812=CARTESIAN_POINT('Ctrl Pts',(-12.1623797632097,107.674999999579,
3.95179673813133));
#295813=CARTESIAN_POINT('Ctrl Pts',(-9.83957192047862,107.824999999579,
7.14886745759505));
#295814=CARTESIAN_POINT('Ctrl Pts',(-7.51676407774753,107.974999999578,
10.3459381770588));
#295815=CARTESIAN_POINT('Ctrl Pts',(-3.7583820388738,108.124999999578,11.5671105274568));
#295816=CARTESIAN_POINT('Ctrl Pts',(-7.24843610946905E-14,108.274999999577,
12.7882828778549));
#295817=CARTESIAN_POINT('Ctrl Pts',(3.75838203887366,108.424999999576,11.5671105274568));
#295818=CARTESIAN_POINT('Ctrl Pts',(7.51676407774738,108.574999999576,10.3459381770588));
#295819=CARTESIAN_POINT('Ctrl Pts',(9.83957192047847,108.724999999575,7.14886745759505));
#295820=CARTESIAN_POINT('Ctrl Pts',(12.1623797632096,108.874999999575,3.95179673813132));
#295821=CARTESIAN_POINT('Ctrl Pts',(12.1623797632096,109.024999999574,-1.48946194470292E-15));
#295822=CARTESIAN_POINT('Ctrl Pts',(12.1623797632096,109.174999999573,-3.95179673813132));
#295823=CARTESIAN_POINT('Ctrl Pts',(9.83957192047847,109.324999999573,-7.14886745759505));
#295824=CARTESIAN_POINT('Ctrl Pts',(7.51676407774738,109.474999999572,-10.3459381770588));
#295825=CARTESIAN_POINT('Ctrl Pts',(3.75838203887365,109.624999999572,-11.5671105274568));
#295826=CARTESIAN_POINT('Ctrl Pts',(-7.64804416691126E-14,109.774999999571,
-12.7882828778549));
#295827=CARTESIAN_POINT('Ctrl Pts',(-3.7583820388738,109.92499999957,-11.5671105274568));
#295828=CARTESIAN_POINT('Ctrl Pts',(-7.51676407774753,110.07499999957,-10.3459381770588));
#295829=CARTESIAN_POINT('Ctrl Pts',(-9.83957192047862,110.224999999569,
-7.14886745759505));
#295830=CARTESIAN_POINT('Ctrl Pts',(-12.1623797632097,110.374999999569,
-3.95179673813132));
#295831=CARTESIAN_POINT('Ctrl Pts',(-12.1623797632097,110.524999999568,
2.97892388940585E-15));
#295832=CARTESIAN_POINT('Ctrl Pts',(-12.1623797632097,110.674999999567,
3.95179673813133));
#295833=CARTESIAN_POINT('Ctrl Pts',(-9.83957192047862,110.824999999567,
7.14886745759505));
#295834=CARTESIAN_POINT('Ctrl Pts',(-7.51676407774753,110.974999999566,
10.3459381770588));
#295835=CARTESIAN_POINT('Ctrl Pts',(-3.7583820388738,111.124999999566,11.5671105274568));
#295836=CARTESIAN_POINT('Ctrl Pts',(-7.42120703663524E-14,111.274999999565,
12.7882828778549));
#295837=CARTESIAN_POINT('Ctrl Pts',(3.75838203887365,111.424999999564,11.5671105274568));
#295838=CARTESIAN_POINT('Ctrl Pts',(7.51676407774738,111.574999999564,10.3459381770588));
#295839=CARTESIAN_POINT('Ctrl Pts',(9.83957192047847,111.724999999563,7.14886745759505));
#295840=CARTESIAN_POINT('Ctrl Pts',(12.1623797632096,111.874999999563,3.95179673813132));
#295841=CARTESIAN_POINT('Ctrl Pts',(12.1623797632096,112.024999999562,-1.48946194470292E-15));
#295842=CARTESIAN_POINT('Ctrl Pts',(12.1623797632096,112.174999999561,-3.95179673813132));
#295843=CARTESIAN_POINT('Ctrl Pts',(9.83957192047847,112.324999999561,-7.14886745759505));
#295844=CARTESIAN_POINT('Ctrl Pts',(7.51676407774738,112.47499999956,-10.3459381770588));
#295845=CARTESIAN_POINT('Ctrl Pts',(3.75838203887365,112.62499999956,-11.5671105274568));
#295846=CARTESIAN_POINT('Ctrl Pts',(-7.82081509407745E-14,112.774999999559,
-12.7882828778549));
#295847=CARTESIAN_POINT('Ctrl Pts',(-3.75838203887381,112.924999999558,
-11.5671105274568));
#295848=CARTESIAN_POINT('Ctrl Pts',(-7.51676407774753,113.074999999558,
-10.3459381770588));
#295849=CARTESIAN_POINT('Ctrl Pts',(-9.83957192047863,113.224999999557,
-7.14886745759505));
#295850=CARTESIAN_POINT('Ctrl Pts',(-12.1623797632097,113.374999999557,
-3.95179673813132));
#295851=CARTESIAN_POINT('Ctrl Pts',(-12.1623797632097,113.524999999556,
2.97892388940585E-15));
#295852=CARTESIAN_POINT('Ctrl Pts',(-12.1623797632097,113.674999999555,
3.95179673813133));
#295853=CARTESIAN_POINT('Ctrl Pts',(-9.83957192047863,113.824999999555,
7.14886745759505));
#295854=CARTESIAN_POINT('Ctrl Pts',(-7.51676407774753,113.974999999554,
10.3459381770588));
#295855=CARTESIAN_POINT('Ctrl Pts',(-3.7583820388738,114.124999999554,11.5671105274568));
#295856=CARTESIAN_POINT('Ctrl Pts',(-7.59397796380142E-14,114.274999999553,
12.7882828778549));
#295857=CARTESIAN_POINT('Ctrl Pts',(3.75838203887365,114.424999999552,11.5671105274568));
#295858=CARTESIAN_POINT('Ctrl Pts',(7.51676407774738,114.574999999552,10.3459381770588));
#295859=CARTESIAN_POINT('Ctrl Pts',(9.83957192047847,114.724999999551,7.14886745759505));
#295860=CARTESIAN_POINT('Ctrl Pts',(12.1623797632096,114.874999999551,3.95179673813132));
#295861=CARTESIAN_POINT('Ctrl Pts',(12.1623797632096,115.02499999955,-1.48946194470292E-15));
#295862=CARTESIAN_POINT('Ctrl Pts',(12.1623797632096,115.174999999549,-3.95179673813132));
#295863=CARTESIAN_POINT('Ctrl Pts',(9.83957192047847,115.324999999549,-7.14886745759505));
#295864=CARTESIAN_POINT('Ctrl Pts',(7.51676407774738,115.474999999548,-10.3459381770588));
#295865=CARTESIAN_POINT('Ctrl Pts',(3.75838203887365,115.624999999548,-11.5671105274568));
#295866=CARTESIAN_POINT('Ctrl Pts',(-7.99358602124363E-14,115.774999999547,
-12.7882828778549));
#295867=CARTESIAN_POINT('Ctrl Pts',(-3.75838203887381,115.924999999546,
-11.5671105274568));
#295868=CARTESIAN_POINT('Ctrl Pts',(-7.51676407774754,116.074999999546,
-10.3459381770588));
#295869=CARTESIAN_POINT('Ctrl Pts',(-9.83957192047863,116.224999999545,
-7.14886745759505));
#295870=CARTESIAN_POINT('Ctrl Pts',(-12.1623797632097,116.374999999545,
-3.95179673813132));
#295871=CARTESIAN_POINT('Ctrl Pts',(-12.1623797632097,116.524999999544,
2.97892388940585E-15));
#295872=CARTESIAN_POINT('Ctrl Pts',(-12.1623797632097,116.674999999543,
3.95179673813133));
#295873=CARTESIAN_POINT('Ctrl Pts',(-9.83957192047863,116.824999999543,
7.14886745759505));
#295874=CARTESIAN_POINT('Ctrl Pts',(-7.51676407774753,116.974999999542,
10.3459381770588));
#295875=CARTESIAN_POINT('Ctrl Pts',(-3.75838203887381,117.124999999542,
11.5671105274568));
#295876=CARTESIAN_POINT('Ctrl Pts',(-7.76674889096761E-14,117.274999999541,
12.7882828778549));
#295877=CARTESIAN_POINT('Ctrl Pts',(3.75838203887365,117.42499999954,11.5671105274568));
#295878=CARTESIAN_POINT('Ctrl Pts',(7.51676407774738,117.57499999954,10.3459381770588));
#295879=CARTESIAN_POINT('Ctrl Pts',(9.83957192047847,117.724999999539,7.14886745759505));
#295880=CARTESIAN_POINT('Ctrl Pts',(12.1623797632096,117.874999999539,3.95179673813132));
#295881=CARTESIAN_POINT('Ctrl Pts',(12.1623797632096,118.024999999538,-1.48946194470292E-15));
#295882=CARTESIAN_POINT('Ctrl Pts',(12.1623797632096,118.174999999537,-3.95179673813132));
#295883=CARTESIAN_POINT('Ctrl Pts',(9.83957192047847,118.324999999537,-7.14886745759505));
#295884=CARTESIAN_POINT('Ctrl Pts',(7.51676407774737,118.474999999536,-10.3459381770588));
#295885=CARTESIAN_POINT('Ctrl Pts',(3.75838203887365,118.624999999536,-11.5671105274568));
#295886=CARTESIAN_POINT('Ctrl Pts',(-8.16635694840981E-14,118.774999999535,
-12.7882828778549));
#295887=CARTESIAN_POINT('Ctrl Pts',(-3.75838203887381,118.924999999534,
-11.5671105274568));
#295888=CARTESIAN_POINT('Ctrl Pts',(-7.51676407774754,119.074999999534,
-10.3459381770588));
#295889=CARTESIAN_POINT('Ctrl Pts',(-9.83957192047863,119.224999999533,
-7.14886745759505));
#295890=CARTESIAN_POINT('Ctrl Pts',(-12.1623797632097,119.374999999533,
-3.95179673813132));
#295891=CARTESIAN_POINT('Ctrl Pts',(-12.1623797632097,119.524999999532,
2.97892388940585E-15));
#295892=CARTESIAN_POINT('Ctrl Pts',(-12.1623797632097,119.674999999531,
3.95179673813133));
#295893=CARTESIAN_POINT('Ctrl Pts',(-9.83957192047863,119.824999999531,
7.14886745759505));
#295894=CARTESIAN_POINT('Ctrl Pts',(-7.51676407774754,119.97499999953,10.3459381770588));
#295895=CARTESIAN_POINT('Ctrl Pts',(-3.75838203887381,120.12499999953,11.5671105274568));
#295896=CARTESIAN_POINT('Ctrl Pts',(-7.93951981813379E-14,120.274999999529,
12.7882828778549));
#295897=CARTESIAN_POINT('Ctrl Pts',(3.75838203887365,120.424999999528,11.5671105274568));
#295898=CARTESIAN_POINT('Ctrl Pts',(7.51676407774738,120.574999999528,10.3459381770588));
#295899=CARTESIAN_POINT('Ctrl Pts',(9.83957192047847,120.724999999527,7.14886745759505));
#295900=CARTESIAN_POINT('Ctrl Pts',(12.1623797632096,120.874999999527,3.95179673813132));
#295901=CARTESIAN_POINT('Ctrl Pts',(12.1623797632096,121.024999999526,-1.48946194470292E-15));
#295902=CARTESIAN_POINT('Ctrl Pts',(12.1623797632096,121.174999999525,-3.95179673813132));
#295903=CARTESIAN_POINT('Ctrl Pts',(9.83957192047847,121.324999999525,-7.14886745759505));
#295904=CARTESIAN_POINT('Ctrl Pts',(7.51676407774737,121.474999999524,-10.3459381770588));
#295905=CARTESIAN_POINT('Ctrl Pts',(3.75838203887364,121.624999999524,-11.5671105274568));
#295906=CARTESIAN_POINT('Ctrl Pts',(-8.339127875576E-14,121.774999999523,
-12.7882828778549));
#295907=CARTESIAN_POINT('Ctrl Pts',(-3.75838203887381,121.924999999522,
-11.5671105274568));
#295908=CARTESIAN_POINT('Ctrl Pts',(-7.51676407774754,122.074999999522,
-10.3459381770588));
#295909=CARTESIAN_POINT('Ctrl Pts',(-9.83957192047863,122.224999999521,
-7.14886745759505));
#295910=CARTESIAN_POINT('Ctrl Pts',(-12.1623797632097,122.374999999521,
-3.95179673813132));
#295911=CARTESIAN_POINT('Ctrl Pts',(-12.1623797632097,122.52499999952,2.97892388940585E-15));
#295912=CARTESIAN_POINT('Ctrl Pts',(-12.1623797632097,122.674999999519,
3.95179673813133));
#295913=CARTESIAN_POINT('Ctrl Pts',(-9.83957192047863,122.824999999519,
7.14886745759505));
#295914=CARTESIAN_POINT('Ctrl Pts',(-7.51676407774754,122.974999999518,
10.3459381770588));
#295915=CARTESIAN_POINT('Ctrl Pts',(-3.75838203887381,123.124999999518,
11.5671105274568));
#295916=CARTESIAN_POINT('Ctrl Pts',(-8.11229074529997E-14,123.274999999517,
12.7882828778549));
#295917=CARTESIAN_POINT('Ctrl Pts',(3.75838203887365,123.424999999516,11.5671105274568));
#295918=CARTESIAN_POINT('Ctrl Pts',(7.51676407774737,123.574999999516,10.3459381770588));
#295919=CARTESIAN_POINT('Ctrl Pts',(9.83957192047846,123.724999999515,7.14886745759505));
#295920=CARTESIAN_POINT('Ctrl Pts',(12.1623797632096,123.874999999515,3.95179673813132));
#295921=CARTESIAN_POINT('Ctrl Pts',(12.1623797632096,124.024999999514,-1.48946194470292E-15));
#295922=CARTESIAN_POINT('Ctrl Pts',(12.1623797632096,124.174999999513,-3.95179673813132));
#295923=CARTESIAN_POINT('Ctrl Pts',(9.83957192047846,124.324999999513,-7.14886745759505));
#295924=CARTESIAN_POINT('Ctrl Pts',(7.51676407774737,124.474999999512,-10.3459381770588));
#295925=CARTESIAN_POINT('Ctrl Pts',(3.75838203887364,124.624999999512,-11.5671105274568));
#295926=CARTESIAN_POINT('Ctrl Pts',(-8.51189880274219E-14,124.774999999511,
-12.7882828778549));
#295927=CARTESIAN_POINT('Ctrl Pts',(-3.75838203887381,124.92499999951,-11.5671105274568));
#295928=CARTESIAN_POINT('Ctrl Pts',(-7.51676407774754,125.07499999951,-10.3459381770588));
#295929=CARTESIAN_POINT('Ctrl Pts',(-9.83957192047863,125.224999999509,
-7.14886745759505));
#295930=CARTESIAN_POINT('Ctrl Pts',(-12.1623797632097,125.374999999509,
-3.95179673813132));
#295931=CARTESIAN_POINT('Ctrl Pts',(-12.1623797632097,125.524999999508,
2.97892388940585E-15));
#295932=CARTESIAN_POINT('Ctrl Pts',(-12.1623797632097,125.674999999507,
3.95179673813133));
#295933=CARTESIAN_POINT('Ctrl Pts',(-9.83957192047863,125.824999999507,
7.14886745759505));
#295934=CARTESIAN_POINT('Ctrl Pts',(-7.51676407774754,125.974999999506,
10.3459381770588));
#295935=CARTESIAN_POINT('Ctrl Pts',(-3.75838203887381,126.124999999506,
11.5671105274568));
#295936=CARTESIAN_POINT('Ctrl Pts',(-8.28506167246616E-14,126.274999999505,
12.7882828778549));
#295937=CARTESIAN_POINT('Ctrl Pts',(3.75838203887364,126.424999999504,11.5671105274568));
#295938=CARTESIAN_POINT('Ctrl Pts',(7.51676407774737,126.574999999504,10.3459381770588));
#295939=CARTESIAN_POINT('Ctrl Pts',(9.83957192047846,126.724999999503,7.14886745759505));
#295940=CARTESIAN_POINT('Ctrl Pts',(12.1623797632096,126.874999999503,3.95179673813132));
#295941=CARTESIAN_POINT('Ctrl Pts',(12.1623797632096,127.024999999502,-1.48946194470292E-15));
#295942=CARTESIAN_POINT('Ctrl Pts',(12.1623797632096,127.174999999501,-3.95179673813132));
#295943=CARTESIAN_POINT('Ctrl Pts',(9.83957192047846,127.324999999501,-7.14886745759505));
#295944=CARTESIAN_POINT('Ctrl Pts',(7.51676407774737,127.4749999995,-10.3459381770588));
#295945=CARTESIAN_POINT('Ctrl Pts',(3.75838203887364,127.6249999995,-11.5671105274568));
#295946=CARTESIAN_POINT('Ctrl Pts',(-8.68466972990837E-14,127.774999999499,
-12.7882828778549));
#295947=CARTESIAN_POINT('Ctrl Pts',(-3.75838203887381,127.924999999498,
-11.5671105274568));
#295948=CARTESIAN_POINT('Ctrl Pts',(-7.51676407774754,128.074999999498,
-10.3459381770588));
#295949=CARTESIAN_POINT('Ctrl Pts',(-9.83957192047864,128.224999999497,
-7.14886745759505));
#295950=CARTESIAN_POINT('Ctrl Pts',(-12.1623797632097,128.374999999497,
-3.95179673813132));
#295951=CARTESIAN_POINT('Ctrl Pts',(-12.1623797632097,128.524999999496,
2.97892388940585E-15));
#295952=CARTESIAN_POINT('Ctrl Pts',(-12.1623797632097,128.674999999495,
3.95179673813133));
#295953=CARTESIAN_POINT('Ctrl Pts',(-9.83957192047864,128.824999999495,
7.14886745759505));
#295954=CARTESIAN_POINT('Ctrl Pts',(-7.51676407774754,128.974999999494,
10.3459381770588));
#295955=CARTESIAN_POINT('Ctrl Pts',(-3.75838203887381,129.124999999494,
11.5671105274568));
#295956=CARTESIAN_POINT('Ctrl Pts',(-8.45783259963234E-14,129.274999999493,
12.7882828778549));
#295957=CARTESIAN_POINT('Ctrl Pts',(3.75838203887364,129.424999999492,11.5671105274568));
#295958=CARTESIAN_POINT('Ctrl Pts',(7.51676407774737,129.574999999492,10.3459381770588));
#295959=CARTESIAN_POINT('Ctrl Pts',(9.83957192047846,129.724999999491,7.14886745759505));
#295960=CARTESIAN_POINT('Ctrl Pts',(12.1623797632096,129.874999999491,3.95179673813132));
#295961=CARTESIAN_POINT('Ctrl Pts',(12.1623797632096,130.02499999949,-1.48946194470292E-15));
#295962=CARTESIAN_POINT('Ctrl Pts',(12.1623797632096,130.174999999489,-3.95179673813132));
#295963=CARTESIAN_POINT('Ctrl Pts',(9.83957192047846,130.324999999489,-7.14886745759505));
#295964=CARTESIAN_POINT('Ctrl Pts',(7.51676407774737,130.474999999488,-10.3459381770588));
#295965=CARTESIAN_POINT('Ctrl Pts',(3.75838203887364,130.624999999488,-11.5671105274568));
#295966=CARTESIAN_POINT('Ctrl Pts',(-8.85744065707455E-14,130.774999999487,
-12.7882828778549));
#295967=CARTESIAN_POINT('Ctrl Pts',(-3.75838203887382,130.924999999486,
-11.5671105274568));
#295968=CARTESIAN_POINT('Ctrl Pts',(-7.51676407774754,131.074999999486,
-10.3459381770588));
#295969=CARTESIAN_POINT('Ctrl Pts',(-9.83957192047864,131.224999999485,
-7.14886745759505));
#295970=CARTESIAN_POINT('Ctrl Pts',(-12.1623797632097,131.374999999485,
-3.95179673813132));
#295971=CARTESIAN_POINT('Ctrl Pts',(-12.1623797632097,131.524999999484,
2.97892388940585E-15));
#295972=CARTESIAN_POINT('Ctrl Pts',(-12.1623797632097,131.674999999483,
3.95179673813133));
#295973=CARTESIAN_POINT('Ctrl Pts',(-9.83957192047864,131.824999999483,
7.14886745759505));
#295974=CARTESIAN_POINT('Ctrl Pts',(-7.51676407774754,131.974999999482,
10.3459381770588));
#295975=CARTESIAN_POINT('Ctrl Pts',(-3.75838203887381,132.124999999482,
11.5671105274568));
#295976=CARTESIAN_POINT('Ctrl Pts',(-8.63060352679853E-14,132.274999999481,
12.7882828778549));
#295977=CARTESIAN_POINT('Ctrl Pts',(3.75838203887364,132.42499999948,11.5671105274568));
#295978=CARTESIAN_POINT('Ctrl Pts',(7.51676407774737,132.57499999948,10.3459381770588));
#295979=CARTESIAN_POINT('Ctrl Pts',(9.83957192047846,132.724999999479,7.14886745759505));
#295980=CARTESIAN_POINT('Ctrl Pts',(12.1623797632096,132.874999999479,3.95179673813132));
#295981=CARTESIAN_POINT('Ctrl Pts',(12.1623797632096,133.024999999478,-1.48946194470292E-15));
#295982=CARTESIAN_POINT('Ctrl Pts',(12.1623797632096,133.174999999477,-3.95179673813132));
#295983=CARTESIAN_POINT('Ctrl Pts',(9.83957192047846,133.324999999477,-7.14886745759505));
#295984=CARTESIAN_POINT('Ctrl Pts',(7.51676407774736,133.474999999476,-10.3459381770588));
#295985=CARTESIAN_POINT('Ctrl Pts',(3.75838203887364,133.624999999476,-11.5671105274568));
#295986=CARTESIAN_POINT('Ctrl Pts',(-9.03021158424074E-14,133.774999999475,
-12.7882828778549));
#295987=CARTESIAN_POINT('Ctrl Pts',(-3.75838203887382,133.924999999474,
-11.5671105274568));
#295988=CARTESIAN_POINT('Ctrl Pts',(-7.51676407774755,134.074999999474,
-10.3459381770588));
#295989=CARTESIAN_POINT('Ctrl Pts',(-9.83957192047864,134.224999999473,
-7.14886745759505));
#295990=CARTESIAN_POINT('Ctrl Pts',(-12.1623797632097,134.374999999473,
-3.95179673813132));
#295991=CARTESIAN_POINT('Ctrl Pts',(-12.1623797632097,134.524999999472,
2.97892388940585E-15));
#295992=CARTESIAN_POINT('Ctrl Pts',(-12.1623797632097,134.674999999471,
3.95179673813133));
#295993=CARTESIAN_POINT('Ctrl Pts',(-9.83957192047864,134.824999999471,
7.14886745759505));
#295994=CARTESIAN_POINT('Ctrl Pts',(-7.51676407774754,134.97499999947,10.3459381770588));
#295995=CARTESIAN_POINT('Ctrl Pts',(-3.75838203887382,135.12499999947,11.5671105274568));
#295996=CARTESIAN_POINT('Ctrl Pts',(-8.80337445396471E-14,135.274999999469,
12.7882828778549));
#295997=CARTESIAN_POINT('Ctrl Pts',(3.75838203887364,135.424999999468,11.5671105274568));
#295998=CARTESIAN_POINT('Ctrl Pts',(7.51676407774737,135.574999999468,10.3459381770588));
#295999=CARTESIAN_POINT('Ctrl Pts',(9.83957192047846,135.724999999467,7.14886745759505));
#296000=CARTESIAN_POINT('Ctrl Pts',(12.1623797632096,135.874999999467,3.95179673813132));
#296001=CARTESIAN_POINT('Ctrl Pts',(12.1623797632096,136.024999999466,-1.48946194470292E-15));
#296002=CARTESIAN_POINT('Ctrl Pts',(12.1623797632095,136.174999999465,-3.95179673813132));
#296003=CARTESIAN_POINT('Ctrl Pts',(9.83957192047846,136.324999999465,-7.14886745759505));
#296004=CARTESIAN_POINT('Ctrl Pts',(7.51676407774736,136.474999999464,-10.3459381770588));
#296005=CARTESIAN_POINT('Ctrl Pts',(3.75838203887364,136.624999999464,-11.5671105274568));
#296006=CARTESIAN_POINT('Ctrl Pts',(-9.20298251140692E-14,136.774999999463,
-12.7882828778549));
#296007=CARTESIAN_POINT('Ctrl Pts',(-3.75838203887382,136.924999999462,
-11.5671105274568));
#296008=CARTESIAN_POINT('Ctrl Pts',(-7.51676407774755,137.074999999462,
-10.3459381770588));
#296009=CARTESIAN_POINT('Ctrl Pts',(-9.83957192047864,137.224999999461,
-7.14886745759505));
#296010=CARTESIAN_POINT('Ctrl Pts',(-12.1623797632097,137.374999999461,
-3.95179673813132));
#296011=CARTESIAN_POINT('Ctrl Pts',(-12.1623797632097,137.52499999946,2.97892388940585E-15));
#296012=CARTESIAN_POINT('Ctrl Pts',(-12.1623797632097,137.674999999459,
3.95179673813133));
#296013=CARTESIAN_POINT('Ctrl Pts',(-9.83957192047864,137.824999999459,
7.14886745759505));
#296014=CARTESIAN_POINT('Ctrl Pts',(-7.51676407774755,137.974999999458,
10.3459381770588));
#296015=CARTESIAN_POINT('Ctrl Pts',(-3.75838203887382,138.124999999458,
11.5671105274568));
#296016=CARTESIAN_POINT('Ctrl Pts',(-8.97614538113089E-14,138.274999999457,
12.7882828778549));
#296017=CARTESIAN_POINT('Ctrl Pts',(3.75838203887364,138.424999999456,11.5671105274568));
#296018=CARTESIAN_POINT('Ctrl Pts',(7.51676407774736,138.574999999456,10.3459381770588));
#296019=CARTESIAN_POINT('Ctrl Pts',(9.83957192047846,138.724999999455,7.14886745759505));
#296020=CARTESIAN_POINT('Ctrl Pts',(12.1623797632096,138.874999999455,3.95179673813132));
#296021=CARTESIAN_POINT('Ctrl Pts',(12.1623797632096,139.024999999454,-1.48946194470292E-15));
#296022=CARTESIAN_POINT('Ctrl Pts',(12.1623797632095,139.174999999453,-3.95179673813132));
#296023=CARTESIAN_POINT('Ctrl Pts',(9.83957192047846,139.324999999453,-7.14886745759505));
#296024=CARTESIAN_POINT('Ctrl Pts',(7.51676407774736,139.474999999452,-10.3459381770588));
#296025=CARTESIAN_POINT('Ctrl Pts',(3.75838203887363,139.624999999452,-11.5671105274568));
#296026=CARTESIAN_POINT('Ctrl Pts',(-9.3757534385731E-14,139.774999999451,
-12.7882828778549));
#296027=CARTESIAN_POINT('Ctrl Pts',(-3.75838203887382,139.92499999945,-11.5671105274568));
#296028=CARTESIAN_POINT('Ctrl Pts',(-7.51676407774755,140.07499999945,-10.3459381770588));
#296029=CARTESIAN_POINT('Ctrl Pts',(-9.83957192047864,140.224999999449,
-7.14886745759505));
#296030=CARTESIAN_POINT('Ctrl Pts',(-12.1623797632097,140.374999999449,
-3.95179673813132));
#296031=CARTESIAN_POINT('Ctrl Pts',(-12.1623797632097,140.524999999448,
2.97892388940585E-15));
#296032=CARTESIAN_POINT('Ctrl Pts',(-12.1623797632097,140.674999999447,
3.95179673813133));
#296033=CARTESIAN_POINT('Ctrl Pts',(-9.83957192047864,140.824999999447,
7.14886745759505));
#296034=CARTESIAN_POINT('Ctrl Pts',(-7.51676407774755,140.974999999446,
10.3459381770588));
#296035=CARTESIAN_POINT('Ctrl Pts',(-3.75838203887382,141.124999999446,
11.5671105274568));
#296036=CARTESIAN_POINT('Ctrl Pts',(-9.14891630829708E-14,141.274999999445,
12.7882828778549));
#296037=CARTESIAN_POINT('Ctrl Pts',(3.75838203887364,141.424999999444,11.5671105274568));
#296038=CARTESIAN_POINT('Ctrl Pts',(7.51676407774736,141.574999999444,10.3459381770588));
#296039=CARTESIAN_POINT('Ctrl Pts',(9.83957192047845,141.724999999443,7.14886745759505));
#296040=CARTESIAN_POINT('Ctrl Pts',(12.1623797632095,141.874999999443,3.95179673813132));
#296041=CARTESIAN_POINT('Ctrl Pts',(12.1623797632095,142.024999999442,-1.48946194470292E-15));
#296042=CARTESIAN_POINT('Ctrl Pts',(12.1623797632095,142.174999999441,-3.95179673813132));
#296043=CARTESIAN_POINT('Ctrl Pts',(9.83957192047845,142.324999999441,-7.14886745759505));
#296044=CARTESIAN_POINT('Ctrl Pts',(7.51676407774736,142.47499999944,-10.3459381770588));
#296045=CARTESIAN_POINT('Ctrl Pts',(3.75838203887363,142.62499999944,-11.5671105274568));
#296046=CARTESIAN_POINT('Ctrl Pts',(-9.54852436573929E-14,142.774999999439,
-12.7882828778549));
#296047=CARTESIAN_POINT('Ctrl Pts',(-3.75838203887382,142.924999999438,
-11.5671105274568));
#296048=CARTESIAN_POINT('Ctrl Pts',(-7.51676407774755,143.074999999438,
-10.3459381770588));
#296049=CARTESIAN_POINT('Ctrl Pts',(-9.83957192047864,143.224999999437,
-7.14886745759505));
#296050=CARTESIAN_POINT('Ctrl Pts',(-12.1623797632097,143.374999999437,
-3.95179673813132));
#296051=CARTESIAN_POINT('Ctrl Pts',(-12.1623797632097,143.524999999436,
2.97892388940585E-15));
#296052=CARTESIAN_POINT('Ctrl Pts',(-12.1623797632097,143.674999999435,
3.95179673813133));
#296053=CARTESIAN_POINT('Ctrl Pts',(-9.83957192047864,143.824999999435,
7.14886745759505));
#296054=CARTESIAN_POINT('Ctrl Pts',(-7.51676407774755,143.974999999434,
10.3459381770588));
#296055=CARTESIAN_POINT('Ctrl Pts',(-3.75838203887382,144.124999999434,
11.5671105274568));
#296056=CARTESIAN_POINT('Ctrl Pts',(-9.32168723546326E-14,144.274999999433,
12.7882828778549));
#296057=CARTESIAN_POINT('Ctrl Pts',(3.75838203887363,144.424999999432,11.5671105274568));
#296058=CARTESIAN_POINT('Ctrl Pts',(7.51676407774736,144.574999999432,10.3459381770588));
#296059=CARTESIAN_POINT('Ctrl Pts',(9.83957192047845,144.724999999431,7.14886745759505));
#296060=CARTESIAN_POINT('Ctrl Pts',(12.1623797632095,144.874999999431,3.95179673813132));
#296061=CARTESIAN_POINT('Ctrl Pts',(12.1623797632095,145.02499999943,-1.48946194470292E-15));
#296062=CARTESIAN_POINT('Ctrl Pts',(12.1623797632095,145.174999999429,-3.95179673813132));
#296063=CARTESIAN_POINT('Ctrl Pts',(9.83957192047845,145.324999999429,-7.14886745759505));
#296064=CARTESIAN_POINT('Ctrl Pts',(7.51676407774736,145.474999999428,-10.3459381770588));
#296065=CARTESIAN_POINT('Ctrl Pts',(3.75838203887363,145.624999999428,-11.5671105274568));
#296066=CARTESIAN_POINT('Ctrl Pts',(-9.72129529290547E-14,145.774999999427,
-12.7882828778549));
#296067=CARTESIAN_POINT('Ctrl Pts',(-3.75838203887382,145.924999999426,
-11.5671105274568));
#296068=CARTESIAN_POINT('Ctrl Pts',(-7.51676407774755,146.074999999426,
-10.3459381770588));
#296069=CARTESIAN_POINT('Ctrl Pts',(-9.83957192047865,146.224999999425,
-7.14886745759505));
#296070=CARTESIAN_POINT('Ctrl Pts',(-12.1623797632097,146.374999999425,
-3.95179673813132));
#296071=CARTESIAN_POINT('Ctrl Pts',(-12.1623797632097,146.524999999424,
2.97892388940585E-15));
#296072=CARTESIAN_POINT('Ctrl Pts',(-12.1623797632097,146.674999999423,
3.95179673813133));
#296073=CARTESIAN_POINT('Ctrl Pts',(-9.83957192047865,146.824999999423,
7.14886745759505));
#296074=CARTESIAN_POINT('Ctrl Pts',(-7.51676407774755,146.974999999422,
10.3459381770588));
#296075=CARTESIAN_POINT('Ctrl Pts',(-3.75838203887382,147.124999999422,
11.5671105274568));
#296076=CARTESIAN_POINT('Ctrl Pts',(-9.49445816262944E-14,147.274999999421,
12.7882828778549));
#296077=CARTESIAN_POINT('Ctrl Pts',(3.75838203887363,147.42499999942,11.5671105274568));
#296078=CARTESIAN_POINT('Ctrl Pts',(7.51676407774736,147.57499999942,10.3459381770588));
#296079=CARTESIAN_POINT('Ctrl Pts',(9.83957192047845,147.724999999419,7.14886745759505));
#296080=CARTESIAN_POINT('Ctrl Pts',(12.1623797632095,147.874999999419,3.95179673813132));
#296081=CARTESIAN_POINT('Ctrl Pts',(12.1623797632095,148.024999999418,-1.48946194470292E-15));
#296082=CARTESIAN_POINT('Ctrl Pts',(12.1623797632095,148.174999999417,-3.95179673813132));
#296083=CARTESIAN_POINT('Ctrl Pts',(9.83957192047845,148.324999999417,-7.14886745759505));
#296084=CARTESIAN_POINT('Ctrl Pts',(7.51676407774736,148.474999999416,-10.3459381770588));
#296085=CARTESIAN_POINT('Ctrl Pts',(3.75838203887363,148.624999999416,-11.5671105274568));
#296086=CARTESIAN_POINT('Ctrl Pts',(-9.89406622007166E-14,148.774999999415,
-12.7882828778549));
#296087=CARTESIAN_POINT('Ctrl Pts',(-3.75838203887383,148.924999999414,
-11.5671105274568));
#296088=CARTESIAN_POINT('Ctrl Pts',(-7.51676407774756,149.074999999414,
-10.3459381770588));
#296089=CARTESIAN_POINT('Ctrl Pts',(-9.83957192047865,149.224999999413,
-7.14886745759505));
#296090=CARTESIAN_POINT('Ctrl Pts',(-12.1623797632097,149.374999999413,
-3.95179673813132));
#296091=CARTESIAN_POINT('Ctrl Pts',(-12.1623797632097,149.524999999412,
2.97892388940585E-15));
#296092=CARTESIAN_POINT('Ctrl Pts',(-12.1623797632097,149.674999999411,
3.95179673813133));
#296093=CARTESIAN_POINT('Ctrl Pts',(-9.83957192047865,149.824999999411,
7.14886745759505));
#296094=CARTESIAN_POINT('Ctrl Pts',(-7.51676407774755,149.97499999941,10.3459381770588));
#296095=CARTESIAN_POINT('Ctrl Pts',(-3.75838203887382,150.12499999941,11.5671105274568));
#296096=CARTESIAN_POINT('Ctrl Pts',(-9.66722908979563E-14,150.274999999409,
12.7882828778549));
#296097=CARTESIAN_POINT('Ctrl Pts',(3.75838203887363,150.424999999408,11.5671105274568));
#296098=CARTESIAN_POINT('Ctrl Pts',(7.51676407774736,150.574999999408,10.3459381770588));
#296099=CARTESIAN_POINT('Ctrl Pts',(9.83957192047845,150.724999999407,7.14886745759505));
#296100=CARTESIAN_POINT('Ctrl Pts',(12.1623797632095,150.874999999407,3.95179673813132));
#296101=CARTESIAN_POINT('Ctrl Pts',(12.1623797632095,151.024999999406,-1.48946194470292E-15));
#296102=CARTESIAN_POINT('Ctrl Pts',(12.1623797632095,151.174999999405,-3.95179673813132));
#296103=CARTESIAN_POINT('Ctrl Pts',(9.83957192047845,151.324999999405,-7.14886745759505));
#296104=CARTESIAN_POINT('Ctrl Pts',(7.51676407774736,151.474999999404,-10.3459381770588));
#296105=CARTESIAN_POINT('Ctrl Pts',(3.75838203887363,151.624999999404,-11.5671105274568));
#296106=CARTESIAN_POINT('Ctrl Pts',(-1.00668371472378E-13,151.774999999403,
-12.7882828778549));
#296107=CARTESIAN_POINT('Ctrl Pts',(-3.75838203887383,151.924999999402,
-11.5671105274568));
#296108=CARTESIAN_POINT('Ctrl Pts',(-7.51676407774756,152.074999999402,
-10.3459381770588));
#296109=CARTESIAN_POINT('Ctrl Pts',(-9.83957192047865,152.224999999401,
-7.14886745759505));
#296110=CARTESIAN_POINT('Ctrl Pts',(-12.1623797632097,152.374999999401,
-3.95179673813132));
#296111=CARTESIAN_POINT('Ctrl Pts',(-12.1623797632097,152.5249999994,2.97892388940585E-15));
#296112=CARTESIAN_POINT('Ctrl Pts',(-12.1623797632097,152.674999999399,
3.95179673813133));
#296113=CARTESIAN_POINT('Ctrl Pts',(-9.83957192047865,152.824999999399,
7.14886745759505));
#296114=CARTESIAN_POINT('Ctrl Pts',(-7.51676407774756,152.974999999398,
10.3459381770588));
#296115=CARTESIAN_POINT('Ctrl Pts',(-3.75838203887383,153.124999999398,
11.5671105274568));
#296116=CARTESIAN_POINT('Ctrl Pts',(-9.84000001696181E-14,153.274999999397,
12.7882828778549));
#296117=CARTESIAN_POINT('Ctrl Pts',(3.75838203887363,153.424999999396,11.5671105274568));
#296118=CARTESIAN_POINT('Ctrl Pts',(7.51676407774736,153.574999999396,10.3459381770588));
#296119=CARTESIAN_POINT('Ctrl Pts',(9.83957192047845,153.724999999395,7.14886745759505));
#296120=CARTESIAN_POINT('Ctrl Pts',(12.1623797632095,153.874999999395,3.95179673813132));
#296121=CARTESIAN_POINT('Ctrl Pts',(12.1623797632095,154.024999999394,-1.48946194470292E-15));
#296122=CARTESIAN_POINT('Ctrl Pts',(12.1623797632095,154.174999999393,-3.95179673813132));
#296123=CARTESIAN_POINT('Ctrl Pts',(9.83957192047845,154.324999999393,-7.14886745759505));
#296124=CARTESIAN_POINT('Ctrl Pts',(7.51676407774735,154.474999999392,-10.3459381770588));
#296125=CARTESIAN_POINT('Ctrl Pts',(3.75838203887363,154.624999999392,-11.5671105274568));
#296126=CARTESIAN_POINT('Ctrl Pts',(-1.0239608074404E-13,154.774999999391,
-12.7882828778549));
#296127=CARTESIAN_POINT('Ctrl Pts',(-3.75838203887383,154.92499999939,-11.5671105274568));
#296128=CARTESIAN_POINT('Ctrl Pts',(-9.73188510064477,91.186,-2.51434197826682));
#296129=CARTESIAN_POINT('Ctrl Pts',(-9.60478494878794,91.186,-3.25683227280792));
#296130=CARTESIAN_POINT('Ctrl Pts',(-9.39476270715683,91.186,-3.98267472639531));
#296131=CARTESIAN_POINT('Ctrl Pts',(-8.80110729028426,91.186,-5.41178772721597));
#296132=CARTESIAN_POINT('Ctrl Pts',(-8.4113556697725,91.186,-6.10153554674208));
#296133=CARTESIAN_POINT('Ctrl Pts',(-7.1594638773909,91.186,-7.83754033530839));
#296134=CARTESIAN_POINT('Ctrl Pts',(-6.16336234352202,91.1859999986483,
-8.77422666970583));
#296135=CARTESIAN_POINT('Ctrl Pts',(-3.45643278380831,91.1859999986483,
-10.4839899487996));
#296136=CARTESIAN_POINT('Ctrl Pts',(-1.95983265628982,91.186,-10.8625608372954));
#296137=CARTESIAN_POINT('Ctrl Pts',(0.487656647838607,91.186,-11.266528763347));
#296138=CARTESIAN_POINT('Ctrl Pts',(1.98204486733221,91.186,-11.2131410528978));
#296139=CARTESIAN_POINT('Ctrl Pts',(4.44770027945387,91.186,-10.6233745503084));
#296140=CARTESIAN_POINT('Ctrl Pts',(5.84635722463119,91.186,-10.1391958336611));
#296141=CARTESIAN_POINT('Ctrl Pts',(8.49239651382177,91.186,-8.32644545870485));
#296142=CARTESIAN_POINT('Ctrl Pts',(9.52161704638934,91.186,-7.28514894739878));
#296143=CARTESIAN_POINT('Ctrl Pts',(10.3435570531184,91.186,-6.08365247930268));
#296144=CARTESIAN_POINT('Ctrl Pts',(10.0514428414941,128.806249999495,-1.23094673026484E-15));
#296145=CARTESIAN_POINT('Ctrl Pts',(10.0514428414941,128.956249999495,-3.26591175476071));
#296146=CARTESIAN_POINT('Ctrl Pts',(8.1317880767571,129.106249999494,-5.90808986649102));
#296147=CARTESIAN_POINT('Ctrl Pts',(6.21213331202013,129.256249999493,-8.55026797822134));
#296148=CARTESIAN_POINT('Ctrl Pts',(3.10606665601002,129.406249999493,-9.5594902125713));
#296149=CARTESIAN_POINT('Ctrl Pts',(-8.77366151879469E-14,129.556249999492,
-10.5687124469213));
#296150=CARTESIAN_POINT('Ctrl Pts',(-3.1060666560102,129.706249999492,-9.5594902125713));
#296151=CARTESIAN_POINT('Ctrl Pts',(-6.2121333120203,129.856249999491,-8.55026797822134));
#296152=CARTESIAN_POINT('Ctrl Pts',(-8.13178807675728,130.00624999949,-5.90808986649102));
#296153=CARTESIAN_POINT('Ctrl Pts',(-10.0514428414943,130.15624999949,-3.2659117547607));
#296154=CARTESIAN_POINT('Ctrl Pts',(-10.0514428414943,130.306249999489,
2.46189346052968E-15));
#296155=CARTESIAN_POINT('Ctrl Pts',(-10.0514428414943,130.456249999489,
3.26591175476071));
#296156=CARTESIAN_POINT('Ctrl Pts',(-8.13178807675728,130.606249999488,
5.90808986649102));
#296157=CARTESIAN_POINT('Ctrl Pts',(-6.80976210866172,130.709551852955,
7.72770250737114));
#296158=CARTESIAN_POINT('Ctrl Pts',(-4.83831102398129,130.817307158506,
8.81034900733485));
#296159=CARTESIAN_POINT('Ctrl Pts',(-12.1623797632103,-3.28749999997638,
2.97892388940601E-15));
#296160=CARTESIAN_POINT('Ctrl Pts',(-12.1623797632103,-3.13749999997698,
3.95179673813154));
#296161=CARTESIAN_POINT('Ctrl Pts',(-9.83957192047908,-2.98749999997758,
7.14886745759543));
#296162=CARTESIAN_POINT('Ctrl Pts',(-7.51676407774787,-2.83749999997817,
10.3459381770593));
#296163=CARTESIAN_POINT('Ctrl Pts',(-3.75838203887394,-2.68749999997877,
11.5671105274575));
#296164=CARTESIAN_POINT('Ctrl Pts',(-8.66709987268145E-15,-2.53749999997937,
12.7882828778556));
#296165=CARTESIAN_POINT('Ctrl Pts',(3.75838203887392,-2.38749999997997,
11.5671105274575));
#296166=CARTESIAN_POINT('Ctrl Pts',(7.51676407774785,-2.23749999998057,
10.3459381770593));
#296167=CARTESIAN_POINT('Ctrl Pts',(9.83957192047906,-2.08749999998117,
7.14886745759543));
#296168=CARTESIAN_POINT('Ctrl Pts',(12.1623797632103,-1.93749999998176,
3.95179673813153));
#296169=CARTESIAN_POINT('Ctrl Pts',(12.1623797632103,-1.78749999998236,
-1.489461944703E-15));
#296170=CARTESIAN_POINT('Ctrl Pts',(12.1623797632103,-1.63749999998296,
-3.95179673813154));
#296171=CARTESIAN_POINT('Ctrl Pts',(9.83957192047906,-1.48749999998357,
-7.14886745759543));
#296172=CARTESIAN_POINT('Ctrl Pts',(7.51676407774784,-1.33749999998417,
-10.3459381770593));
#296173=CARTESIAN_POINT('Ctrl Pts',(3.75838203887392,-1.18749999998477,
-11.5671105274575));
#296174=CARTESIAN_POINT('Ctrl Pts',(-1.26631804471037E-14,-1.03749999998537,
-12.7882828778556));
#296175=CARTESIAN_POINT('Ctrl Pts',(-3.75838203887394,-0.887499999985973,
-11.5671105274575));
#296176=CARTESIAN_POINT('Ctrl Pts',(-7.51676407774787,-0.737499999986575,
-10.3459381770593));
#296177=CARTESIAN_POINT('Ctrl Pts',(-9.83957192047909,-0.587499999987176,
-7.14886745759543));
#296178=CARTESIAN_POINT('Ctrl Pts',(-12.1623797632103,-0.437499999987778,
-3.95179673813153));
#296179=CARTESIAN_POINT('Ctrl Pts',(-12.1623797632103,-0.287499999988378,
2.97892388940601E-15));
#296180=CARTESIAN_POINT('Ctrl Pts',(-12.1623797632103,-0.137499999988978,
3.95179673813154));
#296181=CARTESIAN_POINT('Ctrl Pts',(-9.83957192047909,0.0125000000104236,
7.14886745759543));
#296182=CARTESIAN_POINT('Ctrl Pts',(-7.51676407774787,0.162500000009825,
10.3459381770593));
#296183=CARTESIAN_POINT('Ctrl Pts',(-3.75838203887394,0.312500000009227,
11.5671105274575));
#296184=CARTESIAN_POINT('Ctrl Pts',(-1.03948091443433E-14,0.462500000008629,
12.7882828778556));
#296185=CARTESIAN_POINT('Ctrl Pts',(3.75838203887392,0.612500000008031,
11.5671105274575));
#296186=CARTESIAN_POINT('Ctrl Pts',(7.51676407774785,0.762500000007433,
10.3459381770593));
#296187=CARTESIAN_POINT('Ctrl Pts',(9.83957192047906,0.912500000006835,
7.14886745759543));
#296188=CARTESIAN_POINT('Ctrl Pts',(12.1623797632103,1.06250000000624,3.95179673813153));
#296189=CARTESIAN_POINT('Ctrl Pts',(12.1623797632103,1.21250000000564,-1.489461944703E-15));
#296190=CARTESIAN_POINT('Ctrl Pts',(12.1623797632103,1.36250000000504,-3.95179673813154));
#296191=CARTESIAN_POINT('Ctrl Pts',(9.83957192047906,1.51250000000444,-7.14886745759543));
#296192=CARTESIAN_POINT('Ctrl Pts',(7.51676407774784,1.66250000000383,-10.3459381770593));
#296193=CARTESIAN_POINT('Ctrl Pts',(3.75838203887391,1.81250000000323,-11.5671105274575));
#296194=CARTESIAN_POINT('Ctrl Pts',(-1.43908897187656E-14,1.96250000000263,
-12.7882828778556));
#296195=CARTESIAN_POINT('Ctrl Pts',(-3.75838203887394,2.11250000000203,
-11.5671105274575));
#296196=CARTESIAN_POINT('Ctrl Pts',(-7.51676407774787,2.26250000000143,
-10.3459381770593));
#296197=CARTESIAN_POINT('Ctrl Pts',(-9.83957192047909,2.41250000000082,
-7.14886745759543));
#296198=CARTESIAN_POINT('Ctrl Pts',(-12.1623797632103,2.56250000000022,
-3.95179673813153));
#296199=CARTESIAN_POINT('Ctrl Pts',(-12.1623797632103,2.71249999999962,
2.97892388940601E-15));
#296200=CARTESIAN_POINT('Ctrl Pts',(-12.1623797632103,2.86249999999902,
3.95179673813154));
#296201=CARTESIAN_POINT('Ctrl Pts',(-9.83957192047909,3.01249999999842,
7.14886745759543));
#296202=CARTESIAN_POINT('Ctrl Pts',(-7.51676407774787,3.16249999999782,
10.3459381770593));
#296203=CARTESIAN_POINT('Ctrl Pts',(-3.75838203887394,3.31249999999723,
11.5671105274575));
#296204=CARTESIAN_POINT('Ctrl Pts',(-1.21225184160051E-14,3.46249999999663,
12.7882828778556));
#296205=CARTESIAN_POINT('Ctrl Pts',(3.75838203887392,3.61249999999603,11.5671105274575));
#296206=CARTESIAN_POINT('Ctrl Pts',(7.51676407774784,3.76249999999543,10.3459381770593));
#296207=CARTESIAN_POINT('Ctrl Pts',(9.83957192047906,3.91249999999483,7.14886745759543));
#296208=CARTESIAN_POINT('Ctrl Pts',(12.1623797632103,4.06249999999424,3.95179673813153));
#296209=CARTESIAN_POINT('Ctrl Pts',(12.1623797632103,4.21249999999364,-1.489461944703E-15));
#296210=CARTESIAN_POINT('Ctrl Pts',(12.1623797632103,4.36249999999303,-3.95179673813154));
#296211=CARTESIAN_POINT('Ctrl Pts',(9.83957192047906,4.51249999999243,-7.14886745759543));
#296212=CARTESIAN_POINT('Ctrl Pts',(7.51676407774784,4.66249999999183,-10.3459381770593));
#296213=CARTESIAN_POINT('Ctrl Pts',(3.75838203887391,4.81249999999123,-11.5671105274575));
#296214=CARTESIAN_POINT('Ctrl Pts',(-1.61185989904274E-14,4.96249999999063,
-12.7882828778556));
#296215=CARTESIAN_POINT('Ctrl Pts',(-3.75838203887394,5.11249999999003,
-11.5671105274575));
#296216=CARTESIAN_POINT('Ctrl Pts',(-7.51676407774788,5.26249999998942,
-10.3459381770593));
#296217=CARTESIAN_POINT('Ctrl Pts',(-9.83957192047909,5.41249999998882,
-7.14886745759543));
#296218=CARTESIAN_POINT('Ctrl Pts',(-12.1623797632103,5.56249999998822,
-3.95179673813153));
#296219=CARTESIAN_POINT('Ctrl Pts',(-12.1623797632103,5.71249999998762,
2.97892388940601E-15));
#296220=CARTESIAN_POINT('Ctrl Pts',(-12.1623797632103,5.86249999998702,
3.95179673813154));
#296221=CARTESIAN_POINT('Ctrl Pts',(-9.83957192047909,6.01249999998642,
7.14886745759543));
#296222=CARTESIAN_POINT('Ctrl Pts',(-7.51676407774787,6.16249999998582,
10.3459381770593));
#296223=CARTESIAN_POINT('Ctrl Pts',(-3.75838203887394,6.31249999998523,
11.5671105274575));
#296224=CARTESIAN_POINT('Ctrl Pts',(-1.3850227687667E-14,6.46249999998463,
12.7882828778556));
#296225=CARTESIAN_POINT('Ctrl Pts',(3.75838203887392,6.61249999998403,11.5671105274575));
#296226=CARTESIAN_POINT('Ctrl Pts',(7.51676407774784,6.76249999998343,10.3459381770593));
#296227=CARTESIAN_POINT('Ctrl Pts',(9.83957192047906,6.91249999998283,7.14886745759543));
#296228=CARTESIAN_POINT('Ctrl Pts',(12.1623797632103,7.06249999998224,3.95179673813153));
#296229=CARTESIAN_POINT('Ctrl Pts',(12.1623797632103,7.21249999998164,-1.489461944703E-15));
#296230=CARTESIAN_POINT('Ctrl Pts',(12.1623797632103,7.36249999998104,-3.95179673813154));
#296231=CARTESIAN_POINT('Ctrl Pts',(9.83957192047906,7.51249999998044,-7.14886745759543));
#296232=CARTESIAN_POINT('Ctrl Pts',(7.51676407774784,7.66249999997983,-10.3459381770593));
#296233=CARTESIAN_POINT('Ctrl Pts',(3.75838203887391,7.81249999997923,-11.5671105274575));
#296234=CARTESIAN_POINT('Ctrl Pts',(-1.78463082620892E-14,7.96249999997863,
-12.7882828778556));
#296235=CARTESIAN_POINT('Ctrl Pts',(-3.75838203887395,8.11249999997803,
-11.5671105274575));
#296236=CARTESIAN_POINT('Ctrl Pts',(-7.51676407774788,8.26249999997743,
-10.3459381770593));
#296237=CARTESIAN_POINT('Ctrl Pts',(-9.83957192047909,8.41249999997682,
-7.14886745759543));
#296238=CARTESIAN_POINT('Ctrl Pts',(-12.1623797632103,8.56249999997622,
-3.95179673813153));
#296239=CARTESIAN_POINT('Ctrl Pts',(-12.1623797632103,8.71249999997562,
2.97892388940601E-15));
#296240=CARTESIAN_POINT('Ctrl Pts',(-12.1623797632103,8.86249999997502,
3.95179673813154));
#296241=CARTESIAN_POINT('Ctrl Pts',(-9.83957192047909,9.01249999997442,
7.14886745759543));
#296242=CARTESIAN_POINT('Ctrl Pts',(-7.51676407774787,9.16249999997382,
10.3459381770593));
#296243=CARTESIAN_POINT('Ctrl Pts',(-3.75838203887394,9.31249999997323,
11.5671105274575));
#296244=CARTESIAN_POINT('Ctrl Pts',(-1.55779369593288E-14,9.46249999997263,
12.7882828778556));
#296245=CARTESIAN_POINT('Ctrl Pts',(3.75838203887391,9.61249999997203,11.5671105274575));
#296246=CARTESIAN_POINT('Ctrl Pts',(7.51676407774784,9.76249999997144,10.3459381770593));
#296247=CARTESIAN_POINT('Ctrl Pts',(9.83957192047906,9.91249999997084,7.14886745759543));
#296248=CARTESIAN_POINT('Ctrl Pts',(12.1623797632103,10.0624999999702,3.95179673813153));
#296249=CARTESIAN_POINT('Ctrl Pts',(12.1623797632103,10.2124999999696,-1.489461944703E-15));
#296250=CARTESIAN_POINT('Ctrl Pts',(12.1623797632103,10.362499999969,-3.95179673813154));
#296251=CARTESIAN_POINT('Ctrl Pts',(9.83957192047905,10.5124999999684,-7.14886745759543));
#296252=CARTESIAN_POINT('Ctrl Pts',(7.51676407774784,10.6624999999678,-10.3459381770593));
#296253=CARTESIAN_POINT('Ctrl Pts',(3.75838203887391,10.8124999999672,-11.5671105274575));
#296254=CARTESIAN_POINT('Ctrl Pts',(-1.95740175337511E-14,10.9624999999666,
-12.7882828778556));
#296255=CARTESIAN_POINT('Ctrl Pts',(-3.75838203887395,11.112499999966,-11.5671105274575));
#296256=CARTESIAN_POINT('Ctrl Pts',(-7.51676407774788,11.2624999999654,
-10.3459381770593));
#296257=CARTESIAN_POINT('Ctrl Pts',(-9.83957192047909,11.4124999999648,
-7.14886745759543));
#296258=CARTESIAN_POINT('Ctrl Pts',(-12.1623797632103,11.5624999999642,
-3.95179673813153));
#296259=CARTESIAN_POINT('Ctrl Pts',(-12.1623797632103,11.7124999999636,
2.97892388940601E-15));
#296260=CARTESIAN_POINT('Ctrl Pts',(-12.1623797632103,11.862499999963,3.95179673813154));
#296261=CARTESIAN_POINT('Ctrl Pts',(-9.83957192047909,12.0124999999624,
7.14886745759543));
#296262=CARTESIAN_POINT('Ctrl Pts',(-7.51676407774788,12.1624999999618,
10.3459381770593));
#296263=CARTESIAN_POINT('Ctrl Pts',(-3.75838203887395,12.3124999999612,
11.5671105274575));
#296264=CARTESIAN_POINT('Ctrl Pts',(-1.73056462309906E-14,12.4624999999606,
12.7882828778556));
#296265=CARTESIAN_POINT('Ctrl Pts',(3.75838203887391,12.61249999996,11.5671105274575));
#296266=CARTESIAN_POINT('Ctrl Pts',(7.51676407774784,12.7624999999594,10.3459381770593));
#296267=CARTESIAN_POINT('Ctrl Pts',(9.83957192047906,12.9124999999588,7.14886745759543));
#296268=CARTESIAN_POINT('Ctrl Pts',(12.1623797632103,13.0624999999582,3.95179673813153));
#296269=CARTESIAN_POINT('Ctrl Pts',(12.1623797632103,13.2124999999576,-1.489461944703E-15));
#296270=CARTESIAN_POINT('Ctrl Pts',(12.1623797632103,13.362499999957,-3.95179673813154));
#296271=CARTESIAN_POINT('Ctrl Pts',(9.83957192047905,13.5124999999564,-7.14886745759543));
#296272=CARTESIAN_POINT('Ctrl Pts',(7.51676407774784,13.6624999999558,-10.3459381770593));
#296273=CARTESIAN_POINT('Ctrl Pts',(3.75838203887391,13.8124999999552,-11.5671105274575));
#296274=CARTESIAN_POINT('Ctrl Pts',(-2.13017268054129E-14,13.9624999999546,
-12.7882828778556));
#296275=CARTESIAN_POINT('Ctrl Pts',(-3.75838203887395,14.112499999954,-11.5671105274575));
#296276=CARTESIAN_POINT('Ctrl Pts',(-7.51676407774788,14.2624999999534,
-10.3459381770593));
#296277=CARTESIAN_POINT('Ctrl Pts',(-9.8395719204791,14.4124999999528,-7.14886745759543));
#296278=CARTESIAN_POINT('Ctrl Pts',(-12.1623797632103,14.5624999999522,
-3.95179673813153));
#296279=CARTESIAN_POINT('Ctrl Pts',(-12.1623797632103,14.7124999999516,
2.97892388940601E-15));
#296280=CARTESIAN_POINT('Ctrl Pts',(-12.1623797632103,14.862499999951,3.95179673813154));
#296281=CARTESIAN_POINT('Ctrl Pts',(-9.83957192047909,15.0124999999504,
7.14886745759543));
#296282=CARTESIAN_POINT('Ctrl Pts',(-7.51676407774788,15.1624999999498,
10.3459381770593));
#296283=CARTESIAN_POINT('Ctrl Pts',(-3.75838203887395,15.3124999999492,
11.5671105274575));
#296284=CARTESIAN_POINT('Ctrl Pts',(-1.90333555026525E-14,15.4624999999486,
12.7882828778556));
#296285=CARTESIAN_POINT('Ctrl Pts',(3.75838203887391,15.612499999948,11.5671105274575));
#296286=CARTESIAN_POINT('Ctrl Pts',(7.51676407774784,15.7624999999474,10.3459381770593));
#296287=CARTESIAN_POINT('Ctrl Pts',(9.83957192047905,15.9124999999468,7.14886745759543));
#296288=CARTESIAN_POINT('Ctrl Pts',(12.1623797632103,16.0624999999462,3.95179673813153));
#296289=CARTESIAN_POINT('Ctrl Pts',(12.1623797632103,16.2124999999456,-1.489461944703E-15));
#296290=CARTESIAN_POINT('Ctrl Pts',(12.1623797632103,16.362499999945,-3.95179673813154));
#296291=CARTESIAN_POINT('Ctrl Pts',(9.83957192047905,16.5124999999444,-7.14886745759543));
#296292=CARTESIAN_POINT('Ctrl Pts',(7.51676407774784,16.6624999999438,-10.3459381770593));
#296293=CARTESIAN_POINT('Ctrl Pts',(3.75838203887391,16.8124999999432,-11.5671105274575));
#296294=CARTESIAN_POINT('Ctrl Pts',(-2.30294360770748E-14,16.9624999999426,
-12.7882828778556));
#296295=CARTESIAN_POINT('Ctrl Pts',(-3.75838203887395,17.112499999942,-11.5671105274575));
#296296=CARTESIAN_POINT('Ctrl Pts',(-7.51676407774788,17.2624999999414,
-10.3459381770593));
#296297=CARTESIAN_POINT('Ctrl Pts',(-9.8395719204791,17.4124999999408,-7.14886745759543));
#296298=CARTESIAN_POINT('Ctrl Pts',(-12.1623797632103,17.5624999999402,
-3.95179673813153));
#296299=CARTESIAN_POINT('Ctrl Pts',(-12.1623797632103,17.7124999999396,
2.97892388940601E-15));
#296300=CARTESIAN_POINT('Ctrl Pts',(-12.1623797632103,17.862499999939,3.95179673813154));
#296301=CARTESIAN_POINT('Ctrl Pts',(-9.8395719204791,18.0124999999384,7.14886745759543));
#296302=CARTESIAN_POINT('Ctrl Pts',(-7.51676407774788,18.1624999999378,
10.3459381770593));
#296303=CARTESIAN_POINT('Ctrl Pts',(-3.75838203887395,18.3124999999372,
11.5671105274575));
#296304=CARTESIAN_POINT('Ctrl Pts',(-2.07610647743143E-14,18.4624999999366,
12.7882828778556));
#296305=CARTESIAN_POINT('Ctrl Pts',(3.75838203887391,18.612499999936,11.5671105274575));
#296306=CARTESIAN_POINT('Ctrl Pts',(7.51676407774784,18.7624999999354,10.3459381770593));
#296307=CARTESIAN_POINT('Ctrl Pts',(9.83957192047905,18.9124999999348,7.14886745759543));
#296308=CARTESIAN_POINT('Ctrl Pts',(12.1623797632103,19.0624999999342,3.95179673813153));
#296309=CARTESIAN_POINT('Ctrl Pts',(12.1623797632103,19.2124999999336,-1.489461944703E-15));
#296310=CARTESIAN_POINT('Ctrl Pts',(12.1623797632103,19.362499999933,-3.95179673813154));
#296311=CARTESIAN_POINT('Ctrl Pts',(9.83957192047905,19.5124999999324,-7.14886745759543));
#296312=CARTESIAN_POINT('Ctrl Pts',(7.51676407774784,19.6624999999318,-10.3459381770593));
#296313=CARTESIAN_POINT('Ctrl Pts',(3.7583820388739,19.8124999999312,-11.5671105274575));
#296314=CARTESIAN_POINT('Ctrl Pts',(-2.47571453487366E-14,19.9624999999306,
-12.7882828778556));
#296315=CARTESIAN_POINT('Ctrl Pts',(-3.75838203887395,20.11249999993,-11.5671105274575));
#296316=CARTESIAN_POINT('Ctrl Pts',(-7.51676407774788,20.2624999999294,
-10.3459381770593));
#296317=CARTESIAN_POINT('Ctrl Pts',(-9.8395719204791,20.4124999999288,-7.14886745759543));
#296318=CARTESIAN_POINT('Ctrl Pts',(-12.1623797632103,20.5624999999282,
-3.95179673813153));
#296319=CARTESIAN_POINT('Ctrl Pts',(-12.1623797632103,20.7124999999276,
2.97892388940601E-15));
#296320=CARTESIAN_POINT('Ctrl Pts',(-12.1623797632103,20.862499999927,3.95179673813154));
#296321=CARTESIAN_POINT('Ctrl Pts',(-9.8395719204791,21.0124999999264,7.14886745759543));
#296322=CARTESIAN_POINT('Ctrl Pts',(-7.51676407774788,21.1624999999258,
10.3459381770593));
#296323=CARTESIAN_POINT('Ctrl Pts',(-3.75838203887395,21.3124999999252,
11.5671105274575));
#296324=CARTESIAN_POINT('Ctrl Pts',(-2.24887740459762E-14,21.4624999999246,
12.7882828778556));
#296325=CARTESIAN_POINT('Ctrl Pts',(3.75838203887391,21.612499999924,11.5671105274575));
#296326=CARTESIAN_POINT('Ctrl Pts',(7.51676407774784,21.7624999999234,10.3459381770593));
#296327=CARTESIAN_POINT('Ctrl Pts',(9.83957192047905,21.9124999999228,7.14886745759543));
#296328=CARTESIAN_POINT('Ctrl Pts',(12.1623797632103,22.0624999999222,3.95179673813153));
#296329=CARTESIAN_POINT('Ctrl Pts',(12.1623797632103,22.2124999999216,-1.489461944703E-15));
#296330=CARTESIAN_POINT('Ctrl Pts',(12.1623797632103,22.362499999921,-3.95179673813154));
#296331=CARTESIAN_POINT('Ctrl Pts',(9.83957192047905,22.5124999999204,-7.14886745759543));
#296332=CARTESIAN_POINT('Ctrl Pts',(7.51676407774783,22.6624999999198,-10.3459381770593));
#296333=CARTESIAN_POINT('Ctrl Pts',(3.7583820388739,22.8124999999192,-11.5671105274575));
#296334=CARTESIAN_POINT('Ctrl Pts',(-2.64848546203984E-14,22.9624999999186,
-12.7882828778556));
#296335=CARTESIAN_POINT('Ctrl Pts',(-3.75838203887396,23.112499999918,-11.5671105274575));
#296336=CARTESIAN_POINT('Ctrl Pts',(-7.51676407774788,23.2624999999174,
-10.3459381770593));
#296337=CARTESIAN_POINT('Ctrl Pts',(-9.8395719204791,23.4124999999168,-7.14886745759543));
#296338=CARTESIAN_POINT('Ctrl Pts',(-12.1623797632103,23.5624999999162,
-3.95179673813153));
#296339=CARTESIAN_POINT('Ctrl Pts',(-12.1623797632103,23.7124999999156,
2.97892388940601E-15));
#296340=CARTESIAN_POINT('Ctrl Pts',(-12.1623797632103,23.862499999915,3.95179673813154));
#296341=CARTESIAN_POINT('Ctrl Pts',(-9.8395719204791,24.0124999999144,7.14886745759543));
#296342=CARTESIAN_POINT('Ctrl Pts',(-7.51676407774788,24.1624999999138,
10.3459381770593));
#296343=CARTESIAN_POINT('Ctrl Pts',(-3.75838203887395,24.3124999999132,
11.5671105274575));
#296344=CARTESIAN_POINT('Ctrl Pts',(-2.4216483317638E-14,24.4624999999126,
12.7882828778556));
#296345=CARTESIAN_POINT('Ctrl Pts',(3.7583820388739,24.612499999912,11.5671105274575));
#296346=CARTESIAN_POINT('Ctrl Pts',(7.51676407774783,24.7624999999114,10.3459381770593));
#296347=CARTESIAN_POINT('Ctrl Pts',(9.83957192047905,24.9124999999108,7.14886745759543));
#296348=CARTESIAN_POINT('Ctrl Pts',(12.1623797632103,25.0624999999102,3.95179673813153));
#296349=CARTESIAN_POINT('Ctrl Pts',(12.1623797632103,25.2124999999096,-1.489461944703E-15));
#296350=CARTESIAN_POINT('Ctrl Pts',(12.1623797632103,25.362499999909,-3.95179673813154));
#296351=CARTESIAN_POINT('Ctrl Pts',(9.83957192047905,25.5124999999084,-7.14886745759543));
#296352=CARTESIAN_POINT('Ctrl Pts',(7.51676407774783,25.6624999999078,-10.3459381770593));
#296353=CARTESIAN_POINT('Ctrl Pts',(3.7583820388739,25.8124999999072,-11.5671105274575));
#296354=CARTESIAN_POINT('Ctrl Pts',(-2.82125638920603E-14,25.9624999999066,
-12.7882828778556));
#296355=CARTESIAN_POINT('Ctrl Pts',(-3.75838203887396,26.112499999906,-11.5671105274575));
#296356=CARTESIAN_POINT('Ctrl Pts',(-7.51676407774788,26.2624999999054,
-10.3459381770593));
#296357=CARTESIAN_POINT('Ctrl Pts',(-9.8395719204791,26.4124999999048,-7.14886745759543));
#296358=CARTESIAN_POINT('Ctrl Pts',(-12.1623797632103,26.5624999999042,
-3.95179673813153));
#296359=CARTESIAN_POINT('Ctrl Pts',(-12.1623797632103,26.7124999999036,
2.97892388940601E-15));
#296360=CARTESIAN_POINT('Ctrl Pts',(-12.1623797632103,26.862499999903,3.95179673813154));
#296361=CARTESIAN_POINT('Ctrl Pts',(-9.8395719204791,27.0124999999024,7.14886745759543));
#296362=CARTESIAN_POINT('Ctrl Pts',(-7.51676407774788,27.1624999999018,
10.3459381770593));
#296363=CARTESIAN_POINT('Ctrl Pts',(-3.75838203887396,27.3124999999012,
11.5671105274575));
#296364=CARTESIAN_POINT('Ctrl Pts',(-2.59441925892998E-14,27.4624999999006,
12.7882828778556));
#296365=CARTESIAN_POINT('Ctrl Pts',(3.7583820388739,27.6124999999,11.5671105274575));
#296366=CARTESIAN_POINT('Ctrl Pts',(7.51676407774783,27.7624999998994,10.3459381770593));
#296367=CARTESIAN_POINT('Ctrl Pts',(9.83957192047905,27.9124999998988,7.14886745759543));
#296368=CARTESIAN_POINT('Ctrl Pts',(12.1623797632103,28.0624999998982,3.95179673813153));
#296369=CARTESIAN_POINT('Ctrl Pts',(12.1623797632103,28.2124999998976,-1.489461944703E-15));
#296370=CARTESIAN_POINT('Ctrl Pts',(12.1623797632103,28.362499999897,-3.95179673813154));
#296371=CARTESIAN_POINT('Ctrl Pts',(9.83957192047905,28.5124999998964,-7.14886745759543));
#296372=CARTESIAN_POINT('Ctrl Pts',(7.51676407774783,28.6624999998958,-10.3459381770593));
#296373=CARTESIAN_POINT('Ctrl Pts',(3.7583820388739,28.8124999998952,-11.5671105274575));
#296374=CARTESIAN_POINT('Ctrl Pts',(-2.99402731637221E-14,28.9624999998946,
-12.7882828778556));
#296375=CARTESIAN_POINT('Ctrl Pts',(-3.75838203887396,29.112499999894,-11.5671105274575));
#296376=CARTESIAN_POINT('Ctrl Pts',(-7.51676407774789,29.2624999998934,
-10.3459381770593));
#296377=CARTESIAN_POINT('Ctrl Pts',(-9.8395719204791,29.4124999998928,-7.14886745759543));
#296378=CARTESIAN_POINT('Ctrl Pts',(-12.1623797632103,29.5624999998922,
-3.95179673813153));
#296379=CARTESIAN_POINT('Ctrl Pts',(-12.1623797632103,29.7124999998916,
2.97892388940601E-15));
#296380=CARTESIAN_POINT('Ctrl Pts',(-12.1623797632103,29.862499999891,3.95179673813154));
#296381=CARTESIAN_POINT('Ctrl Pts',(-9.8395719204791,30.0124999998904,7.14886745759543));
#296382=CARTESIAN_POINT('Ctrl Pts',(-7.51676407774788,30.1624999998898,
10.3459381770593));
#296383=CARTESIAN_POINT('Ctrl Pts',(-3.75838203887396,30.3124999998892,
11.5671105274575));
#296384=CARTESIAN_POINT('Ctrl Pts',(-2.76719018609617E-14,30.4624999998886,
12.7882828778556));
#296385=CARTESIAN_POINT('Ctrl Pts',(3.7583820388739,30.612499999888,11.5671105274575));
#296386=CARTESIAN_POINT('Ctrl Pts',(7.51676407774783,30.7624999998874,10.3459381770593));
#296387=CARTESIAN_POINT('Ctrl Pts',(9.83957192047905,30.9124999998868,7.14886745759543));
#296388=CARTESIAN_POINT('Ctrl Pts',(12.1623797632103,31.0624999998862,3.95179673813153));
#296389=CARTESIAN_POINT('Ctrl Pts',(12.1623797632103,31.2124999998856,-1.489461944703E-15));
#296390=CARTESIAN_POINT('Ctrl Pts',(12.1623797632103,31.362499999885,-3.95179673813154));
#296391=CARTESIAN_POINT('Ctrl Pts',(9.83957192047904,31.5124999998844,-7.14886745759543));
#296392=CARTESIAN_POINT('Ctrl Pts',(7.51676407774783,31.6624999998838,-10.3459381770593));
#296393=CARTESIAN_POINT('Ctrl Pts',(3.7583820388739,31.8124999998832,-11.5671105274575));
#296394=CARTESIAN_POINT('Ctrl Pts',(-3.16679824353839E-14,31.9624999998826,
-12.7882828778556));
#296395=CARTESIAN_POINT('Ctrl Pts',(-3.75838203887396,32.112499999882,-11.5671105274575));
#296396=CARTESIAN_POINT('Ctrl Pts',(-7.51676407774789,32.2624999998814,
-10.3459381770593));
#296397=CARTESIAN_POINT('Ctrl Pts',(-9.83957192047911,32.4124999998808,
-7.14886745759543));
#296398=CARTESIAN_POINT('Ctrl Pts',(-12.1623797632103,32.5624999998802,
-3.95179673813153));
#296399=CARTESIAN_POINT('Ctrl Pts',(-12.1623797632103,32.7124999998796,
2.97892388940601E-15));
#296400=CARTESIAN_POINT('Ctrl Pts',(-12.1623797632103,32.862499999879,3.95179673813154));
#296401=CARTESIAN_POINT('Ctrl Pts',(-9.8395719204791,33.0124999998784,7.14886745759543));
#296402=CARTESIAN_POINT('Ctrl Pts',(-7.51676407774789,33.1624999998778,
10.3459381770593));
#296403=CARTESIAN_POINT('Ctrl Pts',(-3.75838203887396,33.3124999998772,
11.5671105274575));
#296404=CARTESIAN_POINT('Ctrl Pts',(-2.93996111326235E-14,33.4624999998766,
12.7882828778556));
#296405=CARTESIAN_POINT('Ctrl Pts',(3.7583820388739,33.612499999876,11.5671105274575));
#296406=CARTESIAN_POINT('Ctrl Pts',(7.51676407774783,33.7624999998754,10.3459381770593));
#296407=CARTESIAN_POINT('Ctrl Pts',(9.83957192047905,33.9124999998748,7.14886745759543));
#296408=CARTESIAN_POINT('Ctrl Pts',(12.1623797632103,34.0624999998742,3.95179673813153));
#296409=CARTESIAN_POINT('Ctrl Pts',(12.1623797632103,34.2124999998736,-1.489461944703E-15));
#296410=CARTESIAN_POINT('Ctrl Pts',(12.1623797632103,34.362499999873,-3.95179673813154));
#296411=CARTESIAN_POINT('Ctrl Pts',(9.83957192047904,34.5124999998724,-7.14886745759543));
#296412=CARTESIAN_POINT('Ctrl Pts',(7.51676407774783,34.6624999998718,-10.3459381770593));
#296413=CARTESIAN_POINT('Ctrl Pts',(3.7583820388739,34.8124999998712,-11.5671105274575));
#296414=CARTESIAN_POINT('Ctrl Pts',(-3.33956917070458E-14,34.9624999998706,
-12.7882828778556));
#296415=CARTESIAN_POINT('Ctrl Pts',(-3.75838203887396,35.11249999987,-11.5671105274575));
#296416=CARTESIAN_POINT('Ctrl Pts',(-7.51676407774789,35.2624999998694,
-10.3459381770593));
#296417=CARTESIAN_POINT('Ctrl Pts',(-9.83957192047911,35.4124999998688,
-7.14886745759543));
#296418=CARTESIAN_POINT('Ctrl Pts',(-12.1623797632103,35.5624999998682,
-3.95179673813153));
#296419=CARTESIAN_POINT('Ctrl Pts',(-12.1623797632103,35.7124999998676,
2.97892388940601E-15));
#296420=CARTESIAN_POINT('Ctrl Pts',(-12.1623797632103,35.862499999867,3.95179673813154));
#296421=CARTESIAN_POINT('Ctrl Pts',(-9.83957192047911,36.0124999998664,
7.14886745759543));
#296422=CARTESIAN_POINT('Ctrl Pts',(-7.51676407774789,36.1624999998658,
10.3459381770593));
#296423=CARTESIAN_POINT('Ctrl Pts',(-3.75838203887396,36.3124999998652,
11.5671105274575));
#296424=CARTESIAN_POINT('Ctrl Pts',(-3.11273204042854E-14,36.4624999998646,
12.7882828778556));
#296425=CARTESIAN_POINT('Ctrl Pts',(3.7583820388739,36.612499999864,11.5671105274575));
#296426=CARTESIAN_POINT('Ctrl Pts',(7.51676407774783,36.7624999998634,10.3459381770593));
#296427=CARTESIAN_POINT('Ctrl Pts',(9.83957192047904,36.9124999998628,7.14886745759543));
#296428=CARTESIAN_POINT('Ctrl Pts',(12.1623797632103,37.0624999998622,3.95179673813153));
#296429=CARTESIAN_POINT('Ctrl Pts',(12.1623797632103,37.2124999998616,-1.489461944703E-15));
#296430=CARTESIAN_POINT('Ctrl Pts',(12.1623797632103,37.362499999861,-3.95179673813154));
#296431=CARTESIAN_POINT('Ctrl Pts',(9.83957192047904,37.5124999998604,-7.14886745759543));
#296432=CARTESIAN_POINT('Ctrl Pts',(7.51676407774782,37.6624999998598,-10.3459381770593));
#296433=CARTESIAN_POINT('Ctrl Pts',(3.75838203887389,37.8124999998592,-11.5671105274575));
#296434=CARTESIAN_POINT('Ctrl Pts',(-3.51234009787076E-14,37.9624999998586,
-12.7882828778556));
#296435=CARTESIAN_POINT('Ctrl Pts',(-3.75838203887396,38.112499999858,-11.5671105274575));
#296436=CARTESIAN_POINT('Ctrl Pts',(-7.51676407774789,38.2624999998574,
-10.3459381770593));
#296437=CARTESIAN_POINT('Ctrl Pts',(-9.83957192047911,38.4124999998568,
-7.14886745759543));
#296438=CARTESIAN_POINT('Ctrl Pts',(-12.1623797632103,38.5624999998562,
-3.95179673813153));
#296439=CARTESIAN_POINT('Ctrl Pts',(-12.1623797632103,38.7124999998556,
2.97892388940601E-15));
#296440=CARTESIAN_POINT('Ctrl Pts',(-12.1623797632103,38.862499999855,3.95179673813154));
#296441=CARTESIAN_POINT('Ctrl Pts',(-9.83957192047911,39.0124999998544,
7.14886745759543));
#296442=CARTESIAN_POINT('Ctrl Pts',(-7.51676407774789,39.1624999998538,
10.3459381770593));
#296443=CARTESIAN_POINT('Ctrl Pts',(-3.75838203887396,39.3124999998532,
11.5671105274575));
#296444=CARTESIAN_POINT('Ctrl Pts',(-3.28550296759472E-14,39.4624999998526,
12.7882828778556));
#296445=CARTESIAN_POINT('Ctrl Pts',(3.7583820388739,39.612499999852,11.5671105274575));
#296446=CARTESIAN_POINT('Ctrl Pts',(7.51676407774782,39.7624999998514,10.3459381770593));
#296447=CARTESIAN_POINT('Ctrl Pts',(9.83957192047904,39.9124999998508,7.14886745759543));
#296448=CARTESIAN_POINT('Ctrl Pts',(12.1623797632103,40.0624999998502,3.95179673813153));
#296449=CARTESIAN_POINT('Ctrl Pts',(12.1623797632103,40.2124999998496,-1.489461944703E-15));
#296450=CARTESIAN_POINT('Ctrl Pts',(12.1623797632103,40.362499999849,-3.95179673813154));
#296451=CARTESIAN_POINT('Ctrl Pts',(9.83957192047904,40.5124999998484,-7.14886745759543));
#296452=CARTESIAN_POINT('Ctrl Pts',(7.51676407774782,40.6624999998478,-10.3459381770593));
#296453=CARTESIAN_POINT('Ctrl Pts',(3.75838203887389,40.8124999998472,-11.5671105274575));
#296454=CARTESIAN_POINT('Ctrl Pts',(-3.68511102503695E-14,40.9624999998466,
-12.7882828778556));
#296455=CARTESIAN_POINT('Ctrl Pts',(-3.75838203887397,41.112499999846,-11.5671105274575));
#296456=CARTESIAN_POINT('Ctrl Pts',(-7.51676407774789,41.2624999998454,
-10.3459381770593));
#296457=CARTESIAN_POINT('Ctrl Pts',(-9.83957192047911,41.4124999998448,
-7.14886745759543));
#296458=CARTESIAN_POINT('Ctrl Pts',(-12.1623797632103,41.5624999998442,
-3.95179673813153));
#296459=CARTESIAN_POINT('Ctrl Pts',(-12.1623797632103,41.7124999998436,
2.97892388940601E-15));
#296460=CARTESIAN_POINT('Ctrl Pts',(-12.1623797632103,41.862499999843,3.95179673813154));
#296461=CARTESIAN_POINT('Ctrl Pts',(-9.83957192047911,42.0124999998424,
7.14886745759543));
#296462=CARTESIAN_POINT('Ctrl Pts',(-7.51676407774789,42.1624999998418,
10.3459381770593));
#296463=CARTESIAN_POINT('Ctrl Pts',(-3.75838203887396,42.3124999998412,
11.5671105274575));
#296464=CARTESIAN_POINT('Ctrl Pts',(-3.4582738947609E-14,42.4624999998406,
12.7882828778556));
#296465=CARTESIAN_POINT('Ctrl Pts',(3.75838203887389,42.61249999984,11.5671105274575));
#296466=CARTESIAN_POINT('Ctrl Pts',(7.51676407774782,42.7624999998394,10.3459381770593));
#296467=CARTESIAN_POINT('Ctrl Pts',(9.83957192047904,42.9124999998388,7.14886745759543));
#296468=CARTESIAN_POINT('Ctrl Pts',(12.1623797632103,43.0624999998382,3.95179673813153));
#296469=CARTESIAN_POINT('Ctrl Pts',(12.1623797632103,43.2124999998376,-1.489461944703E-15));
#296470=CARTESIAN_POINT('Ctrl Pts',(12.1623797632103,43.362499999837,-3.95179673813154));
#296471=CARTESIAN_POINT('Ctrl Pts',(9.83957192047903,43.5124999998364,-7.14886745759543));
#296472=CARTESIAN_POINT('Ctrl Pts',(7.51676407774782,43.6624999998358,-10.3459381770593));
#296473=CARTESIAN_POINT('Ctrl Pts',(3.75838203887389,43.8124999998352,-11.5671105274575));
#296474=CARTESIAN_POINT('Ctrl Pts',(-3.85788195220313E-14,43.9624999998346,
-12.7882828778556));
#296475=CARTESIAN_POINT('Ctrl Pts',(-3.75838203887397,44.112499999834,-11.5671105274575));
#296476=CARTESIAN_POINT('Ctrl Pts',(-7.5167640777479,44.2624999998334,-10.3459381770593));
#296477=CARTESIAN_POINT('Ctrl Pts',(-9.83957192047911,44.4124999998328,
-7.14886745759543));
#296478=CARTESIAN_POINT('Ctrl Pts',(-12.1623797632103,44.5624999998322,
-3.95179673813153));
#296479=CARTESIAN_POINT('Ctrl Pts',(-12.1623797632103,44.7124999998316,
2.97892388940601E-15));
#296480=CARTESIAN_POINT('Ctrl Pts',(-12.1623797632103,44.862499999831,3.95179673813154));
#296481=CARTESIAN_POINT('Ctrl Pts',(-9.83957192047911,45.0124999998304,
7.14886745759543));
#296482=CARTESIAN_POINT('Ctrl Pts',(-7.51676407774789,45.1624999998298,
10.3459381770593));
#296483=CARTESIAN_POINT('Ctrl Pts',(-3.75838203887397,45.3124999998292,
11.5671105274575));
#296484=CARTESIAN_POINT('Ctrl Pts',(-3.63104482192709E-14,45.4624999998286,
12.7882828778556));
#296485=CARTESIAN_POINT('Ctrl Pts',(3.75838203887389,45.612499999828,11.5671105274575));
#296486=CARTESIAN_POINT('Ctrl Pts',(7.51676407774782,45.7624999998274,10.3459381770593));
#296487=CARTESIAN_POINT('Ctrl Pts',(9.83957192047904,45.9124999998268,7.14886745759543));
#296488=CARTESIAN_POINT('Ctrl Pts',(12.1623797632103,46.0624999998262,3.95179673813153));
#296489=CARTESIAN_POINT('Ctrl Pts',(12.1623797632103,46.2124999998256,-1.489461944703E-15));
#296490=CARTESIAN_POINT('Ctrl Pts',(12.1623797632103,46.362499999825,-3.95179673813154));
#296491=CARTESIAN_POINT('Ctrl Pts',(9.83957192047903,46.5124999998244,-7.14886745759543));
#296492=CARTESIAN_POINT('Ctrl Pts',(7.51676407774782,46.6624999998238,-10.3459381770593));
#296493=CARTESIAN_POINT('Ctrl Pts',(3.75838203887389,46.8124999998232,-11.5671105274575));
#296494=CARTESIAN_POINT('Ctrl Pts',(-4.03065287936931E-14,46.9624999998226,
-12.7882828778556));
#296495=CARTESIAN_POINT('Ctrl Pts',(-3.75838203887397,47.112499999822,-11.5671105274575));
#296496=CARTESIAN_POINT('Ctrl Pts',(-7.5167640777479,47.2624999998214,-10.3459381770593));
#296497=CARTESIAN_POINT('Ctrl Pts',(-9.83957192047912,47.4124999998208,
-7.14886745759543));
#296498=CARTESIAN_POINT('Ctrl Pts',(-12.1623797632103,47.5624999998202,
-3.95179673813153));
#296499=CARTESIAN_POINT('Ctrl Pts',(-12.1623797632103,47.7124999998196,
2.97892388940601E-15));
#296500=CARTESIAN_POINT('Ctrl Pts',(-12.1623797632103,47.862499999819,3.95179673813154));
#296501=CARTESIAN_POINT('Ctrl Pts',(-9.83957192047911,48.0124999998184,
7.14886745759543));
#296502=CARTESIAN_POINT('Ctrl Pts',(-7.51676407774789,48.1624999998178,
10.3459381770593));
#296503=CARTESIAN_POINT('Ctrl Pts',(-3.75838203887397,48.3124999998172,
11.5671105274575));
#296504=CARTESIAN_POINT('Ctrl Pts',(-3.80381574909327E-14,48.4624999998166,
12.7882828778556));
#296505=CARTESIAN_POINT('Ctrl Pts',(3.75838203887389,48.612499999816,11.5671105274575));
#296506=CARTESIAN_POINT('Ctrl Pts',(7.51676407774782,48.7624999998154,10.3459381770593));
#296507=CARTESIAN_POINT('Ctrl Pts',(9.83957192047903,48.9124999998148,7.14886745759543));
#296508=CARTESIAN_POINT('Ctrl Pts',(12.1623797632103,49.0624999998142,3.95179673813153));
#296509=CARTESIAN_POINT('Ctrl Pts',(12.1623797632103,49.2124999998136,-1.489461944703E-15));
#296510=CARTESIAN_POINT('Ctrl Pts',(12.1623797632103,49.362499999813,-3.95179673813154));
#296511=CARTESIAN_POINT('Ctrl Pts',(9.83957192047903,49.5124999998124,-7.14886745759543));
#296512=CARTESIAN_POINT('Ctrl Pts',(7.51676407774782,49.6624999998118,-10.3459381770593));
#296513=CARTESIAN_POINT('Ctrl Pts',(3.75838203887389,49.8124999998112,-11.5671105274575));
#296514=CARTESIAN_POINT('Ctrl Pts',(-4.2034238065355E-14,49.9624999998106,
-12.7882828778556));
#296515=CARTESIAN_POINT('Ctrl Pts',(-3.75838203887397,50.11249999981,-11.5671105274575));
#296516=CARTESIAN_POINT('Ctrl Pts',(-7.5167640777479,50.2624999998094,-10.3459381770593));
#296517=CARTESIAN_POINT('Ctrl Pts',(-9.83957192047912,50.4124999998088,
-7.14886745759543));
#296518=CARTESIAN_POINT('Ctrl Pts',(-12.1623797632103,50.5624999998082,
-3.95179673813153));
#296519=CARTESIAN_POINT('Ctrl Pts',(-12.1623797632103,50.7124999998076,
2.97892388940601E-15));
#296520=CARTESIAN_POINT('Ctrl Pts',(-12.1623797632103,50.862499999807,3.95179673813154));
#296521=CARTESIAN_POINT('Ctrl Pts',(-9.83957192047912,51.0124999998064,
7.14886745759543));
#296522=CARTESIAN_POINT('Ctrl Pts',(-7.5167640777479,51.1624999998058,10.3459381770593));
#296523=CARTESIAN_POINT('Ctrl Pts',(-3.75838203887397,51.3124999998052,
11.5671105274575));
#296524=CARTESIAN_POINT('Ctrl Pts',(-3.97658667625946E-14,51.4624999998046,
12.7882828778556));
#296525=CARTESIAN_POINT('Ctrl Pts',(3.75838203887389,51.612499999804,11.5671105274575));
#296526=CARTESIAN_POINT('Ctrl Pts',(7.51676407774782,51.7624999998034,10.3459381770593));
#296527=CARTESIAN_POINT('Ctrl Pts',(9.83957192047903,51.9124999998028,7.14886745759543));
#296528=CARTESIAN_POINT('Ctrl Pts',(12.1623797632103,52.0624999998022,3.95179673813153));
#296529=CARTESIAN_POINT('Ctrl Pts',(12.1623797632103,52.2124999998016,-1.489461944703E-15));
#296530=CARTESIAN_POINT('Ctrl Pts',(12.1623797632103,52.362499999801,-3.95179673813154));
#296531=CARTESIAN_POINT('Ctrl Pts',(9.83957192047903,52.5124999998004,-7.14886745759543));
#296532=CARTESIAN_POINT('Ctrl Pts',(7.51676407774781,52.6624999997998,-10.3459381770593));
#296533=CARTESIAN_POINT('Ctrl Pts',(3.75838203887388,52.8124999997992,-11.5671105274575));
#296534=CARTESIAN_POINT('Ctrl Pts',(-4.37619473370168E-14,52.9624999997986,
-12.7882828778556));
#296535=CARTESIAN_POINT('Ctrl Pts',(-3.75838203887397,53.112499999798,-11.5671105274575));
#296536=CARTESIAN_POINT('Ctrl Pts',(-7.5167640777479,53.2624999997974,-10.3459381770593));
#296537=CARTESIAN_POINT('Ctrl Pts',(-9.83957192047912,53.4124999997968,
-7.14886745759543));
#296538=CARTESIAN_POINT('Ctrl Pts',(-12.1623797632103,53.5624999997962,
-3.95179673813153));
#296539=CARTESIAN_POINT('Ctrl Pts',(-12.1623797632103,53.7124999997956,
2.97892388940601E-15));
#296540=CARTESIAN_POINT('Ctrl Pts',(-12.1623797632103,53.862499999795,3.95179673813154));
#296541=CARTESIAN_POINT('Ctrl Pts',(-9.83957192047912,54.0124999997944,
7.14886745759543));
#296542=CARTESIAN_POINT('Ctrl Pts',(-7.5167640777479,54.1624999997938,10.3459381770593));
#296543=CARTESIAN_POINT('Ctrl Pts',(-3.75838203887397,54.3124999997932,
11.5671105274575));
#296544=CARTESIAN_POINT('Ctrl Pts',(-4.14935760342564E-14,54.4624999997926,
12.7882828778556));
#296545=CARTESIAN_POINT('Ctrl Pts',(3.75838203887389,54.612499999792,11.5671105274575));
#296546=CARTESIAN_POINT('Ctrl Pts',(7.51676407774782,54.7624999997914,10.3459381770593));
#296547=CARTESIAN_POINT('Ctrl Pts',(9.83957192047903,54.9124999997908,7.14886745759543));
#296548=CARTESIAN_POINT('Ctrl Pts',(12.1623797632103,55.0624999997902,3.95179673813153));
#296549=CARTESIAN_POINT('Ctrl Pts',(12.1623797632103,55.2124999997896,-1.489461944703E-15));
#296550=CARTESIAN_POINT('Ctrl Pts',(12.1623797632103,55.362499999789,-3.95179673813154));
#296551=CARTESIAN_POINT('Ctrl Pts',(9.83957192047903,55.5124999997884,-7.14886745759543));
#296552=CARTESIAN_POINT('Ctrl Pts',(7.51676407774781,55.6624999997878,-10.3459381770593));
#296553=CARTESIAN_POINT('Ctrl Pts',(3.75838203887388,55.8124999997872,-11.5671105274575));
#296554=CARTESIAN_POINT('Ctrl Pts',(-4.54896566086787E-14,55.9624999997866,
-12.7882828778556));
#296555=CARTESIAN_POINT('Ctrl Pts',(-3.75838203887397,56.112499999786,-11.5671105274575));
#296556=CARTESIAN_POINT('Ctrl Pts',(-7.5167640777479,56.2624999997854,-10.3459381770593));
#296557=CARTESIAN_POINT('Ctrl Pts',(-9.83957192047912,56.4124999997848,
-7.14886745759543));
#296558=CARTESIAN_POINT('Ctrl Pts',(-12.1623797632103,56.5624999997842,
-3.95179673813153));
#296559=CARTESIAN_POINT('Ctrl Pts',(-12.1623797632103,56.7124999997836,
2.97892388940601E-15));
#296560=CARTESIAN_POINT('Ctrl Pts',(-12.1623797632103,56.862499999783,3.95179673813154));
#296561=CARTESIAN_POINT('Ctrl Pts',(-9.83957192047912,57.0124999997824,
7.14886745759543));
#296562=CARTESIAN_POINT('Ctrl Pts',(-7.5167640777479,57.1624999997818,10.3459381770593));
#296563=CARTESIAN_POINT('Ctrl Pts',(-3.75838203887397,57.3124999997812,
11.5671105274575));
#296564=CARTESIAN_POINT('Ctrl Pts',(-4.32212853059182E-14,57.4624999997806,
12.7882828778556));
#296565=CARTESIAN_POINT('Ctrl Pts',(3.75838203887389,57.61249999978,11.5671105274575));
#296566=CARTESIAN_POINT('Ctrl Pts',(7.51676407774781,57.7624999997794,10.3459381770593));
#296567=CARTESIAN_POINT('Ctrl Pts',(9.83957192047903,57.9124999997788,7.14886745759543));
#296568=CARTESIAN_POINT('Ctrl Pts',(12.1623797632103,58.0624999997782,3.95179673813153));
#296569=CARTESIAN_POINT('Ctrl Pts',(12.1623797632102,58.2124999997776,-1.489461944703E-15));
#296570=CARTESIAN_POINT('Ctrl Pts',(12.1623797632102,58.362499999777,-3.95179673813154));
#296571=CARTESIAN_POINT('Ctrl Pts',(9.83957192047903,58.5124999997764,-7.14886745759543));
#296572=CARTESIAN_POINT('Ctrl Pts',(7.51676407774781,58.6624999997758,-10.3459381770593));
#296573=CARTESIAN_POINT('Ctrl Pts',(3.75838203887388,58.8124999997752,-11.5671105274575));
#296574=CARTESIAN_POINT('Ctrl Pts',(-4.72173658803405E-14,58.9624999997746,
-12.7882828778556));
#296575=CARTESIAN_POINT('Ctrl Pts',(-3.75838203887398,59.112499999774,-11.5671105274575));
#296576=CARTESIAN_POINT('Ctrl Pts',(-7.51676407774791,59.2624999997734,
-10.3459381770593));
#296577=CARTESIAN_POINT('Ctrl Pts',(-9.83957192047912,59.4124999997728,
-7.14886745759543));
#296578=CARTESIAN_POINT('Ctrl Pts',(-12.1623797632103,59.5624999997722,
-3.95179673813153));
#296579=CARTESIAN_POINT('Ctrl Pts',(-12.1623797632103,59.7124999997716,
2.97892388940601E-15));
#296580=CARTESIAN_POINT('Ctrl Pts',(-12.1623797632103,59.862499999771,3.95179673813154));
#296581=CARTESIAN_POINT('Ctrl Pts',(-9.83957192047912,60.0124999997704,
7.14886745759543));
#296582=CARTESIAN_POINT('Ctrl Pts',(-7.5167640777479,60.1624999997698,10.3459381770593));
#296583=CARTESIAN_POINT('Ctrl Pts',(-3.75838203887397,60.3124999997692,
11.5671105274575));
#296584=CARTESIAN_POINT('Ctrl Pts',(-4.49489945775801E-14,60.4624999997686,
12.7882828778556));
#296585=CARTESIAN_POINT('Ctrl Pts',(3.75838203887388,60.612499999768,11.5671105274575));
#296586=CARTESIAN_POINT('Ctrl Pts',(7.51676407774781,60.7624999997674,10.3459381770593));
#296587=CARTESIAN_POINT('Ctrl Pts',(9.83957192047903,60.9124999997668,7.14886745759543));
#296588=CARTESIAN_POINT('Ctrl Pts',(12.1623797632103,61.0624999997662,3.95179673813153));
#296589=CARTESIAN_POINT('Ctrl Pts',(12.1623797632102,61.2124999997656,-1.489461944703E-15));
#296590=CARTESIAN_POINT('Ctrl Pts',(12.1623797632102,61.362499999765,-3.95179673813154));
#296591=CARTESIAN_POINT('Ctrl Pts',(9.83957192047902,61.5124999997644,-7.14886745759543));
#296592=CARTESIAN_POINT('Ctrl Pts',(7.51676407774781,61.6624999997638,-10.3459381770593));
#296593=CARTESIAN_POINT('Ctrl Pts',(3.75838203887388,61.8124999997632,-11.5671105274575));
#296594=CARTESIAN_POINT('Ctrl Pts',(-4.89450751520023E-14,61.9624999997626,
-12.7882828778556));
#296595=CARTESIAN_POINT('Ctrl Pts',(-3.75838203887398,62.112499999762,-11.5671105274575));
#296596=CARTESIAN_POINT('Ctrl Pts',(-7.51676407774791,62.2624999997614,
-10.3459381770593));
#296597=CARTESIAN_POINT('Ctrl Pts',(-9.83957192047912,62.4124999997608,
-7.14886745759543));
#296598=CARTESIAN_POINT('Ctrl Pts',(-12.1623797632103,62.5624999997602,
-3.95179673813153));
#296599=CARTESIAN_POINT('Ctrl Pts',(-12.1623797632103,62.7124999997596,
2.97892388940601E-15));
#296600=CARTESIAN_POINT('Ctrl Pts',(-12.1623797632103,62.862499999759,3.95179673813154));
#296601=CARTESIAN_POINT('Ctrl Pts',(-9.83957192047912,63.0124999997584,
7.14886745759543));
#296602=CARTESIAN_POINT('Ctrl Pts',(-7.5167640777479,63.1624999997578,10.3459381770593));
#296603=CARTESIAN_POINT('Ctrl Pts',(-3.75838203887398,63.3124999997572,
11.5671105274575));
#296604=CARTESIAN_POINT('Ctrl Pts',(-4.66767038492419E-14,63.4624999997566,
12.7882828778556));
#296605=CARTESIAN_POINT('Ctrl Pts',(3.75838203887388,63.612499999756,11.5671105274575));
#296606=CARTESIAN_POINT('Ctrl Pts',(7.51676407774781,63.7624999997554,10.3459381770593));
#296607=CARTESIAN_POINT('Ctrl Pts',(9.83957192047903,63.9124999997548,7.14886745759543));
#296608=CARTESIAN_POINT('Ctrl Pts',(12.1623797632102,64.0624999997542,3.95179673813153));
#296609=CARTESIAN_POINT('Ctrl Pts',(12.1623797632102,64.2124999997536,-1.489461944703E-15));
#296610=CARTESIAN_POINT('Ctrl Pts',(12.1623797632102,64.362499999753,-3.95179673813154));
#296611=CARTESIAN_POINT('Ctrl Pts',(9.83957192047902,64.5124999997524,-7.14886745759543));
#296612=CARTESIAN_POINT('Ctrl Pts',(7.51676407774781,64.6624999997518,-10.3459381770593));
#296613=CARTESIAN_POINT('Ctrl Pts',(3.75838203887388,64.8124999997512,-11.5671105274575));
#296614=CARTESIAN_POINT('Ctrl Pts',(-5.06727844236642E-14,64.9624999997506,
-12.7882828778556));
#296615=CARTESIAN_POINT('Ctrl Pts',(-3.75838203887398,65.11249999975,-11.5671105274575));
#296616=CARTESIAN_POINT('Ctrl Pts',(-7.51676407774791,65.2624999997494,
-10.3459381770593));
#296617=CARTESIAN_POINT('Ctrl Pts',(-9.83957192047913,65.4124999997488,
-7.14886745759543));
#296618=CARTESIAN_POINT('Ctrl Pts',(-12.1623797632103,65.5624999997482,
-3.95179673813153));
#296619=CARTESIAN_POINT('Ctrl Pts',(-12.1623797632103,65.7124999997476,
2.97892388940601E-15));
#296620=CARTESIAN_POINT('Ctrl Pts',(-12.1623797632103,65.862499999747,3.95179673813154));
#296621=CARTESIAN_POINT('Ctrl Pts',(-9.83957192047912,66.0124999997464,
7.14886745759543));
#296622=CARTESIAN_POINT('Ctrl Pts',(-7.51676407774791,66.1624999997458,
10.3459381770593));
#296623=CARTESIAN_POINT('Ctrl Pts',(-3.75838203887398,66.3124999997452,
11.5671105274575));
#296624=CARTESIAN_POINT('Ctrl Pts',(-4.84044131209037E-14,66.4624999997446,
12.7882828778556));
#296625=CARTESIAN_POINT('Ctrl Pts',(3.75838203887388,66.612499999744,11.5671105274575));
#296626=CARTESIAN_POINT('Ctrl Pts',(7.51676407774781,66.7624999997434,10.3459381770593));
#296627=CARTESIAN_POINT('Ctrl Pts',(9.83957192047902,66.9124999997428,7.14886745759543));
#296628=CARTESIAN_POINT('Ctrl Pts',(12.1623797632102,67.0624999997422,3.95179673813153));
#296629=CARTESIAN_POINT('Ctrl Pts',(12.1623797632102,67.2124999997416,-1.489461944703E-15));
#296630=CARTESIAN_POINT('Ctrl Pts',(12.1623797632102,67.362499999741,-3.95179673813154));
#296631=CARTESIAN_POINT('Ctrl Pts',(9.83957192047902,67.5124999997404,-7.14886745759543));
#296632=CARTESIAN_POINT('Ctrl Pts',(7.51676407774781,67.6624999997398,-10.3459381770593));
#296633=CARTESIAN_POINT('Ctrl Pts',(3.75838203887388,67.8124999997392,-11.5671105274575));
#296634=CARTESIAN_POINT('Ctrl Pts',(-5.2400493695326E-14,67.9624999997386,
-12.7882828778556));
#296635=CARTESIAN_POINT('Ctrl Pts',(-3.75838203887398,68.112499999738,-11.5671105274575));
#296636=CARTESIAN_POINT('Ctrl Pts',(-7.51676407774791,68.2624999997374,
-10.3459381770593));
#296637=CARTESIAN_POINT('Ctrl Pts',(-9.83957192047913,68.4124999997368,
-7.14886745759543));
#296638=CARTESIAN_POINT('Ctrl Pts',(-12.1623797632103,68.5624999997362,
-3.95179673813153));
#296639=CARTESIAN_POINT('Ctrl Pts',(-12.1623797632103,68.7124999997356,
2.97892388940601E-15));
#296640=CARTESIAN_POINT('Ctrl Pts',(-12.1623797632103,68.862499999735,3.95179673813154));
#296641=CARTESIAN_POINT('Ctrl Pts',(-9.83957192047913,69.0124999997344,
7.14886745759543));
#296642=CARTESIAN_POINT('Ctrl Pts',(-7.51676407774791,69.1624999997338,
10.3459381770593));
#296643=CARTESIAN_POINT('Ctrl Pts',(-3.75838203887398,69.3124999997332,
11.5671105274575));
#296644=CARTESIAN_POINT('Ctrl Pts',(-5.01321223925656E-14,69.4624999997326,
12.7882828778556));
#296645=CARTESIAN_POINT('Ctrl Pts',(3.75838203887388,69.612499999732,11.5671105274575));
#296646=CARTESIAN_POINT('Ctrl Pts',(7.51676407774781,69.7624999997314,10.3459381770593));
#296647=CARTESIAN_POINT('Ctrl Pts',(9.83957192047902,69.9124999997308,7.14886745759543));
#296648=CARTESIAN_POINT('Ctrl Pts',(12.1623797632102,70.0624999997302,3.95179673813153));
#296649=CARTESIAN_POINT('Ctrl Pts',(12.1623797632102,70.2124999997296,-1.489461944703E-15));
#296650=CARTESIAN_POINT('Ctrl Pts',(12.1623797632102,70.362499999729,-3.95179673813154));
#296651=CARTESIAN_POINT('Ctrl Pts',(9.83957192047902,70.5124999997284,-7.14886745759543));
#296652=CARTESIAN_POINT('Ctrl Pts',(7.5167640777478,70.6624999997278,-10.3459381770593));
#296653=CARTESIAN_POINT('Ctrl Pts',(3.75838203887388,70.8124999997272,-11.5671105274575));
#296654=CARTESIAN_POINT('Ctrl Pts',(-5.41282029669879E-14,70.9624999997266,
-12.7882828778556));
#296655=CARTESIAN_POINT('Ctrl Pts',(-3.75838203887398,71.112499999726,-11.5671105274575));
#296656=CARTESIAN_POINT('Ctrl Pts',(-7.51676407774791,71.2624999997254,
-10.3459381770593));
#296657=CARTESIAN_POINT('Ctrl Pts',(-9.83957192047913,71.4124999997248,
-7.14886745759543));
#296658=CARTESIAN_POINT('Ctrl Pts',(-12.1623797632103,71.5624999997242,
-3.95179673813153));
#296659=CARTESIAN_POINT('Ctrl Pts',(-12.1623797632103,71.7124999997236,
2.97892388940601E-15));
#296660=CARTESIAN_POINT('Ctrl Pts',(-12.1623797632103,71.862499999723,3.95179673813154));
#296661=CARTESIAN_POINT('Ctrl Pts',(-9.83957192047913,72.0124999997224,
7.14886745759543));
#296662=CARTESIAN_POINT('Ctrl Pts',(-7.51676407774791,72.1624999997218,
10.3459381770593));
#296663=CARTESIAN_POINT('Ctrl Pts',(-3.75838203887398,72.3124999997212,
11.5671105274575));
#296664=CARTESIAN_POINT('Ctrl Pts',(-5.18598316642274E-14,72.4624999997206,
12.7882828778556));
#296665=CARTESIAN_POINT('Ctrl Pts',(3.75838203887388,72.61249999972,11.5671105274575));
#296666=CARTESIAN_POINT('Ctrl Pts',(7.51676407774781,72.7624999997194,10.3459381770593));
#296667=CARTESIAN_POINT('Ctrl Pts',(9.83957192047902,72.9124999997188,7.14886745759543));
#296668=CARTESIAN_POINT('Ctrl Pts',(12.1623797632102,73.0624999997182,3.95179673813153));
#296669=CARTESIAN_POINT('Ctrl Pts',(12.1623797632102,73.2124999997176,-1.489461944703E-15));
#296670=CARTESIAN_POINT('Ctrl Pts',(12.1623797632102,73.362499999717,-3.95179673813154));
#296671=CARTESIAN_POINT('Ctrl Pts',(9.83957192047902,73.5124999997164,-7.14886745759543));
#296672=CARTESIAN_POINT('Ctrl Pts',(7.5167640777478,73.6624999997158,-10.3459381770593));
#296673=CARTESIAN_POINT('Ctrl Pts',(3.75838203887387,73.8124999997152,-11.5671105274575));
#296674=CARTESIAN_POINT('Ctrl Pts',(-5.58559122386497E-14,73.9624999997146,
-12.7882828778556));
#296675=CARTESIAN_POINT('Ctrl Pts',(-3.75838203887398,74.112499999714,-11.5671105274575));
#296676=CARTESIAN_POINT('Ctrl Pts',(-7.51676407774791,74.2624999997134,
-10.3459381770593));
#296677=CARTESIAN_POINT('Ctrl Pts',(-9.83957192047913,74.4124999997128,
-7.14886745759543));
#296678=CARTESIAN_POINT('Ctrl Pts',(-12.1623797632103,74.5624999997122,
-3.95179673813153));
#296679=CARTESIAN_POINT('Ctrl Pts',(-12.1623797632103,74.7124999997116,
2.97892388940601E-15));
#296680=CARTESIAN_POINT('Ctrl Pts',(-12.1623797632103,74.862499999711,3.95179673813154));
#296681=CARTESIAN_POINT('Ctrl Pts',(-9.83957192047913,75.0124999997104,
7.14886745759543));
#296682=CARTESIAN_POINT('Ctrl Pts',(-7.51676407774791,75.1624999997098,
10.3459381770593));
#296683=CARTESIAN_POINT('Ctrl Pts',(-3.75838203887398,75.3124999997092,
11.5671105274575));
#296684=CARTESIAN_POINT('Ctrl Pts',(-5.35875409358893E-14,75.4624999997086,
12.7882828778556));
#296685=CARTESIAN_POINT('Ctrl Pts',(3.75838203887388,75.612499999708,11.5671105274575));
#296686=CARTESIAN_POINT('Ctrl Pts',(7.5167640777478,75.7624999997074,10.3459381770593));
#296687=CARTESIAN_POINT('Ctrl Pts',(9.83957192047902,75.9124999997068,7.14886745759543));
#296688=CARTESIAN_POINT('Ctrl Pts',(12.1623797632102,76.0624999997062,3.95179673813153));
#296689=CARTESIAN_POINT('Ctrl Pts',(12.1623797632102,76.2124999997056,-1.489461944703E-15));
#296690=CARTESIAN_POINT('Ctrl Pts',(12.1623797632102,76.362499999705,-3.95179673813154));
#296691=CARTESIAN_POINT('Ctrl Pts',(9.83957192047902,76.5124999997044,-7.14886745759543));
#296692=CARTESIAN_POINT('Ctrl Pts',(7.5167640777478,76.6624999997038,-10.3459381770593));
#296693=CARTESIAN_POINT('Ctrl Pts',(3.75838203887387,76.8124999997032,-11.5671105274575));
#296694=CARTESIAN_POINT('Ctrl Pts',(-5.75836215103115E-14,76.9624999997026,
-12.7882828778556));
#296695=CARTESIAN_POINT('Ctrl Pts',(-3.75838203887399,77.112499999702,-11.5671105274575));
#296696=CARTESIAN_POINT('Ctrl Pts',(-7.51676407774791,77.2624999997014,
-10.3459381770593));
#296697=CARTESIAN_POINT('Ctrl Pts',(-9.83957192047913,77.4124999997008,
-7.14886745759543));
#296698=CARTESIAN_POINT('Ctrl Pts',(-12.1623797632103,77.5624999997002,
-3.95179673813153));
#296699=CARTESIAN_POINT('Ctrl Pts',(-12.1623797632103,77.7124999996996,
2.97892388940601E-15));
#296700=CARTESIAN_POINT('Ctrl Pts',(-12.1623797632103,77.862499999699,3.95179673813154));
#296701=CARTESIAN_POINT('Ctrl Pts',(-9.83957192047913,78.0124999996984,
7.14886745759543));
#296702=CARTESIAN_POINT('Ctrl Pts',(-7.51676407774791,78.1624999996978,
10.3459381770593));
#296703=CARTESIAN_POINT('Ctrl Pts',(-3.75838203887398,78.3124999996972,
11.5671105274575));
#296704=CARTESIAN_POINT('Ctrl Pts',(-5.53152502075511E-14,78.4624999996966,
12.7882828778556));
#296705=CARTESIAN_POINT('Ctrl Pts',(3.75838203887387,78.612499999696,11.5671105274575));
#296706=CARTESIAN_POINT('Ctrl Pts',(7.5167640777478,78.7624999996954,10.3459381770593));
#296707=CARTESIAN_POINT('Ctrl Pts',(9.83957192047902,78.9124999996948,7.14886745759543));
#296708=CARTESIAN_POINT('Ctrl Pts',(12.1623797632102,79.0624999996942,3.95179673813153));
#296709=CARTESIAN_POINT('Ctrl Pts',(12.1623797632102,79.2124999996936,-1.489461944703E-15));
#296710=CARTESIAN_POINT('Ctrl Pts',(12.1623797632102,79.362499999693,-3.95179673813154));
#296711=CARTESIAN_POINT('Ctrl Pts',(9.83957192047902,79.5124999996924,-7.14886745759543));
#296712=CARTESIAN_POINT('Ctrl Pts',(7.5167640777478,79.6624999996918,-10.3459381770593));
#296713=CARTESIAN_POINT('Ctrl Pts',(3.75838203887387,79.8124999996912,-11.5671105274575));
#296714=CARTESIAN_POINT('Ctrl Pts',(-5.93113307819734E-14,79.9624999996906,
-12.7882828778556));
#296715=CARTESIAN_POINT('Ctrl Pts',(-3.75838203887399,80.11249999969,-11.5671105274575));
#296716=CARTESIAN_POINT('Ctrl Pts',(-7.51676407774791,80.2624999996894,
-10.3459381770593));
#296717=CARTESIAN_POINT('Ctrl Pts',(-9.83957192047913,80.4124999996888,
-7.14886745759543));
#296718=CARTESIAN_POINT('Ctrl Pts',(-12.1623797632104,80.5624999996882,
-3.95179673813153));
#296719=CARTESIAN_POINT('Ctrl Pts',(-12.1623797632104,80.7124999996876,
2.97892388940601E-15));
#296720=CARTESIAN_POINT('Ctrl Pts',(-12.1623797632104,80.862499999687,3.95179673813154));
#296721=CARTESIAN_POINT('Ctrl Pts',(-9.83957192047913,81.0124999996864,
7.14886745759543));
#296722=CARTESIAN_POINT('Ctrl Pts',(-7.51676407774791,81.1624999996858,
10.3459381770593));
#296723=CARTESIAN_POINT('Ctrl Pts',(-3.75838203887399,81.3124999996852,
11.5671105274575));
#296724=CARTESIAN_POINT('Ctrl Pts',(-5.70429594792129E-14,81.4624999996846,
12.7882828778556));
#296725=CARTESIAN_POINT('Ctrl Pts',(3.75838203887387,81.612499999684,11.5671105274575));
#296726=CARTESIAN_POINT('Ctrl Pts',(7.5167640777478,81.7624999996834,10.3459381770593));
#296727=CARTESIAN_POINT('Ctrl Pts',(9.83957192047902,81.9124999996828,7.14886745759543));
#296728=CARTESIAN_POINT('Ctrl Pts',(12.1623797632102,82.0624999996822,3.95179673813153));
#296729=CARTESIAN_POINT('Ctrl Pts',(12.1623797632102,82.2124999996816,-1.489461944703E-15));
#296730=CARTESIAN_POINT('Ctrl Pts',(12.1623797632102,82.362499999681,-3.95179673813154));
#296731=CARTESIAN_POINT('Ctrl Pts',(9.83957192047902,82.5124999996804,-7.14886745759543));
#296732=CARTESIAN_POINT('Ctrl Pts',(7.5167640777478,82.6624999996798,-10.3459381770593));
#296733=CARTESIAN_POINT('Ctrl Pts',(3.75838203887387,82.8124999996792,-11.5671105274575));
#296734=CARTESIAN_POINT('Ctrl Pts',(-6.10390400536352E-14,82.9624999996786,
-12.7882828778556));
#296735=CARTESIAN_POINT('Ctrl Pts',(-3.75838203887399,83.112499999678,-11.5671105274575));
#296736=CARTESIAN_POINT('Ctrl Pts',(-7.51676407774792,83.2624999996774,
-10.3459381770593));
#296737=CARTESIAN_POINT('Ctrl Pts',(-9.83957192047914,83.4124999996768,
-7.14886745759543));
#296738=CARTESIAN_POINT('Ctrl Pts',(-12.1623797632104,83.5624999996762,
-3.95179673813153));
#296739=CARTESIAN_POINT('Ctrl Pts',(-12.1623797632104,83.7124999996756,
2.97892388940601E-15));
#296740=CARTESIAN_POINT('Ctrl Pts',(-12.1623797632104,83.862499999675,3.95179673813154));
#296741=CARTESIAN_POINT('Ctrl Pts',(-9.83957192047913,84.0124999996744,
7.14886745759543));
#296742=CARTESIAN_POINT('Ctrl Pts',(-7.51676407774791,84.1624999996738,
10.3459381770593));
#296743=CARTESIAN_POINT('Ctrl Pts',(-3.75838203887399,84.3124999996732,
11.5671105274575));
#296744=CARTESIAN_POINT('Ctrl Pts',(-5.87706687508748E-14,84.4624999996726,
12.7882828778556));
#296745=CARTESIAN_POINT('Ctrl Pts',(3.75838203887387,84.6124999996721,11.5671105274575));
#296746=CARTESIAN_POINT('Ctrl Pts',(7.5167640777478,84.7624999996714,10.3459381770593));
#296747=CARTESIAN_POINT('Ctrl Pts',(9.83957192047902,84.9124999996708,7.14886745759543));
#296748=CARTESIAN_POINT('Ctrl Pts',(12.1623797632102,85.0624999996702,3.95179673813153));
#296749=CARTESIAN_POINT('Ctrl Pts',(12.1623797632102,85.2124999996696,-1.489461944703E-15));
#296750=CARTESIAN_POINT('Ctrl Pts',(12.1623797632102,85.362499999669,-3.95179673813154));
#296751=CARTESIAN_POINT('Ctrl Pts',(9.83957192047901,85.5124999996684,-7.14886745759543));
#296752=CARTESIAN_POINT('Ctrl Pts',(7.5167640777478,85.6624999996678,-10.3459381770593));
#296753=CARTESIAN_POINT('Ctrl Pts',(3.75838203887387,85.8124999996672,-11.5671105274575));
#296754=CARTESIAN_POINT('Ctrl Pts',(-6.27667493252971E-14,85.9624999996666,
-12.7882828778556));
#296755=CARTESIAN_POINT('Ctrl Pts',(-3.75838203887399,86.112499999666,-11.5671105274575));
#296756=CARTESIAN_POINT('Ctrl Pts',(-7.51676407774792,86.2624999996654,
-10.3459381770593));
#296757=CARTESIAN_POINT('Ctrl Pts',(-9.83957192047914,86.4124999996648,
-7.14886745759543));
#296758=CARTESIAN_POINT('Ctrl Pts',(-12.1623797632104,86.5624999996642,
-3.95179673813153));
#296759=CARTESIAN_POINT('Ctrl Pts',(-12.1623797632104,86.7124999996636,
2.97892388940601E-15));
#296760=CARTESIAN_POINT('Ctrl Pts',(-12.1623797632104,86.862499999663,3.95179673813154));
#296761=CARTESIAN_POINT('Ctrl Pts',(-9.83957192047914,87.0124999996624,
7.14886745759543));
#296762=CARTESIAN_POINT('Ctrl Pts',(-7.51676407774792,87.1624999996618,
10.3459381770593));
#296763=CARTESIAN_POINT('Ctrl Pts',(-3.75838203887399,87.3124999996612,
11.5671105274575));
#296764=CARTESIAN_POINT('Ctrl Pts',(-6.04983780225366E-14,87.4624999996606,
12.7882828778556));
#296765=CARTESIAN_POINT('Ctrl Pts',(3.75838203887387,87.61249999966,11.5671105274575));
#296766=CARTESIAN_POINT('Ctrl Pts',(7.5167640777478,87.7624999996594,10.3459381770593));
#296767=CARTESIAN_POINT('Ctrl Pts',(9.83957192047901,87.9124999996588,7.14886745759543));
#296768=CARTESIAN_POINT('Ctrl Pts',(12.1623797632102,88.0624999996582,3.95179673813153));
#296769=CARTESIAN_POINT('Ctrl Pts',(12.1623797632102,88.2124999996576,-1.489461944703E-15));
#296770=CARTESIAN_POINT('Ctrl Pts',(12.1623797632102,88.362499999657,-3.95179673813154));
#296771=CARTESIAN_POINT('Ctrl Pts',(9.83957192047901,88.5124999996564,-7.14886745759543));
#296772=CARTESIAN_POINT('Ctrl Pts',(7.51676407774779,88.6624999996558,-10.3459381770593));
#296773=CARTESIAN_POINT('Ctrl Pts',(3.75838203887386,88.8124999996552,-11.5671105274575));
#296774=CARTESIAN_POINT('Ctrl Pts',(-6.44944585969589E-14,88.9624999996546,
-12.7882828778556));
#296775=CARTESIAN_POINT('Ctrl Pts',(-3.75838203887399,89.112499999654,-11.5671105274575));
#296776=CARTESIAN_POINT('Ctrl Pts',(-7.51676407774792,89.2624999996534,
-10.3459381770593));
#296777=CARTESIAN_POINT('Ctrl Pts',(-9.83957192047914,89.4124999996528,
-7.14886745759543));
#296778=CARTESIAN_POINT('Ctrl Pts',(-12.1623797632104,89.5624999996522,
-3.95179673813153));
#296779=CARTESIAN_POINT('Ctrl Pts',(-12.1623797632104,89.7124999996516,
2.97892388940601E-15));
#296780=CARTESIAN_POINT('Ctrl Pts',(-12.1623797632104,89.862499999651,3.95179673813154));
#296781=CARTESIAN_POINT('Ctrl Pts',(-9.83957192047914,90.0124999996504,
7.14886745759543));
#296782=CARTESIAN_POINT('Ctrl Pts',(-7.51676407774792,90.1624999996498,
10.3459381770593));
#296783=CARTESIAN_POINT('Ctrl Pts',(-3.75838203887399,90.3124999996492,
11.5671105274575));
#296784=CARTESIAN_POINT('Ctrl Pts',(-6.22260872941985E-14,90.4624999996486,
12.7882828778556));
#296785=CARTESIAN_POINT('Ctrl Pts',(3.75838203887387,90.612499999648,11.5671105274575));
#296786=CARTESIAN_POINT('Ctrl Pts',(7.5167640777478,90.7624999996474,10.3459381770593));
#296787=CARTESIAN_POINT('Ctrl Pts',(9.83957192047901,90.9124999996468,7.14886745759543));
#296788=CARTESIAN_POINT('Ctrl Pts',(12.1623797632102,91.0624999996462,3.95179673813153));
#296789=CARTESIAN_POINT('Ctrl Pts',(12.1623797632102,91.2124999996456,-1.489461944703E-15));
#296790=CARTESIAN_POINT('Ctrl Pts',(12.1623797632102,91.362499999645,-3.95179673813154));
#296791=CARTESIAN_POINT('Ctrl Pts',(9.83957192047901,91.5124999996444,-7.14886745759543));
#296792=CARTESIAN_POINT('Ctrl Pts',(7.51676407774779,91.6624999996438,-10.3459381770593));
#296793=CARTESIAN_POINT('Ctrl Pts',(3.75838203887386,91.8124999996432,-11.5671105274575));
#296794=CARTESIAN_POINT('Ctrl Pts',(-6.62221678686207E-14,91.9624999996426,
-12.7882828778556));
#296795=CARTESIAN_POINT('Ctrl Pts',(-3.75838203887399,92.112499999642,-11.5671105274575));
#296796=CARTESIAN_POINT('Ctrl Pts',(-7.51676407774792,92.2624999996414,
-10.3459381770593));
#296797=CARTESIAN_POINT('Ctrl Pts',(-9.83957192047914,92.4124999996408,
-7.14886745759543));
#296798=CARTESIAN_POINT('Ctrl Pts',(-12.1623797632104,92.5624999996402,
-3.95179673813153));
#296799=CARTESIAN_POINT('Ctrl Pts',(-12.1623797632104,92.7124999996396,
2.97892388940601E-15));
#296800=CARTESIAN_POINT('Ctrl Pts',(-12.1623797632104,92.862499999639,3.95179673813154));
#296801=CARTESIAN_POINT('Ctrl Pts',(-9.83957192047914,93.0124999996384,
7.14886745759543));
#296802=CARTESIAN_POINT('Ctrl Pts',(-7.51676407774792,93.1624999996378,
10.3459381770593));
#296803=CARTESIAN_POINT('Ctrl Pts',(-3.75838203887399,93.3124999996372,
11.5671105274575));
#296804=CARTESIAN_POINT('Ctrl Pts',(-6.39537965658603E-14,93.4624999996366,
12.7882828778556));
#296805=CARTESIAN_POINT('Ctrl Pts',(3.75838203887386,93.612499999636,11.5671105274575));
#296806=CARTESIAN_POINT('Ctrl Pts',(7.51676407774779,93.7624999996354,10.3459381770593));
#296807=CARTESIAN_POINT('Ctrl Pts',(9.83957192047901,93.9124999996348,7.14886745759543));
#296808=CARTESIAN_POINT('Ctrl Pts',(12.1623797632102,94.0624999996342,3.95179673813153));
#296809=CARTESIAN_POINT('Ctrl Pts',(12.1623797632102,94.2124999996336,-1.489461944703E-15));
#296810=CARTESIAN_POINT('Ctrl Pts',(12.1623797632102,94.362499999633,-3.95179673813154));
#296811=CARTESIAN_POINT('Ctrl Pts',(9.83957192047901,94.5124999996324,-7.14886745759543));
#296812=CARTESIAN_POINT('Ctrl Pts',(7.51676407774779,94.6624999996318,-10.3459381770593));
#296813=CARTESIAN_POINT('Ctrl Pts',(3.75838203887386,94.8124999996312,-11.5671105274575));
#296814=CARTESIAN_POINT('Ctrl Pts',(-6.79498771402825E-14,94.9624999996306,
-12.7882828778556));
#296815=CARTESIAN_POINT('Ctrl Pts',(-3.758382038874,95.11249999963,-11.5671105274575));
#296816=CARTESIAN_POINT('Ctrl Pts',(-7.51676407774792,95.2624999996294,
-10.3459381770593));
#296817=CARTESIAN_POINT('Ctrl Pts',(-9.83957192047914,95.4124999996288,
-7.14886745759543));
#296818=CARTESIAN_POINT('Ctrl Pts',(-12.1623797632104,95.5624999996282,
-3.95179673813153));
#296819=CARTESIAN_POINT('Ctrl Pts',(-12.1623797632104,95.7124999996276,
2.97892388940601E-15));
#296820=CARTESIAN_POINT('Ctrl Pts',(-12.1623797632104,95.862499999627,3.95179673813154));
#296821=CARTESIAN_POINT('Ctrl Pts',(-9.83957192047914,96.0124999996264,
7.14886745759543));
#296822=CARTESIAN_POINT('Ctrl Pts',(-7.51676407774792,96.1624999996258,
10.3459381770593));
#296823=CARTESIAN_POINT('Ctrl Pts',(-3.75838203887399,96.3124999996252,
11.5671105274575));
#296824=CARTESIAN_POINT('Ctrl Pts',(-6.56815058375222E-14,96.4624999996246,
12.7882828778556));
#296825=CARTESIAN_POINT('Ctrl Pts',(3.75838203887386,96.612499999624,11.5671105274575));
#296826=CARTESIAN_POINT('Ctrl Pts',(7.51676407774779,96.7624999996234,10.3459381770593));
#296827=CARTESIAN_POINT('Ctrl Pts',(9.83957192047901,96.9124999996228,7.14886745759543));
#296828=CARTESIAN_POINT('Ctrl Pts',(12.1623797632102,97.0624999996222,3.95179673813153));
#296829=CARTESIAN_POINT('Ctrl Pts',(12.1623797632102,97.2124999996216,-1.489461944703E-15));
#296830=CARTESIAN_POINT('Ctrl Pts',(12.1623797632102,97.3624999996211,-3.95179673813154));
#296831=CARTESIAN_POINT('Ctrl Pts',(9.83957192047901,97.5124999996204,-7.14886745759543));
#296832=CARTESIAN_POINT('Ctrl Pts',(7.51676407774779,97.6624999996198,-10.3459381770593));
#296833=CARTESIAN_POINT('Ctrl Pts',(3.75838203887386,97.8124999996192,-11.5671105274575));
#296834=CARTESIAN_POINT('Ctrl Pts',(-6.96775864119444E-14,97.9624999996187,
-12.7882828778556));
#296835=CARTESIAN_POINT('Ctrl Pts',(-3.758382038874,98.112499999618,-11.5671105274575));
#296836=CARTESIAN_POINT('Ctrl Pts',(-7.51676407774793,98.2624999996174,
-10.3459381770593));
#296837=CARTESIAN_POINT('Ctrl Pts',(-9.83957192047914,98.4124999996168,
-7.14886745759543));
#296838=CARTESIAN_POINT('Ctrl Pts',(-12.1623797632104,98.5624999996162,
-3.95179673813153));
#296839=CARTESIAN_POINT('Ctrl Pts',(-12.1623797632104,98.7124999996156,
2.97892388940601E-15));
#296840=CARTESIAN_POINT('Ctrl Pts',(-12.1623797632104,98.862499999615,3.95179673813154));
#296841=CARTESIAN_POINT('Ctrl Pts',(-9.83957192047914,99.0124999996144,
7.14886745759543));
#296842=CARTESIAN_POINT('Ctrl Pts',(-7.51676407774792,99.1624999996138,
10.3459381770593));
#296843=CARTESIAN_POINT('Ctrl Pts',(-3.758382038874,99.3124999996132,11.5671105274575));
#296844=CARTESIAN_POINT('Ctrl Pts',(-6.7409215109184E-14,99.4624999996126,
12.7882828778556));
#296845=CARTESIAN_POINT('Ctrl Pts',(3.75838203887386,99.612499999612,11.5671105274575));
#296846=CARTESIAN_POINT('Ctrl Pts',(7.51676407774779,99.7624999996114,10.3459381770593));
#296847=CARTESIAN_POINT('Ctrl Pts',(9.83957192047901,99.9124999996108,7.14886745759543));
#296848=CARTESIAN_POINT('Ctrl Pts',(12.1623797632102,100.06249999961,3.95179673813153));
#296849=CARTESIAN_POINT('Ctrl Pts',(12.1623797632102,100.21249999961,-1.489461944703E-15));
#296850=CARTESIAN_POINT('Ctrl Pts',(12.1623797632102,100.362499999609,-3.95179673813154));
#296851=CARTESIAN_POINT('Ctrl Pts',(9.839571920479,100.512499999608,-7.14886745759543));
#296852=CARTESIAN_POINT('Ctrl Pts',(7.51676407774779,100.662499999608,-10.3459381770593));
#296853=CARTESIAN_POINT('Ctrl Pts',(3.75838203887386,100.812499999607,-11.5671105274575));
#296854=CARTESIAN_POINT('Ctrl Pts',(-7.14052956836063E-14,100.962499999607,
-12.7882828778556));
#296855=CARTESIAN_POINT('Ctrl Pts',(-3.758382038874,101.112499999606,-11.5671105274575));
#296856=CARTESIAN_POINT('Ctrl Pts',(-7.51676407774793,101.262499999605,
-10.3459381770593));
#296857=CARTESIAN_POINT('Ctrl Pts',(-9.83957192047915,101.412499999605,
-7.14886745759543));
#296858=CARTESIAN_POINT('Ctrl Pts',(-12.1623797632104,101.562499999604,
-3.95179673813153));
#296859=CARTESIAN_POINT('Ctrl Pts',(-12.1623797632104,101.712499999604,
2.97892388940601E-15));
#296860=CARTESIAN_POINT('Ctrl Pts',(-12.1623797632104,101.862499999603,
3.95179673813154));
#296861=CARTESIAN_POINT('Ctrl Pts',(-9.83957192047914,102.012499999602,
7.14886745759543));
#296862=CARTESIAN_POINT('Ctrl Pts',(-7.51676407774793,102.162499999602,
10.3459381770593));
#296863=CARTESIAN_POINT('Ctrl Pts',(-3.758382038874,102.312499999601,11.5671105274575));
#296864=CARTESIAN_POINT('Ctrl Pts',(-6.91369243808458E-14,102.462499999601,
12.7882828778556));
#296865=CARTESIAN_POINT('Ctrl Pts',(3.75838203887386,102.6124999996,11.5671105274575));
#296866=CARTESIAN_POINT('Ctrl Pts',(7.51676407774779,102.762499999599,10.3459381770593));
#296867=CARTESIAN_POINT('Ctrl Pts',(9.839571920479,102.912499999599,7.14886745759543));
#296868=CARTESIAN_POINT('Ctrl Pts',(12.1623797632102,103.062499999598,3.95179673813153));
#296869=CARTESIAN_POINT('Ctrl Pts',(12.1623797632102,103.212499999598,-1.489461944703E-15));
#296870=CARTESIAN_POINT('Ctrl Pts',(12.1623797632102,103.362499999597,-3.95179673813154));
#296871=CARTESIAN_POINT('Ctrl Pts',(9.839571920479,103.512499999596,-7.14886745759543));
#296872=CARTESIAN_POINT('Ctrl Pts',(7.51676407774779,103.662499999596,-10.3459381770593));
#296873=CARTESIAN_POINT('Ctrl Pts',(3.75838203887386,103.812499999595,-11.5671105274575));
#296874=CARTESIAN_POINT('Ctrl Pts',(-7.31330049552681E-14,103.962499999595,
-12.7882828778556));
#296875=CARTESIAN_POINT('Ctrl Pts',(-3.758382038874,104.112499999594,-11.5671105274575));
#296876=CARTESIAN_POINT('Ctrl Pts',(-7.51676407774793,104.262499999593,
-10.3459381770593));
#296877=CARTESIAN_POINT('Ctrl Pts',(-9.83957192047915,104.412499999593,
-7.14886745759543));
#296878=CARTESIAN_POINT('Ctrl Pts',(-12.1623797632104,104.562499999592,
-3.95179673813153));
#296879=CARTESIAN_POINT('Ctrl Pts',(-12.1623797632104,104.712499999592,
2.97892388940601E-15));
#296880=CARTESIAN_POINT('Ctrl Pts',(-12.1623797632104,104.862499999591,
3.95179673813154));
#296881=CARTESIAN_POINT('Ctrl Pts',(-9.83957192047915,105.01249999959,7.14886745759543));
#296882=CARTESIAN_POINT('Ctrl Pts',(-7.51676407774793,105.16249999959,10.3459381770593));
#296883=CARTESIAN_POINT('Ctrl Pts',(-3.758382038874,105.312499999589,11.5671105274575));
#296884=CARTESIAN_POINT('Ctrl Pts',(-7.08646336525076E-14,105.462499999589,
12.7882828778556));
#296885=CARTESIAN_POINT('Ctrl Pts',(3.75838203887386,105.612499999588,11.5671105274575));
#296886=CARTESIAN_POINT('Ctrl Pts',(7.51676407774779,105.762499999587,10.3459381770593));
#296887=CARTESIAN_POINT('Ctrl Pts',(9.839571920479,105.912499999587,7.14886745759543));
#296888=CARTESIAN_POINT('Ctrl Pts',(12.1623797632102,106.062499999586,3.95179673813153));
#296889=CARTESIAN_POINT('Ctrl Pts',(12.1623797632102,106.212499999586,-1.489461944703E-15));
#296890=CARTESIAN_POINT('Ctrl Pts',(12.1623797632102,106.362499999585,-3.95179673813154));
#296891=CARTESIAN_POINT('Ctrl Pts',(9.839571920479,106.512499999584,-7.14886745759543));
#296892=CARTESIAN_POINT('Ctrl Pts',(7.51676407774778,106.662499999584,-10.3459381770593));
#296893=CARTESIAN_POINT('Ctrl Pts',(3.75838203887385,106.812499999583,-11.5671105274575));
#296894=CARTESIAN_POINT('Ctrl Pts',(-7.48607142269299E-14,106.962499999583,
-12.7882828778556));
#296895=CARTESIAN_POINT('Ctrl Pts',(-3.758382038874,107.112499999582,-11.5671105274575));
#296896=CARTESIAN_POINT('Ctrl Pts',(-7.51676407774793,107.262499999581,
-10.3459381770593));
#296897=CARTESIAN_POINT('Ctrl Pts',(-9.83957192047915,107.412499999581,
-7.14886745759543));
#296898=CARTESIAN_POINT('Ctrl Pts',(-12.1623797632104,107.56249999958,-3.95179673813153));
#296899=CARTESIAN_POINT('Ctrl Pts',(-12.1623797632104,107.71249999958,2.97892388940601E-15));
#296900=CARTESIAN_POINT('Ctrl Pts',(-12.1623797632104,107.862499999579,
3.95179673813154));
#296901=CARTESIAN_POINT('Ctrl Pts',(-9.83957192047915,108.012499999578,
7.14886745759543));
#296902=CARTESIAN_POINT('Ctrl Pts',(-7.51676407774793,108.162499999578,
10.3459381770593));
#296903=CARTESIAN_POINT('Ctrl Pts',(-3.758382038874,108.312499999577,11.5671105274575));
#296904=CARTESIAN_POINT('Ctrl Pts',(-7.25923429241695E-14,108.462499999577,
12.7882828778556));
#296905=CARTESIAN_POINT('Ctrl Pts',(3.75838203887386,108.612499999576,11.5671105274575));
#296906=CARTESIAN_POINT('Ctrl Pts',(7.51676407774779,108.762499999575,10.3459381770593));
#296907=CARTESIAN_POINT('Ctrl Pts',(9.839571920479,108.912499999575,7.14886745759543));
#296908=CARTESIAN_POINT('Ctrl Pts',(12.1623797632102,109.062499999574,3.95179673813153));
#296909=CARTESIAN_POINT('Ctrl Pts',(12.1623797632102,109.212499999574,-1.489461944703E-15));
#296910=CARTESIAN_POINT('Ctrl Pts',(12.1623797632102,109.362499999573,-3.95179673813154));
#296911=CARTESIAN_POINT('Ctrl Pts',(9.839571920479,109.512499999572,-7.14886745759543));
#296912=CARTESIAN_POINT('Ctrl Pts',(7.51676407774778,109.662499999572,-10.3459381770593));
#296913=CARTESIAN_POINT('Ctrl Pts',(3.75838203887385,109.812499999571,-11.5671105274575));
#296914=CARTESIAN_POINT('Ctrl Pts',(-7.65884234985918E-14,109.962499999571,
-12.7882828778556));
#296915=CARTESIAN_POINT('Ctrl Pts',(-3.75838203887401,110.11249999957,-11.5671105274575));
#296916=CARTESIAN_POINT('Ctrl Pts',(-7.51676407774793,110.262499999569,
-10.3459381770593));
#296917=CARTESIAN_POINT('Ctrl Pts',(-9.83957192047915,110.412499999569,
-7.14886745759543));
#296918=CARTESIAN_POINT('Ctrl Pts',(-12.1623797632104,110.562499999568,
-3.95179673813153));
#296919=CARTESIAN_POINT('Ctrl Pts',(-12.1623797632104,110.712499999568,
2.97892388940601E-15));
#296920=CARTESIAN_POINT('Ctrl Pts',(-12.1623797632104,110.862499999567,
3.95179673813154));
#296921=CARTESIAN_POINT('Ctrl Pts',(-9.83957192047915,111.012499999566,
7.14886745759543));
#296922=CARTESIAN_POINT('Ctrl Pts',(-7.51676407774793,111.162499999566,
10.3459381770593));
#296923=CARTESIAN_POINT('Ctrl Pts',(-3.758382038874,111.312499999565,11.5671105274575));
#296924=CARTESIAN_POINT('Ctrl Pts',(-7.43200521958313E-14,111.462499999565,
12.7882828778556));
#296925=CARTESIAN_POINT('Ctrl Pts',(3.75838203887385,111.612499999564,11.5671105274575));
#296926=CARTESIAN_POINT('Ctrl Pts',(7.51676407774778,111.762499999563,10.3459381770593));
#296927=CARTESIAN_POINT('Ctrl Pts',(9.839571920479,111.912499999563,7.14886745759543));
#296928=CARTESIAN_POINT('Ctrl Pts',(12.1623797632102,112.062499999562,3.95179673813153));
#296929=CARTESIAN_POINT('Ctrl Pts',(12.1623797632102,112.212499999562,-1.489461944703E-15));
#296930=CARTESIAN_POINT('Ctrl Pts',(12.1623797632102,112.362499999561,-3.95179673813154));
#296931=CARTESIAN_POINT('Ctrl Pts',(9.839571920479,112.51249999956,-7.14886745759543));
#296932=CARTESIAN_POINT('Ctrl Pts',(7.51676407774778,112.66249999956,-10.3459381770593));
#296933=CARTESIAN_POINT('Ctrl Pts',(3.75838203887385,112.812499999559,-11.5671105274575));
#296934=CARTESIAN_POINT('Ctrl Pts',(-7.83161327702536E-14,112.962499999559,
-12.7882828778556));
#296935=CARTESIAN_POINT('Ctrl Pts',(-3.75838203887401,113.112499999558,
-11.5671105274575));
#296936=CARTESIAN_POINT('Ctrl Pts',(-7.51676407774793,113.262499999557,
-10.3459381770593));
#296937=CARTESIAN_POINT('Ctrl Pts',(-9.83957192047915,113.412499999557,
-7.14886745759543));
#296938=CARTESIAN_POINT('Ctrl Pts',(-12.1623797632104,113.562499999556,
-3.95179673813153));
#296939=CARTESIAN_POINT('Ctrl Pts',(-12.1623797632104,113.712499999556,
2.97892388940601E-15));
#296940=CARTESIAN_POINT('Ctrl Pts',(-12.1623797632104,113.862499999555,
3.95179673813154));
#296941=CARTESIAN_POINT('Ctrl Pts',(-9.83957192047915,114.012499999554,
7.14886745759543));
#296942=CARTESIAN_POINT('Ctrl Pts',(-7.51676407774793,114.162499999554,
10.3459381770593));
#296943=CARTESIAN_POINT('Ctrl Pts',(-3.758382038874,114.312499999553,11.5671105274575));
#296944=CARTESIAN_POINT('Ctrl Pts',(-7.60477614674932E-14,114.462499999553,
12.7882828778556));
#296945=CARTESIAN_POINT('Ctrl Pts',(3.75838203887385,114.612499999552,11.5671105274575));
#296946=CARTESIAN_POINT('Ctrl Pts',(7.51676407774778,114.762499999551,10.3459381770593));
#296947=CARTESIAN_POINT('Ctrl Pts',(9.839571920479,114.912499999551,7.14886745759543));
#296948=CARTESIAN_POINT('Ctrl Pts',(12.1623797632102,115.06249999955,3.95179673813153));
#296949=CARTESIAN_POINT('Ctrl Pts',(12.1623797632102,115.21249999955,-1.489461944703E-15));
#296950=CARTESIAN_POINT('Ctrl Pts',(12.1623797632102,115.362499999549,-3.95179673813154));
#296951=CARTESIAN_POINT('Ctrl Pts',(9.839571920479,115.512499999548,-7.14886745759543));
#296952=CARTESIAN_POINT('Ctrl Pts',(7.51676407774778,115.662499999548,-10.3459381770593));
#296953=CARTESIAN_POINT('Ctrl Pts',(3.75838203887385,115.812499999547,-11.5671105274575));
#296954=CARTESIAN_POINT('Ctrl Pts',(-8.00438420419154E-14,115.962499999547,
-12.7882828778556));
#296955=CARTESIAN_POINT('Ctrl Pts',(-3.75838203887401,116.112499999546,
-11.5671105274575));
#296956=CARTESIAN_POINT('Ctrl Pts',(-7.51676407774794,116.262499999545,
-10.3459381770593));
#296957=CARTESIAN_POINT('Ctrl Pts',(-9.83957192047916,116.412499999545,
-7.14886745759543));
#296958=CARTESIAN_POINT('Ctrl Pts',(-12.1623797632104,116.562499999544,
-3.95179673813153));
#296959=CARTESIAN_POINT('Ctrl Pts',(-12.1623797632104,116.712499999544,
2.97892388940601E-15));
#296960=CARTESIAN_POINT('Ctrl Pts',(-12.1623797632104,116.862499999543,
3.95179673813154));
#296961=CARTESIAN_POINT('Ctrl Pts',(-9.83957192047915,117.012499999542,
7.14886745759543));
#296962=CARTESIAN_POINT('Ctrl Pts',(-7.51676407774793,117.162499999542,
10.3459381770593));
#296963=CARTESIAN_POINT('Ctrl Pts',(-3.75838203887401,117.312499999541,
11.5671105274575));
#296964=CARTESIAN_POINT('Ctrl Pts',(-7.7775470739155E-14,117.462499999541,
12.7882828778556));
#296965=CARTESIAN_POINT('Ctrl Pts',(3.75838203887385,117.61249999954,11.5671105274575));
#296966=CARTESIAN_POINT('Ctrl Pts',(7.51676407774778,117.762499999539,10.3459381770593));
#296967=CARTESIAN_POINT('Ctrl Pts',(9.839571920479,117.912499999539,7.14886745759543));
#296968=CARTESIAN_POINT('Ctrl Pts',(12.1623797632102,118.062499999538,3.95179673813153));
#296969=CARTESIAN_POINT('Ctrl Pts',(12.1623797632102,118.212499999538,-1.489461944703E-15));
#296970=CARTESIAN_POINT('Ctrl Pts',(12.1623797632102,118.362499999537,-3.95179673813154));
#296971=CARTESIAN_POINT('Ctrl Pts',(9.83957192047899,118.512499999536,-7.14886745759543));
#296972=CARTESIAN_POINT('Ctrl Pts',(7.51676407774778,118.662499999536,-10.3459381770593));
#296973=CARTESIAN_POINT('Ctrl Pts',(3.75838203887385,118.812499999535,-11.5671105274575));
#296974=CARTESIAN_POINT('Ctrl Pts',(-8.17715513135773E-14,118.962499999535,
-12.7882828778556));
#296975=CARTESIAN_POINT('Ctrl Pts',(-3.75838203887401,119.112499999534,
-11.5671105274575));
#296976=CARTESIAN_POINT('Ctrl Pts',(-7.51676407774794,119.262499999533,
-10.3459381770593));
#296977=CARTESIAN_POINT('Ctrl Pts',(-9.83957192047916,119.412499999533,
-7.14886745759543));
#296978=CARTESIAN_POINT('Ctrl Pts',(-12.1623797632104,119.562499999532,
-3.95179673813153));
#296979=CARTESIAN_POINT('Ctrl Pts',(-12.1623797632104,119.712499999532,
2.97892388940601E-15));
#296980=CARTESIAN_POINT('Ctrl Pts',(-12.1623797632104,119.862499999531,
3.95179673813154));
#296981=CARTESIAN_POINT('Ctrl Pts',(-9.83957192047916,120.01249999953,7.14886745759543));
#296982=CARTESIAN_POINT('Ctrl Pts',(-7.51676407774794,120.16249999953,10.3459381770593));
#296983=CARTESIAN_POINT('Ctrl Pts',(-3.75838203887401,120.312499999529,
11.5671105274575));
#296984=CARTESIAN_POINT('Ctrl Pts',(-7.95031800108169E-14,120.462499999529,
12.7882828778556));
#296985=CARTESIAN_POINT('Ctrl Pts',(3.75838203887385,120.612499999528,11.5671105274575));
#296986=CARTESIAN_POINT('Ctrl Pts',(7.51676407774778,120.762499999527,10.3459381770593));
#296987=CARTESIAN_POINT('Ctrl Pts',(9.83957192047899,120.912499999527,7.14886745759543));
#296988=CARTESIAN_POINT('Ctrl Pts',(12.1623797632102,121.062499999526,3.95179673813153));
#296989=CARTESIAN_POINT('Ctrl Pts',(12.1623797632102,121.212499999526,-1.489461944703E-15));
#296990=CARTESIAN_POINT('Ctrl Pts',(12.1623797632102,121.362499999525,-3.95179673813154));
#296991=CARTESIAN_POINT('Ctrl Pts',(9.83957192047899,121.512499999524,-7.14886745759543));
#296992=CARTESIAN_POINT('Ctrl Pts',(7.51676407774777,121.662499999524,-10.3459381770593));
#296993=CARTESIAN_POINT('Ctrl Pts',(3.75838203887385,121.812499999523,-11.5671105274575));
#296994=CARTESIAN_POINT('Ctrl Pts',(-8.34992605852391E-14,121.962499999523,
-12.7882828778556));
#296995=CARTESIAN_POINT('Ctrl Pts',(-3.75838203887401,122.112499999522,
-11.5671105274575));
#296996=CARTESIAN_POINT('Ctrl Pts',(-7.51676407774794,122.262499999521,
-10.3459381770593));
#296997=CARTESIAN_POINT('Ctrl Pts',(-9.83957192047916,122.412499999521,
-7.14886745759543));
#296998=CARTESIAN_POINT('Ctrl Pts',(-12.1623797632104,122.56249999952,-3.95179673813153));
#296999=CARTESIAN_POINT('Ctrl Pts',(-12.1623797632104,122.71249999952,2.97892388940601E-15));
#297000=CARTESIAN_POINT('Ctrl Pts',(-12.1623797632104,122.862499999519,
3.95179673813154));
#297001=CARTESIAN_POINT('Ctrl Pts',(-9.83957192047916,123.012499999518,
7.14886745759543));
#297002=CARTESIAN_POINT('Ctrl Pts',(-7.51676407774794,123.162499999518,
10.3459381770593));
#297003=CARTESIAN_POINT('Ctrl Pts',(-3.75838203887401,123.312499999517,
11.5671105274575));
#297004=CARTESIAN_POINT('Ctrl Pts',(-8.12308892824787E-14,123.462499999517,
12.7882828778556));
#297005=CARTESIAN_POINT('Ctrl Pts',(3.75838203887385,123.612499999516,11.5671105274575));
#297006=CARTESIAN_POINT('Ctrl Pts',(7.51676407774778,123.762499999515,10.3459381770593));
#297007=CARTESIAN_POINT('Ctrl Pts',(9.83957192047899,123.912499999515,7.14886745759543));
#297008=CARTESIAN_POINT('Ctrl Pts',(12.1623797632102,124.062499999514,3.95179673813153));
#297009=CARTESIAN_POINT('Ctrl Pts',(12.1623797632102,124.212499999514,-1.489461944703E-15));
#297010=CARTESIAN_POINT('Ctrl Pts',(12.1623797632102,124.362499999513,-3.95179673813154));
#297011=CARTESIAN_POINT('Ctrl Pts',(9.83957192047899,124.512499999512,-7.14886745759543));
#297012=CARTESIAN_POINT('Ctrl Pts',(7.51676407774777,124.662499999512,-10.3459381770593));
#297013=CARTESIAN_POINT('Ctrl Pts',(3.75838203887384,124.812499999511,-11.5671105274575));
#297014=CARTESIAN_POINT('Ctrl Pts',(-8.52269698569009E-14,124.962499999511,
-12.7882828778556));
#297015=CARTESIAN_POINT('Ctrl Pts',(-3.75838203887401,125.11249999951,-11.5671105274575));
#297016=CARTESIAN_POINT('Ctrl Pts',(-7.51676407774794,125.262499999509,
-10.3459381770593));
#297017=CARTESIAN_POINT('Ctrl Pts',(-9.83957192047916,125.412499999509,
-7.14886745759543));
#297018=CARTESIAN_POINT('Ctrl Pts',(-12.1623797632104,125.562499999508,
-3.95179673813153));
#297019=CARTESIAN_POINT('Ctrl Pts',(-12.1623797632104,125.712499999508,
2.97892388940601E-15));
#297020=CARTESIAN_POINT('Ctrl Pts',(-12.1623797632104,125.862499999507,
3.95179673813154));
#297021=CARTESIAN_POINT('Ctrl Pts',(-9.83957192047916,126.012499999506,
7.14886745759543));
#297022=CARTESIAN_POINT('Ctrl Pts',(-7.51676407774794,126.162499999506,
10.3459381770593));
#297023=CARTESIAN_POINT('Ctrl Pts',(-3.75838203887401,126.312499999505,
11.5671105274575));
#297024=CARTESIAN_POINT('Ctrl Pts',(-8.29585985541405E-14,126.462499999505,
12.7882828778556));
#297025=CARTESIAN_POINT('Ctrl Pts',(3.75838203887385,126.612499999504,11.5671105274575));
#297026=CARTESIAN_POINT('Ctrl Pts',(7.51676407774777,126.762499999503,10.3459381770593));
#297027=CARTESIAN_POINT('Ctrl Pts',(9.83957192047899,126.912499999503,7.14886745759543));
#297028=CARTESIAN_POINT('Ctrl Pts',(12.1623797632102,127.062499999502,3.95179673813153));
#297029=CARTESIAN_POINT('Ctrl Pts',(12.1623797632102,127.212499999502,-1.489461944703E-15));
#297030=CARTESIAN_POINT('Ctrl Pts',(12.1623797632102,127.362499999501,-3.95179673813154));
#297031=CARTESIAN_POINT('Ctrl Pts',(9.83957192047899,127.5124999995,-7.14886745759543));
#297032=CARTESIAN_POINT('Ctrl Pts',(7.51676407774777,127.6624999995,-10.3459381770593));
#297033=CARTESIAN_POINT('Ctrl Pts',(3.75838203887384,127.812499999499,-11.5671105274575));
#297034=CARTESIAN_POINT('Ctrl Pts',(-8.69546791285628E-14,127.962499999499,
-12.7882828778556));
#297035=CARTESIAN_POINT('Ctrl Pts',(-3.75838203887402,128.112499999498,
-11.5671105274575));
#297036=CARTESIAN_POINT('Ctrl Pts',(-7.51676407774795,128.262499999497,
-10.3459381770593));
#297037=CARTESIAN_POINT('Ctrl Pts',(-9.83957192047916,128.412499999497,
-7.14886745759543));
#297038=CARTESIAN_POINT('Ctrl Pts',(-12.1623797632104,128.562499999496,
-3.95179673813153));
#297039=CARTESIAN_POINT('Ctrl Pts',(-12.1623797632104,128.712499999496,
2.97892388940601E-15));
#297040=CARTESIAN_POINT('Ctrl Pts',(-12.1623797632104,128.862499999495,
3.95179673813154));
#297041=CARTESIAN_POINT('Ctrl Pts',(-9.83957192047916,129.012499999494,
7.14886745759543));
#297042=CARTESIAN_POINT('Ctrl Pts',(-7.51676407774794,129.162499999494,
10.3459381770593));
#297043=CARTESIAN_POINT('Ctrl Pts',(-3.75838203887401,129.312499999493,
11.5671105274575));
#297044=CARTESIAN_POINT('Ctrl Pts',(-8.46863078258024E-14,129.462499999493,
12.7882828778556));
#297045=CARTESIAN_POINT('Ctrl Pts',(3.75838203887384,129.612499999492,11.5671105274575));
#297046=CARTESIAN_POINT('Ctrl Pts',(7.51676407774777,129.762499999491,10.3459381770593));
#297047=CARTESIAN_POINT('Ctrl Pts',(9.83957192047899,129.912499999491,7.14886745759543));
#297048=CARTESIAN_POINT('Ctrl Pts',(12.1623797632102,130.06249999949,3.95179673813153));
#297049=CARTESIAN_POINT('Ctrl Pts',(12.1623797632102,130.21249999949,-1.489461944703E-15));
#297050=CARTESIAN_POINT('Ctrl Pts',(12.1623797632102,130.362499999489,-3.95179673813154));
#297051=CARTESIAN_POINT('Ctrl Pts',(9.83957192047899,130.512499999488,-7.14886745759543));
#297052=CARTESIAN_POINT('Ctrl Pts',(7.51676407774777,130.662499999488,-10.3459381770593));
#297053=CARTESIAN_POINT('Ctrl Pts',(3.75838203887384,130.812499999487,-11.5671105274575));
#297054=CARTESIAN_POINT('Ctrl Pts',(-8.86823884002247E-14,130.962499999487,
-12.7882828778556));
#297055=CARTESIAN_POINT('Ctrl Pts',(-3.75838203887402,131.112499999486,
-11.5671105274575));
#297056=CARTESIAN_POINT('Ctrl Pts',(-7.51676407774795,131.262499999485,
-10.3459381770593));
#297057=CARTESIAN_POINT('Ctrl Pts',(-9.83957192047916,131.412499999485,
-7.14886745759543));
#297058=CARTESIAN_POINT('Ctrl Pts',(-12.1623797632104,131.562499999484,
-3.95179673813153));
#297059=CARTESIAN_POINT('Ctrl Pts',(-12.1623797632104,131.712499999484,
2.97892388940601E-15));
#297060=CARTESIAN_POINT('Ctrl Pts',(-12.1623797632104,131.862499999483,
3.95179673813154));
#297061=CARTESIAN_POINT('Ctrl Pts',(-9.83957192047916,132.012499999482,
7.14886745759543));
#297062=CARTESIAN_POINT('Ctrl Pts',(-7.51676407774795,132.162499999482,
10.3459381770593));
#297063=CARTESIAN_POINT('Ctrl Pts',(-3.75838203887402,132.312499999481,
11.5671105274575));
#297064=CARTESIAN_POINT('Ctrl Pts',(-8.64140170974642E-14,132.462499999481,
12.7882828778556));
#297065=CARTESIAN_POINT('Ctrl Pts',(3.75838203887384,132.61249999948,11.5671105274575));
#297066=CARTESIAN_POINT('Ctrl Pts',(7.51676407774777,132.762499999479,10.3459381770593));
#297067=CARTESIAN_POINT('Ctrl Pts',(9.83957192047899,132.912499999479,7.14886745759543));
#297068=CARTESIAN_POINT('Ctrl Pts',(12.1623797632102,133.062499999478,3.95179673813153));
#297069=CARTESIAN_POINT('Ctrl Pts',(12.1623797632102,133.212499999478,-1.489461944703E-15));
#297070=CARTESIAN_POINT('Ctrl Pts',(12.1623797632102,133.362499999477,-3.95179673813154));
#297071=CARTESIAN_POINT('Ctrl Pts',(9.83957192047898,133.512499999476,-7.14886745759543));
#297072=CARTESIAN_POINT('Ctrl Pts',(7.51676407774777,133.662499999476,-10.3459381770593));
#297073=CARTESIAN_POINT('Ctrl Pts',(3.75838203887384,133.812499999475,-11.5671105274575));
#297074=CARTESIAN_POINT('Ctrl Pts',(-9.04100976718865E-14,133.962499999475,
-12.7882828778556));
#297075=CARTESIAN_POINT('Ctrl Pts',(-3.75838203887402,134.112499999474,
-11.5671105274575));
#297076=CARTESIAN_POINT('Ctrl Pts',(-7.51676407774795,134.262499999473,
-10.3459381770593));
#297077=CARTESIAN_POINT('Ctrl Pts',(-9.83957192047917,134.412499999473,
-7.14886745759543));
#297078=CARTESIAN_POINT('Ctrl Pts',(-12.1623797632104,134.562499999472,
-3.95179673813153));
#297079=CARTESIAN_POINT('Ctrl Pts',(-12.1623797632104,134.712499999472,
2.97892388940601E-15));
#297080=CARTESIAN_POINT('Ctrl Pts',(-12.1623797632104,134.862499999471,
3.95179673813154));
#297081=CARTESIAN_POINT('Ctrl Pts',(-9.83957192047916,135.01249999947,7.14886745759543));
#297082=CARTESIAN_POINT('Ctrl Pts',(-7.51676407774795,135.16249999947,10.3459381770593));
#297083=CARTESIAN_POINT('Ctrl Pts',(-3.75838203887402,135.312499999469,
11.5671105274575));
#297084=CARTESIAN_POINT('Ctrl Pts',(-8.8141726369126E-14,135.462499999469,
12.7882828778556));
#297085=CARTESIAN_POINT('Ctrl Pts',(3.75838203887384,135.612499999468,11.5671105274575));
#297086=CARTESIAN_POINT('Ctrl Pts',(7.51676407774777,135.762499999467,10.3459381770593));
#297087=CARTESIAN_POINT('Ctrl Pts',(9.83957192047898,135.912499999467,7.14886745759543));
#297088=CARTESIAN_POINT('Ctrl Pts',(12.1623797632102,136.062499999466,3.95179673813153));
#297089=CARTESIAN_POINT('Ctrl Pts',(12.1623797632102,136.212499999466,-1.489461944703E-15));
#297090=CARTESIAN_POINT('Ctrl Pts',(12.1623797632102,136.362499999465,-3.95179673813154));
#297091=CARTESIAN_POINT('Ctrl Pts',(9.83957192047898,136.512499999464,-7.14886745759543));
#297092=CARTESIAN_POINT('Ctrl Pts',(7.51676407774777,136.662499999464,-10.3459381770593));
#297093=CARTESIAN_POINT('Ctrl Pts',(3.75838203887384,136.812499999463,-11.5671105274575));
#297094=CARTESIAN_POINT('Ctrl Pts',(-9.21378069435483E-14,136.962499999463,
-12.7882828778556));
#297095=CARTESIAN_POINT('Ctrl Pts',(-3.75838203887402,137.112499999462,
-11.5671105274575));
#297096=CARTESIAN_POINT('Ctrl Pts',(-7.51676407774795,137.262499999461,
-10.3459381770593));
#297097=CARTESIAN_POINT('Ctrl Pts',(-9.83957192047917,137.412499999461,
-7.14886745759543));
#297098=CARTESIAN_POINT('Ctrl Pts',(-12.1623797632104,137.56249999946,-3.95179673813153));
#297099=CARTESIAN_POINT('Ctrl Pts',(-12.1623797632104,137.71249999946,2.97892388940601E-15));
#297100=CARTESIAN_POINT('Ctrl Pts',(-12.1623797632104,137.862499999459,
3.95179673813154));
#297101=CARTESIAN_POINT('Ctrl Pts',(-9.83957192047917,138.012499999458,
7.14886745759543));
#297102=CARTESIAN_POINT('Ctrl Pts',(-7.51676407774795,138.162499999458,
10.3459381770593));
#297103=CARTESIAN_POINT('Ctrl Pts',(-3.75838203887402,138.312499999457,
11.5671105274575));
#297104=CARTESIAN_POINT('Ctrl Pts',(-8.98694356407879E-14,138.462499999457,
12.7882828778556));
#297105=CARTESIAN_POINT('Ctrl Pts',(3.75838203887384,138.612499999456,11.5671105274575));
#297106=CARTESIAN_POINT('Ctrl Pts',(7.51676407774777,138.762499999455,10.3459381770593));
#297107=CARTESIAN_POINT('Ctrl Pts',(9.83957192047898,138.912499999455,7.14886745759543));
#297108=CARTESIAN_POINT('Ctrl Pts',(12.1623797632102,139.062499999454,3.95179673813153));
#297109=CARTESIAN_POINT('Ctrl Pts',(12.1623797632102,139.212499999454,-1.489461944703E-15));
#297110=CARTESIAN_POINT('Ctrl Pts',(12.1623797632102,139.362499999453,-3.95179673813154));
#297111=CARTESIAN_POINT('Ctrl Pts',(9.83957192047898,139.512499999452,-7.14886745759543));
#297112=CARTESIAN_POINT('Ctrl Pts',(7.51676407774776,139.662499999452,-10.3459381770593));
#297113=CARTESIAN_POINT('Ctrl Pts',(3.75838203887384,139.812499999451,-11.5671105274575));
#297114=CARTESIAN_POINT('Ctrl Pts',(-9.38655162152102E-14,139.962499999451,
-12.7882828778556));
#297115=CARTESIAN_POINT('Ctrl Pts',(-3.75838203887402,140.11249999945,-11.5671105274575));
#297116=CARTESIAN_POINT('Ctrl Pts',(-7.51676407774795,140.262499999449,
-10.3459381770593));
#297117=CARTESIAN_POINT('Ctrl Pts',(-9.83957192047917,140.412499999449,
-7.14886745759543));
#297118=CARTESIAN_POINT('Ctrl Pts',(-12.1623797632104,140.562499999448,
-3.95179673813153));
#297119=CARTESIAN_POINT('Ctrl Pts',(-12.1623797632104,140.712499999448,
2.97892388940601E-15));
#297120=CARTESIAN_POINT('Ctrl Pts',(-12.1623797632104,140.862499999447,
3.95179673813154));
#297121=CARTESIAN_POINT('Ctrl Pts',(-9.83957192047917,141.012499999446,
7.14886745759543));
#297122=CARTESIAN_POINT('Ctrl Pts',(-7.51676407774795,141.162499999446,
10.3459381770593));
#297123=CARTESIAN_POINT('Ctrl Pts',(-3.75838203887402,141.312499999445,
11.5671105274575));
#297124=CARTESIAN_POINT('Ctrl Pts',(-9.15971449124498E-14,141.462499999445,
12.7882828778556));
#297125=CARTESIAN_POINT('Ctrl Pts',(3.75838203887384,141.612499999444,11.5671105274575));
#297126=CARTESIAN_POINT('Ctrl Pts',(7.51676407774777,141.762499999443,10.3459381770593));
#297127=CARTESIAN_POINT('Ctrl Pts',(9.83957192047898,141.912499999443,7.14886745759543));
#297128=CARTESIAN_POINT('Ctrl Pts',(12.1623797632102,142.062499999442,3.95179673813153));
#297129=CARTESIAN_POINT('Ctrl Pts',(12.1623797632102,142.212499999442,-1.489461944703E-15));
#297130=CARTESIAN_POINT('Ctrl Pts',(12.1623797632102,142.362499999441,-3.95179673813154));
#297131=CARTESIAN_POINT('Ctrl Pts',(9.83957192047898,142.51249999944,-7.14886745759543));
#297132=CARTESIAN_POINT('Ctrl Pts',(7.51676407774776,142.66249999944,-10.3459381770593));
#297133=CARTESIAN_POINT('Ctrl Pts',(3.75838203887383,142.812499999439,-11.5671105274575));
#297134=CARTESIAN_POINT('Ctrl Pts',(-9.5593225486872E-14,142.962499999439,
-12.7882828778556));
#297135=CARTESIAN_POINT('Ctrl Pts',(-3.75838203887402,143.112499999438,
-11.5671105274575));
#297136=CARTESIAN_POINT('Ctrl Pts',(-7.51676407774795,143.262499999437,
-10.3459381770593));
#297137=CARTESIAN_POINT('Ctrl Pts',(-9.83957192047917,143.412499999437,
-7.14886745759543));
#297138=CARTESIAN_POINT('Ctrl Pts',(-12.1623797632104,143.562499999436,
-3.95179673813153));
#297139=CARTESIAN_POINT('Ctrl Pts',(-12.1623797632104,143.712499999436,
2.97892388940601E-15));
#297140=CARTESIAN_POINT('Ctrl Pts',(-12.1623797632104,143.862499999435,
3.95179673813154));
#297141=CARTESIAN_POINT('Ctrl Pts',(-9.83957192047917,144.012499999434,
7.14886745759543));
#297142=CARTESIAN_POINT('Ctrl Pts',(-7.51676407774795,144.162499999434,
10.3459381770593));
#297143=CARTESIAN_POINT('Ctrl Pts',(-3.75838203887402,144.312499999433,
11.5671105274575));
#297144=CARTESIAN_POINT('Ctrl Pts',(-9.33248541841116E-14,144.462499999433,
12.7882828778556));
#297145=CARTESIAN_POINT('Ctrl Pts',(3.75838203887384,144.612499999432,11.5671105274575));
#297146=CARTESIAN_POINT('Ctrl Pts',(7.51676407774776,144.762499999431,10.3459381770593));
#297147=CARTESIAN_POINT('Ctrl Pts',(9.83957192047898,144.912499999431,7.14886745759543));
#297148=CARTESIAN_POINT('Ctrl Pts',(12.1623797632102,145.06249999943,3.95179673813153));
#297149=CARTESIAN_POINT('Ctrl Pts',(12.1623797632102,145.21249999943,-1.489461944703E-15));
#297150=CARTESIAN_POINT('Ctrl Pts',(12.1623797632102,145.362499999429,-3.95179673813154));
#297151=CARTESIAN_POINT('Ctrl Pts',(9.83957192047898,145.512499999428,-7.14886745759543));
#297152=CARTESIAN_POINT('Ctrl Pts',(7.51676407774776,145.662499999428,-10.3459381770593));
#297153=CARTESIAN_POINT('Ctrl Pts',(3.75838203887383,145.812499999427,-11.5671105274575));
#297154=CARTESIAN_POINT('Ctrl Pts',(-9.73209347585338E-14,145.962499999427,
-12.7882828778556));
#297155=CARTESIAN_POINT('Ctrl Pts',(-3.75838203887403,146.112499999426,
-11.5671105274575));
#297156=CARTESIAN_POINT('Ctrl Pts',(-7.51676407774795,146.262499999425,
-10.3459381770593));
#297157=CARTESIAN_POINT('Ctrl Pts',(-9.83957192047917,146.412499999425,
-7.14886745759543));
#297158=CARTESIAN_POINT('Ctrl Pts',(-12.1623797632104,146.562499999424,
-3.95179673813153));
#297159=CARTESIAN_POINT('Ctrl Pts',(-12.1623797632104,146.712499999424,
2.97892388940601E-15));
#297160=CARTESIAN_POINT('Ctrl Pts',(-12.1623797632104,146.862499999423,
3.95179673813154));
#297161=CARTESIAN_POINT('Ctrl Pts',(-9.83957192047917,147.012499999422,
7.14886745759543));
#297162=CARTESIAN_POINT('Ctrl Pts',(-7.51676407774795,147.162499999422,
10.3459381770593));
#297163=CARTESIAN_POINT('Ctrl Pts',(-3.75838203887402,147.312499999421,
11.5671105274575));
#297164=CARTESIAN_POINT('Ctrl Pts',(-9.50525634557734E-14,147.462499999421,
12.7882828778556));
#297165=CARTESIAN_POINT('Ctrl Pts',(3.75838203887383,147.61249999942,11.5671105274575));
#297166=CARTESIAN_POINT('Ctrl Pts',(7.51676407774776,147.762499999419,10.3459381770593));
#297167=CARTESIAN_POINT('Ctrl Pts',(9.83957192047898,147.912499999419,7.14886745759543));
#297168=CARTESIAN_POINT('Ctrl Pts',(12.1623797632102,148.062499999418,3.95179673813153));
#297169=CARTESIAN_POINT('Ctrl Pts',(12.1623797632102,148.212499999418,-1.489461944703E-15));
#297170=CARTESIAN_POINT('Ctrl Pts',(12.1623797632102,148.362499999417,-3.95179673813154));
#297171=CARTESIAN_POINT('Ctrl Pts',(9.83957192047898,148.512499999416,-7.14886745759543));
#297172=CARTESIAN_POINT('Ctrl Pts',(7.51676407774776,148.662499999416,-10.3459381770593));
#297173=CARTESIAN_POINT('Ctrl Pts',(3.75838203887383,148.812499999415,-11.5671105274575));
#297174=CARTESIAN_POINT('Ctrl Pts',(-9.90486440301957E-14,148.962499999415,
-12.7882828778556));
#297175=CARTESIAN_POINT('Ctrl Pts',(-3.75838203887403,149.112499999414,
-11.5671105274575));
#297176=CARTESIAN_POINT('Ctrl Pts',(-7.51676407774795,149.262499999413,
-10.3459381770593));
#297177=CARTESIAN_POINT('Ctrl Pts',(-9.83957192047917,149.412499999413,
-7.14886745759543));
#297178=CARTESIAN_POINT('Ctrl Pts',(-12.1623797632104,149.562499999412,
-3.95179673813153));
#297179=CARTESIAN_POINT('Ctrl Pts',(-12.1623797632104,149.712499999412,
2.97892388940601E-15));
#297180=CARTESIAN_POINT('Ctrl Pts',(-12.1623797632104,149.862499999411,
3.95179673813154));
#297181=CARTESIAN_POINT('Ctrl Pts',(-9.83957192047917,150.01249999941,7.14886745759543));
#297182=CARTESIAN_POINT('Ctrl Pts',(-7.51676407774795,150.16249999941,10.3459381770593));
#297183=CARTESIAN_POINT('Ctrl Pts',(-3.75838203887403,150.312499999409,
11.5671105274575));
#297184=CARTESIAN_POINT('Ctrl Pts',(-9.67802727274353E-14,150.462499999409,
12.7882828778556));
#297185=CARTESIAN_POINT('Ctrl Pts',(3.75838203887383,150.612499999408,11.5671105274575));
#297186=CARTESIAN_POINT('Ctrl Pts',(7.51676407774776,150.762499999407,10.3459381770593));
#297187=CARTESIAN_POINT('Ctrl Pts',(9.83957192047898,150.912499999407,7.14886745759543));
#297188=CARTESIAN_POINT('Ctrl Pts',(12.1623797632102,151.062499999406,3.95179673813153));
#297189=CARTESIAN_POINT('Ctrl Pts',(12.1623797632102,151.212499999406,-1.489461944703E-15));
#297190=CARTESIAN_POINT('Ctrl Pts',(12.1623797632102,151.362499999405,-3.95179673813154));
#297191=CARTESIAN_POINT('Ctrl Pts',(9.83957192047897,151.512499999404,-7.14886745759543));
#297192=CARTESIAN_POINT('Ctrl Pts',(7.51676407774776,151.662499999404,-10.3459381770593));
#297193=CARTESIAN_POINT('Ctrl Pts',(3.75838203887383,151.812499999403,-11.5671105274575));
#297194=CARTESIAN_POINT('Ctrl Pts',(-1.00776353301858E-13,151.962499999403,
-12.7882828778556));
#297195=CARTESIAN_POINT('Ctrl Pts',(-3.75838203887403,152.112499999402,
-11.5671105274575));
#297196=CARTESIAN_POINT('Ctrl Pts',(-10.0514428414942,-2.06874999998125,
2.46189346052968E-15));
#297197=CARTESIAN_POINT('Ctrl Pts',(-10.0514428414942,-1.91874999998185,
3.26591175476071));
#297198=CARTESIAN_POINT('Ctrl Pts',(-8.1317880767572,-1.76874999998245,
5.90808986649102));
#297199=CARTESIAN_POINT('Ctrl Pts',(-6.21213331202023,-1.61874999998305,
8.55026797822134));
#297200=CARTESIAN_POINT('Ctrl Pts',(-3.10606665601012,-1.46874999998365,
9.5594902125713));
#297201=CARTESIAN_POINT('Ctrl Pts',(-9.77671023785295E-15,-1.31874999998425,
10.5687124469213));
#297202=CARTESIAN_POINT('Ctrl Pts',(3.1060666560101,-1.16874999998485,9.5594902125713));
#297203=CARTESIAN_POINT('Ctrl Pts',(6.21213331202021,-1.01874999998544,
8.55026797822134));
#297204=CARTESIAN_POINT('Ctrl Pts',(8.13178807675718,-0.868749999986043,
5.90808986649102));
#297205=CARTESIAN_POINT('Ctrl Pts',(10.0514428414942,-0.718749999986641,
3.2659117547607));
#297206=CARTESIAN_POINT('Ctrl Pts',(10.0514428414942,-0.568749999987242,
-1.23094673026484E-15));
#297207=CARTESIAN_POINT('Ctrl Pts',(10.0514428414942,-0.418749999987842,
-3.26591175476071));
#297208=CARTESIAN_POINT('Ctrl Pts',(8.13178807675718,-0.268749999988443,
-5.90808986649102));
#297209=CARTESIAN_POINT('Ctrl Pts',(6.2121333120202,-0.118749999989044,
-8.55026797822134));
#297210=CARTESIAN_POINT('Ctrl Pts',(3.10606665601009,0.0312500000103543,
-9.5594902125713));
#297211=CARTESIAN_POINT('Ctrl Pts',(-1.322915284753E-14,0.181250000009752,
-10.5687124469213));
#297212=CARTESIAN_POINT('Ctrl Pts',(-3.10606665601012,0.331250000009151,
-9.5594902125713));
#297213=CARTESIAN_POINT('Ctrl Pts',(-6.21213331202023,0.481250000008549,
-8.55026797822134));
#297214=CARTESIAN_POINT('Ctrl Pts',(-8.1317880767572,0.631250000007948,
-5.90808986649102));
#297215=CARTESIAN_POINT('Ctrl Pts',(-10.0514428414942,0.781250000007346,
-3.2659117547607));
#297216=CARTESIAN_POINT('Ctrl Pts',(-10.0514428414942,0.931250000006746,
2.46189346052968E-15));
#297217=CARTESIAN_POINT('Ctrl Pts',(-10.0514428414942,1.08125000000615,
3.26591175476071));
#297218=CARTESIAN_POINT('Ctrl Pts',(-8.1317880767572,1.23125000000555,5.90808986649102));
#297219=CARTESIAN_POINT('Ctrl Pts',(-6.21213331202023,1.38125000000495,
8.55026797822134));
#297220=CARTESIAN_POINT('Ctrl Pts',(-3.10606665601012,1.53125000000435,
9.5594902125713));
#297221=CARTESIAN_POINT('Ctrl Pts',(-1.15044195095148E-14,1.68125000000375,
10.5687124469213));
#297222=CARTESIAN_POINT('Ctrl Pts',(3.1060666560101,1.83125000000315,9.5594902125713));
#297223=CARTESIAN_POINT('Ctrl Pts',(6.2121333120202,1.98125000000256,8.55026797822134));
#297224=CARTESIAN_POINT('Ctrl Pts',(8.13178807675718,2.13125000000196,5.90808986649102));
#297225=CARTESIAN_POINT('Ctrl Pts',(10.0514428414942,2.28125000000136,3.2659117547607));
#297226=CARTESIAN_POINT('Ctrl Pts',(10.0514428414942,2.43125000000076,-1.23094673026484E-15));
#297227=CARTESIAN_POINT('Ctrl Pts',(10.0514428414942,2.58125000000016,-3.26591175476071));
#297228=CARTESIAN_POINT('Ctrl Pts',(8.13178807675718,2.73124999999956,-5.90808986649102));
#297229=CARTESIAN_POINT('Ctrl Pts',(6.2121333120202,2.88124999999896,-8.55026797822134));
#297230=CARTESIAN_POINT('Ctrl Pts',(3.10606665601009,3.03124999999835,-9.5594902125713));
#297231=CARTESIAN_POINT('Ctrl Pts',(-1.49568621191919E-14,3.18124999999775,
-10.5687124469213));
#297232=CARTESIAN_POINT('Ctrl Pts',(-3.10606665601012,3.33124999999715,
-9.5594902125713));
#297233=CARTESIAN_POINT('Ctrl Pts',(-6.21213331202023,3.48124999999655,
-8.55026797822134));
#297234=CARTESIAN_POINT('Ctrl Pts',(-8.13178807675721,3.63124999999595,
-5.90808986649102));
#297235=CARTESIAN_POINT('Ctrl Pts',(-10.0514428414942,3.78124999999535,
-3.2659117547607));
#297236=CARTESIAN_POINT('Ctrl Pts',(-10.0514428414942,3.93124999999475,
2.46189346052968E-15));
#297237=CARTESIAN_POINT('Ctrl Pts',(-10.0514428414942,4.08124999999415,
3.26591175476071));
#297238=CARTESIAN_POINT('Ctrl Pts',(-8.13178807675721,4.23124999999355,
5.90808986649102));
#297239=CARTESIAN_POINT('Ctrl Pts',(-6.21213331202023,4.38124999999295,
8.55026797822134));
#297240=CARTESIAN_POINT('Ctrl Pts',(-3.10606665601012,4.53124999999235,
9.5594902125713));
#297241=CARTESIAN_POINT('Ctrl Pts',(-1.32321287811766E-14,4.68124999999175,
10.5687124469213));
#297242=CARTESIAN_POINT('Ctrl Pts',(3.10606665601009,4.83124999999115,9.5594902125713));
#297243=CARTESIAN_POINT('Ctrl Pts',(6.2121333120202,4.98124999999055,8.55026797822134));
#297244=CARTESIAN_POINT('Ctrl Pts',(8.13178807675718,5.13124999998996,5.90808986649102));
#297245=CARTESIAN_POINT('Ctrl Pts',(10.0514428414942,5.28124999998936,3.2659117547607));
#297246=CARTESIAN_POINT('Ctrl Pts',(10.0514428414941,5.43124999998876,-1.23094673026484E-15));
#297247=CARTESIAN_POINT('Ctrl Pts',(10.0514428414941,5.58124999998816,-3.26591175476071));
#297248=CARTESIAN_POINT('Ctrl Pts',(8.13178807675717,5.73124999998756,-5.90808986649102));
#297249=CARTESIAN_POINT('Ctrl Pts',(6.2121333120202,5.88124999998695,-8.55026797822134));
#297250=CARTESIAN_POINT('Ctrl Pts',(3.10606665601009,6.03124999998635,-9.5594902125713));
#297251=CARTESIAN_POINT('Ctrl Pts',(-1.66845713908537E-14,6.18124999998575,
-10.5687124469213));
#297252=CARTESIAN_POINT('Ctrl Pts',(-3.10606665601012,6.33124999998515,
-9.5594902125713));
#297253=CARTESIAN_POINT('Ctrl Pts',(-6.21213331202023,6.48124999998455,
-8.55026797822134));
#297254=CARTESIAN_POINT('Ctrl Pts',(-8.13178807675721,6.63124999998395,
-5.90808986649102));
#297255=CARTESIAN_POINT('Ctrl Pts',(-10.0514428414942,6.78124999998335,
-3.2659117547607));
#297256=CARTESIAN_POINT('Ctrl Pts',(-10.0514428414942,6.93124999998275,
2.46189346052968E-15));
#297257=CARTESIAN_POINT('Ctrl Pts',(-10.0514428414942,7.08124999998215,
3.26591175476071));
#297258=CARTESIAN_POINT('Ctrl Pts',(-8.13178807675721,7.23124999998155,
5.90808986649102));
#297259=CARTESIAN_POINT('Ctrl Pts',(-6.21213331202023,7.38124999998095,
8.55026797822134));
#297260=CARTESIAN_POINT('Ctrl Pts',(-3.10606665601012,7.53124999998035,
9.5594902125713));
#297261=CARTESIAN_POINT('Ctrl Pts',(-1.49598380528385E-14,7.68124999997975,
10.5687124469213));
#297262=CARTESIAN_POINT('Ctrl Pts',(3.10606665601009,7.83124999997915,9.5594902125713));
#297263=CARTESIAN_POINT('Ctrl Pts',(6.2121333120202,7.98124999997856,8.55026797822134));
#297264=CARTESIAN_POINT('Ctrl Pts',(8.13178807675717,8.13124999997796,5.90808986649102));
#297265=CARTESIAN_POINT('Ctrl Pts',(10.0514428414942,8.28124999997736,3.2659117547607));
#297266=CARTESIAN_POINT('Ctrl Pts',(10.0514428414941,8.43124999997676,-1.23094673026484E-15));
#297267=CARTESIAN_POINT('Ctrl Pts',(10.0514428414941,8.58124999997616,-3.26591175476071));
#297268=CARTESIAN_POINT('Ctrl Pts',(8.13178807675717,8.73124999997556,-5.90808986649102));
#297269=CARTESIAN_POINT('Ctrl Pts',(6.2121333120202,8.88124999997496,-8.55026797822134));
#297270=CARTESIAN_POINT('Ctrl Pts',(3.10606665601009,9.03124999997436,-9.5594902125713));
#297271=CARTESIAN_POINT('Ctrl Pts',(-1.84122806625156E-14,9.18124999997375,
-10.5687124469213));
#297272=CARTESIAN_POINT('Ctrl Pts',(-3.10606665601013,9.33124999997315,
-9.5594902125713));
#297273=CARTESIAN_POINT('Ctrl Pts',(-6.21213331202023,9.48124999997255,
-8.55026797822134));
#297274=CARTESIAN_POINT('Ctrl Pts',(-8.13178807675721,9.63124999997195,
-5.90808986649102));
#297275=CARTESIAN_POINT('Ctrl Pts',(-10.0514428414942,9.78124999997135,
-3.2659117547607));
#297276=CARTESIAN_POINT('Ctrl Pts',(-10.0514428414942,9.93124999997075,
2.46189346052968E-15));
#297277=CARTESIAN_POINT('Ctrl Pts',(-10.0514428414942,10.0812499999701,
3.26591175476071));
#297278=CARTESIAN_POINT('Ctrl Pts',(-8.13178807675721,10.2312499999695,
5.90808986649102));
#297279=CARTESIAN_POINT('Ctrl Pts',(-6.21213331202023,10.3812499999689,
8.55026797822134));
#297280=CARTESIAN_POINT('Ctrl Pts',(-3.10606665601012,10.5312499999684,
9.5594902125713));
#297281=CARTESIAN_POINT('Ctrl Pts',(-1.66875473245003E-14,10.6812499999678,
10.5687124469213));
#297282=CARTESIAN_POINT('Ctrl Pts',(3.10606665601009,10.8312499999672,9.5594902125713));
#297283=CARTESIAN_POINT('Ctrl Pts',(6.2121333120202,10.9812499999666,8.55026797822134));
#297284=CARTESIAN_POINT('Ctrl Pts',(8.13178807675717,11.131249999966,5.90808986649102));
#297285=CARTESIAN_POINT('Ctrl Pts',(10.0514428414941,11.2812499999654,3.2659117547607));
#297286=CARTESIAN_POINT('Ctrl Pts',(10.0514428414941,11.4312499999648,-1.23094673026484E-15));
#297287=CARTESIAN_POINT('Ctrl Pts',(10.0514428414941,11.5812499999642,-3.26591175476071));
#297288=CARTESIAN_POINT('Ctrl Pts',(8.13178807675717,11.7312499999636,-5.90808986649102));
#297289=CARTESIAN_POINT('Ctrl Pts',(6.2121333120202,11.881249999963,-8.55026797822134));
#297290=CARTESIAN_POINT('Ctrl Pts',(3.10606665601009,12.0312499999624,-9.5594902125713));
#297291=CARTESIAN_POINT('Ctrl Pts',(-2.01399899341774E-14,12.1812499999618,
-10.5687124469213));
#297292=CARTESIAN_POINT('Ctrl Pts',(-3.10606665601013,12.3312499999612,
-9.5594902125713));
#297293=CARTESIAN_POINT('Ctrl Pts',(-6.21213331202024,12.4812499999605,
-8.55026797822134));
#297294=CARTESIAN_POINT('Ctrl Pts',(-8.13178807675721,12.6312499999599,
-5.90808986649102));
#297295=CARTESIAN_POINT('Ctrl Pts',(-10.0514428414942,12.7812499999593,
-3.2659117547607));
#297296=CARTESIAN_POINT('Ctrl Pts',(-10.0514428414942,12.9312499999587,
2.46189346052968E-15));
#297297=CARTESIAN_POINT('Ctrl Pts',(-10.0514428414942,13.0812499999581,
3.26591175476071));
#297298=CARTESIAN_POINT('Ctrl Pts',(-8.13178807675721,13.2312499999575,
5.90808986649102));
#297299=CARTESIAN_POINT('Ctrl Pts',(-6.21213331202023,13.3812499999569,
8.55026797822134));
#297300=CARTESIAN_POINT('Ctrl Pts',(-3.10606665601013,13.5312499999564,
9.5594902125713));
#297301=CARTESIAN_POINT('Ctrl Pts',(-1.84152565961621E-14,13.6812499999558,
10.5687124469213));
#297302=CARTESIAN_POINT('Ctrl Pts',(3.10606665601009,13.8312499999552,9.5594902125713));
#297303=CARTESIAN_POINT('Ctrl Pts',(6.2121333120202,13.9812499999546,8.55026797822134));
#297304=CARTESIAN_POINT('Ctrl Pts',(8.13178807675717,14.131249999954,5.90808986649102));
#297305=CARTESIAN_POINT('Ctrl Pts',(10.0514428414941,14.2812499999534,3.2659117547607));
#297306=CARTESIAN_POINT('Ctrl Pts',(10.0514428414941,14.4312499999528,-1.23094673026484E-15));
#297307=CARTESIAN_POINT('Ctrl Pts',(10.0514428414941,14.5812499999522,-3.26591175476071));
#297308=CARTESIAN_POINT('Ctrl Pts',(8.13178807675717,14.7312499999516,-5.90808986649102));
#297309=CARTESIAN_POINT('Ctrl Pts',(6.21213331202019,14.881249999951,-8.55026797822134));
#297310=CARTESIAN_POINT('Ctrl Pts',(3.10606665601009,15.0312499999504,-9.5594902125713));
#297311=CARTESIAN_POINT('Ctrl Pts',(-2.18676992058392E-14,15.1812499999498,
-10.5687124469213));
#297312=CARTESIAN_POINT('Ctrl Pts',(-3.10606665601013,15.3312499999492,
-9.5594902125713));
#297313=CARTESIAN_POINT('Ctrl Pts',(-6.21213331202024,15.4812499999485,
-8.55026797822134));
#297314=CARTESIAN_POINT('Ctrl Pts',(-8.13178807675721,15.6312499999479,
-5.90808986649102));
#297315=CARTESIAN_POINT('Ctrl Pts',(-10.0514428414942,15.7812499999473,
-3.2659117547607));
#297316=CARTESIAN_POINT('Ctrl Pts',(-10.0514428414942,15.9312499999467,
2.46189346052968E-15));
#297317=CARTESIAN_POINT('Ctrl Pts',(-10.0514428414942,16.0812499999461,
3.26591175476071));
#297318=CARTESIAN_POINT('Ctrl Pts',(-8.13178807675721,16.2312499999455,
5.90808986649102));
#297319=CARTESIAN_POINT('Ctrl Pts',(-6.21213331202024,16.3812499999449,
8.55026797822134));
#297320=CARTESIAN_POINT('Ctrl Pts',(-3.10606665601013,16.5312499999444,
9.5594902125713));
#297321=CARTESIAN_POINT('Ctrl Pts',(-2.0142965867824E-14,16.6812499999438,
10.5687124469213));
#297322=CARTESIAN_POINT('Ctrl Pts',(3.10606665601009,16.8312499999432,9.5594902125713));
#297323=CARTESIAN_POINT('Ctrl Pts',(6.21213331202019,16.9812499999426,8.55026797822134));
#297324=CARTESIAN_POINT('Ctrl Pts',(8.13178807675717,17.131249999942,5.90808986649102));
#297325=CARTESIAN_POINT('Ctrl Pts',(10.0514428414941,17.2812499999414,3.2659117547607));
#297326=CARTESIAN_POINT('Ctrl Pts',(10.0514428414941,17.4312499999408,-1.23094673026484E-15));
#297327=CARTESIAN_POINT('Ctrl Pts',(10.0514428414941,17.5812499999402,-3.26591175476071));
#297328=CARTESIAN_POINT('Ctrl Pts',(8.13178807675717,17.7312499999396,-5.90808986649102));
#297329=CARTESIAN_POINT('Ctrl Pts',(6.21213331202019,17.881249999939,-8.55026797822134));
#297330=CARTESIAN_POINT('Ctrl Pts',(3.10606665601008,18.0312499999384,-9.5594902125713));
#297331=CARTESIAN_POINT('Ctrl Pts',(-2.35954084775011E-14,18.1812499999378,
-10.5687124469213));
#297332=CARTESIAN_POINT('Ctrl Pts',(-3.10606665601013,18.3312499999371,
-9.5594902125713));
#297333=CARTESIAN_POINT('Ctrl Pts',(-6.21213331202024,18.4812499999365,
-8.55026797822134));
#297334=CARTESIAN_POINT('Ctrl Pts',(-8.13178807675721,18.6312499999359,
-5.90808986649102));
#297335=CARTESIAN_POINT('Ctrl Pts',(-10.0514428414942,18.7812499999353,
-3.2659117547607));
#297336=CARTESIAN_POINT('Ctrl Pts',(-10.0514428414942,18.9312499999347,
2.46189346052968E-15));
#297337=CARTESIAN_POINT('Ctrl Pts',(-10.0514428414942,19.0812499999341,
3.26591175476071));
#297338=CARTESIAN_POINT('Ctrl Pts',(-8.13178807675721,19.2312499999335,
5.90808986649102));
#297339=CARTESIAN_POINT('Ctrl Pts',(-6.21213331202024,19.381249999933,8.55026797822134));
#297340=CARTESIAN_POINT('Ctrl Pts',(-3.10606665601013,19.5312499999323,
9.5594902125713));
#297341=CARTESIAN_POINT('Ctrl Pts',(-2.18706751394858E-14,19.6812499999318,
10.5687124469213));
#297342=CARTESIAN_POINT('Ctrl Pts',(3.10606665601009,19.8312499999312,9.5594902125713));
#297343=CARTESIAN_POINT('Ctrl Pts',(6.21213331202019,19.9812499999306,8.55026797822134));
#297344=CARTESIAN_POINT('Ctrl Pts',(8.13178807675717,20.13124999993,5.90808986649102));
#297345=CARTESIAN_POINT('Ctrl Pts',(10.0514428414941,20.2812499999294,3.2659117547607));
#297346=CARTESIAN_POINT('Ctrl Pts',(10.0514428414941,20.4312499999288,-1.23094673026484E-15));
#297347=CARTESIAN_POINT('Ctrl Pts',(10.0514428414941,20.5812499999282,-3.26591175476071));
#297348=CARTESIAN_POINT('Ctrl Pts',(8.13178807675716,20.7312499999276,-5.90808986649102));
#297349=CARTESIAN_POINT('Ctrl Pts',(6.21213331202019,20.881249999927,-8.55026797822134));
#297350=CARTESIAN_POINT('Ctrl Pts',(3.10606665601008,21.0312499999264,-9.5594902125713));
#297351=CARTESIAN_POINT('Ctrl Pts',(-2.53231177491629E-14,21.1812499999258,
-10.5687124469213));
#297352=CARTESIAN_POINT('Ctrl Pts',(-3.10606665601013,21.3312499999251,
-9.5594902125713));
#297353=CARTESIAN_POINT('Ctrl Pts',(-6.21213331202024,21.4812499999245,
-8.55026797822134));
#297354=CARTESIAN_POINT('Ctrl Pts',(-8.13178807675722,21.6312499999239,
-5.90808986649102));
#297355=CARTESIAN_POINT('Ctrl Pts',(-10.0514428414942,21.7812499999233,
-3.2659117547607));
#297356=CARTESIAN_POINT('Ctrl Pts',(-10.0514428414942,21.9312499999227,
2.46189346052968E-15));
#297357=CARTESIAN_POINT('Ctrl Pts',(-10.0514428414942,22.0812499999221,
3.26591175476071));
#297358=CARTESIAN_POINT('Ctrl Pts',(-8.13178807675722,22.2312499999215,
5.90808986649102));
#297359=CARTESIAN_POINT('Ctrl Pts',(-6.21213331202024,22.3812499999209,
8.55026797822134));
#297360=CARTESIAN_POINT('Ctrl Pts',(-3.10606665601013,22.5312499999204,
9.5594902125713));
#297361=CARTESIAN_POINT('Ctrl Pts',(-2.35983844111477E-14,22.6812499999198,
10.5687124469213));
#297362=CARTESIAN_POINT('Ctrl Pts',(3.10606665601008,22.8312499999192,9.5594902125713));
#297363=CARTESIAN_POINT('Ctrl Pts',(6.21213331202019,22.9812499999186,8.55026797822134));
#297364=CARTESIAN_POINT('Ctrl Pts',(8.13178807675716,23.131249999918,5.90808986649102));
#297365=CARTESIAN_POINT('Ctrl Pts',(10.0514428414941,23.2812499999174,3.2659117547607));
#297366=CARTESIAN_POINT('Ctrl Pts',(10.0514428414941,23.4312499999168,-1.23094673026484E-15));
#297367=CARTESIAN_POINT('Ctrl Pts',(10.0514428414941,23.5812499999162,-3.26591175476071));
#297368=CARTESIAN_POINT('Ctrl Pts',(8.13178807675716,23.7312499999156,-5.90808986649102));
#297369=CARTESIAN_POINT('Ctrl Pts',(6.21213331202019,23.881249999915,-8.55026797822134));
#297370=CARTESIAN_POINT('Ctrl Pts',(3.10606665601008,24.0312499999144,-9.5594902125713));
#297371=CARTESIAN_POINT('Ctrl Pts',(-2.70508270208248E-14,24.1812499999138,
-10.5687124469213));
#297372=CARTESIAN_POINT('Ctrl Pts',(-3.10606665601014,24.3312499999131,
-9.5594902125713));
#297373=CARTESIAN_POINT('Ctrl Pts',(-6.21213331202024,24.4812499999125,
-8.55026797822134));
#297374=CARTESIAN_POINT('Ctrl Pts',(-8.13178807675722,24.6312499999119,
-5.90808986649102));
#297375=CARTESIAN_POINT('Ctrl Pts',(-10.0514428414942,24.7812499999113,
-3.2659117547607));
#297376=CARTESIAN_POINT('Ctrl Pts',(-10.0514428414942,24.9312499999107,
2.46189346052968E-15));
#297377=CARTESIAN_POINT('Ctrl Pts',(-10.0514428414942,25.0812499999101,
3.26591175476071));
#297378=CARTESIAN_POINT('Ctrl Pts',(-8.13178807675722,25.2312499999095,
5.90808986649102));
#297379=CARTESIAN_POINT('Ctrl Pts',(-6.21213331202024,25.381249999909,8.55026797822134));
#297380=CARTESIAN_POINT('Ctrl Pts',(-3.10606665601013,25.5312499999084,
9.5594902125713));
#297381=CARTESIAN_POINT('Ctrl Pts',(-2.53260936828095E-14,25.6812499999078,
10.5687124469213));
#297382=CARTESIAN_POINT('Ctrl Pts',(3.10606665601008,25.8312499999072,9.5594902125713));
#297383=CARTESIAN_POINT('Ctrl Pts',(6.21213331202019,25.9812499999066,8.55026797822134));
#297384=CARTESIAN_POINT('Ctrl Pts',(8.13178807675716,26.131249999906,5.90808986649102));
#297385=CARTESIAN_POINT('Ctrl Pts',(10.0514428414941,26.2812499999054,3.2659117547607));
#297386=CARTESIAN_POINT('Ctrl Pts',(10.0514428414941,26.4312499999048,-1.23094673026484E-15));
#297387=CARTESIAN_POINT('Ctrl Pts',(10.0514428414941,26.5812499999042,-3.26591175476071));
#297388=CARTESIAN_POINT('Ctrl Pts',(8.13178807675716,26.7312499999036,-5.90808986649102));
#297389=CARTESIAN_POINT('Ctrl Pts',(6.21213331202019,26.881249999903,-8.55026797822134));
#297390=CARTESIAN_POINT('Ctrl Pts',(3.10606665601008,27.0312499999024,-9.5594902125713));
#297391=CARTESIAN_POINT('Ctrl Pts',(-2.87785362924866E-14,27.1812499999018,
-10.5687124469213));
#297392=CARTESIAN_POINT('Ctrl Pts',(-3.10606665601014,27.3312499999011,
-9.5594902125713));
#297393=CARTESIAN_POINT('Ctrl Pts',(-6.21213331202024,27.4812499999005,
-8.55026797822134));
#297394=CARTESIAN_POINT('Ctrl Pts',(-8.13178807675722,27.6312499998999,
-5.90808986649102));
#297395=CARTESIAN_POINT('Ctrl Pts',(-10.0514428414942,27.7812499998993,
-3.2659117547607));
#297396=CARTESIAN_POINT('Ctrl Pts',(-10.0514428414942,27.9312499998987,
2.46189346052968E-15));
#297397=CARTESIAN_POINT('Ctrl Pts',(-10.0514428414942,28.0812499998981,
3.26591175476071));
#297398=CARTESIAN_POINT('Ctrl Pts',(-8.13178807675722,28.2312499998975,
5.90808986649102));
#297399=CARTESIAN_POINT('Ctrl Pts',(-6.21213331202024,28.3812499998969,
8.55026797822134));
#297400=CARTESIAN_POINT('Ctrl Pts',(-3.10606665601014,28.5312499998964,
9.5594902125713));
#297401=CARTESIAN_POINT('Ctrl Pts',(-2.70538029544713E-14,28.6812499998958,
10.5687124469213));
#297402=CARTESIAN_POINT('Ctrl Pts',(3.10606665601008,28.8312499998952,9.5594902125713));
#297403=CARTESIAN_POINT('Ctrl Pts',(6.21213331202019,28.9812499998946,8.55026797822134));
#297404=CARTESIAN_POINT('Ctrl Pts',(8.13178807675716,29.131249999894,5.90808986649102));
#297405=CARTESIAN_POINT('Ctrl Pts',(10.0514428414941,29.2812499998934,3.2659117547607));
#297406=CARTESIAN_POINT('Ctrl Pts',(10.0514428414941,29.4312499998928,-1.23094673026484E-15));
#297407=CARTESIAN_POINT('Ctrl Pts',(10.0514428414941,29.5812499998922,-3.26591175476071));
#297408=CARTESIAN_POINT('Ctrl Pts',(8.13178807675716,29.7312499998916,-5.90808986649102));
#297409=CARTESIAN_POINT('Ctrl Pts',(6.21213331202019,29.881249999891,-8.55026797822134));
#297410=CARTESIAN_POINT('Ctrl Pts',(3.10606665601008,30.0312499998904,-9.5594902125713));
#297411=CARTESIAN_POINT('Ctrl Pts',(-3.05062455641484E-14,30.1812499998898,
-10.5687124469213));
#297412=CARTESIAN_POINT('Ctrl Pts',(-3.10606665601014,30.3312499998892,
-9.5594902125713));
#297413=CARTESIAN_POINT('Ctrl Pts',(-6.21213331202025,30.4812499998885,
-8.55026797822134));
#297414=CARTESIAN_POINT('Ctrl Pts',(-8.13178807675722,30.6312499998879,
-5.90808986649102));
#297415=CARTESIAN_POINT('Ctrl Pts',(-10.0514428414942,30.7812499998873,
-3.2659117547607));
#297416=CARTESIAN_POINT('Ctrl Pts',(-10.0514428414942,30.9312499998867,
2.46189346052968E-15));
#297417=CARTESIAN_POINT('Ctrl Pts',(-10.0514428414942,31.0812499998861,
3.26591175476071));
#297418=CARTESIAN_POINT('Ctrl Pts',(-8.13178807675722,31.2312499998855,
5.90808986649102));
#297419=CARTESIAN_POINT('Ctrl Pts',(-6.21213331202024,31.381249999885,8.55026797822134));
#297420=CARTESIAN_POINT('Ctrl Pts',(-3.10606665601014,31.5312499998843,
9.5594902125713));
#297421=CARTESIAN_POINT('Ctrl Pts',(-2.87815122261332E-14,31.6812499998838,
10.5687124469213));
#297422=CARTESIAN_POINT('Ctrl Pts',(3.10606665601008,31.8312499998832,9.5594902125713));
#297423=CARTESIAN_POINT('Ctrl Pts',(6.21213331202019,31.9812499998826,8.55026797822134));
#297424=CARTESIAN_POINT('Ctrl Pts',(8.13178807675716,32.131249999882,5.90808986649102));
#297425=CARTESIAN_POINT('Ctrl Pts',(10.0514428414941,32.2812499998814,3.2659117547607));
#297426=CARTESIAN_POINT('Ctrl Pts',(10.0514428414941,32.4312499998808,-1.23094673026484E-15));
#297427=CARTESIAN_POINT('Ctrl Pts',(10.0514428414941,32.5812499998802,-3.26591175476071));
#297428=CARTESIAN_POINT('Ctrl Pts',(8.13178807675716,32.7312499998796,-5.90808986649102));
#297429=CARTESIAN_POINT('Ctrl Pts',(6.21213331202019,32.8812499998789,-8.55026797822134));
#297430=CARTESIAN_POINT('Ctrl Pts',(3.10606665601008,33.0312499998784,-9.5594902125713));
#297431=CARTESIAN_POINT('Ctrl Pts',(-3.22339548358103E-14,33.1812499998777,
-10.5687124469213));
#297432=CARTESIAN_POINT('Ctrl Pts',(-3.10606665601014,33.3312499998772,
-9.5594902125713));
#297433=CARTESIAN_POINT('Ctrl Pts',(-6.21213331202025,33.4812499998766,
-8.55026797822134));
#297434=CARTESIAN_POINT('Ctrl Pts',(-8.13178807675722,33.6312499998759,
-5.90808986649102));
#297435=CARTESIAN_POINT('Ctrl Pts',(-10.0514428414942,33.7812499998753,
-3.2659117547607));
#297436=CARTESIAN_POINT('Ctrl Pts',(-10.0514428414942,33.9312499998747,
2.46189346052968E-15));
#297437=CARTESIAN_POINT('Ctrl Pts',(-10.0514428414942,34.0812499998741,
3.26591175476071));
#297438=CARTESIAN_POINT('Ctrl Pts',(-8.13178807675722,34.2312499998735,
5.90808986649102));
#297439=CARTESIAN_POINT('Ctrl Pts',(-6.21213331202024,34.3812499998729,
8.55026797822134));
#297440=CARTESIAN_POINT('Ctrl Pts',(-3.10606665601014,34.5312499998724,
9.5594902125713));
#297441=CARTESIAN_POINT('Ctrl Pts',(-3.0509221497795E-14,34.6812499998718,
10.5687124469213));
#297442=CARTESIAN_POINT('Ctrl Pts',(3.10606665601008,34.8312499998712,9.5594902125713));
#297443=CARTESIAN_POINT('Ctrl Pts',(6.21213331202019,34.9812499998706,8.55026797822134));
#297444=CARTESIAN_POINT('Ctrl Pts',(8.13178807675716,35.13124999987,5.90808986649102));
#297445=CARTESIAN_POINT('Ctrl Pts',(10.0514428414941,35.2812499998694,3.2659117547607));
#297446=CARTESIAN_POINT('Ctrl Pts',(10.0514428414941,35.4312499998688,-1.23094673026484E-15));
#297447=CARTESIAN_POINT('Ctrl Pts',(10.0514428414941,35.5812499998682,-3.26591175476071));
#297448=CARTESIAN_POINT('Ctrl Pts',(8.13178807675716,35.7312499998676,-5.90808986649102));
#297449=CARTESIAN_POINT('Ctrl Pts',(6.21213331202018,35.881249999867,-8.55026797822134));
#297450=CARTESIAN_POINT('Ctrl Pts',(3.10606665601007,36.0312499998664,-9.5594902125713));
#297451=CARTESIAN_POINT('Ctrl Pts',(-3.39616641074721E-14,36.1812499998658,
-10.5687124469213));
#297452=CARTESIAN_POINT('Ctrl Pts',(-3.10606665601014,36.3312499998652,
-9.5594902125713));
#297453=CARTESIAN_POINT('Ctrl Pts',(-6.21213331202025,36.4812499998646,
-8.55026797822134));
#297454=CARTESIAN_POINT('Ctrl Pts',(-8.13178807675722,36.6312499998639,
-5.90808986649102));
#297455=CARTESIAN_POINT('Ctrl Pts',(-10.0514428414942,36.7812499998634,
-3.2659117547607));
#297456=CARTESIAN_POINT('Ctrl Pts',(-10.0514428414942,36.9312499998627,
2.46189346052968E-15));
#297457=CARTESIAN_POINT('Ctrl Pts',(-10.0514428414942,37.0812499998621,
3.26591175476071));
#297458=CARTESIAN_POINT('Ctrl Pts',(-8.13178807675722,37.2312499998615,
5.90808986649102));
#297459=CARTESIAN_POINT('Ctrl Pts',(-6.21213331202025,37.3812499998609,
8.55026797822134));
#297460=CARTESIAN_POINT('Ctrl Pts',(-3.10606665601014,37.5312499998603,
9.5594902125713));
#297461=CARTESIAN_POINT('Ctrl Pts',(-3.22369307694568E-14,37.6812499998598,
10.5687124469213));
#297462=CARTESIAN_POINT('Ctrl Pts',(3.10606665601008,37.8312499998592,9.5594902125713));
#297463=CARTESIAN_POINT('Ctrl Pts',(6.21213331202018,37.9812499998586,8.55026797822134));
#297464=CARTESIAN_POINT('Ctrl Pts',(8.13178807675716,38.131249999858,5.90808986649102));
#297465=CARTESIAN_POINT('Ctrl Pts',(10.0514428414941,38.2812499998574,3.2659117547607));
#297466=CARTESIAN_POINT('Ctrl Pts',(10.0514428414941,38.4312499998568,-1.23094673026484E-15));
#297467=CARTESIAN_POINT('Ctrl Pts',(10.0514428414941,38.5812499998562,-3.26591175476071));
#297468=CARTESIAN_POINT('Ctrl Pts',(8.13178807675715,38.7312499998556,-5.90808986649102));
#297469=CARTESIAN_POINT('Ctrl Pts',(6.21213331202018,38.881249999855,-8.55026797822134));
#297470=CARTESIAN_POINT('Ctrl Pts',(3.10606665601007,39.0312499998544,-9.5594902125713));
#297471=CARTESIAN_POINT('Ctrl Pts',(-3.5689373379134E-14,39.1812499998538,
-10.5687124469213));
#297472=CARTESIAN_POINT('Ctrl Pts',(-3.10606665601014,39.3312499998532,
-9.5594902125713));
#297473=CARTESIAN_POINT('Ctrl Pts',(-6.21213331202025,39.4812499998525,
-8.55026797822134));
#297474=CARTESIAN_POINT('Ctrl Pts',(-8.13178807675723,39.6312499998519,
-5.90808986649102));
#297475=CARTESIAN_POINT('Ctrl Pts',(-10.0514428414942,39.7812499998513,
-3.2659117547607));
#297476=CARTESIAN_POINT('Ctrl Pts',(-10.0514428414942,39.9312499998507,
2.46189346052968E-15));
#297477=CARTESIAN_POINT('Ctrl Pts',(-10.0514428414942,40.0812499998502,
3.26591175476071));
#297478=CARTESIAN_POINT('Ctrl Pts',(-8.13178807675723,40.2312499998495,
5.90808986649102));
#297479=CARTESIAN_POINT('Ctrl Pts',(-6.21213331202025,40.3812499998489,
8.55026797822134));
#297480=CARTESIAN_POINT('Ctrl Pts',(-3.10606665601014,40.5312499998483,
9.5594902125713));
#297481=CARTESIAN_POINT('Ctrl Pts',(-3.39646400411187E-14,40.6812499998478,
10.5687124469213));
#297482=CARTESIAN_POINT('Ctrl Pts',(3.10606665601007,40.8312499998472,9.5594902125713));
#297483=CARTESIAN_POINT('Ctrl Pts',(6.21213331202018,40.9812499998466,8.55026797822134));
#297484=CARTESIAN_POINT('Ctrl Pts',(8.13178807675715,41.131249999846,5.90808986649102));
#297485=CARTESIAN_POINT('Ctrl Pts',(10.0514428414941,41.2812499998454,3.2659117547607));
#297486=CARTESIAN_POINT('Ctrl Pts',(10.0514428414941,41.4312499998448,-1.23094673026484E-15));
#297487=CARTESIAN_POINT('Ctrl Pts',(10.0514428414941,41.5812499998442,-3.26591175476071));
#297488=CARTESIAN_POINT('Ctrl Pts',(8.13178807675715,41.7312499998436,-5.90808986649102));
#297489=CARTESIAN_POINT('Ctrl Pts',(6.21213331202018,41.881249999843,-8.55026797822134));
#297490=CARTESIAN_POINT('Ctrl Pts',(3.10606665601007,42.0312499998423,-9.5594902125713));
#297491=CARTESIAN_POINT('Ctrl Pts',(-3.74170826507958E-14,42.1812499998418,
-10.5687124469213));
#297492=CARTESIAN_POINT('Ctrl Pts',(-3.10606665601015,42.3312499998411,
-9.5594902125713));
#297493=CARTESIAN_POINT('Ctrl Pts',(-6.21213331202025,42.4812499998406,
-8.55026797822134));
#297494=CARTESIAN_POINT('Ctrl Pts',(-8.13178807675723,42.6312499998399,
-5.90808986649102));
#297495=CARTESIAN_POINT('Ctrl Pts',(-10.0514428414942,42.7812499998393,
-3.2659117547607));
#297496=CARTESIAN_POINT('Ctrl Pts',(-10.0514428414942,42.9312499998387,
2.46189346052968E-15));
#297497=CARTESIAN_POINT('Ctrl Pts',(-10.0514428414942,43.0812499998381,
3.26591175476071));
#297498=CARTESIAN_POINT('Ctrl Pts',(-8.13178807675723,43.2312499998375,
5.90808986649102));
#297499=CARTESIAN_POINT('Ctrl Pts',(-6.21213331202025,43.3812499998369,
8.55026797822134));
#297500=CARTESIAN_POINT('Ctrl Pts',(-3.10606665601014,43.5312499998363,
9.5594902125713));
#297501=CARTESIAN_POINT('Ctrl Pts',(-3.56923493127805E-14,43.6812499998357,
10.5687124469213));
#297502=CARTESIAN_POINT('Ctrl Pts',(3.10606665601007,43.8312499998352,9.5594902125713));
#297503=CARTESIAN_POINT('Ctrl Pts',(6.21213331202018,43.9812499998345,8.55026797822134));
#297504=CARTESIAN_POINT('Ctrl Pts',(8.13178807675715,44.131249999834,5.90808986649102));
#297505=CARTESIAN_POINT('Ctrl Pts',(10.0514428414941,44.2812499998334,3.2659117547607));
#297506=CARTESIAN_POINT('Ctrl Pts',(10.0514428414941,44.4312499998328,-1.23094673026484E-15));
#297507=CARTESIAN_POINT('Ctrl Pts',(10.0514428414941,44.5812499998322,-3.26591175476071));
#297508=CARTESIAN_POINT('Ctrl Pts',(8.13178807675715,44.7312499998316,-5.90808986649102));
#297509=CARTESIAN_POINT('Ctrl Pts',(6.21213331202018,44.881249999831,-8.55026797822134));
#297510=CARTESIAN_POINT('Ctrl Pts',(3.10606665601007,45.0312499998304,-9.5594902125713));
#297511=CARTESIAN_POINT('Ctrl Pts',(-3.91447919224576E-14,45.1812499998297,
-10.5687124469213));
#297512=CARTESIAN_POINT('Ctrl Pts',(-3.10606665601015,45.3312499998292,
-9.5594902125713));
#297513=CARTESIAN_POINT('Ctrl Pts',(-6.21213331202026,45.4812499998285,
-8.55026797822134));
#297514=CARTESIAN_POINT('Ctrl Pts',(-8.13178807675723,45.6312499998279,
-5.90808986649102));
#297515=CARTESIAN_POINT('Ctrl Pts',(-10.0514428414942,45.7812499998273,
-3.2659117547607));
#297516=CARTESIAN_POINT('Ctrl Pts',(-10.0514428414942,45.9312499998267,
2.46189346052968E-15));
#297517=CARTESIAN_POINT('Ctrl Pts',(-10.0514428414942,46.0812499998261,
3.26591175476071));
#297518=CARTESIAN_POINT('Ctrl Pts',(-8.13178807675723,46.2312499998255,
5.90808986649102));
#297519=CARTESIAN_POINT('Ctrl Pts',(-6.21213331202025,46.3812499998249,
8.55026797822134));
#297520=CARTESIAN_POINT('Ctrl Pts',(-3.10606665601015,46.5312499998244,
9.5594902125713));
#297521=CARTESIAN_POINT('Ctrl Pts',(-3.74200585844424E-14,46.6812499998238,
10.5687124469213));
#297522=CARTESIAN_POINT('Ctrl Pts',(3.10606665601007,46.8312499998232,9.5594902125713));
#297523=CARTESIAN_POINT('Ctrl Pts',(6.21213331202018,46.9812499998226,8.55026797822134));
#297524=CARTESIAN_POINT('Ctrl Pts',(8.13178807675715,47.131249999822,5.90808986649102));
#297525=CARTESIAN_POINT('Ctrl Pts',(10.0514428414941,47.2812499998214,3.2659117547607));
#297526=CARTESIAN_POINT('Ctrl Pts',(10.0514428414941,47.4312499998208,-1.23094673026484E-15));
#297527=CARTESIAN_POINT('Ctrl Pts',(10.0514428414941,47.5812499998202,-3.26591175476071));
#297528=CARTESIAN_POINT('Ctrl Pts',(8.13178807675715,47.7312499998196,-5.90808986649102));
#297529=CARTESIAN_POINT('Ctrl Pts',(6.21213331202017,47.881249999819,-8.55026797822134));
#297530=CARTESIAN_POINT('Ctrl Pts',(3.10606665601007,48.0312499998184,-9.5594902125713));
#297531=CARTESIAN_POINT('Ctrl Pts',(-4.08725011941195E-14,48.1812499998178,
-10.5687124469213));
#297532=CARTESIAN_POINT('Ctrl Pts',(-3.10606665601015,48.3312499998172,
-9.5594902125713));
#297533=CARTESIAN_POINT('Ctrl Pts',(-6.21213331202026,48.4812499998166,
-8.55026797822134));
#297534=CARTESIAN_POINT('Ctrl Pts',(-8.13178807675723,48.6312499998159,
-5.90808986649102));
#297535=CARTESIAN_POINT('Ctrl Pts',(-10.0514428414942,48.7812499998153,
-3.2659117547607));
#297536=CARTESIAN_POINT('Ctrl Pts',(-10.0514428414942,48.9312499998147,
2.46189346052968E-15));
#297537=CARTESIAN_POINT('Ctrl Pts',(-10.0514428414942,49.0812499998141,
3.26591175476071));
#297538=CARTESIAN_POINT('Ctrl Pts',(-8.13178807675723,49.2312499998135,
5.90808986649102));
#297539=CARTESIAN_POINT('Ctrl Pts',(-6.21213331202026,49.3812499998129,
8.55026797822134));
#297540=CARTESIAN_POINT('Ctrl Pts',(-3.10606665601015,49.5312499998124,
9.5594902125713));
#297541=CARTESIAN_POINT('Ctrl Pts',(-3.91477678561042E-14,49.6812499998117,
10.5687124469213));
#297542=CARTESIAN_POINT('Ctrl Pts',(3.10606665601007,49.8312499998111,9.5594902125713));
#297543=CARTESIAN_POINT('Ctrl Pts',(6.21213331202017,49.9812499998106,8.55026797822134));
#297544=CARTESIAN_POINT('Ctrl Pts',(8.13178807675715,50.13124999981,5.90808986649102));
#297545=CARTESIAN_POINT('Ctrl Pts',(10.0514428414941,50.2812499998094,3.2659117547607));
#297546=CARTESIAN_POINT('Ctrl Pts',(10.0514428414941,50.4312499998088,-1.23094673026484E-15));
#297547=CARTESIAN_POINT('Ctrl Pts',(10.0514428414941,50.5812499998082,-3.26591175476071));
#297548=CARTESIAN_POINT('Ctrl Pts',(8.13178807675715,50.7312499998076,-5.90808986649102));
#297549=CARTESIAN_POINT('Ctrl Pts',(6.21213331202017,50.881249999807,-8.55026797822134));
#297550=CARTESIAN_POINT('Ctrl Pts',(3.10606665601007,51.0312499998064,-9.5594902125713));
#297551=CARTESIAN_POINT('Ctrl Pts',(-4.26002104657813E-14,51.1812499998058,
-10.5687124469213));
#297552=CARTESIAN_POINT('Ctrl Pts',(-3.10606665601015,51.3312499998052,
-9.5594902125713));
#297553=CARTESIAN_POINT('Ctrl Pts',(-6.21213331202026,51.4812499998045,
-8.55026797822134));
#297554=CARTESIAN_POINT('Ctrl Pts',(-8.13178807675723,51.631249999804,-5.90808986649102));
#297555=CARTESIAN_POINT('Ctrl Pts',(-10.0514428414942,51.7812499998034,
-3.2659117547607));
#297556=CARTESIAN_POINT('Ctrl Pts',(-10.0514428414942,51.9312499998027,
2.46189346052968E-15));
#297557=CARTESIAN_POINT('Ctrl Pts',(-10.0514428414942,52.0812499998021,
3.26591175476071));
#297558=CARTESIAN_POINT('Ctrl Pts',(-8.13178807675723,52.2312499998015,
5.90808986649102));
#297559=CARTESIAN_POINT('Ctrl Pts',(-6.21213331202026,52.3812499998009,
8.55026797822134));
#297560=CARTESIAN_POINT('Ctrl Pts',(-3.10606665601015,52.5312499998004,
9.5594902125713));
#297561=CARTESIAN_POINT('Ctrl Pts',(-4.08754771277661E-14,52.6812499997998,
10.5687124469213));
#297562=CARTESIAN_POINT('Ctrl Pts',(3.10606665601007,52.8312499997991,9.5594902125713));
#297563=CARTESIAN_POINT('Ctrl Pts',(6.21213331202017,52.9812499997986,8.55026797822134));
#297564=CARTESIAN_POINT('Ctrl Pts',(8.13178807675715,53.131249999798,5.90808986649102));
#297565=CARTESIAN_POINT('Ctrl Pts',(10.0514428414941,53.2812499997974,3.2659117547607));
#297566=CARTESIAN_POINT('Ctrl Pts',(10.0514428414941,53.4312499997968,-1.23094673026484E-15));
#297567=CARTESIAN_POINT('Ctrl Pts',(10.0514428414941,53.5812499997962,-3.26591175476071));
#297568=CARTESIAN_POINT('Ctrl Pts',(8.13178807675714,53.7312499997956,-5.90808986649102));
#297569=CARTESIAN_POINT('Ctrl Pts',(6.21213331202017,53.881249999795,-8.55026797822134));
#297570=CARTESIAN_POINT('Ctrl Pts',(3.10606665601006,54.0312499997944,-9.5594902125713));
#297571=CARTESIAN_POINT('Ctrl Pts',(-4.43279197374432E-14,54.1812499997938,
-10.5687124469213));
#297572=CARTESIAN_POINT('Ctrl Pts',(-3.10606665601015,54.3312499997932,
-9.5594902125713));
#297573=CARTESIAN_POINT('Ctrl Pts',(-6.21213331202026,54.4812499997926,
-8.55026797822134));
#297574=CARTESIAN_POINT('Ctrl Pts',(-8.13178807675724,54.6312499997919,
-5.90808986649102));
#297575=CARTESIAN_POINT('Ctrl Pts',(-10.0514428414942,54.7812499997914,
-3.2659117547607));
#297576=CARTESIAN_POINT('Ctrl Pts',(-10.0514428414942,54.9312499997907,
2.46189346052968E-15));
#297577=CARTESIAN_POINT('Ctrl Pts',(-10.0514428414942,55.0812499997901,
3.26591175476071));
#297578=CARTESIAN_POINT('Ctrl Pts',(-8.13178807675724,55.2312499997895,
5.90808986649102));
#297579=CARTESIAN_POINT('Ctrl Pts',(-6.21213331202026,55.3812499997889,
8.55026797822134));
#297580=CARTESIAN_POINT('Ctrl Pts',(-3.10606665601015,55.5312499997884,
9.5594902125713));
#297581=CARTESIAN_POINT('Ctrl Pts',(-4.26031863994279E-14,55.6812499997877,
10.5687124469213));
#297582=CARTESIAN_POINT('Ctrl Pts',(3.10606665601006,55.8312499997871,9.5594902125713));
#297583=CARTESIAN_POINT('Ctrl Pts',(6.21213331202017,55.9812499997865,8.55026797822134));
#297584=CARTESIAN_POINT('Ctrl Pts',(8.13178807675714,56.131249999786,5.90808986649102));
#297585=CARTESIAN_POINT('Ctrl Pts',(10.0514428414941,56.2812499997854,3.2659117547607));
#297586=CARTESIAN_POINT('Ctrl Pts',(10.0514428414941,56.4312499997848,-1.23094673026484E-15));
#297587=CARTESIAN_POINT('Ctrl Pts',(10.0514428414941,56.5812499997842,-3.26591175476071));
#297588=CARTESIAN_POINT('Ctrl Pts',(8.13178807675714,56.7312499997836,-5.90808986649102));
#297589=CARTESIAN_POINT('Ctrl Pts',(6.21213331202017,56.881249999783,-8.55026797822134));
#297590=CARTESIAN_POINT('Ctrl Pts',(3.10606665601006,57.0312499997824,-9.5594902125713));
#297591=CARTESIAN_POINT('Ctrl Pts',(-4.6055629009105E-14,57.1812499997818,
-10.5687124469213));
#297592=CARTESIAN_POINT('Ctrl Pts',(-3.10606665601015,57.3312499997812,
-9.5594902125713));
#297593=CARTESIAN_POINT('Ctrl Pts',(-6.21213331202026,57.4812499997805,
-8.55026797822134));
#297594=CARTESIAN_POINT('Ctrl Pts',(-8.13178807675724,57.6312499997799,
-5.90808986649102));
#297595=CARTESIAN_POINT('Ctrl Pts',(-10.0514428414942,57.7812499997793,
-3.2659117547607));
#297596=CARTESIAN_POINT('Ctrl Pts',(-10.0514428414942,57.9312499997787,
2.46189346052968E-15));
#297597=CARTESIAN_POINT('Ctrl Pts',(-10.0514428414942,58.0812499997781,
3.26591175476071));
#297598=CARTESIAN_POINT('Ctrl Pts',(-8.13178807675724,58.2312499997775,
5.90808986649102));
#297599=CARTESIAN_POINT('Ctrl Pts',(-6.21213331202026,58.3812499997769,
8.55026797822134));
#297600=CARTESIAN_POINT('Ctrl Pts',(-3.10606665601015,58.5312499997763,
9.5594902125713));
#297601=CARTESIAN_POINT('Ctrl Pts',(-4.43308956710897E-14,58.6812499997758,
10.5687124469213));
#297602=CARTESIAN_POINT('Ctrl Pts',(3.10606665601006,58.8312499997751,9.5594902125713));
#297603=CARTESIAN_POINT('Ctrl Pts',(6.21213331202017,58.9812499997745,8.55026797822134));
#297604=CARTESIAN_POINT('Ctrl Pts',(8.13178807675714,59.131249999774,5.90808986649102));
#297605=CARTESIAN_POINT('Ctrl Pts',(10.0514428414941,59.2812499997734,3.2659117547607));
#297606=CARTESIAN_POINT('Ctrl Pts',(10.0514428414941,59.4312499997728,-1.23094673026484E-15));
#297607=CARTESIAN_POINT('Ctrl Pts',(10.0514428414941,59.5812499997722,-3.26591175476071));
#297608=CARTESIAN_POINT('Ctrl Pts',(8.13178807675714,59.7312499997716,-5.90808986649102));
#297609=CARTESIAN_POINT('Ctrl Pts',(6.21213331202017,59.881249999771,-8.55026797822134));
#297610=CARTESIAN_POINT('Ctrl Pts',(3.10606665601006,60.0312499997704,-9.5594902125713));
#297611=CARTESIAN_POINT('Ctrl Pts',(-4.77833382807668E-14,60.1812499997698,
-10.5687124469213));
#297612=CARTESIAN_POINT('Ctrl Pts',(-3.10606665601016,60.3312499997692,
-9.5594902125713));
#297613=CARTESIAN_POINT('Ctrl Pts',(-6.21213331202026,60.4812499997686,
-8.55026797822134));
#297614=CARTESIAN_POINT('Ctrl Pts',(-8.13178807675724,60.6312499997679,
-5.90808986649102));
#297615=CARTESIAN_POINT('Ctrl Pts',(-10.0514428414942,60.7812499997674,
-3.2659117547607));
#297616=CARTESIAN_POINT('Ctrl Pts',(-10.0514428414942,60.9312499997667,
2.46189346052968E-15));
#297617=CARTESIAN_POINT('Ctrl Pts',(-10.0514428414942,61.0812499997661,
3.26591175476071));
#297618=CARTESIAN_POINT('Ctrl Pts',(-8.13178807675724,61.2312499997655,
5.90808986649102));
#297619=CARTESIAN_POINT('Ctrl Pts',(-6.21213331202026,61.3812499997649,
8.55026797822134));
#297620=CARTESIAN_POINT('Ctrl Pts',(-3.10606665601015,61.5312499997643,
9.5594902125713));
#297621=CARTESIAN_POINT('Ctrl Pts',(-4.60586049427516E-14,61.6812499997638,
10.5687124469213));
#297622=CARTESIAN_POINT('Ctrl Pts',(3.10606665601006,61.8312499997632,9.5594902125713));
#297623=CARTESIAN_POINT('Ctrl Pts',(6.21213331202017,61.9812499997625,8.55026797822134));
#297624=CARTESIAN_POINT('Ctrl Pts',(8.13178807675714,62.131249999762,5.90808986649102));
#297625=CARTESIAN_POINT('Ctrl Pts',(10.0514428414941,62.2812499997614,3.2659117547607));
#297626=CARTESIAN_POINT('Ctrl Pts',(10.0514428414941,62.4312499997608,-1.23094673026484E-15));
#297627=CARTESIAN_POINT('Ctrl Pts',(10.0514428414941,62.5812499997602,-3.26591175476071));
#297628=CARTESIAN_POINT('Ctrl Pts',(8.13178807675714,62.7312499997596,-5.90808986649102));
#297629=CARTESIAN_POINT('Ctrl Pts',(6.21213331202017,62.881249999759,-8.55026797822134));
#297630=CARTESIAN_POINT('Ctrl Pts',(3.10606665601006,63.0312499997584,-9.5594902125713));
#297631=CARTESIAN_POINT('Ctrl Pts',(-4.95110475524287E-14,63.1812499997578,
-10.5687124469213));
#297632=CARTESIAN_POINT('Ctrl Pts',(-3.10606665601016,63.3312499997572,
-9.5594902125713));
#297633=CARTESIAN_POINT('Ctrl Pts',(-6.21213331202027,63.4812499997565,
-8.55026797822134));
#297634=CARTESIAN_POINT('Ctrl Pts',(-8.13178807675724,63.631249999756,-5.90808986649102));
#297635=CARTESIAN_POINT('Ctrl Pts',(-10.0514428414942,63.7812499997553,
-3.2659117547607));
#297636=CARTESIAN_POINT('Ctrl Pts',(-10.0514428414942,63.9312499997548,
2.46189346052968E-15));
#297637=CARTESIAN_POINT('Ctrl Pts',(-10.0514428414942,64.0812499997541,
3.26591175476071));
#297638=CARTESIAN_POINT('Ctrl Pts',(-8.13178807675724,64.2312499997535,
5.90808986649102));
#297639=CARTESIAN_POINT('Ctrl Pts',(-6.21213331202026,64.381249999753,8.55026797822134));
#297640=CARTESIAN_POINT('Ctrl Pts',(-3.10606665601016,64.5312499997523,
9.5594902125713));
#297641=CARTESIAN_POINT('Ctrl Pts',(-4.77863142144134E-14,64.6812499997518,
10.5687124469213));
#297642=CARTESIAN_POINT('Ctrl Pts',(3.10606665601006,64.8312499997512,9.5594902125713));
#297643=CARTESIAN_POINT('Ctrl Pts',(6.21213331202017,64.9812499997506,8.55026797822134));
#297644=CARTESIAN_POINT('Ctrl Pts',(8.13178807675714,65.13124999975,5.90808986649102));
#297645=CARTESIAN_POINT('Ctrl Pts',(10.0514428414941,65.2812499997493,3.2659117547607));
#297646=CARTESIAN_POINT('Ctrl Pts',(10.0514428414941,65.4312499997488,-1.23094673026484E-15));
#297647=CARTESIAN_POINT('Ctrl Pts',(10.0514428414941,65.5812499997482,-3.26591175476071));
#297648=CARTESIAN_POINT('Ctrl Pts',(8.13178807675714,65.7312499997475,-5.90808986649102));
#297649=CARTESIAN_POINT('Ctrl Pts',(6.21213331202016,65.881249999747,-8.55026797822134));
#297650=CARTESIAN_POINT('Ctrl Pts',(3.10606665601006,66.0312499997464,-9.5594902125713));
#297651=CARTESIAN_POINT('Ctrl Pts',(-5.12387568240905E-14,66.1812499997457,
-10.5687124469213));
#297652=CARTESIAN_POINT('Ctrl Pts',(-3.10606665601016,66.3312499997451,
-9.5594902125713));
#297653=CARTESIAN_POINT('Ctrl Pts',(-6.21213331202027,66.4812499997445,
-8.55026797822134));
#297654=CARTESIAN_POINT('Ctrl Pts',(-8.13178807675724,66.6312499997439,
-5.90808986649102));
#297655=CARTESIAN_POINT('Ctrl Pts',(-10.0514428414942,66.7812499997433,
-3.2659117547607));
#297656=CARTESIAN_POINT('Ctrl Pts',(-10.0514428414942,66.9312499997427,
2.46189346052968E-15));
#297657=CARTESIAN_POINT('Ctrl Pts',(-10.0514428414942,67.0812499997421,
3.26591175476071));
#297658=CARTESIAN_POINT('Ctrl Pts',(-8.13178807675724,67.2312499997416,
5.90808986649102));
#297659=CARTESIAN_POINT('Ctrl Pts',(-6.21213331202027,67.3812499997409,
8.55026797822134));
#297660=CARTESIAN_POINT('Ctrl Pts',(-3.10606665601016,67.5312499997404,
9.5594902125713));
#297661=CARTESIAN_POINT('Ctrl Pts',(-4.95140234860752E-14,67.6812499997397,
10.5687124469213));
#297662=CARTESIAN_POINT('Ctrl Pts',(3.10606665601006,67.8312499997391,9.5594902125713));
#297663=CARTESIAN_POINT('Ctrl Pts',(6.21213331202017,67.9812499997385,8.55026797822134));
#297664=CARTESIAN_POINT('Ctrl Pts',(8.13178807675714,68.1312499997379,5.90808986649102));
#297665=CARTESIAN_POINT('Ctrl Pts',(10.0514428414941,68.2812499997374,3.2659117547607));
#297666=CARTESIAN_POINT('Ctrl Pts',(10.0514428414941,68.4312499997367,-1.23094673026484E-15));
#297667=CARTESIAN_POINT('Ctrl Pts',(10.0514428414941,68.5812499997361,-3.26591175476071));
#297668=CARTESIAN_POINT('Ctrl Pts',(8.13178807675714,68.7312499997356,-5.90808986649102));
#297669=CARTESIAN_POINT('Ctrl Pts',(6.21213331202016,68.881249999735,-8.55026797822134));
#297670=CARTESIAN_POINT('Ctrl Pts',(3.10606665601006,69.0312499997344,-9.5594902125713));
#297671=CARTESIAN_POINT('Ctrl Pts',(-5.29664660957524E-14,69.1812499997337,
-10.5687124469213));
#297672=CARTESIAN_POINT('Ctrl Pts',(-3.10606665601016,69.3312499997332,
-9.5594902125713));
#297673=CARTESIAN_POINT('Ctrl Pts',(-6.21213331202027,69.4812499997326,
-8.55026797822134));
#297674=CARTESIAN_POINT('Ctrl Pts',(-8.13178807675724,69.6312499997319,
-5.90808986649102));
#297675=CARTESIAN_POINT('Ctrl Pts',(-10.0514428414942,69.7812499997313,
-3.2659117547607));
#297676=CARTESIAN_POINT('Ctrl Pts',(-10.0514428414942,69.9312499997307,
2.46189346052968E-15));
#297677=CARTESIAN_POINT('Ctrl Pts',(-10.0514428414942,70.0812499997301,
3.26591175476071));
#297678=CARTESIAN_POINT('Ctrl Pts',(-8.13178807675724,70.2312499997295,
5.90808986649102));
#297679=CARTESIAN_POINT('Ctrl Pts',(-6.21213331202027,70.3812499997289,
8.55026797822134));
#297680=CARTESIAN_POINT('Ctrl Pts',(-3.10606665601016,70.5312499997283,
9.5594902125713));
#297681=CARTESIAN_POINT('Ctrl Pts',(-5.12417327577371E-14,70.6812499997277,
10.5687124469213));
#297682=CARTESIAN_POINT('Ctrl Pts',(3.10606665601006,70.8312499997271,9.5594902125713));
#297683=CARTESIAN_POINT('Ctrl Pts',(6.21213331202016,70.9812499997265,8.55026797822134));
#297684=CARTESIAN_POINT('Ctrl Pts',(8.13178807675714,71.131249999726,5.90808986649102));
#297685=CARTESIAN_POINT('Ctrl Pts',(10.0514428414941,71.2812499997253,3.2659117547607));
#297686=CARTESIAN_POINT('Ctrl Pts',(10.0514428414941,71.4312499997248,-1.23094673026484E-15));
#297687=CARTESIAN_POINT('Ctrl Pts',(10.0514428414941,71.5812499997242,-3.26591175476071));
#297688=CARTESIAN_POINT('Ctrl Pts',(8.13178807675713,71.7312499997236,-5.90808986649102));
#297689=CARTESIAN_POINT('Ctrl Pts',(6.21213331202016,71.881249999723,-8.55026797822134));
#297690=CARTESIAN_POINT('Ctrl Pts',(3.10606665601005,72.0312499997223,-9.5594902125713));
#297691=CARTESIAN_POINT('Ctrl Pts',(-5.46941753674142E-14,72.1812499997217,
-10.5687124469213));
#297692=CARTESIAN_POINT('Ctrl Pts',(-3.10606665601016,72.3312499997212,
-9.5594902125713));
#297693=CARTESIAN_POINT('Ctrl Pts',(-6.21213331202027,72.4812499997205,
-8.55026797822134));
#297694=CARTESIAN_POINT('Ctrl Pts',(-8.13178807675725,72.63124999972,-5.90808986649102));
#297695=CARTESIAN_POINT('Ctrl Pts',(-10.0514428414942,72.7812499997193,
-3.2659117547607));
#297696=CARTESIAN_POINT('Ctrl Pts',(-10.0514428414942,72.9312499997187,
2.46189346052968E-15));
#297697=CARTESIAN_POINT('Ctrl Pts',(-10.0514428414942,73.0812499997181,
3.26591175476071));
#297698=CARTESIAN_POINT('Ctrl Pts',(-8.13178807675725,73.2312499997175,
5.90808986649102));
#297699=CARTESIAN_POINT('Ctrl Pts',(-6.21213331202027,73.381249999717,8.55026797822134));
#297700=CARTESIAN_POINT('Ctrl Pts',(-3.10606665601016,73.5312499997164,
9.5594902125713));
#297701=CARTESIAN_POINT('Ctrl Pts',(-5.29694420293989E-14,73.6812499997157,
10.5687124469213));
#297702=CARTESIAN_POINT('Ctrl Pts',(3.10606665601005,73.8312499997151,9.5594902125713));
#297703=CARTESIAN_POINT('Ctrl Pts',(6.21213331202016,73.9812499997146,8.55026797822134));
#297704=CARTESIAN_POINT('Ctrl Pts',(8.13178807675713,74.1312499997139,5.90808986649102));
#297705=CARTESIAN_POINT('Ctrl Pts',(10.0514428414941,74.2812499997134,3.2659117547607));
#297706=CARTESIAN_POINT('Ctrl Pts',(10.0514428414941,74.4312499997127,-1.23094673026484E-15));
#297707=CARTESIAN_POINT('Ctrl Pts',(10.0514428414941,74.5812499997122,-3.26591175476071));
#297708=CARTESIAN_POINT('Ctrl Pts',(8.13178807675713,74.7312499997116,-5.90808986649102));
#297709=CARTESIAN_POINT('Ctrl Pts',(6.21213331202016,74.8812499997109,-8.55026797822134));
#297710=CARTESIAN_POINT('Ctrl Pts',(3.10606665601005,75.0312499997104,-9.5594902125713));
#297711=CARTESIAN_POINT('Ctrl Pts',(-5.6421884639076E-14,75.1812499997098,
-10.5687124469213));
#297712=CARTESIAN_POINT('Ctrl Pts',(-3.10606665601016,75.3312499997092,
-9.5594902125713));
#297713=CARTESIAN_POINT('Ctrl Pts',(-6.21213331202027,75.4812499997086,
-8.55026797822134));
#297714=CARTESIAN_POINT('Ctrl Pts',(-8.13178807675725,75.6312499997079,
-5.90808986649102));
#297715=CARTESIAN_POINT('Ctrl Pts',(-10.0514428414942,75.7812499997073,
-3.2659117547607));
#297716=CARTESIAN_POINT('Ctrl Pts',(-10.0514428414942,75.9312499997068,
2.46189346052968E-15));
#297717=CARTESIAN_POINT('Ctrl Pts',(-10.0514428414942,76.0812499997061,
3.26591175476071));
#297718=CARTESIAN_POINT('Ctrl Pts',(-8.13178807675725,76.2312499997055,
5.90808986649102));
#297719=CARTESIAN_POINT('Ctrl Pts',(-6.21213331202027,76.3812499997049,
8.55026797822134));
#297720=CARTESIAN_POINT('Ctrl Pts',(-3.10606665601016,76.5312499997043,
9.5594902125713));
#297721=CARTESIAN_POINT('Ctrl Pts',(-5.46971513010608E-14,76.6812499997037,
10.5687124469213));
#297722=CARTESIAN_POINT('Ctrl Pts',(3.10606665601005,76.8312499997031,9.5594902125713));
#297723=CARTESIAN_POINT('Ctrl Pts',(6.21213331202016,76.9812499997025,8.55026797822134));
#297724=CARTESIAN_POINT('Ctrl Pts',(8.13178807675713,77.131249999702,5.90808986649102));
#297725=CARTESIAN_POINT('Ctrl Pts',(10.0514428414941,77.2812499997013,3.2659117547607));
#297726=CARTESIAN_POINT('Ctrl Pts',(10.0514428414941,77.4312499997008,-1.23094673026484E-15));
#297727=CARTESIAN_POINT('Ctrl Pts',(10.0514428414941,77.5812499997001,-3.26591175476071));
#297728=CARTESIAN_POINT('Ctrl Pts',(8.13178807675713,77.7312499996995,-5.90808986649102));
#297729=CARTESIAN_POINT('Ctrl Pts',(6.21213331202016,77.881249999699,-8.55026797822134));
#297730=CARTESIAN_POINT('Ctrl Pts',(3.10606665601005,78.0312499996984,-9.5594902125713));
#297731=CARTESIAN_POINT('Ctrl Pts',(-5.81495939107379E-14,78.1812499996978,
-10.5687124469213));
#297732=CARTESIAN_POINT('Ctrl Pts',(-3.10606665601017,78.3312499996971,
-9.5594902125713));
#297733=CARTESIAN_POINT('Ctrl Pts',(-6.21213331202028,78.4812499996966,
-8.55026797822134));
#297734=CARTESIAN_POINT('Ctrl Pts',(-8.13178807675725,78.631249999696,-5.90808986649102));
#297735=CARTESIAN_POINT('Ctrl Pts',(-10.0514428414942,78.7812499996954,
-3.2659117547607));
#297736=CARTESIAN_POINT('Ctrl Pts',(-10.0514428414942,78.9312499996948,
2.46189346052968E-15));
#297737=CARTESIAN_POINT('Ctrl Pts',(-10.0514428414942,79.0812499996942,
3.26591175476071));
#297738=CARTESIAN_POINT('Ctrl Pts',(-8.13178807675725,79.2312499996936,
5.90808986649102));
#297739=CARTESIAN_POINT('Ctrl Pts',(-6.21213331202027,79.381249999693,8.55026797822134));
#297740=CARTESIAN_POINT('Ctrl Pts',(-3.10606665601016,79.5312499996923,
9.5594902125713));
#297741=CARTESIAN_POINT('Ctrl Pts',(-5.64248605727226E-14,79.6812499996917,
10.5687124469213));
#297742=CARTESIAN_POINT('Ctrl Pts',(3.10606665601005,79.8312499996911,9.5594902125713));
#297743=CARTESIAN_POINT('Ctrl Pts',(6.21213331202016,79.9812499996905,8.55026797822134));
#297744=CARTESIAN_POINT('Ctrl Pts',(8.13178807675713,80.1312499996899,5.90808986649102));
#297745=CARTESIAN_POINT('Ctrl Pts',(10.0514428414941,80.2812499996894,3.2659117547607));
#297746=CARTESIAN_POINT('Ctrl Pts',(10.0514428414941,80.4312499996887,-1.23094673026484E-15));
#297747=CARTESIAN_POINT('Ctrl Pts',(10.0514428414941,80.5812499996882,-3.26591175476071));
#297748=CARTESIAN_POINT('Ctrl Pts',(8.13178807675713,80.7312499996875,-5.90808986649102));
#297749=CARTESIAN_POINT('Ctrl Pts',(6.21213331202016,80.881249999687,-8.55026797822134));
#297750=CARTESIAN_POINT('Ctrl Pts',(3.10606665601005,81.0312499996864,-9.5594902125713));
#297751=CARTESIAN_POINT('Ctrl Pts',(-5.98773031823997E-14,81.1812499996858,
-10.5687124469213));
#297752=CARTESIAN_POINT('Ctrl Pts',(-3.10606665601017,81.3312499996851,
-9.5594902125713));
#297753=CARTESIAN_POINT('Ctrl Pts',(-6.21213331202028,81.4812499996845,
-8.55026797822134));
#297754=CARTESIAN_POINT('Ctrl Pts',(-8.13178807675725,81.6312499996839,
-5.90808986649102));
#297755=CARTESIAN_POINT('Ctrl Pts',(-10.0514428414942,81.7812499996834,
-3.2659117547607));
#297756=CARTESIAN_POINT('Ctrl Pts',(-10.0514428414942,81.9312499996827,
2.46189346052968E-15));
#297757=CARTESIAN_POINT('Ctrl Pts',(-10.0514428414942,82.0812499996821,
3.26591175476071));
#297758=CARTESIAN_POINT('Ctrl Pts',(-8.13178807675725,82.2312499996816,
5.90808986649102));
#297759=CARTESIAN_POINT('Ctrl Pts',(-6.21213331202028,82.381249999681,8.55026797822134));
#297760=CARTESIAN_POINT('Ctrl Pts',(-3.10606665601017,82.5312499996804,
9.5594902125713));
#297761=CARTESIAN_POINT('Ctrl Pts',(-5.81525698443845E-14,82.6812499996797,
10.5687124469213));
#297762=CARTESIAN_POINT('Ctrl Pts',(3.10606665601005,82.8312499996792,9.5594902125713));
#297763=CARTESIAN_POINT('Ctrl Pts',(6.21213331202016,82.9812499996786,8.55026797822134));
#297764=CARTESIAN_POINT('Ctrl Pts',(8.13178807675713,83.131249999678,5.90808986649102));
#297765=CARTESIAN_POINT('Ctrl Pts',(10.0514428414941,83.2812499996773,3.2659117547607));
#297766=CARTESIAN_POINT('Ctrl Pts',(10.0514428414941,83.4312499996767,-1.23094673026484E-15));
#297767=CARTESIAN_POINT('Ctrl Pts',(10.0514428414941,83.5812499996761,-3.26591175476071));
#297768=CARTESIAN_POINT('Ctrl Pts',(8.13178807675713,83.7312499996756,-5.90808986649102));
#297769=CARTESIAN_POINT('Ctrl Pts',(6.21213331202016,83.8812499996749,-8.55026797822134));
#297770=CARTESIAN_POINT('Ctrl Pts',(3.10606665601005,84.0312499996743,-9.5594902125713));
#297771=CARTESIAN_POINT('Ctrl Pts',(-6.16050124540615E-14,84.1812499996738,
-10.5687124469213));
#297772=CARTESIAN_POINT('Ctrl Pts',(-3.10606665601017,84.3312499996732,
-9.5594902125713));
#297773=CARTESIAN_POINT('Ctrl Pts',(-6.21213331202028,84.4812499996725,
-8.55026797822134));
#297774=CARTESIAN_POINT('Ctrl Pts',(-8.13178807675725,84.631249999672,-5.90808986649102));
#297775=CARTESIAN_POINT('Ctrl Pts',(-10.0514428414942,84.7812499996714,
-3.2659117547607));
#297776=CARTESIAN_POINT('Ctrl Pts',(-10.0514428414942,84.9312499996708,
2.46189346052968E-15));
#297777=CARTESIAN_POINT('Ctrl Pts',(-10.0514428414942,85.0812499996701,
3.26591175476071));
#297778=CARTESIAN_POINT('Ctrl Pts',(-8.13178807675725,85.2312499996695,
5.90808986649102));
#297779=CARTESIAN_POINT('Ctrl Pts',(-6.21213331202028,85.381249999669,8.55026797822134));
#297780=CARTESIAN_POINT('Ctrl Pts',(-3.10606665601017,85.5312499996683,
9.5594902125713));
#297781=CARTESIAN_POINT('Ctrl Pts',(-5.98802791160463E-14,85.6812499996678,
10.5687124469213));
#297782=CARTESIAN_POINT('Ctrl Pts',(3.10606665601005,85.8312499996672,9.5594902125713));
#297783=CARTESIAN_POINT('Ctrl Pts',(6.21213331202016,85.9812499996666,8.55026797822134));
#297784=CARTESIAN_POINT('Ctrl Pts',(8.13178807675713,86.1312499996659,5.90808986649102));
#297785=CARTESIAN_POINT('Ctrl Pts',(10.0514428414941,86.2812499996653,3.2659117547607));
#297786=CARTESIAN_POINT('Ctrl Pts',(10.0514428414941,86.4312499996647,-1.23094673026484E-15));
#297787=CARTESIAN_POINT('Ctrl Pts',(10.0514428414941,86.5812499996642,-3.26591175476071));
#297788=CARTESIAN_POINT('Ctrl Pts',(8.13178807675713,86.7312499996635,-5.90808986649102));
#297789=CARTESIAN_POINT('Ctrl Pts',(6.21213331202015,86.8812499996629,-8.55026797822134));
#297790=CARTESIAN_POINT('Ctrl Pts',(3.10606665601004,87.0312499996624,-9.5594902125713));
#297791=CARTESIAN_POINT('Ctrl Pts',(-6.33327217257234E-14,87.1812499996618,
-10.5687124469213));
#297792=CARTESIAN_POINT('Ctrl Pts',(-3.10606665601017,87.3312499996611,
-9.5594902125713));
#297793=CARTESIAN_POINT('Ctrl Pts',(-6.21213331202028,87.4812499996605,
-8.55026797822134));
#297794=CARTESIAN_POINT('Ctrl Pts',(-8.13178807675726,87.6312499996599,
-5.90808986649102));
#297795=CARTESIAN_POINT('Ctrl Pts',(-10.0514428414942,87.7812499996594,
-3.2659117547607));
#297796=CARTESIAN_POINT('Ctrl Pts',(-10.0514428414942,87.9312499996587,
2.46189346052968E-15));
#297797=CARTESIAN_POINT('Ctrl Pts',(-10.0514428414942,88.0812499996581,
3.26591175476071));
#297798=CARTESIAN_POINT('Ctrl Pts',(-8.13178807675726,88.2312499996575,
5.90808986649102));
#297799=CARTESIAN_POINT('Ctrl Pts',(-6.21213331202028,88.3812499996569,
8.55026797822134));
#297800=CARTESIAN_POINT('Ctrl Pts',(-3.10606665601017,88.5312499996564,
9.5594902125713));
#297801=CARTESIAN_POINT('Ctrl Pts',(-6.16079883877081E-14,88.6812499996557,
10.5687124469213));
#297802=CARTESIAN_POINT('Ctrl Pts',(3.10606665601005,88.8312499996552,9.5594902125713));
#297803=CARTESIAN_POINT('Ctrl Pts',(6.21213331202016,88.9812499996546,8.55026797822134));
#297804=CARTESIAN_POINT('Ctrl Pts',(8.13178807675713,89.131249999654,5.90808986649102));
#297805=CARTESIAN_POINT('Ctrl Pts',(10.0514428414941,89.2812499996533,3.2659117547607));
#297806=CARTESIAN_POINT('Ctrl Pts',(10.0514428414941,89.4312499996527,-1.23094673026484E-15));
#297807=CARTESIAN_POINT('Ctrl Pts',(10.0514428414941,89.5812499996521,-3.26591175476071));
#297808=CARTESIAN_POINT('Ctrl Pts',(8.13178807675713,89.7312499996515,-5.90808986649102));
#297809=CARTESIAN_POINT('Ctrl Pts',(6.21213331202015,89.8812499996509,-8.55026797822134));
#297810=CARTESIAN_POINT('Ctrl Pts',(3.10606665601004,90.0312499996504,-9.5594902125713));
#297811=CARTESIAN_POINT('Ctrl Pts',(-6.50604309973852E-14,90.1812499996498,
-10.5687124469213));
#297812=CARTESIAN_POINT('Ctrl Pts',(-3.10606665601017,90.3312499996491,
-9.5594902125713));
#297813=CARTESIAN_POINT('Ctrl Pts',(-6.21213331202028,90.4812499996485,
-8.55026797822134));
#297814=CARTESIAN_POINT('Ctrl Pts',(-8.13178807675726,90.631249999648,-5.90808986649102));
#297815=CARTESIAN_POINT('Ctrl Pts',(-10.0514428414942,90.7812499996473,
-3.2659117547607));
#297816=CARTESIAN_POINT('Ctrl Pts',(-10.0514428414942,90.9312499996468,
2.46189346052968E-15));
#297817=CARTESIAN_POINT('Ctrl Pts',(-10.0514428414942,91.0812499996461,
3.26591175476071));
#297818=CARTESIAN_POINT('Ctrl Pts',(-8.13178807675726,91.2312499996455,
5.90808986649102));
#297819=CARTESIAN_POINT('Ctrl Pts',(-6.21213331202028,91.381249999645,8.55026797822134));
#297820=CARTESIAN_POINT('Ctrl Pts',(-3.10606665601017,91.5312499996443,
9.5594902125713));
#297821=CARTESIAN_POINT('Ctrl Pts',(-6.333569765937E-14,91.6812499996438,
10.5687124469213));
#297822=CARTESIAN_POINT('Ctrl Pts',(3.10606665601004,91.8312499996431,9.5594902125713));
#297823=CARTESIAN_POINT('Ctrl Pts',(6.21213331202015,91.9812499996426,8.55026797822134));
#297824=CARTESIAN_POINT('Ctrl Pts',(8.13178807675712,92.131249999642,5.90808986649102));
#297825=CARTESIAN_POINT('Ctrl Pts',(10.0514428414941,92.2812499996414,3.2659117547607));
#297826=CARTESIAN_POINT('Ctrl Pts',(10.0514428414941,92.4312499996408,-1.23094673026484E-15));
#297827=CARTESIAN_POINT('Ctrl Pts',(10.0514428414941,92.5812499996402,-3.26591175476071));
#297828=CARTESIAN_POINT('Ctrl Pts',(8.13178807675712,92.7312499996396,-5.90808986649102));
#297829=CARTESIAN_POINT('Ctrl Pts',(6.21213331202015,92.8812499996389,-8.55026797822134));
#297830=CARTESIAN_POINT('Ctrl Pts',(3.10606665601004,93.0312499996383,-9.5594902125713));
#297831=CARTESIAN_POINT('Ctrl Pts',(-6.67881402690471E-14,93.1812499996377,
-10.5687124469213));
#297832=CARTESIAN_POINT('Ctrl Pts',(-3.10606665601018,93.3312499996371,
-9.5594902125713));
#297833=CARTESIAN_POINT('Ctrl Pts',(-6.21213331202028,93.4812499996365,
-8.55026797822134));
#297834=CARTESIAN_POINT('Ctrl Pts',(-8.13178807675726,93.6312499996359,
-5.90808986649102));
#297835=CARTESIAN_POINT('Ctrl Pts',(-10.0514428414942,93.7812499996353,
-3.2659117547607));
#297836=CARTESIAN_POINT('Ctrl Pts',(-10.0514428414942,93.9312499996347,
2.46189346052968E-15));
#297837=CARTESIAN_POINT('Ctrl Pts',(-10.0514428414942,94.0812499996341,
3.26591175476071));
#297838=CARTESIAN_POINT('Ctrl Pts',(-8.13178807675726,94.2312499996335,
5.90808986649102));
#297839=CARTESIAN_POINT('Ctrl Pts',(-6.21213331202028,94.381249999633,8.55026797822134));
#297840=CARTESIAN_POINT('Ctrl Pts',(-3.10606665601017,94.5312499996324,
9.5594902125713));
#297841=CARTESIAN_POINT('Ctrl Pts',(-6.50634069310318E-14,94.6812499996317,
10.5687124469213));
#297842=CARTESIAN_POINT('Ctrl Pts',(3.10606665601004,94.8312499996312,9.5594902125713));
#297843=CARTESIAN_POINT('Ctrl Pts',(6.21213331202015,94.9812499996306,8.55026797822134));
#297844=CARTESIAN_POINT('Ctrl Pts',(8.13178807675712,95.13124999963,5.90808986649102));
#297845=CARTESIAN_POINT('Ctrl Pts',(10.0514428414941,95.2812499996293,3.2659117547607));
#297846=CARTESIAN_POINT('Ctrl Pts',(10.0514428414941,95.4312499996288,-1.23094673026484E-15));
#297847=CARTESIAN_POINT('Ctrl Pts',(10.0514428414941,95.5812499996282,-3.26591175476071));
#297848=CARTESIAN_POINT('Ctrl Pts',(8.13178807675712,95.7312499996276,-5.90808986649102));
#297849=CARTESIAN_POINT('Ctrl Pts',(6.21213331202015,95.8812499996269,-8.55026797822134));
#297850=CARTESIAN_POINT('Ctrl Pts',(3.10606665601004,96.0312499996264,-9.5594902125713));
#297851=CARTESIAN_POINT('Ctrl Pts',(-6.85158495407089E-14,96.1812499996257,
-10.5687124469213));
#297852=CARTESIAN_POINT('Ctrl Pts',(-3.10606665601018,96.3312499996252,
-9.5594902125713));
#297853=CARTESIAN_POINT('Ctrl Pts',(-6.21213331202028,96.4812499996245,
-8.55026797822134));
#297854=CARTESIAN_POINT('Ctrl Pts',(-8.13178807675726,96.6312499996239,
-5.90808986649102));
#297855=CARTESIAN_POINT('Ctrl Pts',(-10.0514428414942,96.7812499996234,
-3.2659117547607));
#297856=CARTESIAN_POINT('Ctrl Pts',(-10.0514428414942,96.9312499996227,
2.46189346052968E-15));
#297857=CARTESIAN_POINT('Ctrl Pts',(-10.0514428414942,97.0812499996221,
3.26591175476071));
#297858=CARTESIAN_POINT('Ctrl Pts',(-8.13178807675726,97.2312499996215,
5.90808986649102));
#297859=CARTESIAN_POINT('Ctrl Pts',(-6.21213331202028,97.381249999621,8.55026797822134));
#297860=CARTESIAN_POINT('Ctrl Pts',(-3.10606665601017,97.5312499996203,
9.5594902125713));
#297861=CARTESIAN_POINT('Ctrl Pts',(-6.67911162026936E-14,97.6812499996197,
10.5687124469213));
#297862=CARTESIAN_POINT('Ctrl Pts',(3.10606665601004,97.8312499996191,9.5594902125713));
#297863=CARTESIAN_POINT('Ctrl Pts',(6.21213331202015,97.9812499996186,8.55026797822134));
#297864=CARTESIAN_POINT('Ctrl Pts',(8.13178807675712,98.1312499996179,5.90808986649102));
#297865=CARTESIAN_POINT('Ctrl Pts',(10.0514428414941,98.2812499996173,3.2659117547607));
#297866=CARTESIAN_POINT('Ctrl Pts',(10.0514428414941,98.4312499996168,-1.23094673026484E-15));
#297867=CARTESIAN_POINT('Ctrl Pts',(10.0514428414941,98.5812499996162,-3.26591175476071));
#297868=CARTESIAN_POINT('Ctrl Pts',(8.13178807675712,98.7312499996156,-5.90808986649102));
#297869=CARTESIAN_POINT('Ctrl Pts',(6.21213331202015,98.8812499996149,-8.55026797822134));
#297870=CARTESIAN_POINT('Ctrl Pts',(3.10606665601004,99.0312499996143,-9.5594902125713));
#297871=CARTESIAN_POINT('Ctrl Pts',(-7.02435588123707E-14,99.1812499996138,
-10.5687124469213));
#297872=CARTESIAN_POINT('Ctrl Pts',(-3.10606665601018,99.3312499996131,
-9.5594902125713));
#297873=CARTESIAN_POINT('Ctrl Pts',(-6.21213331202028,99.4812499996125,
-8.55026797822134));
#297874=CARTESIAN_POINT('Ctrl Pts',(-8.13178807675726,99.631249999612,-5.90808986649102));
#297875=CARTESIAN_POINT('Ctrl Pts',(-10.0514428414942,99.7812499996113,
-3.2659117547607));
#297876=CARTESIAN_POINT('Ctrl Pts',(-10.0514428414942,99.9312499996108,
2.46189346052968E-15));
#297877=CARTESIAN_POINT('Ctrl Pts',(-10.0514428414942,100.08124999961,3.26591175476071));
#297878=CARTESIAN_POINT('Ctrl Pts',(-8.13178807675726,100.23124999961,5.90808986649102));
#297879=CARTESIAN_POINT('Ctrl Pts',(-6.21213331202028,100.381249999609,
8.55026797822134));
#297880=CARTESIAN_POINT('Ctrl Pts',(-3.10606665601018,100.531249999608,
9.5594902125713));
#297881=CARTESIAN_POINT('Ctrl Pts',(-6.85188254743555E-14,100.681249999608,
10.5687124469213));
#297882=CARTESIAN_POINT('Ctrl Pts',(3.10606665601004,100.831249999607,9.5594902125713));
#297883=CARTESIAN_POINT('Ctrl Pts',(6.21213331202015,100.981249999607,8.55026797822134));
#297884=CARTESIAN_POINT('Ctrl Pts',(8.13178807675712,101.131249999606,5.90808986649102));
#297885=CARTESIAN_POINT('Ctrl Pts',(10.0514428414941,101.281249999605,3.2659117547607));
#297886=CARTESIAN_POINT('Ctrl Pts',(10.0514428414941,101.431249999605,-1.23094673026484E-15));
#297887=CARTESIAN_POINT('Ctrl Pts',(10.0514428414941,101.581249999604,-3.26591175476071));
#297888=CARTESIAN_POINT('Ctrl Pts',(8.13178807675712,101.731249999604,-5.90808986649102));
#297889=CARTESIAN_POINT('Ctrl Pts',(6.21213331202014,101.881249999603,-8.55026797822134));
#297890=CARTESIAN_POINT('Ctrl Pts',(3.10606665601004,102.031249999602,-9.5594902125713));
#297891=CARTESIAN_POINT('Ctrl Pts',(-7.19712680840326E-14,102.181249999602,
-10.5687124469213));
#297892=CARTESIAN_POINT('Ctrl Pts',(-3.10606665601018,102.331249999601,
-9.5594902125713));
#297893=CARTESIAN_POINT('Ctrl Pts',(-6.21213331202029,102.481249999601,
-8.55026797822134));
#297894=CARTESIAN_POINT('Ctrl Pts',(-8.13178807675726,102.6312499996,-5.90808986649102));
#297895=CARTESIAN_POINT('Ctrl Pts',(-10.0514428414942,102.781249999599,
-3.2659117547607));
#297896=CARTESIAN_POINT('Ctrl Pts',(-10.0514428414942,102.931249999599,
2.46189346052968E-15));
#297897=CARTESIAN_POINT('Ctrl Pts',(-10.0514428414942,103.081249999598,
3.26591175476071));
#297898=CARTESIAN_POINT('Ctrl Pts',(-8.13178807675726,103.231249999598,
5.90808986649102));
#297899=CARTESIAN_POINT('Ctrl Pts',(-6.21213331202028,103.381249999597,
8.55026797822134));
#297900=CARTESIAN_POINT('Ctrl Pts',(-3.10606665601018,103.531249999596,
9.5594902125713));
#297901=CARTESIAN_POINT('Ctrl Pts',(-7.02465347460173E-14,103.681249999596,
10.5687124469213));
#297902=CARTESIAN_POINT('Ctrl Pts',(3.10606665601004,103.831249999595,9.5594902125713));
#297903=CARTESIAN_POINT('Ctrl Pts',(6.21213331202015,103.981249999595,8.55026797822134));
#297904=CARTESIAN_POINT('Ctrl Pts',(8.13178807675712,104.131249999594,5.90808986649102));
#297905=CARTESIAN_POINT('Ctrl Pts',(10.0514428414941,104.281249999593,3.2659117547607));
#297906=CARTESIAN_POINT('Ctrl Pts',(10.0514428414941,104.431249999593,-1.23094673026484E-15));
#297907=CARTESIAN_POINT('Ctrl Pts',(10.0514428414941,104.581249999592,-3.26591175476071));
#297908=CARTESIAN_POINT('Ctrl Pts',(8.13178807675712,104.731249999592,-5.90808986649102));
#297909=CARTESIAN_POINT('Ctrl Pts',(6.21213331202014,104.881249999591,-8.55026797822134));
#297910=CARTESIAN_POINT('Ctrl Pts',(3.10606665601003,105.03124999959,-9.5594902125713));
#297911=CARTESIAN_POINT('Ctrl Pts',(-7.36989773556944E-14,105.18124999959,
-10.5687124469213));
#297912=CARTESIAN_POINT('Ctrl Pts',(-3.10606665601018,105.331249999589,
-9.5594902125713));
#297913=CARTESIAN_POINT('Ctrl Pts',(-6.21213331202029,105.481249999589,
-8.55026797822134));
#297914=CARTESIAN_POINT('Ctrl Pts',(-8.13178807675726,105.631249999588,
-5.90808986649102));
#297915=CARTESIAN_POINT('Ctrl Pts',(-10.0514428414942,105.781249999587,
-3.2659117547607));
#297916=CARTESIAN_POINT('Ctrl Pts',(-10.0514428414942,105.931249999587,
2.46189346052968E-15));
#297917=CARTESIAN_POINT('Ctrl Pts',(-10.0514428414942,106.081249999586,
3.26591175476071));
#297918=CARTESIAN_POINT('Ctrl Pts',(-8.13178807675726,106.231249999586,
5.90808986649102));
#297919=CARTESIAN_POINT('Ctrl Pts',(-6.21213331202029,106.381249999585,
8.55026797822134));
#297920=CARTESIAN_POINT('Ctrl Pts',(-3.10606665601018,106.531249999584,
9.5594902125713));
#297921=CARTESIAN_POINT('Ctrl Pts',(-7.19742440176792E-14,106.681249999584,
10.5687124469213));
#297922=CARTESIAN_POINT('Ctrl Pts',(3.10606665601004,106.831249999583,9.5594902125713));
#297923=CARTESIAN_POINT('Ctrl Pts',(6.21213331202014,106.981249999583,8.55026797822134));
#297924=CARTESIAN_POINT('Ctrl Pts',(8.13178807675711,107.131249999582,5.90808986649102));
#297925=CARTESIAN_POINT('Ctrl Pts',(10.0514428414941,107.281249999581,3.2659117547607));
#297926=CARTESIAN_POINT('Ctrl Pts',(10.0514428414941,107.431249999581,-1.23094673026484E-15));
#297927=CARTESIAN_POINT('Ctrl Pts',(10.0514428414941,107.58124999958,-3.26591175476071));
#297928=CARTESIAN_POINT('Ctrl Pts',(8.13178807675711,107.73124999958,-5.90808986649102));
#297929=CARTESIAN_POINT('Ctrl Pts',(6.21213331202014,107.881249999579,-8.55026797822134));
#297930=CARTESIAN_POINT('Ctrl Pts',(3.10606665601003,108.031249999578,-9.5594902125713));
#297931=CARTESIAN_POINT('Ctrl Pts',(-7.54266866273562E-14,108.181249999578,
-10.5687124469213));
#297932=CARTESIAN_POINT('Ctrl Pts',(-3.10606665601018,108.331249999577,
-9.5594902125713));
#297933=CARTESIAN_POINT('Ctrl Pts',(-6.21213331202029,108.481249999577,
-8.55026797822134));
#297934=CARTESIAN_POINT('Ctrl Pts',(-8.13178807675727,108.631249999576,
-5.90808986649102));
#297935=CARTESIAN_POINT('Ctrl Pts',(-10.0514428414942,108.781249999575,
-3.2659117547607));
#297936=CARTESIAN_POINT('Ctrl Pts',(-10.0514428414942,108.931249999575,
2.46189346052968E-15));
#297937=CARTESIAN_POINT('Ctrl Pts',(-10.0514428414942,109.081249999574,
3.26591175476071));
#297938=CARTESIAN_POINT('Ctrl Pts',(-8.13178807675727,109.231249999574,
5.90808986649102));
#297939=CARTESIAN_POINT('Ctrl Pts',(-6.21213331202029,109.381249999573,
8.55026797822134));
#297940=CARTESIAN_POINT('Ctrl Pts',(-3.10606665601018,109.531249999572,
9.5594902125713));
#297941=CARTESIAN_POINT('Ctrl Pts',(-7.3701953289341E-14,109.681249999572,
10.5687124469213));
#297942=CARTESIAN_POINT('Ctrl Pts',(3.10606665601003,109.831249999571,9.5594902125713));
#297943=CARTESIAN_POINT('Ctrl Pts',(6.21213331202014,109.981249999571,8.55026797822134));
#297944=CARTESIAN_POINT('Ctrl Pts',(8.13178807675711,110.13124999957,5.90808986649102));
#297945=CARTESIAN_POINT('Ctrl Pts',(10.0514428414941,110.281249999569,3.2659117547607));
#297946=CARTESIAN_POINT('Ctrl Pts',(10.0514428414941,110.431249999569,-1.23094673026484E-15));
#297947=CARTESIAN_POINT('Ctrl Pts',(10.0514428414941,110.581249999568,-3.26591175476071));
#297948=CARTESIAN_POINT('Ctrl Pts',(8.13178807675711,110.731249999568,-5.90808986649102));
#297949=CARTESIAN_POINT('Ctrl Pts',(6.21213331202014,110.881249999567,-8.55026797822134));
#297950=CARTESIAN_POINT('Ctrl Pts',(3.10606665601003,111.031249999566,-9.5594902125713));
#297951=CARTESIAN_POINT('Ctrl Pts',(-7.71543958990181E-14,111.181249999566,
-10.5687124469213));
#297952=CARTESIAN_POINT('Ctrl Pts',(-3.10606665601019,111.331249999565,
-9.5594902125713));
#297953=CARTESIAN_POINT('Ctrl Pts',(-6.21213331202029,111.481249999565,
-8.55026797822134));
#297954=CARTESIAN_POINT('Ctrl Pts',(-8.13178807675727,111.631249999564,
-5.90808986649102));
#297955=CARTESIAN_POINT('Ctrl Pts',(-10.0514428414942,111.781249999563,
-3.2659117547607));
#297956=CARTESIAN_POINT('Ctrl Pts',(-10.0514428414942,111.931249999563,
2.46189346052968E-15));
#297957=CARTESIAN_POINT('Ctrl Pts',(-10.0514428414942,112.081249999562,
3.26591175476071));
#297958=CARTESIAN_POINT('Ctrl Pts',(-8.13178807675727,112.231249999562,
5.90808986649102));
#297959=CARTESIAN_POINT('Ctrl Pts',(-6.21213331202029,112.381249999561,
8.55026797822134));
#297960=CARTESIAN_POINT('Ctrl Pts',(-3.10606665601018,112.53124999956,9.5594902125713));
#297961=CARTESIAN_POINT('Ctrl Pts',(-7.54296625610028E-14,112.68124999956,
10.5687124469213));
#297962=CARTESIAN_POINT('Ctrl Pts',(3.10606665601003,112.831249999559,9.5594902125713));
#297963=CARTESIAN_POINT('Ctrl Pts',(6.21213331202014,112.981249999559,8.55026797822134));
#297964=CARTESIAN_POINT('Ctrl Pts',(8.13178807675711,113.131249999558,5.90808986649102));
#297965=CARTESIAN_POINT('Ctrl Pts',(10.0514428414941,113.281249999557,3.2659117547607));
#297966=CARTESIAN_POINT('Ctrl Pts',(10.0514428414941,113.431249999557,-1.23094673026484E-15));
#297967=CARTESIAN_POINT('Ctrl Pts',(10.0514428414941,113.581249999556,-3.26591175476071));
#297968=CARTESIAN_POINT('Ctrl Pts',(8.13178807675711,113.731249999556,-5.90808986649102));
#297969=CARTESIAN_POINT('Ctrl Pts',(6.21213331202014,113.881249999555,-8.55026797822134));
#297970=CARTESIAN_POINT('Ctrl Pts',(3.10606665601003,114.031249999554,-9.5594902125713));
#297971=CARTESIAN_POINT('Ctrl Pts',(-7.88821051706799E-14,114.181249999554,
-10.5687124469213));
#297972=CARTESIAN_POINT('Ctrl Pts',(-3.10606665601019,114.331249999553,
-9.5594902125713));
#297973=CARTESIAN_POINT('Ctrl Pts',(-6.2121333120203,114.481249999553,-8.55026797822134));
#297974=CARTESIAN_POINT('Ctrl Pts',(-8.13178807675727,114.631249999552,
-5.90808986649102));
#297975=CARTESIAN_POINT('Ctrl Pts',(-10.0514428414942,114.781249999551,
-3.2659117547607));
#297976=CARTESIAN_POINT('Ctrl Pts',(-10.0514428414942,114.931249999551,
2.46189346052968E-15));
#297977=CARTESIAN_POINT('Ctrl Pts',(-10.0514428414942,115.08124999955,3.26591175476071));
#297978=CARTESIAN_POINT('Ctrl Pts',(-8.13178807675727,115.23124999955,5.90808986649102));
#297979=CARTESIAN_POINT('Ctrl Pts',(-6.21213331202029,115.381249999549,
8.55026797822134));
#297980=CARTESIAN_POINT('Ctrl Pts',(-3.10606665601018,115.531249999548,
9.5594902125713));
#297981=CARTESIAN_POINT('Ctrl Pts',(-7.71573718326647E-14,115.681249999548,
10.5687124469213));
#297982=CARTESIAN_POINT('Ctrl Pts',(3.10606665601003,115.831249999547,9.5594902125713));
#297983=CARTESIAN_POINT('Ctrl Pts',(6.21213331202014,115.981249999547,8.55026797822134));
#297984=CARTESIAN_POINT('Ctrl Pts',(8.13178807675711,116.131249999546,5.90808986649102));
#297985=CARTESIAN_POINT('Ctrl Pts',(10.0514428414941,116.281249999545,3.2659117547607));
#297986=CARTESIAN_POINT('Ctrl Pts',(10.0514428414941,116.431249999545,-1.23094673026484E-15));
#297987=CARTESIAN_POINT('Ctrl Pts',(10.0514428414941,116.581249999544,-3.26591175476071));
#297988=CARTESIAN_POINT('Ctrl Pts',(8.13178807675711,116.731249999544,-5.90808986649102));
#297989=CARTESIAN_POINT('Ctrl Pts',(6.21213331202014,116.881249999543,-8.55026797822134));
#297990=CARTESIAN_POINT('Ctrl Pts',(3.10606665601003,117.031249999542,-9.5594902125713));
#297991=CARTESIAN_POINT('Ctrl Pts',(-8.06098144423418E-14,117.181249999542,
-10.5687124469213));
#297992=CARTESIAN_POINT('Ctrl Pts',(-3.10606665601019,117.331249999541,
-9.5594902125713));
#297993=CARTESIAN_POINT('Ctrl Pts',(-6.2121333120203,117.481249999541,-8.55026797822134));
#297994=CARTESIAN_POINT('Ctrl Pts',(-8.13178807675727,117.63124999954,-5.90808986649102));
#297995=CARTESIAN_POINT('Ctrl Pts',(-10.0514428414942,117.781249999539,
-3.2659117547607));
#297996=CARTESIAN_POINT('Ctrl Pts',(-10.0514428414942,117.931249999539,
2.46189346052968E-15));
#297997=CARTESIAN_POINT('Ctrl Pts',(-10.0514428414942,118.081249999538,
3.26591175476071));
#297998=CARTESIAN_POINT('Ctrl Pts',(-8.13178807675727,118.231249999538,
5.90808986649102));
#297999=CARTESIAN_POINT('Ctrl Pts',(-6.2121333120203,118.381249999537,8.55026797822134));
#298000=CARTESIAN_POINT('Ctrl Pts',(-3.10606665601019,118.531249999536,
9.5594902125713));
#298001=CARTESIAN_POINT('Ctrl Pts',(-7.88850811043265E-14,118.681249999536,
10.5687124469213));
#298002=CARTESIAN_POINT('Ctrl Pts',(3.10606665601003,118.831249999535,9.5594902125713));
#298003=CARTESIAN_POINT('Ctrl Pts',(6.21213331202014,118.981249999535,8.55026797822134));
#298004=CARTESIAN_POINT('Ctrl Pts',(8.13178807675711,119.131249999534,5.90808986649102));
#298005=CARTESIAN_POINT('Ctrl Pts',(10.0514428414941,119.281249999533,3.2659117547607));
#298006=CARTESIAN_POINT('Ctrl Pts',(10.0514428414941,119.431249999533,-1.23094673026484E-15));
#298007=CARTESIAN_POINT('Ctrl Pts',(10.0514428414941,119.581249999532,-3.26591175476071));
#298008=CARTESIAN_POINT('Ctrl Pts',(8.13178807675711,119.731249999532,-5.90808986649102));
#298009=CARTESIAN_POINT('Ctrl Pts',(6.21213331202013,119.881249999531,-8.55026797822134));
#298010=CARTESIAN_POINT('Ctrl Pts',(3.10606665601003,120.03124999953,-9.5594902125713));
#298011=CARTESIAN_POINT('Ctrl Pts',(-8.23375237140036E-14,120.18124999953,
-10.5687124469213));
#298012=CARTESIAN_POINT('Ctrl Pts',(-3.10606665601019,120.331249999529,
-9.5594902125713));
#298013=CARTESIAN_POINT('Ctrl Pts',(-6.2121333120203,120.481249999529,-8.55026797822134));
#298014=CARTESIAN_POINT('Ctrl Pts',(-8.13178807675727,120.631249999528,
-5.90808986649102));
#298015=CARTESIAN_POINT('Ctrl Pts',(-10.0514428414943,120.781249999527,
-3.2659117547607));
#298016=CARTESIAN_POINT('Ctrl Pts',(-10.0514428414943,120.931249999527,
2.46189346052968E-15));
#298017=CARTESIAN_POINT('Ctrl Pts',(-10.0514428414943,121.081249999526,
3.26591175476071));
#298018=CARTESIAN_POINT('Ctrl Pts',(-8.13178807675727,121.231249999526,
5.90808986649102));
#298019=CARTESIAN_POINT('Ctrl Pts',(-6.2121333120203,121.381249999525,8.55026797822134));
#298020=CARTESIAN_POINT('Ctrl Pts',(-3.10606665601019,121.531249999524,
9.5594902125713));
#298021=CARTESIAN_POINT('Ctrl Pts',(-8.06127903759884E-14,121.681249999524,
10.5687124469213));
#298022=CARTESIAN_POINT('Ctrl Pts',(3.10606665601003,121.831249999523,9.5594902125713));
#298023=CARTESIAN_POINT('Ctrl Pts',(6.21213331202014,121.981249999523,8.55026797822134));
#298024=CARTESIAN_POINT('Ctrl Pts',(8.13178807675711,122.131249999522,5.90808986649102));
#298025=CARTESIAN_POINT('Ctrl Pts',(10.0514428414941,122.281249999521,3.2659117547607));
#298026=CARTESIAN_POINT('Ctrl Pts',(10.0514428414941,122.431249999521,-1.23094673026484E-15));
#298027=CARTESIAN_POINT('Ctrl Pts',(10.0514428414941,122.58124999952,-3.26591175476071));
#298028=CARTESIAN_POINT('Ctrl Pts',(8.13178807675711,122.73124999952,-5.90808986649102));
#298029=CARTESIAN_POINT('Ctrl Pts',(6.21213331202013,122.881249999519,-8.55026797822134));
#298030=CARTESIAN_POINT('Ctrl Pts',(3.10606665601002,123.031249999518,-9.5594902125713));
#298031=CARTESIAN_POINT('Ctrl Pts',(-8.40652329856655E-14,123.181249999518,
-10.5687124469213));
#298032=CARTESIAN_POINT('Ctrl Pts',(-3.10606665601019,123.331249999517,
-9.5594902125713));
#298033=CARTESIAN_POINT('Ctrl Pts',(-6.2121333120203,123.481249999517,-8.55026797822134));
#298034=CARTESIAN_POINT('Ctrl Pts',(-8.13178807675727,123.631249999516,
-5.90808986649102));
#298035=CARTESIAN_POINT('Ctrl Pts',(-10.0514428414943,123.781249999515,
-3.2659117547607));
#298036=CARTESIAN_POINT('Ctrl Pts',(-10.0514428414943,123.931249999515,
2.46189346052968E-15));
#298037=CARTESIAN_POINT('Ctrl Pts',(-10.0514428414943,124.081249999514,
3.26591175476071));
#298038=CARTESIAN_POINT('Ctrl Pts',(-8.13178807675727,124.231249999514,
5.90808986649102));
#298039=CARTESIAN_POINT('Ctrl Pts',(-6.2121333120203,124.381249999513,8.55026797822134));
#298040=CARTESIAN_POINT('Ctrl Pts',(-3.10606665601019,124.531249999512,
9.5594902125713));
#298041=CARTESIAN_POINT('Ctrl Pts',(-8.23404996476502E-14,124.681249999512,
10.5687124469213));
#298042=CARTESIAN_POINT('Ctrl Pts',(3.10606665601002,124.831249999511,9.5594902125713));
#298043=CARTESIAN_POINT('Ctrl Pts',(6.21213331202013,124.981249999511,8.55026797822134));
#298044=CARTESIAN_POINT('Ctrl Pts',(8.13178807675711,125.13124999951,5.90808986649102));
#298045=CARTESIAN_POINT('Ctrl Pts',(10.0514428414941,125.281249999509,3.2659117547607));
#298046=CARTESIAN_POINT('Ctrl Pts',(10.0514428414941,125.431249999509,-1.23094673026484E-15));
#298047=CARTESIAN_POINT('Ctrl Pts',(10.0514428414941,125.581249999508,-3.26591175476071));
#298048=CARTESIAN_POINT('Ctrl Pts',(8.13178807675711,125.731249999508,-5.90808986649102));
#298049=CARTESIAN_POINT('Ctrl Pts',(6.21213331202013,125.881249999507,-8.55026797822134));
#298050=CARTESIAN_POINT('Ctrl Pts',(3.10606665601002,126.031249999506,-9.5594902125713));
#298051=CARTESIAN_POINT('Ctrl Pts',(-8.57929422573273E-14,126.181249999506,
-10.5687124469213));
#298052=CARTESIAN_POINT('Ctrl Pts',(-3.10606665601019,126.331249999505,
-9.5594902125713));
#298053=CARTESIAN_POINT('Ctrl Pts',(-6.2121333120203,126.481249999505,-8.55026797822134));
#298054=CARTESIAN_POINT('Ctrl Pts',(-8.13178807675728,126.631249999504,
-5.90808986649102));
#298055=CARTESIAN_POINT('Ctrl Pts',(-10.0514428414943,126.781249999503,
-3.2659117547607));
#298056=CARTESIAN_POINT('Ctrl Pts',(-10.0514428414943,126.931249999503,
2.46189346052968E-15));
#298057=CARTESIAN_POINT('Ctrl Pts',(-10.0514428414943,127.081249999502,
3.26591175476071));
#298058=CARTESIAN_POINT('Ctrl Pts',(-8.13178807675728,127.231249999502,
5.90808986649102));
#298059=CARTESIAN_POINT('Ctrl Pts',(-6.2121333120203,127.381249999501,8.55026797822134));
#298060=CARTESIAN_POINT('Ctrl Pts',(-3.10606665601019,127.5312499995,9.5594902125713));
#298061=CARTESIAN_POINT('Ctrl Pts',(-8.4068208919312E-14,127.6812499995,
10.5687124469213));
#298062=CARTESIAN_POINT('Ctrl Pts',(3.10606665601002,127.831249999499,9.5594902125713));
#298063=CARTESIAN_POINT('Ctrl Pts',(6.21213331202013,127.981249999499,8.55026797822134));
#298064=CARTESIAN_POINT('Ctrl Pts',(8.1317880767571,128.131249999498,5.90808986649102));
#298065=CARTESIAN_POINT('Ctrl Pts',(10.0514428414941,128.281249999497,3.2659117547607));
#298066=CARTESIAN_POINT('Ctrl Pts',(10.0514428414941,128.431249999497,-1.23094673026484E-15));
#298067=CARTESIAN_POINT('Ctrl Pts',(10.0514428414941,128.581249999496,-3.26591175476071));
#298068=CARTESIAN_POINT('Ctrl Pts',(8.1317880767571,128.731249999496,-5.90808986649102));
#298069=CARTESIAN_POINT('Ctrl Pts',(6.21213331202013,128.881249999495,-8.55026797822134));
#298070=CARTESIAN_POINT('Ctrl Pts',(3.10606665601002,129.031249999494,-9.5594902125713));
#298071=CARTESIAN_POINT('Ctrl Pts',(-8.75206515289892E-14,129.181249999494,
-10.5687124469213));
#298072=CARTESIAN_POINT('Ctrl Pts',(-3.1060666560102,129.331249999493,-9.5594902125713));
#298073=CARTESIAN_POINT('Ctrl Pts',(-6.2121333120203,129.481249999493,-8.55026797822134));
#298074=CARTESIAN_POINT('Ctrl Pts',(-8.13178807675728,129.631249999492,
-5.90808986649102));
#298075=CARTESIAN_POINT('Ctrl Pts',(-10.0514428414943,129.781249999491,
-3.2659117547607));
#298076=CARTESIAN_POINT('Ctrl Pts',(-10.0514428414943,129.931249999491,
2.46189346052968E-15));
#298077=CARTESIAN_POINT('Ctrl Pts',(-10.0514428414943,130.08124999949,3.26591175476071));
#298078=CARTESIAN_POINT('Ctrl Pts',(-8.13178807675728,130.23124999949,5.90808986649102));
#298079=CARTESIAN_POINT('Ctrl Pts',(-6.2121333120203,130.381249999489,8.55026797822134));
#298080=CARTESIAN_POINT('Ctrl Pts',(-3.10606665601019,130.531249999488,
9.5594902125713));
#298081=CARTESIAN_POINT('Ctrl Pts',(-8.57959181909739E-14,130.681249999488,
10.5687124469213));
#298082=CARTESIAN_POINT('Ctrl Pts',(3.10606665601002,130.831249999487,9.5594902125713));
#298083=CARTESIAN_POINT('Ctrl Pts',(6.21213331202013,130.981249999487,8.55026797822134));
#298084=CARTESIAN_POINT('Ctrl Pts',(8.1317880767571,131.131249999486,5.90808986649102));
#298085=CARTESIAN_POINT('Ctrl Pts',(10.0514428414941,131.281249999485,3.2659117547607));
#298086=CARTESIAN_POINT('Ctrl Pts',(10.0514428414941,131.431249999485,-1.23094673026484E-15));
#298087=CARTESIAN_POINT('Ctrl Pts',(10.0514428414941,131.581249999484,-3.26591175476071));
#298088=CARTESIAN_POINT('Ctrl Pts',(8.1317880767571,131.731249999484,-5.90808986649102));
#298089=CARTESIAN_POINT('Ctrl Pts',(6.21213331202012,131.881249999483,-8.55026797822134));
#298090=CARTESIAN_POINT('Ctrl Pts',(3.10606665601002,132.031249999482,-9.5594902125713));
#298091=CARTESIAN_POINT('Ctrl Pts',(-8.9248360800651E-14,132.181249999482,
-10.5687124469213));
#298092=CARTESIAN_POINT('Ctrl Pts',(-3.1060666560102,132.331249999481,-9.5594902125713));
#298093=CARTESIAN_POINT('Ctrl Pts',(-6.2121333120203,132.48124999948,-8.55026797822134));
#298094=CARTESIAN_POINT('Ctrl Pts',(-8.13178807675728,132.63124999948,-5.90808986649102));
#298095=CARTESIAN_POINT('Ctrl Pts',(-10.0514428414943,132.781249999479,
-3.2659117547607));
#298096=CARTESIAN_POINT('Ctrl Pts',(-10.0514428414943,132.931249999479,
2.46189346052968E-15));
#298097=CARTESIAN_POINT('Ctrl Pts',(-10.0514428414943,133.081249999478,
3.26591175476071));
#298098=CARTESIAN_POINT('Ctrl Pts',(-8.13178807675728,133.231249999478,
5.90808986649102));
#298099=CARTESIAN_POINT('Ctrl Pts',(-6.2121333120203,133.381249999477,8.55026797822134));
#298100=CARTESIAN_POINT('Ctrl Pts',(-3.1060666560102,133.531249999476,9.5594902125713));
#298101=CARTESIAN_POINT('Ctrl Pts',(-8.75236274626357E-14,133.681249999476,
10.5687124469213));
#298102=CARTESIAN_POINT('Ctrl Pts',(3.10606665601002,133.831249999475,9.5594902125713));
#298103=CARTESIAN_POINT('Ctrl Pts',(6.21213331202013,133.981249999475,8.55026797822134));
#298104=CARTESIAN_POINT('Ctrl Pts',(8.1317880767571,134.131249999474,5.90808986649102));
#298105=CARTESIAN_POINT('Ctrl Pts',(10.0514428414941,134.281249999473,3.2659117547607));
#298106=CARTESIAN_POINT('Ctrl Pts',(10.0514428414941,134.431249999473,-1.23094673026484E-15));
#298107=CARTESIAN_POINT('Ctrl Pts',(10.0514428414941,134.581249999472,-3.26591175476071));
#298108=CARTESIAN_POINT('Ctrl Pts',(8.1317880767571,134.731249999472,-5.90808986649102));
#298109=CARTESIAN_POINT('Ctrl Pts',(6.21213331202012,134.881249999471,-8.55026797822134));
#298110=CARTESIAN_POINT('Ctrl Pts',(3.10606665601002,135.03124999947,-9.5594902125713));
#298111=CARTESIAN_POINT('Ctrl Pts',(-9.09760700723128E-14,135.18124999947,
-10.5687124469213));
#298112=CARTESIAN_POINT('Ctrl Pts',(-3.1060666560102,135.331249999469,-9.5594902125713));
#298113=CARTESIAN_POINT('Ctrl Pts',(-6.21213331202031,135.481249999469,
-8.55026797822134));
#298114=CARTESIAN_POINT('Ctrl Pts',(-8.13178807675728,135.631249999468,
-5.90808986649102));
#298115=CARTESIAN_POINT('Ctrl Pts',(-10.0514428414943,135.781249999467,
-3.2659117547607));
#298116=CARTESIAN_POINT('Ctrl Pts',(-10.0514428414943,135.931249999467,
2.46189346052968E-15));
#298117=CARTESIAN_POINT('Ctrl Pts',(-10.0514428414943,136.081249999466,
3.26591175476071));
#298118=CARTESIAN_POINT('Ctrl Pts',(-8.13178807675728,136.231249999466,
5.90808986649102));
#298119=CARTESIAN_POINT('Ctrl Pts',(-6.2121333120203,136.381249999465,8.55026797822134));
#298120=CARTESIAN_POINT('Ctrl Pts',(-3.1060666560102,136.531249999464,9.5594902125713));
#298121=CARTESIAN_POINT('Ctrl Pts',(-8.92513367342975E-14,136.681249999464,
10.5687124469213));
#298122=CARTESIAN_POINT('Ctrl Pts',(3.10606665601002,136.831249999463,9.5594902125713));
#298123=CARTESIAN_POINT('Ctrl Pts',(6.21213331202012,136.981249999463,8.55026797822134));
#298124=CARTESIAN_POINT('Ctrl Pts',(8.1317880767571,137.131249999462,5.90808986649102));
#298125=CARTESIAN_POINT('Ctrl Pts',(10.0514428414941,137.281249999461,3.2659117547607));
#298126=CARTESIAN_POINT('Ctrl Pts',(10.0514428414941,137.431249999461,-1.23094673026484E-15));
#298127=CARTESIAN_POINT('Ctrl Pts',(10.0514428414941,137.58124999946,-3.26591175476071));
#298128=CARTESIAN_POINT('Ctrl Pts',(8.1317880767571,137.73124999946,-5.90808986649102));
#298129=CARTESIAN_POINT('Ctrl Pts',(6.21213331202012,137.881249999459,-8.55026797822134));
#298130=CARTESIAN_POINT('Ctrl Pts',(3.10606665601002,138.031249999458,-9.5594902125713));
#298131=CARTESIAN_POINT('Ctrl Pts',(-9.27037793439746E-14,138.181249999458,
-10.5687124469213));
#298132=CARTESIAN_POINT('Ctrl Pts',(-3.1060666560102,138.331249999457,-9.5594902125713));
#298133=CARTESIAN_POINT('Ctrl Pts',(-6.21213331202031,138.481249999456,
-8.55026797822134));
#298134=CARTESIAN_POINT('Ctrl Pts',(-8.13178807675728,138.631249999456,
-5.90808986649102));
#298135=CARTESIAN_POINT('Ctrl Pts',(-10.0514428414943,138.781249999455,
-3.2659117547607));
#298136=CARTESIAN_POINT('Ctrl Pts',(-10.0514428414943,138.931249999455,
2.46189346052968E-15));
#298137=CARTESIAN_POINT('Ctrl Pts',(-10.0514428414943,139.081249999454,
3.26591175476071));
#298138=CARTESIAN_POINT('Ctrl Pts',(-8.13178807675728,139.231249999454,
5.90808986649102));
#298139=CARTESIAN_POINT('Ctrl Pts',(-6.21213331202031,139.381249999453,
8.55026797822134));
#298140=CARTESIAN_POINT('Ctrl Pts',(-3.1060666560102,139.531249999452,9.5594902125713));
#298141=CARTESIAN_POINT('Ctrl Pts',(-9.09790460059594E-14,139.681249999452,
10.5687124469213));
#298142=CARTESIAN_POINT('Ctrl Pts',(3.10606665601002,139.831249999451,9.5594902125713));
#298143=CARTESIAN_POINT('Ctrl Pts',(6.21213331202012,139.981249999451,8.55026797822134));
#298144=CARTESIAN_POINT('Ctrl Pts',(8.1317880767571,140.13124999945,5.90808986649102));
#298145=CARTESIAN_POINT('Ctrl Pts',(10.0514428414941,140.281249999449,3.2659117547607));
#298146=CARTESIAN_POINT('Ctrl Pts',(10.0514428414941,140.431249999449,-1.23094673026484E-15));
#298147=CARTESIAN_POINT('Ctrl Pts',(10.0514428414941,140.581249999448,-3.26591175476071));
#298148=CARTESIAN_POINT('Ctrl Pts',(8.1317880767571,140.731249999448,-5.90808986649102));
#298149=CARTESIAN_POINT('Ctrl Pts',(6.21213331202012,140.881249999447,-8.55026797822134));
#298150=CARTESIAN_POINT('Ctrl Pts',(3.10606665601001,141.031249999446,-9.5594902125713));
#298151=CARTESIAN_POINT('Ctrl Pts',(-9.44314886156365E-14,141.181249999446,
-10.5687124469213));
#298152=CARTESIAN_POINT('Ctrl Pts',(-3.1060666560102,141.331249999445,-9.5594902125713));
#298153=CARTESIAN_POINT('Ctrl Pts',(-6.21213331202031,141.481249999445,
-8.55026797822134));
#298154=CARTESIAN_POINT('Ctrl Pts',(-8.13178807675729,141.631249999444,
-5.90808986649102));
#298155=CARTESIAN_POINT('Ctrl Pts',(-10.0514428414943,141.781249999443,
-3.2659117547607));
#298156=CARTESIAN_POINT('Ctrl Pts',(-10.0514428414943,141.931249999443,
2.46189346052968E-15));
#298157=CARTESIAN_POINT('Ctrl Pts',(-10.0514428414943,142.081249999442,
3.26591175476071));
#298158=CARTESIAN_POINT('Ctrl Pts',(-8.13178807675729,142.231249999442,
5.90808986649102));
#298159=CARTESIAN_POINT('Ctrl Pts',(-6.21213331202031,142.381249999441,
8.55026797822134));
#298160=CARTESIAN_POINT('Ctrl Pts',(-3.1060666560102,142.53124999944,9.5594902125713));
#298161=CARTESIAN_POINT('Ctrl Pts',(-9.27067552776212E-14,142.68124999944,
10.5687124469213));
#298162=CARTESIAN_POINT('Ctrl Pts',(3.10606665601001,142.831249999439,9.5594902125713));
#298163=CARTESIAN_POINT('Ctrl Pts',(6.21213331202012,142.981249999439,8.55026797822134));
#298164=CARTESIAN_POINT('Ctrl Pts',(8.1317880767571,143.131249999438,5.90808986649102));
#298165=CARTESIAN_POINT('Ctrl Pts',(10.0514428414941,143.281249999437,3.2659117547607));
#298166=CARTESIAN_POINT('Ctrl Pts',(10.0514428414941,143.431249999437,-1.23094673026484E-15));
#298167=CARTESIAN_POINT('Ctrl Pts',(10.0514428414941,143.581249999436,-3.26591175476071));
#298168=CARTESIAN_POINT('Ctrl Pts',(8.1317880767571,143.731249999436,-5.90808986649102));
#298169=CARTESIAN_POINT('Ctrl Pts',(6.21213331202012,143.881249999435,-8.55026797822134));
#298170=CARTESIAN_POINT('Ctrl Pts',(3.10606665601001,144.031249999434,-9.5594902125713));
#298171=CARTESIAN_POINT('Ctrl Pts',(-9.61591978872984E-14,144.181249999434,
-10.5687124469213));
#298172=CARTESIAN_POINT('Ctrl Pts',(-3.1060666560102,144.331249999433,-9.5594902125713));
#298173=CARTESIAN_POINT('Ctrl Pts',(-6.21213331202031,144.481249999432,
-8.55026797822134));
#298174=CARTESIAN_POINT('Ctrl Pts',(-8.13178807675729,144.631249999432,
-5.90808986649102));
#298175=CARTESIAN_POINT('Ctrl Pts',(-10.0514428414943,144.781249999431,
-3.2659117547607));
#298176=CARTESIAN_POINT('Ctrl Pts',(-10.0514428414943,144.931249999431,
2.46189346052968E-15));
#298177=CARTESIAN_POINT('Ctrl Pts',(-10.0514428414943,145.08124999943,3.26591175476071));
#298178=CARTESIAN_POINT('Ctrl Pts',(-8.13178807675729,145.23124999943,5.90808986649102));
#298179=CARTESIAN_POINT('Ctrl Pts',(-6.21213331202031,145.381249999429,
8.55026797822134));
#298180=CARTESIAN_POINT('Ctrl Pts',(-3.1060666560102,145.531249999428,9.5594902125713));
#298181=CARTESIAN_POINT('Ctrl Pts',(-9.44344645492831E-14,145.681249999428,
10.5687124469213));
#298182=CARTESIAN_POINT('Ctrl Pts',(3.10606665601001,145.831249999427,9.5594902125713));
#298183=CARTESIAN_POINT('Ctrl Pts',(6.21213331202012,145.981249999427,8.55026797822134));
#298184=CARTESIAN_POINT('Ctrl Pts',(8.13178807675709,146.131249999426,5.90808986649102));
#298185=CARTESIAN_POINT('Ctrl Pts',(10.0514428414941,146.281249999425,3.2659117547607));
#298186=CARTESIAN_POINT('Ctrl Pts',(10.0514428414941,146.431249999425,-1.23094673026484E-15));
#298187=CARTESIAN_POINT('Ctrl Pts',(10.0514428414941,146.581249999424,-3.26591175476071));
#298188=CARTESIAN_POINT('Ctrl Pts',(8.13178807675709,146.731249999424,-5.90808986649102));
#298189=CARTESIAN_POINT('Ctrl Pts',(6.21213331202012,146.881249999423,-8.55026797822134));
#298190=CARTESIAN_POINT('Ctrl Pts',(3.10606665601001,147.031249999422,-9.5594902125713));
#298191=CARTESIAN_POINT('Ctrl Pts',(-9.78869071589602E-14,147.181249999422,
-10.5687124469213));
#298192=CARTESIAN_POINT('Ctrl Pts',(-3.10606665601021,147.331249999421,
-9.5594902125713));
#298193=CARTESIAN_POINT('Ctrl Pts',(-6.21213331202032,147.481249999421,
-8.55026797822134));
#298194=CARTESIAN_POINT('Ctrl Pts',(-8.13178807675729,147.63124999942,-5.90808986649102));
#298195=CARTESIAN_POINT('Ctrl Pts',(-10.0514428414943,147.781249999419,
-3.2659117547607));
#298196=CARTESIAN_POINT('Ctrl Pts',(-10.0514428414943,147.931249999419,
2.46189346052968E-15));
#298197=CARTESIAN_POINT('Ctrl Pts',(-10.0514428414943,148.081249999418,
3.26591175476071));
#298198=CARTESIAN_POINT('Ctrl Pts',(-8.13178807675729,148.231249999418,
5.90808986649102));
#298199=CARTESIAN_POINT('Ctrl Pts',(-6.21213331202031,148.381249999417,
8.55026797822134));
#298200=CARTESIAN_POINT('Ctrl Pts',(-3.1060666560102,148.531249999416,9.5594902125713));
#298201=CARTESIAN_POINT('Ctrl Pts',(-9.61621738209449E-14,148.681249999416,
10.5687124469213));
#298202=CARTESIAN_POINT('Ctrl Pts',(3.10606665601001,148.831249999415,9.5594902125713));
#298203=CARTESIAN_POINT('Ctrl Pts',(6.21213331202012,148.981249999415,8.55026797822134));
#298204=CARTESIAN_POINT('Ctrl Pts',(8.13178807675709,149.131249999414,5.90808986649102));
#298205=CARTESIAN_POINT('Ctrl Pts',(10.0514428414941,149.281249999413,3.2659117547607));
#298206=CARTESIAN_POINT('Ctrl Pts',(10.0514428414941,149.431249999413,-1.23094673026484E-15));
#298207=CARTESIAN_POINT('Ctrl Pts',(10.0514428414941,149.581249999412,-3.26591175476071));
#298208=CARTESIAN_POINT('Ctrl Pts',(8.13178807675709,149.731249999412,-5.90808986649102));
#298209=CARTESIAN_POINT('Ctrl Pts',(6.21213331202012,149.881249999411,-8.55026797822134));
#298210=CARTESIAN_POINT('Ctrl Pts',(3.10606665601001,150.03124999941,-9.5594902125713));
#298211=CARTESIAN_POINT('Ctrl Pts',(-9.9614616430622E-14,150.18124999941,
-10.5687124469213));
#298212=CARTESIAN_POINT('Ctrl Pts',(-3.10606665601021,150.331249999409,
-9.5594902125713));
#298213=CARTESIAN_POINT('Ctrl Pts',(-6.21213331202032,150.481249999409,
-8.55026797822134));
#298214=CARTESIAN_POINT('Ctrl Pts',(-8.13178807675729,150.631249999408,
-5.90808986649102));
#298215=CARTESIAN_POINT('Ctrl Pts',(-10.0514428414943,150.781249999407,
-3.2659117547607));
#298216=CARTESIAN_POINT('Ctrl Pts',(-10.0514428414943,150.931249999407,
2.46189346052968E-15));
#298217=CARTESIAN_POINT('Ctrl Pts',(-10.0514428414943,151.081249999406,
3.26591175476071));
#298218=CARTESIAN_POINT('Ctrl Pts',(-8.13178807675729,151.231249999406,
5.90808986649102));
#298219=CARTESIAN_POINT('Ctrl Pts',(-6.21213331202032,151.381249999405,
8.55026797822134));
#298220=CARTESIAN_POINT('Ctrl Pts',(-3.10606665601021,151.531249999404,
9.5594902125713));
#298221=CARTESIAN_POINT('Ctrl Pts',(-9.78898830926068E-14,151.681249999404,
10.5687124469213));
#298222=CARTESIAN_POINT('Ctrl Pts',(3.10606665601001,151.831249999403,9.5594902125713));
#298223=CARTESIAN_POINT('Ctrl Pts',(6.21213331202012,151.981249999403,8.55026797822134));
#298224=CARTESIAN_POINT('Ctrl Pts',(8.13178807675709,152.131249999402,5.90808986649102));
#298225=CARTESIAN_POINT('Ctrl Pts',(10.0514428414941,152.281249999401,3.2659117547607));
#298226=CARTESIAN_POINT('Ctrl Pts',(10.0514428414941,152.431249999401,-1.23094673026484E-15));
#298227=CARTESIAN_POINT('Ctrl Pts',(10.0514428414941,152.5812499994,-3.26591175476071));
#298228=CARTESIAN_POINT('Ctrl Pts',(8.13178807675709,152.7312499994,-5.90808986649102));
#298229=CARTESIAN_POINT('Ctrl Pts',(6.21213331202012,152.881249999399,-8.55026797822134));
#298230=CARTESIAN_POINT('Ctrl Pts',(3.10606665601001,153.031249999398,-9.5594902125713));
#298231=CARTESIAN_POINT('Ctrl Pts',(-1.01342325702284E-13,153.181249999398,
-10.5687124469213));
#298232=CARTESIAN_POINT('Ctrl Pts',(-3.10606665601021,153.331249999397,
-9.5594902125713));
#298233=CARTESIAN_POINT('Ctrl Pts',(11.6184932898974,91.186,3.00176842421395));
#298234=CARTESIAN_POINT('Ctrl Pts',(11.2700427515582,91.186,4.04399430707808));
#298235=CARTESIAN_POINT('Ctrl Pts',(10.7791667820617,91.185999999732,5.03296359596024));
#298236=CARTESIAN_POINT('Ctrl Pts',(9.52052428043545,91.185999999732,6.8774807324221));
#298237=CARTESIAN_POINT('Ctrl Pts',(8.77953392736288,91.185999997219,7.68371450615621));
#298238=CARTESIAN_POINT('Ctrl Pts',(7.39526332234894,91.185999997219,8.81855324040878));
#298239=CARTESIAN_POINT('Ctrl Pts',(6.81132012907742,91.186,9.21313481182541));
#298240=CARTESIAN_POINT('Ctrl Pts',(5.05918236890942,91.186,10.1743250327452));
#298241=CARTESIAN_POINT('Ctrl Pts',(3.67332182531712,91.186,10.6827925701586));
#298242=CARTESIAN_POINT('Ctrl Pts',(0.735795623987487,91.186,11.0280650073144));
#298243=CARTESIAN_POINT('Ctrl Pts',(-0.652494305311852,91.186,10.9270735304368));
#298244=CARTESIAN_POINT('Ctrl Pts',(-2.97093150664768,91.186,10.3045254405431));
#298245=CARTESIAN_POINT('Ctrl Pts',(-4.34343559193747,91.1860000000001,
9.79240651982437));
#298246=CARTESIAN_POINT('Ctrl Pts',(-6.33964933794428,91.1860000000001,
8.2393064142999));
#298247=CARTESIAN_POINT('Ctrl Pts',(-6.89998590554459,91.186,7.69134457042996));
#298248=CARTESIAN_POINT('Ctrl Pts',(-7.82072333918513,91.186,6.5609072669913));
#298249=CARTESIAN_POINT('Ctrl Pts',(-8.27453946661952,91.186,5.90162129296699));
#298250=CARTESIAN_POINT('Ctrl Pts',(-8.66397270809382,91.186,5.09579043026947));
#298251=CARTESIAN_POINT('Ctrl Pts',(10.0514428414941,128.431249999497,-1.23094673026484E-15));
#298252=CARTESIAN_POINT('Ctrl Pts',(10.0514428414941,128.581249999496,-3.26591175476071));
#298253=CARTESIAN_POINT('Ctrl Pts',(8.1317880767571,128.731249999496,-5.90808986649102));
#298254=CARTESIAN_POINT('Ctrl Pts',(6.21213331202013,128.881249999495,-8.55026797822134));
#298255=CARTESIAN_POINT('Ctrl Pts',(3.10606665601002,129.031249999494,-9.5594902125713));
#298256=CARTESIAN_POINT('Ctrl Pts',(-8.75206515289892E-14,129.181249999494,
-10.5687124469213));
#298257=CARTESIAN_POINT('Ctrl Pts',(-3.1060666560102,129.331249999493,-9.5594902125713));
#298258=CARTESIAN_POINT('Ctrl Pts',(-6.2121333120203,129.481249999493,-8.55026797822134));
#298259=CARTESIAN_POINT('Ctrl Pts',(-8.13178807675728,129.631249999492,
-5.90808986649102));
#298260=CARTESIAN_POINT('Ctrl Pts',(-10.0514428414943,129.781249999491,
-3.2659117547607));
#298261=CARTESIAN_POINT('Ctrl Pts',(-10.0514428414943,129.931249999491,
2.46189346052968E-15));
#298262=CARTESIAN_POINT('Ctrl Pts',(-10.0514428414943,130.08124999949,3.26591175476071));
#298263=CARTESIAN_POINT('Ctrl Pts',(-8.13178807675728,130.23124999949,5.90808986649102));
#298264=CARTESIAN_POINT('Ctrl Pts',(-6.2121333120203,130.381249999489,8.55026797822134));
#298265=CARTESIAN_POINT('Ctrl Pts',(-3.10606665601019,130.531249999488,
9.5594902125713));
#298266=CARTESIAN_POINT('Ctrl Pts',(-0.158086395373697,130.673615598191,
10.5173470633579));
#298267=CARTESIAN_POINT('Ctrl Pts',(2.81735069959344,130.817307158506,9.64852518426128));
#298268=CARTESIAN_POINT('Origin',(-3.77475828372553E-14,-1.881249999982,
2.68644078414671E-15));
#298269=CARTESIAN_POINT('Origin',(-8.79029313101884E-14,130.96875,0.));
#298270=CARTESIAN_POINT('Origin',(0.,91.186,0.));
#298271=CARTESIAN_POINT('',(24.9999999999999,91.186,30.));
#298272=CARTESIAN_POINT('',(24.9999999999999,91.186,-30.));
#298273=CARTESIAN_POINT('',(24.9999999999999,91.186,30.));
#298274=CARTESIAN_POINT('',(-25.0000000000001,91.186,-30.));
#298275=CARTESIAN_POINT('',(-25.0000000000001,91.186,-30.));
#298276=CARTESIAN_POINT('',(-25.0000000000001,91.186,30.));
#298277=CARTESIAN_POINT('',(-25.0000000000001,91.186,30.));
#298278=CARTESIAN_POINT('',(-25.0000000000001,91.186,30.));
#298279=CARTESIAN_POINT('Origin',(0.,76.2,0.));
#298280=CARTESIAN_POINT('',(24.9999999999999,76.2,30.));
#298281=CARTESIAN_POINT('',(24.9999999999999,76.2,-30.));
#298282=CARTESIAN_POINT('',(24.9999999999999,76.2,30.));
#298283=CARTESIAN_POINT('',(-25.0000000000001,76.2,30.));
#298284=CARTESIAN_POINT('',(-25.0000000000001,76.2,30.));
#298285=CARTESIAN_POINT('',(-25.0000000000001,76.2,-30.));
#298286=CARTESIAN_POINT('',(-25.0000000000001,76.2,30.));
#298287=CARTESIAN_POINT('',(-25.0000000000001,76.2,-30.));
#298288=CARTESIAN_POINT('',(-15.58845726812,76.2,9.00000000000004));
#298289=CARTESIAN_POINT('',(-1.78703160926406E-13,76.2,18.));
#298290=CARTESIAN_POINT('Origin',(-1.78703160926406E-13,76.2,6.74376190435982E-14));
#298291=CARTESIAN_POINT('',(15.5884572681197,76.2,9.00000000000003));
#298292=CARTESIAN_POINT('Origin',(-1.78703160926406E-13,76.2,2.60289135494012E-29));
#298293=CARTESIAN_POINT('',(15.5884572681198,76.2,-9.00000000000011));
#298294=CARTESIAN_POINT('Origin',(-1.78703160926406E-13,76.2,6.74376190435982E-14));
#298295=CARTESIAN_POINT('',(-1.78703160926406E-13,76.2,-18.0000000000001));
#298296=CARTESIAN_POINT('Origin',(-1.78703160926406E-13,76.2,6.74376190435982E-14));
#298297=CARTESIAN_POINT('',(-15.5884572681201,76.2,-8.99999999999997));
#298298=CARTESIAN_POINT('Origin',(-1.78703160926406E-13,76.2,6.74376190435982E-14));
#298299=CARTESIAN_POINT('Origin',(-1.78703160926406E-13,76.2,6.74376190435982E-14));
#298300=CARTESIAN_POINT('Origin',(24.9999999999999,91.186,30.));
#298301=CARTESIAN_POINT('',(24.9999999999999,91.186,-30.));
#298302=CARTESIAN_POINT('',(24.9999999999999,91.186,30.));
#298303=CARTESIAN_POINT('Origin',(-25.0000000000001,91.186,-30.));
#298304=CARTESIAN_POINT('',(-25.0000000000001,91.186,-30.));
#298305=CARTESIAN_POINT('Origin',(-25.0000000000001,91.186,30.));
#298306=CARTESIAN_POINT('',(-25.0000000000001,91.186,30.));
#298307=CARTESIAN_POINT('Origin',(-25.0000000000001,91.186,30.));
#298308=CARTESIAN_POINT('Origin',(10.3923048454132,57.2,18.));
#298309=CARTESIAN_POINT('',(20.7846096908265,58.8076951545868,-8.45698818236971E-15));
#298310=CARTESIAN_POINT('',(20.7846096908265,74.5923048454133,-9.10794141489568E-15));
#298311=CARTESIAN_POINT('',(20.7846096908265,57.2,-9.10794141489568E-15));
#298312=CARTESIAN_POINT('Ctrl Pts',(20.7846096908597,74.5923048453941,-5.76297439360145E-11));
#298313=CARTESIAN_POINT('Ctrl Pts',(18.0000000000132,76.2,4.82308546373715));
#298314=CARTESIAN_POINT('Ctrl Pts',(15.5884572681197,76.2,9.00000000000019));
#298315=CARTESIAN_POINT('',(10.3923048454132,74.5923048454133,18.));
#298316=CARTESIAN_POINT('Ctrl Pts',(15.5884572681197,76.2,9.00000000000019));
#298317=CARTESIAN_POINT('Ctrl Pts',(13.1769145362263,76.2,13.1769145362631));
#298318=CARTESIAN_POINT('Ctrl Pts',(10.3923048453799,74.592304845394,18.0000000000577));
#298319=CARTESIAN_POINT('',(10.3923048454132,58.8076951545868,18.));
#298320=CARTESIAN_POINT('',(10.3923048454132,57.2,18.));
#298321=CARTESIAN_POINT('',(15.5884572681197,57.2,9.00000000000005));
#298322=CARTESIAN_POINT('Ctrl Pts',(15.5884572681198,57.2000000000001,9.00000000000012));
#298323=CARTESIAN_POINT('Ctrl Pts',(13.1769145362263,57.2000000000001,13.176914536263));
#298324=CARTESIAN_POINT('Ctrl Pts',(10.3923048453799,58.807695154606,18.0000000000576));
#298325=CARTESIAN_POINT('Ctrl Pts',(20.7846096908597,58.807695154606,-5.75819548439033E-11));
#298326=CARTESIAN_POINT('Ctrl Pts',(18.0000000000133,57.2000000000001,4.82308546373711));
#298327=CARTESIAN_POINT('Ctrl Pts',(15.5884572681198,57.2000000000001,9.0000000000001));
#298328=CARTESIAN_POINT('Origin',(-10.3923048454133,57.2,18.));
#298329=CARTESIAN_POINT('Ctrl Pts',(10.3923048454797,74.5923048453941,18.));
#298330=CARTESIAN_POINT('Ctrl Pts',(4.82308546378683,76.2,18.));
#298331=CARTESIAN_POINT('Ctrl Pts',(-1.71095103011815E-13,76.2,18.));
#298332=CARTESIAN_POINT('',(-10.3923048454133,74.5923048454133,18.));
#298333=CARTESIAN_POINT('Ctrl Pts',(-1.41221354866895E-13,76.2,18.));
#298334=CARTESIAN_POINT('Ctrl Pts',(-4.82308546378711,76.2,18.));
#298335=CARTESIAN_POINT('Ctrl Pts',(-10.39230484548,74.5923048453941,18.));
#298336=CARTESIAN_POINT('',(-10.3923048454133,58.8076951545867,18.));
#298337=CARTESIAN_POINT('',(-10.3923048454133,57.2,18.));
#298338=CARTESIAN_POINT('',(-1.37604970778725E-13,57.2,18.));
#298339=CARTESIAN_POINT('Ctrl Pts',(-1.34884499199791E-13,57.2,18.));
#298340=CARTESIAN_POINT('Ctrl Pts',(-4.82308546378705,57.2,18.));
#298341=CARTESIAN_POINT('Ctrl Pts',(-10.3923048454799,58.8076951546059,
18.));
#298342=CARTESIAN_POINT('Ctrl Pts',(10.3923048454797,58.807695154606,18.));
#298343=CARTESIAN_POINT('Ctrl Pts',(4.82308546378685,57.2,18.));
#298344=CARTESIAN_POINT('Ctrl Pts',(-1.27642378437386E-13,57.2,18.));
#298345=CARTESIAN_POINT('Origin',(-20.7846096908266,57.2,-3.51753081198983E-15));
#298346=CARTESIAN_POINT('Ctrl Pts',(-10.3923048453801,74.5923048453941,
18.0000000000576));
#298347=CARTESIAN_POINT('Ctrl Pts',(-13.1769145362265,76.2,13.1769145362629));
#298348=CARTESIAN_POINT('Ctrl Pts',(-15.58845726812,76.2,8.99999999999997));
#298349=CARTESIAN_POINT('',(-20.7846096908266,74.5923048454133,-3.06716835895631E-15));
#298350=CARTESIAN_POINT('Ctrl Pts',(-15.5884572681199,76.2000000000001,
9.00000000000014));
#298351=CARTESIAN_POINT('Ctrl Pts',(-18.0000000000134,76.2000000000001,
4.82308546373712));
#298352=CARTESIAN_POINT('Ctrl Pts',(-20.7846096908599,74.5923048453941,
-5.76355956615787E-11));
#298353=CARTESIAN_POINT('',(-20.7846096908266,58.8076951545866,-4.94143077032127E-15));
#298354=CARTESIAN_POINT('',(-20.7846096908266,57.2,-3.51753081198983E-15));
#298355=CARTESIAN_POINT('',(-15.58845726812,57.2,9.00000000000005));
#298356=CARTESIAN_POINT('Ctrl Pts',(-15.5884572681199,57.1999999999999,
9.00000000000004));
#298357=CARTESIAN_POINT('Ctrl Pts',(-18.0000000000134,57.1999999999999,
4.82308546373706));
#298358=CARTESIAN_POINT('Ctrl Pts',(-20.7846096908598,58.8076951546058,
-5.76404720995493E-11));
#298359=CARTESIAN_POINT('Ctrl Pts',(-10.39230484538,58.8076951546059,18.0000000000577));
#298360=CARTESIAN_POINT('Ctrl Pts',(-13.1769145362264,57.1999999999999,
13.176914536263));
#298361=CARTESIAN_POINT('Ctrl Pts',(-15.5884572681199,57.1999999999999,
9.00000000000004));
#298362=CARTESIAN_POINT('Origin',(-10.3923048454133,57.2,-18.));
#298363=CARTESIAN_POINT('Ctrl Pts',(-20.7846096908599,74.5923048453941,
5.76073123213497E-11));
#298364=CARTESIAN_POINT('Ctrl Pts',(-18.0000000000135,76.2,-4.823085463737));
#298365=CARTESIAN_POINT('Ctrl Pts',(-15.58845726812,76.2,-8.99999999999991));
#298366=CARTESIAN_POINT('',(-10.3923048454133,74.5923048454133,-18.));
#298367=CARTESIAN_POINT('Ctrl Pts',(-15.58845726812,76.2,-8.9999999999999));
#298368=CARTESIAN_POINT('Ctrl Pts',(-13.1769145362265,76.2000000000001,
-13.1769145362629));
#298369=CARTESIAN_POINT('Ctrl Pts',(-10.3923048453801,74.5923048453941,
-18.0000000000576));
#298370=CARTESIAN_POINT('',(-10.3923048454133,58.8076951545867,-18.));
#298371=CARTESIAN_POINT('',(-10.3923048454133,57.2,-18.));
#298372=CARTESIAN_POINT('',(-15.5884572681201,57.2,-8.99999999999995));
#298373=CARTESIAN_POINT('Ctrl Pts',(-15.58845726812,57.1999999999999,-8.99999999999989));
#298374=CARTESIAN_POINT('Ctrl Pts',(-13.1769145362265,57.1999999999999,
-13.1769145362629));
#298375=CARTESIAN_POINT('Ctrl Pts',(-10.39230484538,58.8076951546059,-18.0000000000576));
#298376=CARTESIAN_POINT('Ctrl Pts',(-20.7846096908598,58.8076951546058,
5.75917077198438E-11));
#298377=CARTESIAN_POINT('Ctrl Pts',(-18.0000000000135,57.1999999999999,
-4.82308546373701));
#298378=CARTESIAN_POINT('Ctrl Pts',(-15.58845726812,57.1999999999999,-8.99999999999989));
#298379=CARTESIAN_POINT('Origin',(10.3923048454132,57.2,-18.));
#298380=CARTESIAN_POINT('Ctrl Pts',(-10.3923048454799,74.5923048453941,
-18.));
#298381=CARTESIAN_POINT('Ctrl Pts',(-4.82308546378714,76.2,-18.));
#298382=CARTESIAN_POINT('Ctrl Pts',(-2.77011119161987E-13,76.2,-18.));
#298383=CARTESIAN_POINT('',(10.3923048454132,74.5923048454133,-18.));
#298384=CARTESIAN_POINT('Ctrl Pts',(-9.95791604830673E-14,76.2,-18.));
#298385=CARTESIAN_POINT('Ctrl Pts',(4.82308546378685,76.2,-18.));
#298386=CARTESIAN_POINT('Ctrl Pts',(10.3923048454797,74.5923048453941,-18.));
#298387=CARTESIAN_POINT('',(10.3923048454132,58.8076951545868,-18.));
#298388=CARTESIAN_POINT('',(10.3923048454132,57.2,-18.));
#298389=CARTESIAN_POINT('',(-1.406095999762E-13,57.2,-18.));
#298390=CARTESIAN_POINT('Ctrl Pts',(-1.37600294485693E-13,57.2,-18.));
#298391=CARTESIAN_POINT('Ctrl Pts',(4.82308546378685,57.2,-18.));
#298392=CARTESIAN_POINT('Ctrl Pts',(10.3923048454797,58.807695154606,-18.));
#298393=CARTESIAN_POINT('Ctrl Pts',(-10.3923048454799,58.8076951546059,
-18.));
#298394=CARTESIAN_POINT('Ctrl Pts',(-4.82308546378706,57.2,-18.));
#298395=CARTESIAN_POINT('Ctrl Pts',(-1.54800331296405E-13,57.2,-18.));
#298396=CARTESIAN_POINT('Origin',(20.7846096908265,57.2,-9.10794141489568E-15));
#298397=CARTESIAN_POINT('Ctrl Pts',(10.3923048453799,74.5923048453941,-18.0000000000576));
#298398=CARTESIAN_POINT('Ctrl Pts',(13.1769145362263,76.2,-13.176914536263));
#298399=CARTESIAN_POINT('Ctrl Pts',(15.5884572681198,76.2,-9.00000000000015));
#298400=CARTESIAN_POINT('Ctrl Pts',(15.5884572681198,76.2,-9.00000000000015));
#298401=CARTESIAN_POINT('Ctrl Pts',(18.0000000000133,76.2,-4.82308546373714));
#298402=CARTESIAN_POINT('Ctrl Pts',(20.7846096908597,74.592304845394,5.7606337033756E-11));
#298403=CARTESIAN_POINT('',(15.5884572681199,57.2,-8.99999999999999));
#298404=CARTESIAN_POINT('Ctrl Pts',(15.5884572681199,57.2000000000001,-8.99999999999997));
#298405=CARTESIAN_POINT('Ctrl Pts',(18.0000000000133,57.2000000000001,-4.82308546373704));
#298406=CARTESIAN_POINT('Ctrl Pts',(20.7846096908597,58.807695154606,5.76160899096971E-11));
#298407=CARTESIAN_POINT('Ctrl Pts',(10.3923048453799,58.807695154606,-18.0000000000576));
#298408=CARTESIAN_POINT('Ctrl Pts',(13.1769145362264,57.2000000000001,-13.176914536263));
#298409=CARTESIAN_POINT('Ctrl Pts',(15.5884572681199,57.2000000000001,-8.99999999999999));
#298410=CARTESIAN_POINT('Origin',(4.24836511114714E-14,57.2,0.));
#298411=CARTESIAN_POINT('Origin',(-1.37604970778725E-13,57.2,1.95387645016502E-29));
#298412=CARTESIAN_POINT('Origin',(-1.37604970778725E-13,57.2,6.74376190435982E-14));
#298413=CARTESIAN_POINT('Origin',(-1.37604970778725E-13,57.2,6.74376190435982E-14));
#298414=CARTESIAN_POINT('Origin',(-1.37604970778725E-13,57.2,6.74376190435982E-14));
#298415=CARTESIAN_POINT('Origin',(-1.37604970778725E-13,57.2,6.74376190435982E-14));
#298416=CARTESIAN_POINT('Origin',(-1.37604970778725E-13,57.2,6.74376190435982E-14));
#298417=CARTESIAN_POINT('Origin',(-1.37604970778725E-13,57.2,1.95387645016502E-29));
#298418=CARTESIAN_POINT('Origin',(-1.37604970778725E-13,57.2,1.95387645016502E-29));
#298419=CARTESIAN_POINT('Origin',(-1.37604970778725E-13,57.2,1.95387645016502E-29));
#298420=CARTESIAN_POINT('Origin',(-1.37604970778725E-13,57.2,1.95387645016502E-29));
#298421=CARTESIAN_POINT('Origin',(-1.37604970778725E-13,57.2,1.95387645016502E-29));
#298422=CARTESIAN_POINT('Origin',(-1.37604970778725E-13,57.2,1.95387645016502E-29));
#298423=CARTESIAN_POINT('Origin',(-1.78703160926406E-13,76.2,2.60289135494012E-29));
#298424=CARTESIAN_POINT('Origin',(-1.78703160926406E-13,76.2,2.60289135494012E-29));
#298425=CARTESIAN_POINT('Origin',(-1.78703160926406E-13,76.2,2.60289135494012E-29));
#298426=CARTESIAN_POINT('Origin',(-1.78703160926406E-13,76.2,2.60289135494012E-29));
#298427=CARTESIAN_POINT('Origin',(-1.78703160926406E-13,76.2,2.60289135494012E-29));
#298428=CARTESIAN_POINT('Origin',(-1.78703160926406E-13,76.2,2.60289135494012E-29));
#298429=CARTESIAN_POINT('Origin',(-1.38777878078145E-14,2.43125000000001,
0.));
#298430=CARTESIAN_POINT('Ctrl Pts',(-12.,2.43125000000001,1.10592091040473E-12));
#298431=CARTESIAN_POINT('Ctrl Pts',(-11.8804643241478,2.43125000000001,
1.79391945396996));
#298432=CARTESIAN_POINT('Ctrl Pts',(-11.3990610613138,2.43125000000001,
3.13396898737023));
#298433=CARTESIAN_POINT('Ctrl Pts',(-10.4104157884427,2.43125000000001,
5.318570795906));
#298434=CARTESIAN_POINT('Ctrl Pts',(-9.57359601299618,2.43125000000001,
6.56829747585552));
#298435=CARTESIAN_POINT('Ctrl Pts',(-7.38873844522587,2.43125000000001,
8.65742934749614));
#298436=CARTESIAN_POINT('Ctrl Pts',(-6.14298665404833,2.43125,9.45156675706131));
#298437=CARTESIAN_POINT('Ctrl Pts',(-3.8073824930157,2.43125,10.362657594245));
#298438=CARTESIAN_POINT('Ctrl Pts',(-2.35484140538957,2.43125000000001,
10.778449175978));
#298439=CARTESIAN_POINT('Ctrl Pts',(1.15015301169903,2.43125000000001,10.6841950237441));
#298440=CARTESIAN_POINT('Ctrl Pts',(2.53388342843634,2.43125000000001,10.2413561793839));
#298441=CARTESIAN_POINT('Ctrl Pts',(4.18319669729398,2.43125000000002,9.5097960999229));
#298442=CARTESIAN_POINT('Ctrl Pts',(4.85072362354194,2.43125000000002,9.11749903031561));
#298443=CARTESIAN_POINT('Ctrl Pts',(6.06416700972034,2.43125000000002,8.20405583130882));
#298444=CARTESIAN_POINT('Ctrl Pts',(6.60953367471901,2.43125000000002,7.69028293020246));
#298445=CARTESIAN_POINT('Ctrl Pts',(7.09357268597975,2.43125000000002,7.12128708482873));
#298446=CARTESIAN_POINT('Ctrl Pts',(10.0514428414954,2.43125000000002,1.00613961606655E-13));
#298447=CARTESIAN_POINT('Ctrl Pts',(10.1143780835885,2.43125000000002,-0.791127473640706));
#298448=CARTESIAN_POINT('Ctrl Pts',(10.0855072982437,2.43125000000002,-1.58682843497015));
#298449=CARTESIAN_POINT('Ctrl Pts',(9.84523379682252,2.43125000000002,-3.15557179232318));
#298450=CARTESIAN_POINT('Ctrl Pts',(9.63470068842676,2.43125000000002,-3.92325055631404));
#298451=CARTESIAN_POINT('Ctrl Pts',(8.67230516055593,2.43125000000002,-6.30994543448733));
#298452=CARTESIAN_POINT('Ctrl Pts',(7.71286120753459,2.43125000000002,-7.46066276667367));
#298453=CARTESIAN_POINT('Ctrl Pts',(6.06627958599162,2.43125000000002,-9.1152206243862));
#298454=CARTESIAN_POINT('Ctrl Pts',(4.9464571378071,2.43125000000001,-9.88345895797583));
#298455=CARTESIAN_POINT('Ctrl Pts',(2.75597210659317,2.43125000000001,-10.8484833593829));
#298456=CARTESIAN_POINT('Ctrl Pts',(1.37406648240357,2.43125000000002,-11.29221051564));
#298457=CARTESIAN_POINT('Ctrl Pts',(-1.98461349922251,2.43125000000001,
-11.4457083135333));
#298458=CARTESIAN_POINT('Ctrl Pts',(-3.50022085878334,2.43125000000001,
-11.1473855441023));
#298459=CARTESIAN_POINT('Ctrl Pts',(-6.14735486447011,2.43125000000001,
-10.1719281614562));
#298460=CARTESIAN_POINT('Ctrl Pts',(-7.38835529811323,2.43125000000001,
-9.4385927042382));
#298461=CARTESIAN_POINT('Ctrl Pts',(-8.46872171229246,2.43125000000001,
-8.50180878165033));
#298462=CARTESIAN_POINT('Ctrl Pts',(-10.0514428414942,-1.69374999998275,
2.46189346052968E-15));
#298463=CARTESIAN_POINT('Ctrl Pts',(-10.0514428414942,-1.54374999998335,
3.26591175476071));
#298464=CARTESIAN_POINT('Ctrl Pts',(-8.1317880767572,-1.39374999998395,
5.90808986649102));
#298465=CARTESIAN_POINT('Ctrl Pts',(-6.21213331202023,-1.24374999998455,
8.55026797822134));
#298466=CARTESIAN_POINT('Ctrl Pts',(-3.10606665601012,-1.09374999998515,
9.5594902125713));
#298467=CARTESIAN_POINT('Ctrl Pts',(-9.99267389681068E-15,-0.943749999985747,
10.5687124469213));
#298468=CARTESIAN_POINT('Ctrl Pts',(3.1060666560101,-0.793749999986346,
9.5594902125713));
#298469=CARTESIAN_POINT('Ctrl Pts',(6.21213331202021,-0.643749999986944,
8.55026797822134));
#298470=CARTESIAN_POINT('Ctrl Pts',(8.13178807675718,-0.493749999987543,
5.90808986649102));
#298471=CARTESIAN_POINT('Ctrl Pts',(10.0514428414942,-0.343749999988142,
3.2659117547607));
#298472=CARTESIAN_POINT('Ctrl Pts',(10.0514428414942,-0.193749999988742,
-1.23094673026484E-15));
#298473=CARTESIAN_POINT('Ctrl Pts',(10.0514428414942,-0.0437499999893418,
-3.26591175476071));
#298474=CARTESIAN_POINT('Ctrl Pts',(8.13178807675718,0.106250000010057,
-5.90808986649102));
#298475=CARTESIAN_POINT('Ctrl Pts',(6.2121333120202,0.256250000009456,-8.55026797822134));
#298476=CARTESIAN_POINT('Ctrl Pts',(3.10606665601009,0.406250000008854,
-9.5594902125713));
#298477=CARTESIAN_POINT('Ctrl Pts',(-1.34451165064878E-14,0.556250000008252,
-10.5687124469213));
#298478=CARTESIAN_POINT('Ctrl Pts',(-3.10606665601012,0.70625000000765,
-9.5594902125713));
#298479=CARTESIAN_POINT('Ctrl Pts',(-6.21213331202023,0.856250000007049,
-8.55026797822134));
#298480=CARTESIAN_POINT('Ctrl Pts',(-8.1317880767572,1.00625000000645,-5.90808986649102));
#298481=CARTESIAN_POINT('Ctrl Pts',(-10.0514428414942,1.15625000000585,
-3.2659117547607));
#298482=CARTESIAN_POINT('Ctrl Pts',(-10.0514428414942,1.30625000000525,
2.46189346052968E-15));
#298483=CARTESIAN_POINT('Ctrl Pts',(-10.0514428414942,1.45625000000465,
3.26591175476071));
#298484=CARTESIAN_POINT('Ctrl Pts',(-8.1317880767572,1.60625000000405,5.90808986649102));
#298485=CARTESIAN_POINT('Ctrl Pts',(-6.21213331202023,1.75625000000345,
8.55026797822134));
#298486=CARTESIAN_POINT('Ctrl Pts',(-3.10606665601012,1.90625000000285,
9.5594902125713));
#298487=CARTESIAN_POINT('Ctrl Pts',(-1.17203831684725E-14,2.05625000000225,
10.5687124469213));
#298488=CARTESIAN_POINT('Ctrl Pts',(3.1060666560101,2.20625000000165,9.5594902125713));
#298489=CARTESIAN_POINT('Ctrl Pts',(6.2121333120202,2.35625000000106,8.55026797822134));
#298490=CARTESIAN_POINT('Ctrl Pts',(8.13178807675718,2.50625000000046,5.90808986649102));
#298491=CARTESIAN_POINT('Ctrl Pts',(10.0514428414942,2.65624999999986,3.2659117547607));
#298492=CARTESIAN_POINT('Ctrl Pts',(10.0514428414942,2.80624999999926,-1.23094673026484E-15));
#298493=CARTESIAN_POINT('Ctrl Pts',(10.0514428414942,2.95624999999866,-3.26591175476071));
#298494=CARTESIAN_POINT('Ctrl Pts',(8.13178807675718,3.10624999999806,-5.90808986649102));
#298495=CARTESIAN_POINT('Ctrl Pts',(6.2121333120202,3.25624999999746,-8.55026797822134));
#298496=CARTESIAN_POINT('Ctrl Pts',(3.10606665601009,3.40624999999685,-9.5594902125713));
#298497=CARTESIAN_POINT('Ctrl Pts',(-1.51728257781496E-14,3.55624999999625,
-10.5687124469213));
#298498=CARTESIAN_POINT('Ctrl Pts',(-3.10606665601012,3.70624999999565,
-9.5594902125713));
#298499=CARTESIAN_POINT('Ctrl Pts',(-6.21213331202023,3.85624999999505,
-8.55026797822134));
#298500=CARTESIAN_POINT('Ctrl Pts',(-8.13178807675721,4.00624999999445,
-5.90808986649102));
#298501=CARTESIAN_POINT('Ctrl Pts',(-10.0514428414942,4.15624999999385,
-3.2659117547607));
#298502=CARTESIAN_POINT('Ctrl Pts',(-10.0514428414942,4.30624999999325,
2.46189346052968E-15));
#298503=CARTESIAN_POINT('Ctrl Pts',(-10.0514428414942,4.45624999999265,
3.26591175476071));
#298504=CARTESIAN_POINT('Ctrl Pts',(-8.13178807675721,4.60624999999205,
5.90808986649102));
#298505=CARTESIAN_POINT('Ctrl Pts',(-6.21213331202023,4.75624999999145,
8.55026797822134));
#298506=CARTESIAN_POINT('Ctrl Pts',(-3.10606665601012,4.90624999999085,
9.5594902125713));
#298507=CARTESIAN_POINT('Ctrl Pts',(-1.34480924401344E-14,5.05624999999025,
10.5687124469213));
#298508=CARTESIAN_POINT('Ctrl Pts',(3.10606665601009,5.20624999998966,9.5594902125713));
#298509=CARTESIAN_POINT('Ctrl Pts',(6.2121333120202,5.35624999998906,8.55026797822134));
#298510=CARTESIAN_POINT('Ctrl Pts',(8.13178807675718,5.50624999998846,5.90808986649102));
#298511=CARTESIAN_POINT('Ctrl Pts',(10.0514428414942,5.65624999998786,3.2659117547607));
#298512=CARTESIAN_POINT('Ctrl Pts',(10.0514428414941,5.80624999998726,-1.23094673026484E-15));
#298513=CARTESIAN_POINT('Ctrl Pts',(10.0514428414941,5.95624999998666,-3.26591175476071));
#298514=CARTESIAN_POINT('Ctrl Pts',(8.13178807675717,6.10624999998606,-5.90808986649102));
#298515=CARTESIAN_POINT('Ctrl Pts',(6.2121333120202,6.25624999998545,-8.55026797822134));
#298516=CARTESIAN_POINT('Ctrl Pts',(3.10606665601009,6.40624999998485,-9.5594902125713));
#298517=CARTESIAN_POINT('Ctrl Pts',(-1.69005350498115E-14,6.55624999998425,
-10.5687124469213));
#298518=CARTESIAN_POINT('Ctrl Pts',(-3.10606665601013,6.70624999998365,
-9.5594902125713));
#298519=CARTESIAN_POINT('Ctrl Pts',(-6.21213331202023,6.85624999998305,
-8.55026797822134));
#298520=CARTESIAN_POINT('Ctrl Pts',(-8.13178807675721,7.00624999998245,
-5.90808986649102));
#298521=CARTESIAN_POINT('Ctrl Pts',(-10.0514428414942,7.15624999998184,
-3.2659117547607));
#298522=CARTESIAN_POINT('Ctrl Pts',(-10.0514428414942,7.30624999998125,
2.46189346052968E-15));
#298523=CARTESIAN_POINT('Ctrl Pts',(-10.0514428414942,7.45624999998065,
3.26591175476071));
#298524=CARTESIAN_POINT('Ctrl Pts',(-8.13178807675721,7.60624999998005,
5.90808986649102));
#298525=CARTESIAN_POINT('Ctrl Pts',(-6.21213331202023,7.75624999997945,
8.55026797822134));
#298526=CARTESIAN_POINT('Ctrl Pts',(-3.10606665601012,7.90624999997885,
9.5594902125713));
#298527=CARTESIAN_POINT('Ctrl Pts',(-1.51758017117962E-14,8.05624999997825,
10.5687124469213));
#298528=CARTESIAN_POINT('Ctrl Pts',(3.10606665601009,8.20624999997765,9.5594902125713));
#298529=CARTESIAN_POINT('Ctrl Pts',(6.2121333120202,8.35624999997706,8.55026797822134));
#298530=CARTESIAN_POINT('Ctrl Pts',(8.13178807675717,8.50624999997646,5.90808986649102));
#298531=CARTESIAN_POINT('Ctrl Pts',(10.0514428414942,8.65624999997586,3.2659117547607));
#298532=CARTESIAN_POINT('Ctrl Pts',(10.0514428414941,8.80624999997526,-1.23094673026484E-15));
#298533=CARTESIAN_POINT('Ctrl Pts',(10.0514428414941,8.95624999997466,-3.26591175476071));
#298534=CARTESIAN_POINT('Ctrl Pts',(8.13178807675717,9.10624999997406,-5.90808986649102));
#298535=CARTESIAN_POINT('Ctrl Pts',(6.2121333120202,9.25624999997346,-8.55026797822134));
#298536=CARTESIAN_POINT('Ctrl Pts',(3.10606665601009,9.40624999997286,-9.5594902125713));
#298537=CARTESIAN_POINT('Ctrl Pts',(-1.86282443214733E-14,9.55624999997225,
-10.5687124469213));
#298538=CARTESIAN_POINT('Ctrl Pts',(-3.10606665601013,9.70624999997165,
-9.5594902125713));
#298539=CARTESIAN_POINT('Ctrl Pts',(-6.21213331202023,9.85624999997105,
-8.55026797822134));
#298540=CARTESIAN_POINT('Ctrl Pts',(-8.13178807675721,10.0062499999704,
-5.90808986649102));
#298541=CARTESIAN_POINT('Ctrl Pts',(-10.0514428414942,10.1562499999698,
-3.2659117547607));
#298542=CARTESIAN_POINT('Ctrl Pts',(-10.0514428414942,10.3062499999692,
2.46189346052968E-15));
#298543=CARTESIAN_POINT('Ctrl Pts',(-10.0514428414942,10.4562499999686,
3.26591175476071));
#298544=CARTESIAN_POINT('Ctrl Pts',(-8.13178807675721,10.606249999968,5.90808986649102));
#298545=CARTESIAN_POINT('Ctrl Pts',(-6.21213331202023,10.7562499999674,
8.55026797822134));
#298546=CARTESIAN_POINT('Ctrl Pts',(-3.10606665601013,10.9062499999668,
9.5594902125713));
#298547=CARTESIAN_POINT('Ctrl Pts',(-1.6903510983458E-14,11.0562499999663,
10.5687124469213));
#298548=CARTESIAN_POINT('Ctrl Pts',(3.10606665601009,11.2062499999657,9.5594902125713));
#298549=CARTESIAN_POINT('Ctrl Pts',(6.2121333120202,11.3562499999651,8.55026797822134));
#298550=CARTESIAN_POINT('Ctrl Pts',(8.13178807675717,11.5062499999645,5.90808986649102));
#298551=CARTESIAN_POINT('Ctrl Pts',(10.0514428414941,11.6562499999639,3.2659117547607));
#298552=CARTESIAN_POINT('Ctrl Pts',(10.0514428414941,11.8062499999633,-1.23094673026484E-15));
#298553=CARTESIAN_POINT('Ctrl Pts',(10.0514428414941,11.9562499999627,-3.26591175476071));
#298554=CARTESIAN_POINT('Ctrl Pts',(8.13178807675717,12.1062499999621,-5.90808986649102));
#298555=CARTESIAN_POINT('Ctrl Pts',(6.2121333120202,12.2562499999615,-8.55026797822134));
#298556=CARTESIAN_POINT('Ctrl Pts',(3.10606665601009,12.4062499999609,-9.5594902125713));
#298557=CARTESIAN_POINT('Ctrl Pts',(-2.03559535931351E-14,12.5562499999603,
-10.5687124469213));
#298558=CARTESIAN_POINT('Ctrl Pts',(-3.10606665601013,12.7062499999597,
-9.5594902125713));
#298559=CARTESIAN_POINT('Ctrl Pts',(-6.21213331202024,12.856249999959,-8.55026797822134));
#298560=CARTESIAN_POINT('Ctrl Pts',(-8.13178807675721,13.0062499999584,
-5.90808986649102));
#298561=CARTESIAN_POINT('Ctrl Pts',(-10.0514428414942,13.1562499999578,
-3.2659117547607));
#298562=CARTESIAN_POINT('Ctrl Pts',(-10.0514428414942,13.3062499999572,
2.46189346052968E-15));
#298563=CARTESIAN_POINT('Ctrl Pts',(-10.0514428414942,13.4562499999566,
3.26591175476071));
#298564=CARTESIAN_POINT('Ctrl Pts',(-8.13178807675721,13.606249999956,5.90808986649102));
#298565=CARTESIAN_POINT('Ctrl Pts',(-6.21213331202023,13.7562499999554,
8.55026797822134));
#298566=CARTESIAN_POINT('Ctrl Pts',(-3.10606665601013,13.9062499999549,
9.5594902125713));
#298567=CARTESIAN_POINT('Ctrl Pts',(-1.86312202551199E-14,14.0562499999543,
10.5687124469213));
#298568=CARTESIAN_POINT('Ctrl Pts',(3.10606665601009,14.2062499999537,9.5594902125713));
#298569=CARTESIAN_POINT('Ctrl Pts',(6.2121333120202,14.3562499999531,8.55026797822134));
#298570=CARTESIAN_POINT('Ctrl Pts',(8.13178807675717,14.5062499999525,5.90808986649102));
#298571=CARTESIAN_POINT('Ctrl Pts',(10.0514428414941,14.6562499999519,3.2659117547607));
#298572=CARTESIAN_POINT('Ctrl Pts',(10.0514428414941,14.8062499999513,-1.23094673026484E-15));
#298573=CARTESIAN_POINT('Ctrl Pts',(10.0514428414941,14.9562499999507,-3.26591175476071));
#298574=CARTESIAN_POINT('Ctrl Pts',(8.13178807675717,15.1062499999501,-5.90808986649102));
#298575=CARTESIAN_POINT('Ctrl Pts',(6.21213331202019,15.2562499999495,-8.55026797822134));
#298576=CARTESIAN_POINT('Ctrl Pts',(3.10606665601009,15.4062499999489,-9.5594902125713));
#298577=CARTESIAN_POINT('Ctrl Pts',(-2.2083662864797E-14,15.5562499999482,
-10.5687124469213));
#298578=CARTESIAN_POINT('Ctrl Pts',(-3.10606665601013,15.7062499999477,
-9.5594902125713));
#298579=CARTESIAN_POINT('Ctrl Pts',(-6.21213331202024,15.856249999947,-8.55026797822134));
#298580=CARTESIAN_POINT('Ctrl Pts',(-8.13178807675721,16.0062499999464,
-5.90808986649102));
#298581=CARTESIAN_POINT('Ctrl Pts',(-10.0514428414942,16.1562499999458,
-3.2659117547607));
#298582=CARTESIAN_POINT('Ctrl Pts',(-10.0514428414942,16.3062499999452,
2.46189346052968E-15));
#298583=CARTESIAN_POINT('Ctrl Pts',(-10.0514428414942,16.4562499999446,
3.26591175476071));
#298584=CARTESIAN_POINT('Ctrl Pts',(-8.13178807675721,16.606249999944,5.90808986649102));
#298585=CARTESIAN_POINT('Ctrl Pts',(-6.21213331202024,16.7562499999434,
8.55026797822134));
#298586=CARTESIAN_POINT('Ctrl Pts',(-3.10606665601013,16.9062499999428,
9.5594902125713));
#298587=CARTESIAN_POINT('Ctrl Pts',(-2.03589295267817E-14,17.0562499999422,
10.5687124469213));
#298588=CARTESIAN_POINT('Ctrl Pts',(3.10606665601009,17.2062499999417,9.5594902125713));
#298589=CARTESIAN_POINT('Ctrl Pts',(6.21213331202019,17.3562499999411,8.55026797822134));
#298590=CARTESIAN_POINT('Ctrl Pts',(8.13178807675717,17.5062499999405,5.90808986649102));
#298591=CARTESIAN_POINT('Ctrl Pts',(10.0514428414941,17.6562499999399,3.2659117547607));
#298592=CARTESIAN_POINT('Ctrl Pts',(10.0514428414941,17.8062499999393,-1.23094673026484E-15));
#298593=CARTESIAN_POINT('Ctrl Pts',(10.0514428414941,17.9562499999387,-3.26591175476071));
#298594=CARTESIAN_POINT('Ctrl Pts',(8.13178807675717,18.1062499999381,-5.90808986649102));
#298595=CARTESIAN_POINT('Ctrl Pts',(6.21213331202019,18.2562499999375,-8.55026797822134));
#298596=CARTESIAN_POINT('Ctrl Pts',(3.10606665601008,18.4062499999369,-9.5594902125713));
#298597=CARTESIAN_POINT('Ctrl Pts',(-2.38113721364588E-14,18.5562499999362,
-10.5687124469213));
#298598=CARTESIAN_POINT('Ctrl Pts',(-3.10606665601013,18.7062499999357,
-9.5594902125713));
#298599=CARTESIAN_POINT('Ctrl Pts',(-6.21213331202024,18.856249999935,-8.55026797822134));
#298600=CARTESIAN_POINT('Ctrl Pts',(-8.13178807675721,19.0062499999344,
-5.90808986649102));
#298601=CARTESIAN_POINT('Ctrl Pts',(-10.0514428414942,19.1562499999338,
-3.2659117547607));
#298602=CARTESIAN_POINT('Ctrl Pts',(-10.0514428414942,19.3062499999332,
2.46189346052968E-15));
#298603=CARTESIAN_POINT('Ctrl Pts',(-10.0514428414942,19.4562499999326,
3.26591175476071));
#298604=CARTESIAN_POINT('Ctrl Pts',(-8.13178807675721,19.606249999932,5.90808986649102));
#298605=CARTESIAN_POINT('Ctrl Pts',(-6.21213331202024,19.7562499999314,
8.55026797822134));
#298606=CARTESIAN_POINT('Ctrl Pts',(-3.10606665601013,19.9062499999308,
9.5594902125713));
#298607=CARTESIAN_POINT('Ctrl Pts',(-2.20866387984435E-14,20.0562499999302,
10.5687124469213));
#298608=CARTESIAN_POINT('Ctrl Pts',(3.10606665601009,20.2062499999297,9.5594902125713));
#298609=CARTESIAN_POINT('Ctrl Pts',(6.21213331202019,20.356249999929,8.55026797822134));
#298610=CARTESIAN_POINT('Ctrl Pts',(8.13178807675717,20.5062499999285,5.90808986649102));
#298611=CARTESIAN_POINT('Ctrl Pts',(10.0514428414941,20.6562499999279,3.2659117547607));
#298612=CARTESIAN_POINT('Ctrl Pts',(10.0514428414941,20.8062499999273,-1.23094673026484E-15));
#298613=CARTESIAN_POINT('Ctrl Pts',(10.0514428414941,20.9562499999267,-3.26591175476071));
#298614=CARTESIAN_POINT('Ctrl Pts',(8.13178807675716,21.1062499999261,-5.90808986649102));
#298615=CARTESIAN_POINT('Ctrl Pts',(6.21213331202019,21.2562499999255,-8.55026797822134));
#298616=CARTESIAN_POINT('Ctrl Pts',(3.10606665601008,21.4062499999249,-9.5594902125713));
#298617=CARTESIAN_POINT('Ctrl Pts',(-2.55390814081207E-14,21.5562499999242,
-10.5687124469213));
#298618=CARTESIAN_POINT('Ctrl Pts',(-3.10606665601013,21.7062499999237,
-9.5594902125713));
#298619=CARTESIAN_POINT('Ctrl Pts',(-6.21213331202024,21.856249999923,-8.55026797822134));
#298620=CARTESIAN_POINT('Ctrl Pts',(-8.13178807675722,22.0062499999224,
-5.90808986649102));
#298621=CARTESIAN_POINT('Ctrl Pts',(-10.0514428414942,22.1562499999218,
-3.2659117547607));
#298622=CARTESIAN_POINT('Ctrl Pts',(-10.0514428414942,22.3062499999212,
2.46189346052968E-15));
#298623=CARTESIAN_POINT('Ctrl Pts',(-10.0514428414942,22.4562499999206,
3.26591175476071));
#298624=CARTESIAN_POINT('Ctrl Pts',(-8.13178807675722,22.60624999992,5.90808986649102));
#298625=CARTESIAN_POINT('Ctrl Pts',(-6.21213331202024,22.7562499999194,
8.55026797822134));
#298626=CARTESIAN_POINT('Ctrl Pts',(-3.10606665601013,22.9062499999188,
9.5594902125713));
#298627=CARTESIAN_POINT('Ctrl Pts',(-2.38143480701054E-14,23.0562499999182,
10.5687124469213));
#298628=CARTESIAN_POINT('Ctrl Pts',(3.10606665601008,23.2062499999177,9.5594902125713));
#298629=CARTESIAN_POINT('Ctrl Pts',(6.21213331202019,23.3562499999171,8.55026797822134));
#298630=CARTESIAN_POINT('Ctrl Pts',(8.13178807675716,23.5062499999165,5.90808986649102));
#298631=CARTESIAN_POINT('Ctrl Pts',(10.0514428414941,23.6562499999159,3.2659117547607));
#298632=CARTESIAN_POINT('Ctrl Pts',(10.0514428414941,23.8062499999153,-1.23094673026484E-15));
#298633=CARTESIAN_POINT('Ctrl Pts',(10.0514428414941,23.9562499999147,-3.26591175476071));
#298634=CARTESIAN_POINT('Ctrl Pts',(8.13178807675716,24.1062499999141,-5.90808986649102));
#298635=CARTESIAN_POINT('Ctrl Pts',(6.21213331202019,24.2562499999135,-8.55026797822134));
#298636=CARTESIAN_POINT('Ctrl Pts',(3.10606665601008,24.4062499999129,-9.5594902125713));
#298637=CARTESIAN_POINT('Ctrl Pts',(-2.72667906797825E-14,24.5562499999122,
-10.5687124469213));
#298638=CARTESIAN_POINT('Ctrl Pts',(-3.10606665601014,24.7062499999116,
-9.5594902125713));
#298639=CARTESIAN_POINT('Ctrl Pts',(-6.21213331202024,24.856249999911,-8.55026797822134));
#298640=CARTESIAN_POINT('Ctrl Pts',(-8.13178807675722,25.0062499999104,
-5.90808986649102));
#298641=CARTESIAN_POINT('Ctrl Pts',(-10.0514428414942,25.1562499999098,
-3.2659117547607));
#298642=CARTESIAN_POINT('Ctrl Pts',(-10.0514428414942,25.3062499999092,
2.46189346052968E-15));
#298643=CARTESIAN_POINT('Ctrl Pts',(-10.0514428414942,25.4562499999086,
3.26591175476071));
#298644=CARTESIAN_POINT('Ctrl Pts',(-8.13178807675722,25.6062499999081,
5.90808986649102));
#298645=CARTESIAN_POINT('Ctrl Pts',(-6.21213331202024,25.7562499999074,
8.55026797822134));
#298646=CARTESIAN_POINT('Ctrl Pts',(-3.10606665601013,25.9062499999069,
9.5594902125713));
#298647=CARTESIAN_POINT('Ctrl Pts',(-2.55420573417672E-14,26.0562499999062,
10.5687124469213));
#298648=CARTESIAN_POINT('Ctrl Pts',(3.10606665601008,26.2062499999057,9.5594902125713));
#298649=CARTESIAN_POINT('Ctrl Pts',(6.21213331202019,26.356249999905,8.55026797822134));
#298650=CARTESIAN_POINT('Ctrl Pts',(8.13178807675716,26.5062499999045,5.90808986649102));
#298651=CARTESIAN_POINT('Ctrl Pts',(10.0514428414941,26.6562499999039,3.2659117547607));
#298652=CARTESIAN_POINT('Ctrl Pts',(10.0514428414941,26.8062499999033,-1.23094673026484E-15));
#298653=CARTESIAN_POINT('Ctrl Pts',(10.0514428414941,26.9562499999027,-3.26591175476071));
#298654=CARTESIAN_POINT('Ctrl Pts',(8.13178807675716,27.1062499999021,-5.90808986649102));
#298655=CARTESIAN_POINT('Ctrl Pts',(6.21213331202019,27.2562499999015,-8.55026797822134));
#298656=CARTESIAN_POINT('Ctrl Pts',(3.10606665601008,27.4062499999009,-9.5594902125713));
#298657=CARTESIAN_POINT('Ctrl Pts',(-2.89944999514443E-14,27.5562499999002,
-10.5687124469213));
#298658=CARTESIAN_POINT('Ctrl Pts',(-3.10606665601014,27.7062499998996,
-9.5594902125713));
#298659=CARTESIAN_POINT('Ctrl Pts',(-6.21213331202024,27.856249999899,-8.55026797822134));
#298660=CARTESIAN_POINT('Ctrl Pts',(-8.13178807675722,28.0062499998984,
-5.90808986649102));
#298661=CARTESIAN_POINT('Ctrl Pts',(-10.0514428414942,28.1562499998978,
-3.2659117547607));
#298662=CARTESIAN_POINT('Ctrl Pts',(-10.0514428414942,28.3062499998973,
2.46189346052968E-15));
#298663=CARTESIAN_POINT('Ctrl Pts',(-10.0514428414942,28.4562499998966,
3.26591175476071));
#298664=CARTESIAN_POINT('Ctrl Pts',(-8.13178807675722,28.606249999896,5.90808986649102));
#298665=CARTESIAN_POINT('Ctrl Pts',(-6.21213331202024,28.7562499998954,
8.55026797822134));
#298666=CARTESIAN_POINT('Ctrl Pts',(-3.10606665601014,28.9062499998949,
9.5594902125713));
#298667=CARTESIAN_POINT('Ctrl Pts',(-2.72697666134291E-14,29.0562499998942,
10.5687124469213));
#298668=CARTESIAN_POINT('Ctrl Pts',(3.10606665601008,29.2062499998937,9.5594902125713));
#298669=CARTESIAN_POINT('Ctrl Pts',(6.21213331202019,29.356249999893,8.55026797822134));
#298670=CARTESIAN_POINT('Ctrl Pts',(8.13178807675716,29.5062499998925,5.90808986649102));
#298671=CARTESIAN_POINT('Ctrl Pts',(10.0514428414941,29.6562499998919,3.2659117547607));
#298672=CARTESIAN_POINT('Ctrl Pts',(10.0514428414941,29.8062499998913,-1.23094673026484E-15));
#298673=CARTESIAN_POINT('Ctrl Pts',(10.0514428414941,29.9562499998907,-3.26591175476071));
#298674=CARTESIAN_POINT('Ctrl Pts',(8.13178807675716,30.1062499998901,-5.90808986649102));
#298675=CARTESIAN_POINT('Ctrl Pts',(6.21213331202019,30.2562499998895,-8.55026797822134));
#298676=CARTESIAN_POINT('Ctrl Pts',(3.10606665601008,30.4062499998889,-9.5594902125713));
#298677=CARTESIAN_POINT('Ctrl Pts',(-3.07222092231062E-14,30.5562499998883,
-10.5687124469213));
#298678=CARTESIAN_POINT('Ctrl Pts',(-3.10606665601014,30.7062499998877,
-9.5594902125713));
#298679=CARTESIAN_POINT('Ctrl Pts',(-6.21213331202025,30.8562499998871,
-8.55026797822134));
#298680=CARTESIAN_POINT('Ctrl Pts',(-8.13178807675722,31.0062499998864,
-5.90808986649102));
#298681=CARTESIAN_POINT('Ctrl Pts',(-10.0514428414942,31.1562499998858,
-3.2659117547607));
#298682=CARTESIAN_POINT('Ctrl Pts',(-10.0514428414942,31.3062499998852,
2.46189346052968E-15));
#298683=CARTESIAN_POINT('Ctrl Pts',(-10.0514428414942,31.4562499998847,
3.26591175476071));
#298684=CARTESIAN_POINT('Ctrl Pts',(-8.13178807675722,31.606249999884,5.90808986649102));
#298685=CARTESIAN_POINT('Ctrl Pts',(-6.21213331202024,31.7562499998835,
8.55026797822134));
#298686=CARTESIAN_POINT('Ctrl Pts',(-3.10606665601014,31.9062499998829,
9.5594902125713));
#298687=CARTESIAN_POINT('Ctrl Pts',(-2.89974758850909E-14,32.0562499998822,
10.5687124469213));
#298688=CARTESIAN_POINT('Ctrl Pts',(3.10606665601008,32.2062499998816,9.5594902125713));
#298689=CARTESIAN_POINT('Ctrl Pts',(6.21213331202019,32.3562499998811,8.55026797822134));
#298690=CARTESIAN_POINT('Ctrl Pts',(8.13178807675716,32.5062499998805,5.90808986649102));
#298691=CARTESIAN_POINT('Ctrl Pts',(10.0514428414941,32.6562499998798,3.2659117547607));
#298692=CARTESIAN_POINT('Ctrl Pts',(10.0514428414941,32.8062499998793,-1.23094673026484E-15));
#298693=CARTESIAN_POINT('Ctrl Pts',(10.0514428414941,32.9562499998787,-3.26591175476071));
#298694=CARTESIAN_POINT('Ctrl Pts',(8.13178807675716,33.1062499998781,-5.90808986649102));
#298695=CARTESIAN_POINT('Ctrl Pts',(6.21213331202019,33.2562499998775,-8.55026797822134));
#298696=CARTESIAN_POINT('Ctrl Pts',(3.10606665601008,33.4062499998769,-9.5594902125713));
#298697=CARTESIAN_POINT('Ctrl Pts',(-3.2449918494768E-14,33.5562499998763,
-10.5687124469213));
#298698=CARTESIAN_POINT('Ctrl Pts',(-3.10606665601014,33.7062499998756,
-9.5594902125713));
#298699=CARTESIAN_POINT('Ctrl Pts',(-6.21213331202025,33.8562499998751,
-8.55026797822134));
#298700=CARTESIAN_POINT('Ctrl Pts',(-8.13178807675722,34.0062499998744,
-5.90808986649102));
#298701=CARTESIAN_POINT('Ctrl Pts',(-10.0514428414942,34.1562499998739,
-3.2659117547607));
#298702=CARTESIAN_POINT('Ctrl Pts',(-10.0514428414942,34.3062499998732,
2.46189346052968E-15));
#298703=CARTESIAN_POINT('Ctrl Pts',(-10.0514428414942,34.4562499998727,
3.26591175476071));
#298704=CARTESIAN_POINT('Ctrl Pts',(-8.13178807675722,34.606249999872,5.90808986649102));
#298705=CARTESIAN_POINT('Ctrl Pts',(-6.21213331202024,34.7562499998715,
8.55026797822134));
#298706=CARTESIAN_POINT('Ctrl Pts',(-3.10606665601014,34.9062499998708,
9.5594902125713));
#298707=CARTESIAN_POINT('Ctrl Pts',(-3.07251851567527E-14,35.0562499998703,
10.5687124469213));
#298708=CARTESIAN_POINT('Ctrl Pts',(3.10606665601008,35.2062499998697,9.5594902125713));
#298709=CARTESIAN_POINT('Ctrl Pts',(6.21213331202019,35.3562499998691,8.55026797822134));
#298710=CARTESIAN_POINT('Ctrl Pts',(8.13178807675716,35.5062499998685,5.90808986649102));
#298711=CARTESIAN_POINT('Ctrl Pts',(10.0514428414941,35.6562499998679,3.2659117547607));
#298712=CARTESIAN_POINT('Ctrl Pts',(10.0514428414941,35.8062499998673,-1.23094673026484E-15));
#298713=CARTESIAN_POINT('Ctrl Pts',(10.0514428414941,35.9562499998667,-3.26591175476071));
#298714=CARTESIAN_POINT('Ctrl Pts',(8.13178807675716,36.1062499998661,-5.90808986649102));
#298715=CARTESIAN_POINT('Ctrl Pts',(6.21213331202018,36.2562499998655,-8.55026797822134));
#298716=CARTESIAN_POINT('Ctrl Pts',(3.10606665601007,36.4062499998649,-9.5594902125713));
#298717=CARTESIAN_POINT('Ctrl Pts',(-3.41776277664299E-14,36.5562499998642,
-10.5687124469213));
#298718=CARTESIAN_POINT('Ctrl Pts',(-3.10606665601014,36.7062499998636,
-9.5594902125713));
#298719=CARTESIAN_POINT('Ctrl Pts',(-6.21213331202025,36.856249999863,-8.55026797822134));
#298720=CARTESIAN_POINT('Ctrl Pts',(-8.13178807675722,37.0062499998624,
-5.90808986649102));
#298721=CARTESIAN_POINT('Ctrl Pts',(-10.0514428414942,37.1562499998618,
-3.2659117547607));
#298722=CARTESIAN_POINT('Ctrl Pts',(-10.0514428414942,37.3062499998613,
2.46189346052968E-15));
#298723=CARTESIAN_POINT('Ctrl Pts',(-10.0514428414942,37.4562499998606,
3.26591175476071));
#298724=CARTESIAN_POINT('Ctrl Pts',(-8.13178807675722,37.60624999986,5.90808986649102));
#298725=CARTESIAN_POINT('Ctrl Pts',(-6.21213331202025,37.7562499998594,
8.55026797822134));
#298726=CARTESIAN_POINT('Ctrl Pts',(-3.10606665601014,37.9062499998588,
9.5594902125713));
#298727=CARTESIAN_POINT('Ctrl Pts',(-3.24528944284146E-14,38.0562499998583,
10.5687124469213));
#298728=CARTESIAN_POINT('Ctrl Pts',(3.10606665601007,38.2062499998577,9.5594902125713));
#298729=CARTESIAN_POINT('Ctrl Pts',(6.21213331202018,38.3562499998571,8.55026797822134));
#298730=CARTESIAN_POINT('Ctrl Pts',(8.13178807675716,38.5062499998565,5.90808986649102));
#298731=CARTESIAN_POINT('Ctrl Pts',(10.0514428414941,38.6562499998559,3.2659117547607));
#298732=CARTESIAN_POINT('Ctrl Pts',(10.0514428414941,38.8062499998553,-1.23094673026484E-15));
#298733=CARTESIAN_POINT('Ctrl Pts',(10.0514428414941,38.9562499998547,-3.26591175476071));
#298734=CARTESIAN_POINT('Ctrl Pts',(8.13178807675715,39.1062499998541,-5.90808986649102));
#298735=CARTESIAN_POINT('Ctrl Pts',(6.21213331202018,39.2562499998535,-8.55026797822134));
#298736=CARTESIAN_POINT('Ctrl Pts',(3.10606665601007,39.4062499998529,-9.5594902125713));
#298737=CARTESIAN_POINT('Ctrl Pts',(-3.59053370380917E-14,39.5562499998523,
-10.5687124469213));
#298738=CARTESIAN_POINT('Ctrl Pts',(-3.10606665601014,39.7062499998516,
-9.5594902125713));
#298739=CARTESIAN_POINT('Ctrl Pts',(-6.21213331202025,39.856249999851,-8.55026797822134));
#298740=CARTESIAN_POINT('Ctrl Pts',(-8.13178807675723,40.0062499998505,
-5.90808986649102));
#298741=CARTESIAN_POINT('Ctrl Pts',(-10.0514428414942,40.1562499998499,
-3.2659117547607));
#298742=CARTESIAN_POINT('Ctrl Pts',(-10.0514428414942,40.3062499998493,
2.46189346052968E-15));
#298743=CARTESIAN_POINT('Ctrl Pts',(-10.0514428414942,40.4562499998487,
3.26591175476071));
#298744=CARTESIAN_POINT('Ctrl Pts',(-8.13178807675723,40.606249999848,5.90808986649102));
#298745=CARTESIAN_POINT('Ctrl Pts',(-6.21213331202025,40.7562499998475,
8.55026797822134));
#298746=CARTESIAN_POINT('Ctrl Pts',(-3.10606665601014,40.9062499998468,
9.5594902125713));
#298747=CARTESIAN_POINT('Ctrl Pts',(-3.41806037000764E-14,41.0562499998463,
10.5687124469213));
#298748=CARTESIAN_POINT('Ctrl Pts',(3.10606665601007,41.2062499998457,9.5594902125713));
#298749=CARTESIAN_POINT('Ctrl Pts',(6.21213331202018,41.3562499998451,8.55026797822134));
#298750=CARTESIAN_POINT('Ctrl Pts',(8.13178807675715,41.5062499998444,5.90808986649102));
#298751=CARTESIAN_POINT('Ctrl Pts',(10.0514428414941,41.6562499998439,3.2659117547607));
#298752=CARTESIAN_POINT('Ctrl Pts',(10.0514428414941,41.8062499998433,-1.23094673026484E-15));
#298753=CARTESIAN_POINT('Ctrl Pts',(10.0514428414941,41.9562499998427,-3.26591175476071));
#298754=CARTESIAN_POINT('Ctrl Pts',(8.13178807675715,42.1062499998421,-5.90808986649102));
#298755=CARTESIAN_POINT('Ctrl Pts',(6.21213331202018,42.2562499998414,-8.55026797822134));
#298756=CARTESIAN_POINT('Ctrl Pts',(3.10606665601007,42.4062499998408,-9.5594902125713));
#298757=CARTESIAN_POINT('Ctrl Pts',(-3.76330463097535E-14,42.5562499998402,
-10.5687124469213));
#298758=CARTESIAN_POINT('Ctrl Pts',(-3.10606665601015,42.7062499998396,
-9.5594902125713));
#298759=CARTESIAN_POINT('Ctrl Pts',(-6.21213331202025,42.8562499998391,
-8.55026797822134));
#298760=CARTESIAN_POINT('Ctrl Pts',(-8.13178807675723,43.0062499998385,
-5.90808986649102));
#298761=CARTESIAN_POINT('Ctrl Pts',(-10.0514428414942,43.1562499998379,
-3.2659117547607));
#298762=CARTESIAN_POINT('Ctrl Pts',(-10.0514428414942,43.3062499998373,
2.46189346052968E-15));
#298763=CARTESIAN_POINT('Ctrl Pts',(-10.0514428414942,43.4562499998366,
3.26591175476071));
#298764=CARTESIAN_POINT('Ctrl Pts',(-8.13178807675723,43.6062499998361,
5.90808986649102));
#298765=CARTESIAN_POINT('Ctrl Pts',(-6.21213331202025,43.7562499998354,
8.55026797822134));
#298766=CARTESIAN_POINT('Ctrl Pts',(-3.10606665601014,43.9062499998348,
9.5594902125713));
#298767=CARTESIAN_POINT('Ctrl Pts',(-3.59083129717383E-14,44.0562499998343,
10.5687124469213));
#298768=CARTESIAN_POINT('Ctrl Pts',(3.10606665601007,44.2062499998337,9.5594902125713));
#298769=CARTESIAN_POINT('Ctrl Pts',(6.21213331202018,44.3562499998331,8.55026797822134));
#298770=CARTESIAN_POINT('Ctrl Pts',(8.13178807675715,44.5062499998324,5.90808986649102));
#298771=CARTESIAN_POINT('Ctrl Pts',(10.0514428414941,44.6562499998319,3.2659117547607));
#298772=CARTESIAN_POINT('Ctrl Pts',(10.0514428414941,44.8062499998313,-1.23094673026484E-15));
#298773=CARTESIAN_POINT('Ctrl Pts',(10.0514428414941,44.9562499998307,-3.26591175476071));
#298774=CARTESIAN_POINT('Ctrl Pts',(8.13178807675715,45.1062499998301,-5.90808986649102));
#298775=CARTESIAN_POINT('Ctrl Pts',(6.21213331202018,45.2562499998295,-8.55026797822134));
#298776=CARTESIAN_POINT('Ctrl Pts',(3.10606665601007,45.4062499998289,-9.5594902125713));
#298777=CARTESIAN_POINT('Ctrl Pts',(-3.93607555814154E-14,45.5562499998283,
-10.5687124469213));
#298778=CARTESIAN_POINT('Ctrl Pts',(-3.10606665601015,45.7062499998276,
-9.5594902125713));
#298779=CARTESIAN_POINT('Ctrl Pts',(-6.21213331202026,45.856249999827,-8.55026797822134));
#298780=CARTESIAN_POINT('Ctrl Pts',(-8.13178807675723,46.0062499998265,
-5.90808986649102));
#298781=CARTESIAN_POINT('Ctrl Pts',(-10.0514428414942,46.1562499998259,
-3.2659117547607));
#298782=CARTESIAN_POINT('Ctrl Pts',(-10.0514428414942,46.3062499998252,
2.46189346052968E-15));
#298783=CARTESIAN_POINT('Ctrl Pts',(-10.0514428414942,46.4562499998247,
3.26591175476071));
#298784=CARTESIAN_POINT('Ctrl Pts',(-8.13178807675723,46.606249999824,5.90808986649102));
#298785=CARTESIAN_POINT('Ctrl Pts',(-6.21213331202025,46.7562499998235,
8.55026797822134));
#298786=CARTESIAN_POINT('Ctrl Pts',(-3.10606665601015,46.9062499998228,
9.5594902125713));
#298787=CARTESIAN_POINT('Ctrl Pts',(-3.76360222434001E-14,47.0562499998223,
10.5687124469213));
#298788=CARTESIAN_POINT('Ctrl Pts',(3.10606665601007,47.2062499998217,9.5594902125713));
#298789=CARTESIAN_POINT('Ctrl Pts',(6.21213331202018,47.3562499998211,8.55026797822134));
#298790=CARTESIAN_POINT('Ctrl Pts',(8.13178807675715,47.5062499998204,5.90808986649102));
#298791=CARTESIAN_POINT('Ctrl Pts',(10.0514428414941,47.6562499998198,3.2659117547607));
#298792=CARTESIAN_POINT('Ctrl Pts',(10.0514428414941,47.8062499998193,-1.23094673026484E-15));
#298793=CARTESIAN_POINT('Ctrl Pts',(10.0514428414941,47.9562499998186,-3.26591175476071));
#298794=CARTESIAN_POINT('Ctrl Pts',(8.13178807675715,48.1062499998181,-5.90808986649102));
#298795=CARTESIAN_POINT('Ctrl Pts',(6.21213331202017,48.2562499998174,-8.55026797822134));
#298796=CARTESIAN_POINT('Ctrl Pts',(3.10606665601007,48.4062499998169,-9.5594902125713));
#298797=CARTESIAN_POINT('Ctrl Pts',(-4.10884648530772E-14,48.5562499998163,
-10.5687124469213));
#298798=CARTESIAN_POINT('Ctrl Pts',(-3.10606665601015,48.7062499998157,
-9.5594902125713));
#298799=CARTESIAN_POINT('Ctrl Pts',(-6.21213331202026,48.8562499998151,
-8.55026797822134));
#298800=CARTESIAN_POINT('Ctrl Pts',(-8.13178807675723,49.0062499998145,
-5.90808986649102));
#298801=CARTESIAN_POINT('Ctrl Pts',(-10.0514428414942,49.1562499998138,
-3.2659117547607));
#298802=CARTESIAN_POINT('Ctrl Pts',(-10.0514428414942,49.3062499998132,
2.46189346052968E-15));
#298803=CARTESIAN_POINT('Ctrl Pts',(-10.0514428414942,49.4562499998126,
3.26591175476071));
#298804=CARTESIAN_POINT('Ctrl Pts',(-8.13178807675723,49.6062499998121,
5.90808986649102));
#298805=CARTESIAN_POINT('Ctrl Pts',(-6.21213331202026,49.7562499998114,
8.55026797822134));
#298806=CARTESIAN_POINT('Ctrl Pts',(-3.10606665601015,49.9062499998109,
9.5594902125713));
#298807=CARTESIAN_POINT('Ctrl Pts',(-3.9363731515062E-14,50.0562499998103,
10.5687124469213));
#298808=CARTESIAN_POINT('Ctrl Pts',(3.10606665601007,50.2062499998097,9.5594902125713));
#298809=CARTESIAN_POINT('Ctrl Pts',(6.21213331202017,50.3562499998091,8.55026797822134));
#298810=CARTESIAN_POINT('Ctrl Pts',(8.13178807675715,50.5062499998085,5.90808986649102));
#298811=CARTESIAN_POINT('Ctrl Pts',(10.0514428414941,50.6562499998078,3.2659117547607));
#298812=CARTESIAN_POINT('Ctrl Pts',(10.0514428414941,50.8062499998072,-1.23094673026484E-15));
#298813=CARTESIAN_POINT('Ctrl Pts',(10.0514428414941,50.9562499998067,-3.26591175476071));
#298814=CARTESIAN_POINT('Ctrl Pts',(8.13178807675715,51.1062499998061,-5.90808986649102));
#298815=CARTESIAN_POINT('Ctrl Pts',(6.21213331202017,51.2562499998055,-8.55026797822134));
#298816=CARTESIAN_POINT('Ctrl Pts',(3.10606665601006,51.4062499998048,-9.5594902125713));
#298817=CARTESIAN_POINT('Ctrl Pts',(-4.2816174124739E-14,51.5562499998043,
-10.5687124469213));
#298818=CARTESIAN_POINT('Ctrl Pts',(-3.10606665601015,51.7062499998037,
-9.5594902125713));
#298819=CARTESIAN_POINT('Ctrl Pts',(-6.21213331202026,51.856249999803,-8.55026797822134));
#298820=CARTESIAN_POINT('Ctrl Pts',(-8.13178807675723,52.0062499998025,
-5.90808986649102));
#298821=CARTESIAN_POINT('Ctrl Pts',(-10.0514428414942,52.1562499998019,
-3.2659117547607));
#298822=CARTESIAN_POINT('Ctrl Pts',(-10.0514428414942,52.3062499998012,
2.46189346052968E-15));
#298823=CARTESIAN_POINT('Ctrl Pts',(-10.0514428414942,52.4562499998006,
3.26591175476071));
#298824=CARTESIAN_POINT('Ctrl Pts',(-8.13178807675723,52.6062499998,5.90808986649102));
#298825=CARTESIAN_POINT('Ctrl Pts',(-6.21213331202026,52.7562499997994,
8.55026797822134));
#298826=CARTESIAN_POINT('Ctrl Pts',(-3.10606665601015,52.9062499997988,
9.5594902125713));
#298827=CARTESIAN_POINT('Ctrl Pts',(-4.10914407867238E-14,53.0562499997983,
10.5687124469213));
#298828=CARTESIAN_POINT('Ctrl Pts',(3.10606665601007,53.2062499997976,9.5594902125713));
#298829=CARTESIAN_POINT('Ctrl Pts',(6.21213331202017,53.3562499997971,8.55026797822134));
#298830=CARTESIAN_POINT('Ctrl Pts',(8.13178807675715,53.5062499997965,5.90808986649102));
#298831=CARTESIAN_POINT('Ctrl Pts',(10.0514428414941,53.6562499997959,3.2659117547607));
#298832=CARTESIAN_POINT('Ctrl Pts',(10.0514428414941,53.8062499997953,-1.23094673026484E-15));
#298833=CARTESIAN_POINT('Ctrl Pts',(10.0514428414941,53.9562499997946,-3.26591175476071));
#298834=CARTESIAN_POINT('Ctrl Pts',(8.13178807675714,54.106249999794,-5.90808986649102));
#298835=CARTESIAN_POINT('Ctrl Pts',(6.21213331202017,54.2562499997934,-8.55026797822134));
#298836=CARTESIAN_POINT('Ctrl Pts',(3.10606665601006,54.4062499997928,-9.5594902125713));
#298837=CARTESIAN_POINT('Ctrl Pts',(-4.45438833964009E-14,54.5562499997923,
-10.5687124469213));
#298838=CARTESIAN_POINT('Ctrl Pts',(-3.10606665601015,54.7062499997917,
-9.5594902125713));
#298839=CARTESIAN_POINT('Ctrl Pts',(-6.21213331202026,54.856249999791,-8.55026797822134));
#298840=CARTESIAN_POINT('Ctrl Pts',(-8.13178807675724,55.0062499997905,
-5.90808986649102));
#298841=CARTESIAN_POINT('Ctrl Pts',(-10.0514428414942,55.1562499997898,
-3.2659117547607));
#298842=CARTESIAN_POINT('Ctrl Pts',(-10.0514428414942,55.3062499997893,
2.46189346052968E-15));
#298843=CARTESIAN_POINT('Ctrl Pts',(-10.0514428414942,55.4562499997886,
3.26591175476071));
#298844=CARTESIAN_POINT('Ctrl Pts',(-8.13178807675724,55.606249999788,5.90808986649102));
#298845=CARTESIAN_POINT('Ctrl Pts',(-6.21213331202026,55.7562499997874,
8.55026797822134));
#298846=CARTESIAN_POINT('Ctrl Pts',(-3.10606665601015,55.9062499997869,
9.5594902125713));
#298847=CARTESIAN_POINT('Ctrl Pts',(-4.28191500583856E-14,56.0562499997862,
10.5687124469213));
#298848=CARTESIAN_POINT('Ctrl Pts',(3.10606665601006,56.2062499997857,9.5594902125713));
#298849=CARTESIAN_POINT('Ctrl Pts',(6.21213331202017,56.356249999785,8.55026797822134));
#298850=CARTESIAN_POINT('Ctrl Pts',(8.13178807675714,56.5062499997845,5.90808986649102));
#298851=CARTESIAN_POINT('Ctrl Pts',(10.0514428414941,56.6562499997839,3.2659117547607));
#298852=CARTESIAN_POINT('Ctrl Pts',(10.0514428414941,56.8062499997833,-1.23094673026484E-15));
#298853=CARTESIAN_POINT('Ctrl Pts',(10.0514428414941,56.9562499997827,-3.26591175476071));
#298854=CARTESIAN_POINT('Ctrl Pts',(8.13178807675714,57.1062499997821,-5.90808986649102));
#298855=CARTESIAN_POINT('Ctrl Pts',(6.21213331202017,57.2562499997814,-8.55026797822134));
#298856=CARTESIAN_POINT('Ctrl Pts',(3.10606665601006,57.4062499997808,-9.5594902125713));
#298857=CARTESIAN_POINT('Ctrl Pts',(-4.62715926680627E-14,57.5562499997802,
-10.5687124469213));
#298858=CARTESIAN_POINT('Ctrl Pts',(-3.10606665601015,57.7062499997797,
-9.5594902125713));
#298859=CARTESIAN_POINT('Ctrl Pts',(-6.21213331202026,57.856249999779,-8.55026797822134));
#298860=CARTESIAN_POINT('Ctrl Pts',(-8.13178807675724,58.0062499997784,
-5.90808986649102));
#298861=CARTESIAN_POINT('Ctrl Pts',(-10.0514428414942,58.1562499997778,
-3.2659117547607));
#298862=CARTESIAN_POINT('Ctrl Pts',(-10.0514428414942,58.3062499997773,
2.46189346052968E-15));
#298863=CARTESIAN_POINT('Ctrl Pts',(-10.0514428414942,58.4562499997766,
3.26591175476071));
#298864=CARTESIAN_POINT('Ctrl Pts',(-8.13178807675724,58.6062499997761,
5.90808986649102));
#298865=CARTESIAN_POINT('Ctrl Pts',(-6.21213331202026,58.7562499997754,
8.55026797822134));
#298866=CARTESIAN_POINT('Ctrl Pts',(-3.10606665601015,58.9062499997749,
9.5594902125713));
#298867=CARTESIAN_POINT('Ctrl Pts',(-4.45468593300475E-14,59.0562499997743,
10.5687124469213));
#298868=CARTESIAN_POINT('Ctrl Pts',(3.10606665601006,59.2062499997736,9.5594902125713));
#298869=CARTESIAN_POINT('Ctrl Pts',(6.21213331202017,59.356249999773,8.55026797822134));
#298870=CARTESIAN_POINT('Ctrl Pts',(8.13178807675714,59.5062499997725,5.90808986649102));
#298871=CARTESIAN_POINT('Ctrl Pts',(10.0514428414941,59.6562499997718,3.2659117547607));
#298872=CARTESIAN_POINT('Ctrl Pts',(10.0514428414941,59.8062499997713,-1.23094673026484E-15));
#298873=CARTESIAN_POINT('Ctrl Pts',(10.0514428414941,59.9562499997706,-3.26591175476071));
#298874=CARTESIAN_POINT('Ctrl Pts',(8.13178807675714,60.10624999977,-5.90808986649102));
#298875=CARTESIAN_POINT('Ctrl Pts',(6.21213331202017,60.2562499997694,-8.55026797822134));
#298876=CARTESIAN_POINT('Ctrl Pts',(3.10606665601006,60.4062499997689,-9.5594902125713));
#298877=CARTESIAN_POINT('Ctrl Pts',(-4.79993019397246E-14,60.5562499997682,
-10.5687124469213));
#298878=CARTESIAN_POINT('Ctrl Pts',(-3.10606665601016,60.7062499997676,
-9.5594902125713));
#298879=CARTESIAN_POINT('Ctrl Pts',(-6.21213331202026,60.856249999767,-8.55026797822134));
#298880=CARTESIAN_POINT('Ctrl Pts',(-8.13178807675724,61.0062499997664,
-5.90808986649102));
#298881=CARTESIAN_POINT('Ctrl Pts',(-10.0514428414942,61.1562499997658,
-3.2659117547607));
#298882=CARTESIAN_POINT('Ctrl Pts',(-10.0514428414942,61.3062499997652,
2.46189346052968E-15));
#298883=CARTESIAN_POINT('Ctrl Pts',(-10.0514428414942,61.4562499997646,
3.26591175476071));
#298884=CARTESIAN_POINT('Ctrl Pts',(-8.13178807675724,61.6062499997641,
5.90808986649102));
#298885=CARTESIAN_POINT('Ctrl Pts',(-6.21213331202026,61.7562499997634,
8.55026797822134));
#298886=CARTESIAN_POINT('Ctrl Pts',(-3.10606665601015,61.9062499997628,
9.5594902125713));
#298887=CARTESIAN_POINT('Ctrl Pts',(-4.62745686017093E-14,62.0562499997622,
10.5687124469213));
#298888=CARTESIAN_POINT('Ctrl Pts',(3.10606665601006,62.2062499997617,9.5594902125713));
#298889=CARTESIAN_POINT('Ctrl Pts',(6.21213331202017,62.356249999761,8.55026797822134));
#298890=CARTESIAN_POINT('Ctrl Pts',(8.13178807675714,62.5062499997605,5.90808986649102));
#298891=CARTESIAN_POINT('Ctrl Pts',(10.0514428414941,62.6562499997599,3.2659117547607));
#298892=CARTESIAN_POINT('Ctrl Pts',(10.0514428414941,62.8062499997593,-1.23094673026484E-15));
#298893=CARTESIAN_POINT('Ctrl Pts',(10.0514428414941,62.9562499997587,-3.26591175476071));
#298894=CARTESIAN_POINT('Ctrl Pts',(8.13178807675714,63.1062499997581,-5.90808986649102));
#298895=CARTESIAN_POINT('Ctrl Pts',(6.21213331202017,63.2562499997575,-8.55026797822134));
#298896=CARTESIAN_POINT('Ctrl Pts',(3.10606665601006,63.4062499997568,-9.5594902125713));
#298897=CARTESIAN_POINT('Ctrl Pts',(-4.97270112113864E-14,63.5562499997562,
-10.5687124469213));
#298898=CARTESIAN_POINT('Ctrl Pts',(-3.10606665601016,63.7062499997556,
-9.5594902125713));
#298899=CARTESIAN_POINT('Ctrl Pts',(-6.21213331202027,63.8562499997551,
-8.55026797822134));
#298900=CARTESIAN_POINT('Ctrl Pts',(-8.13178807675724,64.0062499997544,
-5.90808986649102));
#298901=CARTESIAN_POINT('Ctrl Pts',(-10.0514428414942,64.1562499997538,
-3.2659117547607));
#298902=CARTESIAN_POINT('Ctrl Pts',(-10.0514428414942,64.3062499997532,
2.46189346052968E-15));
#298903=CARTESIAN_POINT('Ctrl Pts',(-10.0514428414942,64.4562499997526,
3.26591175476071));
#298904=CARTESIAN_POINT('Ctrl Pts',(-8.13178807675724,64.606249999752,5.90808986649102));
#298905=CARTESIAN_POINT('Ctrl Pts',(-6.21213331202026,64.7562499997514,
8.55026797822134));
#298906=CARTESIAN_POINT('Ctrl Pts',(-3.10606665601016,64.9062499997509,
9.5594902125713));
#298907=CARTESIAN_POINT('Ctrl Pts',(-4.80022778733711E-14,65.0562499997502,
10.5687124469213));
#298908=CARTESIAN_POINT('Ctrl Pts',(3.10606665601006,65.2062499997497,9.5594902125713));
#298909=CARTESIAN_POINT('Ctrl Pts',(6.21213331202017,65.3562499997491,8.55026797822134));
#298910=CARTESIAN_POINT('Ctrl Pts',(8.13178807675714,65.5062499997484,5.90808986649102));
#298911=CARTESIAN_POINT('Ctrl Pts',(10.0514428414941,65.6562499997479,3.2659117547607));
#298912=CARTESIAN_POINT('Ctrl Pts',(10.0514428414941,65.8062499997473,-1.23094673026484E-15));
#298913=CARTESIAN_POINT('Ctrl Pts',(10.0514428414941,65.9562499997467,-3.26591175476071));
#298914=CARTESIAN_POINT('Ctrl Pts',(8.13178807675714,66.1062499997461,-5.90808986649102));
#298915=CARTESIAN_POINT('Ctrl Pts',(6.21213331202016,66.2562499997454,-8.55026797822134));
#298916=CARTESIAN_POINT('Ctrl Pts',(3.10606665601006,66.4062499997449,-9.5594902125713));
#298917=CARTESIAN_POINT('Ctrl Pts',(-5.14547204830482E-14,66.5562499997443,
-10.5687124469213));
#298918=CARTESIAN_POINT('Ctrl Pts',(-3.10606665601016,66.7062499997436,
-9.5594902125713));
#298919=CARTESIAN_POINT('Ctrl Pts',(-6.21213331202027,66.8562499997431,
-8.55026797822134));
#298920=CARTESIAN_POINT('Ctrl Pts',(-8.13178807675724,67.0062499997424,
-5.90808986649102));
#298921=CARTESIAN_POINT('Ctrl Pts',(-10.0514428414942,67.1562499997418,
-3.2659117547607));
#298922=CARTESIAN_POINT('Ctrl Pts',(-10.0514428414942,67.3062499997412,
2.46189346052968E-15));
#298923=CARTESIAN_POINT('Ctrl Pts',(-10.0514428414942,67.4562499997406,
3.26591175476071));
#298924=CARTESIAN_POINT('Ctrl Pts',(-8.13178807675724,67.60624999974,5.90808986649102));
#298925=CARTESIAN_POINT('Ctrl Pts',(-6.21213331202027,67.7562499997395,
8.55026797822134));
#298926=CARTESIAN_POINT('Ctrl Pts',(-3.10606665601016,67.9062499997388,
9.5594902125713));
#298927=CARTESIAN_POINT('Ctrl Pts',(-4.9729987145033E-14,68.0562499997382,
10.5687124469213));
#298928=CARTESIAN_POINT('Ctrl Pts',(3.10606665601006,68.2062499997377,9.5594902125713));
#298929=CARTESIAN_POINT('Ctrl Pts',(6.21213331202017,68.356249999737,8.55026797822134));
#298930=CARTESIAN_POINT('Ctrl Pts',(8.13178807675714,68.5062499997365,5.90808986649102));
#298931=CARTESIAN_POINT('Ctrl Pts',(10.0514428414941,68.6562499997358,3.2659117547607));
#298932=CARTESIAN_POINT('Ctrl Pts',(10.0514428414941,68.8062499997353,-1.23094673026484E-15));
#298933=CARTESIAN_POINT('Ctrl Pts',(10.0514428414941,68.9562499997347,-3.26591175476071));
#298934=CARTESIAN_POINT('Ctrl Pts',(8.13178807675714,69.1062499997341,-5.90808986649102));
#298935=CARTESIAN_POINT('Ctrl Pts',(6.21213331202016,69.2562499997335,-8.55026797822134));
#298936=CARTESIAN_POINT('Ctrl Pts',(3.10606665601005,69.4062499997329,-9.5594902125713));
#298937=CARTESIAN_POINT('Ctrl Pts',(-5.31824297547101E-14,69.5562499997323,
-10.5687124469213));
#298938=CARTESIAN_POINT('Ctrl Pts',(-3.10606665601016,69.7062499997317,
-9.5594902125713));
#298939=CARTESIAN_POINT('Ctrl Pts',(-6.21213331202027,69.856249999731,-8.55026797822134));
#298940=CARTESIAN_POINT('Ctrl Pts',(-8.13178807675724,70.0062499997304,
-5.90808986649102));
#298941=CARTESIAN_POINT('Ctrl Pts',(-10.0514428414942,70.1562499997298,
-3.2659117547607));
#298942=CARTESIAN_POINT('Ctrl Pts',(-10.0514428414942,70.3062499997292,
2.46189346052968E-15));
#298943=CARTESIAN_POINT('Ctrl Pts',(-10.0514428414942,70.4562499997286,
3.26591175476071));
#298944=CARTESIAN_POINT('Ctrl Pts',(-8.13178807675724,70.606249999728,5.90808986649102));
#298945=CARTESIAN_POINT('Ctrl Pts',(-6.21213331202027,70.7562499997274,
8.55026797822134));
#298946=CARTESIAN_POINT('Ctrl Pts',(-3.10606665601016,70.9062499997269,
9.5594902125713));
#298947=CARTESIAN_POINT('Ctrl Pts',(-5.14576964166948E-14,71.0562499997262,
10.5687124469213));
#298948=CARTESIAN_POINT('Ctrl Pts',(3.10606665601006,71.2062499997256,9.5594902125713));
#298949=CARTESIAN_POINT('Ctrl Pts',(6.21213331202016,71.3562499997251,8.55026797822134));
#298950=CARTESIAN_POINT('Ctrl Pts',(8.13178807675714,71.5062499997244,5.90808986649102));
#298951=CARTESIAN_POINT('Ctrl Pts',(10.0514428414941,71.6562499997239,3.2659117547607));
#298952=CARTESIAN_POINT('Ctrl Pts',(10.0514428414941,71.8062499997232,-1.23094673026484E-15));
#298953=CARTESIAN_POINT('Ctrl Pts',(10.0514428414941,71.9562499997227,-3.26591175476071));
#298954=CARTESIAN_POINT('Ctrl Pts',(8.13178807675713,72.1062499997221,-5.90808986649102));
#298955=CARTESIAN_POINT('Ctrl Pts',(6.21213331202016,72.2562499997215,-8.55026797822134));
#298956=CARTESIAN_POINT('Ctrl Pts',(3.10606665601005,72.4062499997209,-9.5594902125713));
#298957=CARTESIAN_POINT('Ctrl Pts',(-5.49101390263719E-14,72.5562499997203,
-10.5687124469213));
#298958=CARTESIAN_POINT('Ctrl Pts',(-3.10606665601016,72.7062499997197,
-9.5594902125713));
#298959=CARTESIAN_POINT('Ctrl Pts',(-6.21213331202027,72.8562499997191,
-8.55026797822134));
#298960=CARTESIAN_POINT('Ctrl Pts',(-8.13178807675725,73.0062499997184,
-5.90808986649102));
#298961=CARTESIAN_POINT('Ctrl Pts',(-10.0514428414942,73.1562499997178,
-3.2659117547607));
#298962=CARTESIAN_POINT('Ctrl Pts',(-10.0514428414942,73.3062499997172,
2.46189346052968E-15));
#298963=CARTESIAN_POINT('Ctrl Pts',(-10.0514428414942,73.4562499997166,
3.26591175476071));
#298964=CARTESIAN_POINT('Ctrl Pts',(-8.13178807675725,73.606249999716,5.90808986649102));
#298965=CARTESIAN_POINT('Ctrl Pts',(-6.21213331202027,73.7562499997155,
8.55026797822134));
#298966=CARTESIAN_POINT('Ctrl Pts',(-3.10606665601016,73.9062499997148,
9.5594902125713));
#298967=CARTESIAN_POINT('Ctrl Pts',(-5.31854056883567E-14,74.0562499997143,
10.5687124469213));
#298968=CARTESIAN_POINT('Ctrl Pts',(3.10606665601005,74.2062499997136,9.5594902125713));
#298969=CARTESIAN_POINT('Ctrl Pts',(6.21213331202016,74.3562499997131,8.55026797822134));
#298970=CARTESIAN_POINT('Ctrl Pts',(8.13178807675713,74.5062499997125,5.90808986649102));
#298971=CARTESIAN_POINT('Ctrl Pts',(10.0514428414941,74.6562499997118,3.2659117547607));
#298972=CARTESIAN_POINT('Ctrl Pts',(10.0514428414941,74.8062499997113,-1.23094673026484E-15));
#298973=CARTESIAN_POINT('Ctrl Pts',(10.0514428414941,74.9562499997106,-3.26591175476071));
#298974=CARTESIAN_POINT('Ctrl Pts',(8.13178807675713,75.10624999971,-5.90808986649102));
#298975=CARTESIAN_POINT('Ctrl Pts',(6.21213331202016,75.2562499997094,-8.55026797822134));
#298976=CARTESIAN_POINT('Ctrl Pts',(3.10606665601005,75.4062499997088,-9.5594902125713));
#298977=CARTESIAN_POINT('Ctrl Pts',(-5.66378482980338E-14,75.5562499997083,
-10.5687124469213));
#298978=CARTESIAN_POINT('Ctrl Pts',(-3.10606665601016,75.7062499997077,
-9.5594902125713));
#298979=CARTESIAN_POINT('Ctrl Pts',(-6.21213331202027,75.856249999707,-8.55026797822134));
#298980=CARTESIAN_POINT('Ctrl Pts',(-8.13178807675725,76.0062499997065,
-5.90808986649102));
#298981=CARTESIAN_POINT('Ctrl Pts',(-10.0514428414942,76.1562499997058,
-3.2659117547607));
#298982=CARTESIAN_POINT('Ctrl Pts',(-10.0514428414942,76.3062499997052,
2.46189346052968E-15));
#298983=CARTESIAN_POINT('Ctrl Pts',(-10.0514428414942,76.4562499997046,
3.26591175476071));
#298984=CARTESIAN_POINT('Ctrl Pts',(-8.13178807675725,76.606249999704,5.90808986649102));
#298985=CARTESIAN_POINT('Ctrl Pts',(-6.21213331202027,76.7562499997035,
8.55026797822134));
#298986=CARTESIAN_POINT('Ctrl Pts',(-3.10606665601016,76.9062499997029,
9.5594902125713));
#298987=CARTESIAN_POINT('Ctrl Pts',(-5.49131149600185E-14,77.0562499997022,
10.5687124469213));
#298988=CARTESIAN_POINT('Ctrl Pts',(3.10606665601005,77.2062499997016,9.5594902125713));
#298989=CARTESIAN_POINT('Ctrl Pts',(6.21213331202016,77.356249999701,8.55026797822134));
#298990=CARTESIAN_POINT('Ctrl Pts',(8.13178807675713,77.5062499997004,5.90808986649102));
#298991=CARTESIAN_POINT('Ctrl Pts',(10.0514428414941,77.6562499996998,3.2659117547607));
#298992=CARTESIAN_POINT('Ctrl Pts',(10.0514428414941,77.8062499996992,-1.23094673026484E-15));
#298993=CARTESIAN_POINT('Ctrl Pts',(10.0514428414941,77.9562499996987,-3.26591175476071));
#298994=CARTESIAN_POINT('Ctrl Pts',(8.13178807675713,78.1062499996981,-5.90808986649102));
#298995=CARTESIAN_POINT('Ctrl Pts',(6.21213331202016,78.2562499996974,-8.55026797822134));
#298996=CARTESIAN_POINT('Ctrl Pts',(3.10606665601005,78.4062499996969,-9.5594902125713));
#298997=CARTESIAN_POINT('Ctrl Pts',(-5.83655575696956E-14,78.5562499996963,
-10.5687124469213));
#298998=CARTESIAN_POINT('Ctrl Pts',(-3.10606665601017,78.7062499996957,
-9.5594902125713));
#298999=CARTESIAN_POINT('Ctrl Pts',(-6.21213331202028,78.8562499996951,
-8.55026797822134));
#299000=CARTESIAN_POINT('Ctrl Pts',(-8.13178807675725,79.0062499996944,
-5.90808986649102));
#299001=CARTESIAN_POINT('Ctrl Pts',(-10.0514428414942,79.1562499996939,
-3.2659117547607));
#299002=CARTESIAN_POINT('Ctrl Pts',(-10.0514428414942,79.3062499996932,
2.46189346052968E-15));
#299003=CARTESIAN_POINT('Ctrl Pts',(-10.0514428414942,79.4562499996926,
3.26591175476071));
#299004=CARTESIAN_POINT('Ctrl Pts',(-8.13178807675725,79.606249999692,5.90808986649102));
#299005=CARTESIAN_POINT('Ctrl Pts',(-6.21213331202027,79.7562499996915,
8.55026797822134));
#299006=CARTESIAN_POINT('Ctrl Pts',(-3.10606665601016,79.9062499996908,
9.5594902125713));
#299007=CARTESIAN_POINT('Ctrl Pts',(-5.66408242316803E-14,80.0562499996902,
10.5687124469213));
#299008=CARTESIAN_POINT('Ctrl Pts',(3.10606665601005,80.2062499996896,9.5594902125713));
#299009=CARTESIAN_POINT('Ctrl Pts',(6.21213331202016,80.356249999689,8.55026797822134));
#299010=CARTESIAN_POINT('Ctrl Pts',(8.13178807675713,80.5062499996884,5.90808986649102));
#299011=CARTESIAN_POINT('Ctrl Pts',(10.0514428414941,80.6562499996878,3.2659117547607));
#299012=CARTESIAN_POINT('Ctrl Pts',(10.0514428414941,80.8062499996873,-1.23094673026484E-15));
#299013=CARTESIAN_POINT('Ctrl Pts',(10.0514428414941,80.9562499996866,-3.26591175476071));
#299014=CARTESIAN_POINT('Ctrl Pts',(8.13178807675713,81.1062499996861,-5.90808986649102));
#299015=CARTESIAN_POINT('Ctrl Pts',(6.21213331202016,81.2562499996854,-8.55026797822134));
#299016=CARTESIAN_POINT('Ctrl Pts',(3.10606665601005,81.4062499996849,-9.5594902125713));
#299017=CARTESIAN_POINT('Ctrl Pts',(-6.00932668413574E-14,81.5562499996843,
-10.5687124469213));
#299018=CARTESIAN_POINT('Ctrl Pts',(-3.10606665601017,81.7062499996837,
-9.5594902125713));
#299019=CARTESIAN_POINT('Ctrl Pts',(-6.21213331202028,81.856249999683,-8.55026797822134));
#299020=CARTESIAN_POINT('Ctrl Pts',(-8.13178807675725,82.0062499996824,
-5.90808986649102));
#299021=CARTESIAN_POINT('Ctrl Pts',(-10.0514428414942,82.1562499996818,
-3.2659117547607));
#299022=CARTESIAN_POINT('Ctrl Pts',(-10.0514428414942,82.3062499996813,
2.46189346052968E-15));
#299023=CARTESIAN_POINT('Ctrl Pts',(-10.0514428414942,82.4562499996806,
3.26591175476071));
#299024=CARTESIAN_POINT('Ctrl Pts',(-8.13178807675725,82.60624999968,5.90808986649102));
#299025=CARTESIAN_POINT('Ctrl Pts',(-6.21213331202028,82.7562499996795,
8.55026797822134));
#299026=CARTESIAN_POINT('Ctrl Pts',(-3.10606665601017,82.9062499996789,
9.5594902125713));
#299027=CARTESIAN_POINT('Ctrl Pts',(-5.83685335033422E-14,83.0562499996782,
10.5687124469213));
#299028=CARTESIAN_POINT('Ctrl Pts',(3.10606665601005,83.2062499996776,9.5594902125713));
#299029=CARTESIAN_POINT('Ctrl Pts',(6.21213331202016,83.356249999677,8.55026797822134));
#299030=CARTESIAN_POINT('Ctrl Pts',(8.13178807675713,83.5062499996764,5.90808986649102));
#299031=CARTESIAN_POINT('Ctrl Pts',(10.0514428414941,83.6562499996759,3.2659117547607));
#299032=CARTESIAN_POINT('Ctrl Pts',(10.0514428414941,83.8062499996752,-1.23094673026484E-15));
#299033=CARTESIAN_POINT('Ctrl Pts',(10.0514428414941,83.9562499996747,-3.26591175476071));
#299034=CARTESIAN_POINT('Ctrl Pts',(8.13178807675713,84.106249999674,-5.90808986649102));
#299035=CARTESIAN_POINT('Ctrl Pts',(6.21213331202016,84.2562499996734,-8.55026797822134));
#299036=CARTESIAN_POINT('Ctrl Pts',(3.10606665601005,84.4062499996729,-9.5594902125713));
#299037=CARTESIAN_POINT('Ctrl Pts',(-6.18209761130193E-14,84.5562499996723,
-10.5687124469213));
#299038=CARTESIAN_POINT('Ctrl Pts',(-3.10606665601017,84.7062499996717,
-9.5594902125713));
#299039=CARTESIAN_POINT('Ctrl Pts',(-6.21213331202028,84.856249999671,-8.55026797822134));
#299040=CARTESIAN_POINT('Ctrl Pts',(-8.13178807675725,85.0062499996704,
-5.90808986649102));
#299041=CARTESIAN_POINT('Ctrl Pts',(-10.0514428414942,85.1562499996699,
-3.2659117547607));
#299042=CARTESIAN_POINT('Ctrl Pts',(-10.0514428414942,85.3062499996692,
2.46189346052968E-15));
#299043=CARTESIAN_POINT('Ctrl Pts',(-10.0514428414942,85.4562499996686,
3.26591175476071));
#299044=CARTESIAN_POINT('Ctrl Pts',(-8.13178807675725,85.606249999668,5.90808986649102));
#299045=CARTESIAN_POINT('Ctrl Pts',(-6.21213331202028,85.7562499996675,
8.55026797822134));
#299046=CARTESIAN_POINT('Ctrl Pts',(-3.10606665601017,85.9062499996669,
9.5594902125713));
#299047=CARTESIAN_POINT('Ctrl Pts',(-6.0096242775004E-14,86.0562499996662,
10.5687124469213));
#299048=CARTESIAN_POINT('Ctrl Pts',(3.10606665601005,86.2062499996657,9.5594902125713));
#299049=CARTESIAN_POINT('Ctrl Pts',(6.21213331202016,86.3562499996651,8.55026797822134));
#299050=CARTESIAN_POINT('Ctrl Pts',(8.13178807675713,86.5062499996644,5.90808986649102));
#299051=CARTESIAN_POINT('Ctrl Pts',(10.0514428414941,86.6562499996638,3.2659117547607));
#299052=CARTESIAN_POINT('Ctrl Pts',(10.0514428414941,86.8062499996633,-1.23094673026484E-15));
#299053=CARTESIAN_POINT('Ctrl Pts',(10.0514428414941,86.9562499996626,-3.26591175476071));
#299054=CARTESIAN_POINT('Ctrl Pts',(8.13178807675713,87.1062499996621,-5.90808986649102));
#299055=CARTESIAN_POINT('Ctrl Pts',(6.21213331202015,87.2562499996614,-8.55026797822134));
#299056=CARTESIAN_POINT('Ctrl Pts',(3.10606665601004,87.4062499996609,-9.5594902125713));
#299057=CARTESIAN_POINT('Ctrl Pts',(-6.35486853846811E-14,87.5562499996603,
-10.5687124469213));
#299058=CARTESIAN_POINT('Ctrl Pts',(-3.10606665601017,87.7062499996597,
-9.5594902125713));
#299059=CARTESIAN_POINT('Ctrl Pts',(-6.21213331202028,87.856249999659,-8.55026797822134));
#299060=CARTESIAN_POINT('Ctrl Pts',(-8.13178807675726,88.0062499996585,
-5.90808986649102));
#299061=CARTESIAN_POINT('Ctrl Pts',(-10.0514428414942,88.1562499996578,
-3.2659117547607));
#299062=CARTESIAN_POINT('Ctrl Pts',(-10.0514428414942,88.3062499996572,
2.46189346052968E-15));
#299063=CARTESIAN_POINT('Ctrl Pts',(-10.0514428414942,88.4562499996566,
3.26591175476071));
#299064=CARTESIAN_POINT('Ctrl Pts',(-8.13178807675726,88.6062499996561,
5.90808986649102));
#299065=CARTESIAN_POINT('Ctrl Pts',(-6.21213331202028,88.7562499996555,
8.55026797822134));
#299066=CARTESIAN_POINT('Ctrl Pts',(-3.10606665601017,88.9062499996548,
9.5594902125713));
#299067=CARTESIAN_POINT('Ctrl Pts',(-6.18239520466659E-14,89.0562499996542,
10.5687124469213));
#299068=CARTESIAN_POINT('Ctrl Pts',(3.10606665601005,89.2062499996537,9.5594902125713));
#299069=CARTESIAN_POINT('Ctrl Pts',(6.21213331202016,89.3562499996531,8.55026797822134));
#299070=CARTESIAN_POINT('Ctrl Pts',(8.13178807675713,89.5062499996525,5.90808986649102));
#299071=CARTESIAN_POINT('Ctrl Pts',(10.0514428414941,89.6562499996518,3.2659117547607));
#299072=CARTESIAN_POINT('Ctrl Pts',(10.0514428414941,89.8062499996512,-1.23094673026484E-15));
#299073=CARTESIAN_POINT('Ctrl Pts',(10.0514428414941,89.9562499996507,-3.26591175476071));
#299074=CARTESIAN_POINT('Ctrl Pts',(8.13178807675713,90.10624999965,-5.90808986649102));
#299075=CARTESIAN_POINT('Ctrl Pts',(6.21213331202015,90.2562499996494,-8.55026797822134));
#299076=CARTESIAN_POINT('Ctrl Pts',(3.10606665601004,90.4062499996488,-9.5594902125713));
#299077=CARTESIAN_POINT('Ctrl Pts',(-6.52763946563429E-14,90.5562499996483,
-10.5687124469213));
#299078=CARTESIAN_POINT('Ctrl Pts',(-3.10606665601017,90.7062499996476,
-9.5594902125713));
#299079=CARTESIAN_POINT('Ctrl Pts',(-6.21213331202028,90.856249999647,-8.55026797822134));
#299080=CARTESIAN_POINT('Ctrl Pts',(-8.13178807675726,91.0062499996464,
-5.90808986649102));
#299081=CARTESIAN_POINT('Ctrl Pts',(-10.0514428414942,91.1562499996458,
-3.2659117547607));
#299082=CARTESIAN_POINT('Ctrl Pts',(-10.0514428414942,91.3062499996452,
2.46189346052968E-15));
#299083=CARTESIAN_POINT('Ctrl Pts',(-10.0514428414942,91.4562499996446,
3.26591175476071));
#299084=CARTESIAN_POINT('Ctrl Pts',(-8.13178807675726,91.606249999644,5.90808986649102));
#299085=CARTESIAN_POINT('Ctrl Pts',(-6.21213331202028,91.7562499996434,
8.55026797822134));
#299086=CARTESIAN_POINT('Ctrl Pts',(-3.10606665601017,91.9062499996429,
9.5594902125713));
#299087=CARTESIAN_POINT('Ctrl Pts',(-6.35516613183277E-14,92.0562499996422,
10.5687124469213));
#299088=CARTESIAN_POINT('Ctrl Pts',(3.10606665601004,92.2062499996417,9.5594902125713));
#299089=CARTESIAN_POINT('Ctrl Pts',(6.21213331202015,92.3562499996411,8.55026797822134));
#299090=CARTESIAN_POINT('Ctrl Pts',(8.13178807675712,92.5062499996404,5.90808986649102));
#299091=CARTESIAN_POINT('Ctrl Pts',(10.0514428414941,92.6562499996398,3.2659117547607));
#299092=CARTESIAN_POINT('Ctrl Pts',(10.0514428414941,92.8062499996392,-1.23094673026484E-15));
#299093=CARTESIAN_POINT('Ctrl Pts',(10.0514428414941,92.9562499996387,-3.26591175476071));
#299094=CARTESIAN_POINT('Ctrl Pts',(8.13178807675712,93.1062499996381,-5.90808986649102));
#299095=CARTESIAN_POINT('Ctrl Pts',(6.21213331202015,93.2562499996374,-8.55026797822134));
#299096=CARTESIAN_POINT('Ctrl Pts',(3.10606665601004,93.4062499996369,-9.5594902125713));
#299097=CARTESIAN_POINT('Ctrl Pts',(-6.70041039280048E-14,93.5562499996362,
-10.5687124469213));
#299098=CARTESIAN_POINT('Ctrl Pts',(-3.10606665601018,93.7062499996357,
-9.5594902125713));
#299099=CARTESIAN_POINT('Ctrl Pts',(-6.21213331202028,93.856249999635,-8.55026797822134));
#299100=CARTESIAN_POINT('Ctrl Pts',(-8.13178807675726,94.0062499996344,
-5.90808986649102));
#299101=CARTESIAN_POINT('Ctrl Pts',(-10.0514428414942,94.1562499996338,
-3.2659117547607));
#299102=CARTESIAN_POINT('Ctrl Pts',(-10.0514428414942,94.3062499996333,
2.46189346052968E-15));
#299103=CARTESIAN_POINT('Ctrl Pts',(-10.0514428414942,94.4562499996326,
3.26591175476071));
#299104=CARTESIAN_POINT('Ctrl Pts',(-8.13178807675726,94.606249999632,5.90808986649102));
#299105=CARTESIAN_POINT('Ctrl Pts',(-6.21213331202028,94.7562499996315,
8.55026797822134));
#299106=CARTESIAN_POINT('Ctrl Pts',(-3.10606665601017,94.9062499996309,
9.5594902125713));
#299107=CARTESIAN_POINT('Ctrl Pts',(-6.52793705899895E-14,95.0562499996302,
10.5687124469213));
#299108=CARTESIAN_POINT('Ctrl Pts',(3.10606665601004,95.2062499996296,9.5594902125713));
#299109=CARTESIAN_POINT('Ctrl Pts',(6.21213331202015,95.3562499996291,8.55026797822134));
#299110=CARTESIAN_POINT('Ctrl Pts',(8.13178807675712,95.5062499996285,5.90808986649102));
#299111=CARTESIAN_POINT('Ctrl Pts',(10.0514428414941,95.6562499996278,3.2659117547607));
#299112=CARTESIAN_POINT('Ctrl Pts',(10.0514428414941,95.8062499996273,-1.23094673026484E-15));
#299113=CARTESIAN_POINT('Ctrl Pts',(10.0514428414941,95.9562499996266,-3.26591175476071));
#299114=CARTESIAN_POINT('Ctrl Pts',(8.13178807675712,96.1062499996261,-5.90808986649102));
#299115=CARTESIAN_POINT('Ctrl Pts',(6.21213331202015,96.2562499996255,-8.55026797822134));
#299116=CARTESIAN_POINT('Ctrl Pts',(3.10606665601004,96.4062499996248,-9.5594902125713));
#299117=CARTESIAN_POINT('Ctrl Pts',(-6.87318131996666E-14,96.5562499996243,
-10.5687124469213));
#299118=CARTESIAN_POINT('Ctrl Pts',(-3.10606665601018,96.7062499996236,
-9.5594902125713));
#299119=CARTESIAN_POINT('Ctrl Pts',(-6.21213331202028,96.856249999623,-8.55026797822134));
#299120=CARTESIAN_POINT('Ctrl Pts',(-8.13178807675726,97.0062499996224,
-5.90808986649102));
#299121=CARTESIAN_POINT('Ctrl Pts',(-10.0514428414942,97.1562499996218,
-3.2659117547607));
#299122=CARTESIAN_POINT('Ctrl Pts',(-10.0514428414942,97.3062499996212,
2.46189346052968E-15));
#299123=CARTESIAN_POINT('Ctrl Pts',(-10.0514428414942,97.4562499996206,
3.26591175476071));
#299124=CARTESIAN_POINT('Ctrl Pts',(-8.13178807675726,97.60624999962,5.90808986649102));
#299125=CARTESIAN_POINT('Ctrl Pts',(-6.21213331202028,97.7562499996195,
8.55026797822134));
#299126=CARTESIAN_POINT('Ctrl Pts',(-3.10606665601018,97.9062499996189,
9.5594902125713));
#299127=CARTESIAN_POINT('Ctrl Pts',(-6.70070798616514E-14,98.0562499996182,
10.5687124469213));
#299128=CARTESIAN_POINT('Ctrl Pts',(3.10606665601004,98.2062499996177,9.5594902125713));
#299129=CARTESIAN_POINT('Ctrl Pts',(6.21213331202015,98.3562499996171,8.55026797822134));
#299130=CARTESIAN_POINT('Ctrl Pts',(8.13178807675712,98.5062499996165,5.90808986649102));
#299131=CARTESIAN_POINT('Ctrl Pts',(10.0514428414941,98.6562499996158,3.2659117547607));
#299132=CARTESIAN_POINT('Ctrl Pts',(10.0514428414941,98.8062499996153,-1.23094673026484E-15));
#299133=CARTESIAN_POINT('Ctrl Pts',(10.0514428414941,98.9562499996147,-3.26591175476071));
#299134=CARTESIAN_POINT('Ctrl Pts',(8.13178807675712,99.1062499996141,-5.90808986649102));
#299135=CARTESIAN_POINT('Ctrl Pts',(6.21213331202015,99.2562499996134,-8.55026797822134));
#299136=CARTESIAN_POINT('Ctrl Pts',(3.10606665601004,99.4062499996129,-9.5594902125713));
#299137=CARTESIAN_POINT('Ctrl Pts',(-7.04595224713284E-14,99.5562499996123,
-10.5687124469213));
#299138=CARTESIAN_POINT('Ctrl Pts',(-3.10606665601018,99.7062499996117,
-9.5594902125713));
#299139=CARTESIAN_POINT('Ctrl Pts',(-6.21213331202028,99.856249999611,-8.55026797822134));
#299140=CARTESIAN_POINT('Ctrl Pts',(-8.13178807675726,100.00624999961,-5.90808986649102));
#299141=CARTESIAN_POINT('Ctrl Pts',(-10.0514428414942,100.15624999961,-3.2659117547607));
#299142=CARTESIAN_POINT('Ctrl Pts',(-10.0514428414942,100.306249999609,
2.46189346052968E-15));
#299143=CARTESIAN_POINT('Ctrl Pts',(-10.0514428414942,100.456249999609,
3.26591175476071));
#299144=CARTESIAN_POINT('Ctrl Pts',(-8.13178807675726,100.606249999608,
5.90808986649102));
#299145=CARTESIAN_POINT('Ctrl Pts',(-6.21213331202028,100.756249999607,
8.55026797822134));
#299146=CARTESIAN_POINT('Ctrl Pts',(-3.10606665601018,100.906249999607,
9.5594902125713));
#299147=CARTESIAN_POINT('Ctrl Pts',(-6.87347891333132E-14,101.056249999606,
10.5687124469213));
#299148=CARTESIAN_POINT('Ctrl Pts',(3.10606665601004,101.206249999606,9.5594902125713));
#299149=CARTESIAN_POINT('Ctrl Pts',(6.21213331202015,101.356249999605,8.55026797822134));
#299150=CARTESIAN_POINT('Ctrl Pts',(8.13178807675712,101.506249999604,5.90808986649102));
#299151=CARTESIAN_POINT('Ctrl Pts',(10.0514428414941,101.656249999604,3.2659117547607));
#299152=CARTESIAN_POINT('Ctrl Pts',(10.0514428414941,101.806249999603,-1.23094673026484E-15));
#299153=CARTESIAN_POINT('Ctrl Pts',(10.0514428414941,101.956249999603,-3.26591175476071));
#299154=CARTESIAN_POINT('Ctrl Pts',(8.13178807675712,102.106249999602,-5.90808986649102));
#299155=CARTESIAN_POINT('Ctrl Pts',(6.21213331202014,102.256249999601,-8.55026797822134));
#299156=CARTESIAN_POINT('Ctrl Pts',(3.10606665601004,102.406249999601,-9.5594902125713));
#299157=CARTESIAN_POINT('Ctrl Pts',(-7.21872317429903E-14,102.5562499996,
-10.5687124469213));
#299158=CARTESIAN_POINT('Ctrl Pts',(-3.10606665601018,102.7062499996,-9.5594902125713));
#299159=CARTESIAN_POINT('Ctrl Pts',(-6.21213331202029,102.856249999599,
-8.55026797822134));
#299160=CARTESIAN_POINT('Ctrl Pts',(-8.13178807675726,103.006249999598,
-5.90808986649102));
#299161=CARTESIAN_POINT('Ctrl Pts',(-10.0514428414942,103.156249999598,
-3.2659117547607));
#299162=CARTESIAN_POINT('Ctrl Pts',(-10.0514428414942,103.306249999597,
2.46189346052968E-15));
#299163=CARTESIAN_POINT('Ctrl Pts',(-10.0514428414942,103.456249999597,
3.26591175476071));
#299164=CARTESIAN_POINT('Ctrl Pts',(-8.13178807675726,103.606249999596,
5.90808986649102));
#299165=CARTESIAN_POINT('Ctrl Pts',(-6.21213331202028,103.756249999595,
8.55026797822134));
#299166=CARTESIAN_POINT('Ctrl Pts',(-3.10606665601018,103.906249999595,
9.5594902125713));
#299167=CARTESIAN_POINT('Ctrl Pts',(-7.04624984049751E-14,104.056249999594,
10.5687124469213));
#299168=CARTESIAN_POINT('Ctrl Pts',(3.10606665601004,104.206249999594,9.5594902125713));
#299169=CARTESIAN_POINT('Ctrl Pts',(6.21213331202015,104.356249999593,8.55026797822134));
#299170=CARTESIAN_POINT('Ctrl Pts',(8.13178807675712,104.506249999592,5.90808986649102));
#299171=CARTESIAN_POINT('Ctrl Pts',(10.0514428414941,104.656249999592,3.2659117547607));
#299172=CARTESIAN_POINT('Ctrl Pts',(10.0514428414941,104.806249999591,-1.23094673026484E-15));
#299173=CARTESIAN_POINT('Ctrl Pts',(10.0514428414941,104.956249999591,-3.26591175476071));
#299174=CARTESIAN_POINT('Ctrl Pts',(8.13178807675712,105.10624999959,-5.90808986649102));
#299175=CARTESIAN_POINT('Ctrl Pts',(6.21213331202014,105.256249999589,-8.55026797822134));
#299176=CARTESIAN_POINT('Ctrl Pts',(3.10606665601003,105.406249999589,-9.5594902125713));
#299177=CARTESIAN_POINT('Ctrl Pts',(-7.39149410146522E-14,105.556249999588,
-10.5687124469213));
#299178=CARTESIAN_POINT('Ctrl Pts',(-3.10606665601018,105.706249999588,
-9.5594902125713));
#299179=CARTESIAN_POINT('Ctrl Pts',(-6.21213331202029,105.856249999587,
-8.55026797822134));
#299180=CARTESIAN_POINT('Ctrl Pts',(-8.13178807675726,106.006249999586,
-5.90808986649102));
#299181=CARTESIAN_POINT('Ctrl Pts',(-10.0514428414942,106.156249999586,
-3.2659117547607));
#299182=CARTESIAN_POINT('Ctrl Pts',(-10.0514428414942,106.306249999585,
2.46189346052968E-15));
#299183=CARTESIAN_POINT('Ctrl Pts',(-10.0514428414942,106.456249999585,
3.26591175476071));
#299184=CARTESIAN_POINT('Ctrl Pts',(-8.13178807675726,106.606249999584,
5.90808986649102));
#299185=CARTESIAN_POINT('Ctrl Pts',(-6.21213331202029,106.756249999583,
8.55026797822134));
#299186=CARTESIAN_POINT('Ctrl Pts',(-3.10606665601018,106.906249999583,
9.5594902125713));
#299187=CARTESIAN_POINT('Ctrl Pts',(-7.21902076766369E-14,107.056249999582,
10.5687124469213));
#299188=CARTESIAN_POINT('Ctrl Pts',(3.10606665601003,107.206249999582,9.5594902125713));
#299189=CARTESIAN_POINT('Ctrl Pts',(6.21213331202014,107.356249999581,8.55026797822134));
#299190=CARTESIAN_POINT('Ctrl Pts',(8.13178807675711,107.50624999958,5.90808986649102));
#299191=CARTESIAN_POINT('Ctrl Pts',(10.0514428414941,107.65624999958,3.2659117547607));
#299192=CARTESIAN_POINT('Ctrl Pts',(10.0514428414941,107.806249999579,-1.23094673026484E-15));
#299193=CARTESIAN_POINT('Ctrl Pts',(10.0514428414941,107.956249999579,-3.26591175476071));
#299194=CARTESIAN_POINT('Ctrl Pts',(8.13178807675711,108.106249999578,-5.90808986649102));
#299195=CARTESIAN_POINT('Ctrl Pts',(6.21213331202014,108.256249999577,-8.55026797822134));
#299196=CARTESIAN_POINT('Ctrl Pts',(3.10606665601003,108.406249999577,-9.5594902125713));
#299197=CARTESIAN_POINT('Ctrl Pts',(-7.5642650286314E-14,108.556249999576,
-10.5687124469213));
#299198=CARTESIAN_POINT('Ctrl Pts',(-3.10606665601018,108.706249999576,
-9.5594902125713));
#299199=CARTESIAN_POINT('Ctrl Pts',(-6.21213331202029,108.856249999575,
-8.55026797822134));
#299200=CARTESIAN_POINT('Ctrl Pts',(-8.13178807675727,109.006249999574,
-5.90808986649102));
#299201=CARTESIAN_POINT('Ctrl Pts',(-10.0514428414942,109.156249999574,
-3.2659117547607));
#299202=CARTESIAN_POINT('Ctrl Pts',(-10.0514428414942,109.306249999573,
2.46189346052968E-15));
#299203=CARTESIAN_POINT('Ctrl Pts',(-10.0514428414942,109.456249999573,
3.26591175476071));
#299204=CARTESIAN_POINT('Ctrl Pts',(-8.13178807675727,109.606249999572,
5.90808986649102));
#299205=CARTESIAN_POINT('Ctrl Pts',(-6.21213331202029,109.756249999571,
8.55026797822134));
#299206=CARTESIAN_POINT('Ctrl Pts',(-3.10606665601018,109.906249999571,
9.5594902125713));
#299207=CARTESIAN_POINT('Ctrl Pts',(-7.39179169482987E-14,110.05624999957,
10.5687124469213));
#299208=CARTESIAN_POINT('Ctrl Pts',(3.10606665601003,110.20624999957,9.5594902125713));
#299209=CARTESIAN_POINT('Ctrl Pts',(6.21213331202014,110.356249999569,8.55026797822134));
#299210=CARTESIAN_POINT('Ctrl Pts',(8.13178807675711,110.506249999568,5.90808986649102));
#299211=CARTESIAN_POINT('Ctrl Pts',(10.0514428414941,110.656249999568,3.2659117547607));
#299212=CARTESIAN_POINT('Ctrl Pts',(10.0514428414941,110.806249999567,-1.23094673026484E-15));
#299213=CARTESIAN_POINT('Ctrl Pts',(10.0514428414941,110.956249999567,-3.26591175476071));
#299214=CARTESIAN_POINT('Ctrl Pts',(8.13178807675711,111.106249999566,-5.90808986649102));
#299215=CARTESIAN_POINT('Ctrl Pts',(6.21213331202014,111.256249999565,-8.55026797822134));
#299216=CARTESIAN_POINT('Ctrl Pts',(3.10606665601003,111.406249999565,-9.5594902125713));
#299217=CARTESIAN_POINT('Ctrl Pts',(-7.73703595579758E-14,111.556249999564,
-10.5687124469213));
#299218=CARTESIAN_POINT('Ctrl Pts',(-3.10606665601019,111.706249999564,
-9.5594902125713));
#299219=CARTESIAN_POINT('Ctrl Pts',(-6.21213331202029,111.856249999563,
-8.55026797822134));
#299220=CARTESIAN_POINT('Ctrl Pts',(-8.13178807675727,112.006249999562,
-5.90808986649102));
#299221=CARTESIAN_POINT('Ctrl Pts',(-10.0514428414942,112.156249999562,
-3.2659117547607));
#299222=CARTESIAN_POINT('Ctrl Pts',(-10.0514428414942,112.306249999561,
2.46189346052968E-15));
#299223=CARTESIAN_POINT('Ctrl Pts',(-10.0514428414942,112.456249999561,
3.26591175476071));
#299224=CARTESIAN_POINT('Ctrl Pts',(-8.13178807675727,112.60624999956,5.90808986649102));
#299225=CARTESIAN_POINT('Ctrl Pts',(-6.21213331202029,112.756249999559,
8.55026797822134));
#299226=CARTESIAN_POINT('Ctrl Pts',(-3.10606665601018,112.906249999559,
9.5594902125713));
#299227=CARTESIAN_POINT('Ctrl Pts',(-7.56456262199606E-14,113.056249999558,
10.5687124469213));
#299228=CARTESIAN_POINT('Ctrl Pts',(3.10606665601003,113.206249999558,9.5594902125713));
#299229=CARTESIAN_POINT('Ctrl Pts',(6.21213331202014,113.356249999557,8.55026797822134));
#299230=CARTESIAN_POINT('Ctrl Pts',(8.13178807675711,113.506249999556,5.90808986649102));
#299231=CARTESIAN_POINT('Ctrl Pts',(10.0514428414941,113.656249999556,3.2659117547607));
#299232=CARTESIAN_POINT('Ctrl Pts',(10.0514428414941,113.806249999555,-1.23094673026484E-15));
#299233=CARTESIAN_POINT('Ctrl Pts',(10.0514428414941,113.956249999555,-3.26591175476071));
#299234=CARTESIAN_POINT('Ctrl Pts',(8.13178807675711,114.106249999554,-5.90808986649102));
#299235=CARTESIAN_POINT('Ctrl Pts',(6.21213331202014,114.256249999553,-8.55026797822134));
#299236=CARTESIAN_POINT('Ctrl Pts',(3.10606665601003,114.406249999553,-9.5594902125713));
#299237=CARTESIAN_POINT('Ctrl Pts',(-7.90980688296377E-14,114.556249999552,
-10.5687124469213));
#299238=CARTESIAN_POINT('Ctrl Pts',(-3.10606665601019,114.706249999552,
-9.5594902125713));
#299239=CARTESIAN_POINT('Ctrl Pts',(-6.2121333120203,114.856249999551,-8.55026797822134));
#299240=CARTESIAN_POINT('Ctrl Pts',(-8.13178807675727,115.00624999955,-5.90808986649102));
#299241=CARTESIAN_POINT('Ctrl Pts',(-10.0514428414942,115.15624999955,-3.2659117547607));
#299242=CARTESIAN_POINT('Ctrl Pts',(-10.0514428414942,115.306249999549,
2.46189346052968E-15));
#299243=CARTESIAN_POINT('Ctrl Pts',(-10.0514428414942,115.456249999549,
3.26591175476071));
#299244=CARTESIAN_POINT('Ctrl Pts',(-8.13178807675727,115.606249999548,
5.90808986649102));
#299245=CARTESIAN_POINT('Ctrl Pts',(-6.21213331202029,115.756249999547,
8.55026797822134));
#299246=CARTESIAN_POINT('Ctrl Pts',(-3.10606665601019,115.906249999547,
9.5594902125713));
#299247=CARTESIAN_POINT('Ctrl Pts',(-7.73733354916224E-14,116.056249999546,
10.5687124469213));
#299248=CARTESIAN_POINT('Ctrl Pts',(3.10606665601003,116.206249999546,9.5594902125713));
#299249=CARTESIAN_POINT('Ctrl Pts',(6.21213331202014,116.356249999545,8.55026797822134));
#299250=CARTESIAN_POINT('Ctrl Pts',(8.13178807675711,116.506249999544,5.90808986649102));
#299251=CARTESIAN_POINT('Ctrl Pts',(10.0514428414941,116.656249999544,3.2659117547607));
#299252=CARTESIAN_POINT('Ctrl Pts',(10.0514428414941,116.806249999543,-1.23094673026484E-15));
#299253=CARTESIAN_POINT('Ctrl Pts',(10.0514428414941,116.956249999543,-3.26591175476071));
#299254=CARTESIAN_POINT('Ctrl Pts',(8.13178807675711,117.106249999542,-5.90808986649102));
#299255=CARTESIAN_POINT('Ctrl Pts',(6.21213331202014,117.256249999541,-8.55026797822134));
#299256=CARTESIAN_POINT('Ctrl Pts',(3.10606665601003,117.406249999541,-9.5594902125713));
#299257=CARTESIAN_POINT('Ctrl Pts',(-8.08257781012995E-14,117.55624999954,
-10.5687124469213));
#299258=CARTESIAN_POINT('Ctrl Pts',(-3.10606665601019,117.70624999954,-9.5594902125713));
#299259=CARTESIAN_POINT('Ctrl Pts',(-6.2121333120203,117.856249999539,-8.55026797822134));
#299260=CARTESIAN_POINT('Ctrl Pts',(-8.13178807675727,118.006249999538,
-5.90808986649102));
#299261=CARTESIAN_POINT('Ctrl Pts',(-10.0514428414942,118.156249999538,
-3.2659117547607));
#299262=CARTESIAN_POINT('Ctrl Pts',(-10.0514428414942,118.306249999537,
2.46189346052968E-15));
#299263=CARTESIAN_POINT('Ctrl Pts',(-10.0514428414942,118.456249999537,
3.26591175476071));
#299264=CARTESIAN_POINT('Ctrl Pts',(-8.13178807675727,118.606249999536,
5.90808986649102));
#299265=CARTESIAN_POINT('Ctrl Pts',(-6.2121333120203,118.756249999535,8.55026797822134));
#299266=CARTESIAN_POINT('Ctrl Pts',(-3.10606665601019,118.906249999535,
9.5594902125713));
#299267=CARTESIAN_POINT('Ctrl Pts',(-7.91010447632842E-14,119.056249999534,
10.5687124469213));
#299268=CARTESIAN_POINT('Ctrl Pts',(3.10606665601003,119.206249999534,9.5594902125713));
#299269=CARTESIAN_POINT('Ctrl Pts',(6.21213331202014,119.356249999533,8.55026797822134));
#299270=CARTESIAN_POINT('Ctrl Pts',(8.13178807675711,119.506249999532,5.90808986649102));
#299271=CARTESIAN_POINT('Ctrl Pts',(10.0514428414941,119.656249999532,3.2659117547607));
#299272=CARTESIAN_POINT('Ctrl Pts',(10.0514428414941,119.806249999531,-1.23094673026484E-15));
#299273=CARTESIAN_POINT('Ctrl Pts',(10.0514428414941,119.956249999531,-3.26591175476071));
#299274=CARTESIAN_POINT('Ctrl Pts',(8.13178807675711,120.10624999953,-5.90808986649102));
#299275=CARTESIAN_POINT('Ctrl Pts',(6.21213331202013,120.256249999529,-8.55026797822134));
#299276=CARTESIAN_POINT('Ctrl Pts',(3.10606665601003,120.406249999529,-9.5594902125713));
#299277=CARTESIAN_POINT('Ctrl Pts',(-8.25534873729613E-14,120.556249999528,
-10.5687124469213));
#299278=CARTESIAN_POINT('Ctrl Pts',(-3.10606665601019,120.706249999528,
-9.5594902125713));
#299279=CARTESIAN_POINT('Ctrl Pts',(-6.2121333120203,120.856249999527,-8.55026797822134));
#299280=CARTESIAN_POINT('Ctrl Pts',(-8.13178807675727,121.006249999526,
-5.90808986649102));
#299281=CARTESIAN_POINT('Ctrl Pts',(-10.0514428414943,121.156249999526,
-3.2659117547607));
#299282=CARTESIAN_POINT('Ctrl Pts',(-10.0514428414943,121.306249999525,
2.46189346052968E-15));
#299283=CARTESIAN_POINT('Ctrl Pts',(-10.0514428414943,121.456249999525,
3.26591175476071));
#299284=CARTESIAN_POINT('Ctrl Pts',(-8.13178807675727,121.606249999524,
5.90808986649102));
#299285=CARTESIAN_POINT('Ctrl Pts',(-6.2121333120203,121.756249999523,8.55026797822134));
#299286=CARTESIAN_POINT('Ctrl Pts',(-3.10606665601019,121.906249999523,
9.5594902125713));
#299287=CARTESIAN_POINT('Ctrl Pts',(-8.08287540349461E-14,122.056249999522,
10.5687124469213));
#299288=CARTESIAN_POINT('Ctrl Pts',(3.10606665601003,122.206249999522,9.5594902125713));
#299289=CARTESIAN_POINT('Ctrl Pts',(6.21213331202014,122.356249999521,8.55026797822134));
#299290=CARTESIAN_POINT('Ctrl Pts',(8.13178807675711,122.50624999952,5.90808986649102));
#299291=CARTESIAN_POINT('Ctrl Pts',(10.0514428414941,122.65624999952,3.2659117547607));
#299292=CARTESIAN_POINT('Ctrl Pts',(10.0514428414941,122.806249999519,-1.23094673026484E-15));
#299293=CARTESIAN_POINT('Ctrl Pts',(10.0514428414941,122.956249999519,-3.26591175476071));
#299294=CARTESIAN_POINT('Ctrl Pts',(8.13178807675711,123.106249999518,-5.90808986649102));
#299295=CARTESIAN_POINT('Ctrl Pts',(6.21213331202013,123.256249999517,-8.55026797822134));
#299296=CARTESIAN_POINT('Ctrl Pts',(3.10606665601002,123.406249999517,-9.5594902125713));
#299297=CARTESIAN_POINT('Ctrl Pts',(-8.42811966446232E-14,123.556249999516,
-10.5687124469213));
#299298=CARTESIAN_POINT('Ctrl Pts',(-3.10606665601019,123.706249999516,
-9.5594902125713));
#299299=CARTESIAN_POINT('Ctrl Pts',(-6.2121333120203,123.856249999515,-8.55026797822134));
#299300=CARTESIAN_POINT('Ctrl Pts',(-8.13178807675727,124.006249999514,
-5.90808986649102));
#299301=CARTESIAN_POINT('Ctrl Pts',(-10.0514428414943,124.156249999514,
-3.2659117547607));
#299302=CARTESIAN_POINT('Ctrl Pts',(-10.0514428414943,124.306249999513,
2.46189346052968E-15));
#299303=CARTESIAN_POINT('Ctrl Pts',(-10.0514428414943,124.456249999513,
3.26591175476071));
#299304=CARTESIAN_POINT('Ctrl Pts',(-8.13178807675727,124.606249999512,
5.90808986649102));
#299305=CARTESIAN_POINT('Ctrl Pts',(-6.2121333120203,124.756249999511,8.55026797822134));
#299306=CARTESIAN_POINT('Ctrl Pts',(-3.10606665601019,124.906249999511,
9.5594902125713));
#299307=CARTESIAN_POINT('Ctrl Pts',(-8.25564633066079E-14,125.05624999951,
10.5687124469213));
#299308=CARTESIAN_POINT('Ctrl Pts',(3.10606665601002,125.20624999951,9.5594902125713));
#299309=CARTESIAN_POINT('Ctrl Pts',(6.21213331202013,125.356249999509,8.55026797822134));
#299310=CARTESIAN_POINT('Ctrl Pts',(8.13178807675711,125.506249999508,5.90808986649102));
#299311=CARTESIAN_POINT('Ctrl Pts',(10.0514428414941,125.656249999508,3.2659117547607));
#299312=CARTESIAN_POINT('Ctrl Pts',(10.0514428414941,125.806249999507,-1.23094673026484E-15));
#299313=CARTESIAN_POINT('Ctrl Pts',(10.0514428414941,125.956249999507,-3.26591175476071));
#299314=CARTESIAN_POINT('Ctrl Pts',(8.13178807675711,126.106249999506,-5.90808986649102));
#299315=CARTESIAN_POINT('Ctrl Pts',(6.21213331202013,126.256249999505,-8.55026797822134));
#299316=CARTESIAN_POINT('Ctrl Pts',(3.10606665601002,126.406249999505,-9.5594902125713));
#299317=CARTESIAN_POINT('Ctrl Pts',(-8.6008905916285E-14,126.556249999504,
-10.5687124469213));
#299318=CARTESIAN_POINT('Ctrl Pts',(-3.10606665601019,126.706249999504,
-9.5594902125713));
#299319=CARTESIAN_POINT('Ctrl Pts',(-6.2121333120203,126.856249999503,-8.55026797822134));
#299320=CARTESIAN_POINT('Ctrl Pts',(-8.13178807675728,127.006249999502,
-5.90808986649102));
#299321=CARTESIAN_POINT('Ctrl Pts',(-10.0514428414943,127.156249999502,
-3.2659117547607));
#299322=CARTESIAN_POINT('Ctrl Pts',(-10.0514428414943,127.306249999501,
2.46189346052968E-15));
#299323=CARTESIAN_POINT('Ctrl Pts',(-10.0514428414943,127.456249999501,
3.26591175476071));
#299324=CARTESIAN_POINT('Ctrl Pts',(-8.13178807675728,127.6062499995,5.90808986649102));
#299325=CARTESIAN_POINT('Ctrl Pts',(-6.2121333120203,127.756249999499,8.55026797822134));
#299326=CARTESIAN_POINT('Ctrl Pts',(-3.10606665601019,127.906249999499,
9.5594902125713));
#299327=CARTESIAN_POINT('Ctrl Pts',(-8.42841725782698E-14,128.056249999498,
10.5687124469213));
#299328=CARTESIAN_POINT('Ctrl Pts',(3.10606665601002,128.206249999498,9.5594902125713));
#299329=CARTESIAN_POINT('Ctrl Pts',(6.21213331202013,128.356249999497,8.55026797822134));
#299330=CARTESIAN_POINT('Ctrl Pts',(8.1317880767571,128.506249999496,5.90808986649102));
#299331=CARTESIAN_POINT('Ctrl Pts',(10.0514428414941,128.656249999496,3.2659117547607));
#299332=CARTESIAN_POINT('Ctrl Pts',(10.0514428414941,128.806249999495,-1.23094673026484E-15));
#299333=CARTESIAN_POINT('Ctrl Pts',(10.0514428414941,128.956249999495,-3.26591175476071));
#299334=CARTESIAN_POINT('Ctrl Pts',(8.1317880767571,129.106249999494,-5.90808986649102));
#299335=CARTESIAN_POINT('Ctrl Pts',(6.21213331202013,129.256249999493,-8.55026797822134));
#299336=CARTESIAN_POINT('Ctrl Pts',(3.10606665601002,129.406249999493,-9.5594902125713));
#299337=CARTESIAN_POINT('Ctrl Pts',(-8.77366151879469E-14,129.556249999492,
-10.5687124469213));
#299338=CARTESIAN_POINT('Ctrl Pts',(-3.1060666560102,129.706249999492,-9.5594902125713));
#299339=CARTESIAN_POINT('Ctrl Pts',(-6.2121333120203,129.856249999491,-8.55026797822134));
#299340=CARTESIAN_POINT('Ctrl Pts',(-8.13178807675728,130.00624999949,-5.90808986649102));
#299341=CARTESIAN_POINT('Ctrl Pts',(-10.0514428414943,130.15624999949,-3.2659117547607));
#299342=CARTESIAN_POINT('Ctrl Pts',(-10.0514428414943,130.306249999489,
2.46189346052968E-15));
#299343=CARTESIAN_POINT('Ctrl Pts',(-10.0514428414943,130.456249999489,
3.26591175476071));
#299344=CARTESIAN_POINT('Ctrl Pts',(-8.13178807675728,130.606249999488,
5.90808986649102));
#299345=CARTESIAN_POINT('Ctrl Pts',(-6.2121333120203,130.756249999487,8.55026797822134));
#299346=CARTESIAN_POINT('Ctrl Pts',(-3.10606665601019,130.906249999487,
9.5594902125713));
#299347=CARTESIAN_POINT('Ctrl Pts',(-8.60118818499316E-14,131.056249999486,
10.5687124469213));
#299348=CARTESIAN_POINT('Ctrl Pts',(3.10606665601002,131.206249999486,9.5594902125713));
#299349=CARTESIAN_POINT('Ctrl Pts',(6.21213331202013,131.356249999485,8.55026797822134));
#299350=CARTESIAN_POINT('Ctrl Pts',(8.1317880767571,131.506249999484,5.90808986649102));
#299351=CARTESIAN_POINT('Ctrl Pts',(10.0514428414941,131.656249999484,3.2659117547607));
#299352=CARTESIAN_POINT('Ctrl Pts',(10.0514428414941,131.806249999483,-1.23094673026484E-15));
#299353=CARTESIAN_POINT('Ctrl Pts',(10.0514428414941,131.956249999483,-3.26591175476071));
#299354=CARTESIAN_POINT('Ctrl Pts',(8.1317880767571,132.106249999482,-5.90808986649102));
#299355=CARTESIAN_POINT('Ctrl Pts',(6.21213331202012,132.256249999481,-8.55026797822134));
#299356=CARTESIAN_POINT('Ctrl Pts',(3.10606665601002,132.406249999481,-9.5594902125713));
#299357=CARTESIAN_POINT('Ctrl Pts',(-8.94643244596087E-14,132.55624999948,
-10.5687124469213));
#299358=CARTESIAN_POINT('Ctrl Pts',(-3.1060666560102,132.70624999948,-9.5594902125713));
#299359=CARTESIAN_POINT('Ctrl Pts',(-6.2121333120203,132.856249999479,-8.55026797822134));
#299360=CARTESIAN_POINT('Ctrl Pts',(-8.13178807675728,133.006249999478,
-5.90808986649102));
#299361=CARTESIAN_POINT('Ctrl Pts',(-10.0514428414943,133.156249999478,
-3.2659117547607));
#299362=CARTESIAN_POINT('Ctrl Pts',(-10.0514428414943,133.306249999477,
2.46189346052968E-15));
#299363=CARTESIAN_POINT('Ctrl Pts',(-10.0514428414943,133.456249999477,
3.26591175476071));
#299364=CARTESIAN_POINT('Ctrl Pts',(-8.13178807675728,133.606249999476,
5.90808986649102));
#299365=CARTESIAN_POINT('Ctrl Pts',(-6.2121333120203,133.756249999475,8.55026797822134));
#299366=CARTESIAN_POINT('Ctrl Pts',(-3.1060666560102,133.906249999475,9.5594902125713));
#299367=CARTESIAN_POINT('Ctrl Pts',(-8.77395911215934E-14,134.056249999474,
10.5687124469213));
#299368=CARTESIAN_POINT('Ctrl Pts',(3.10606665601002,134.206249999474,9.5594902125713));
#299369=CARTESIAN_POINT('Ctrl Pts',(6.21213331202013,134.356249999473,8.55026797822134));
#299370=CARTESIAN_POINT('Ctrl Pts',(8.1317880767571,134.506249999472,5.90808986649102));
#299371=CARTESIAN_POINT('Ctrl Pts',(10.0514428414941,134.656249999472,3.2659117547607));
#299372=CARTESIAN_POINT('Ctrl Pts',(10.0514428414941,134.806249999471,-1.23094673026484E-15));
#299373=CARTESIAN_POINT('Ctrl Pts',(10.0514428414941,134.956249999471,-3.26591175476071));
#299374=CARTESIAN_POINT('Ctrl Pts',(8.1317880767571,135.10624999947,-5.90808986649102));
#299375=CARTESIAN_POINT('Ctrl Pts',(6.21213331202012,135.256249999469,-8.55026797822134));
#299376=CARTESIAN_POINT('Ctrl Pts',(3.10606665601002,135.406249999469,-9.5594902125713));
#299377=CARTESIAN_POINT('Ctrl Pts',(-9.11920337312706E-14,135.556249999468,
-10.5687124469213));
#299378=CARTESIAN_POINT('Ctrl Pts',(-3.1060666560102,135.706249999468,-9.5594902125713));
#299379=CARTESIAN_POINT('Ctrl Pts',(-6.21213331202031,135.856249999467,
-8.55026797822134));
#299380=CARTESIAN_POINT('Ctrl Pts',(-8.13178807675728,136.006249999466,
-5.90808986649102));
#299381=CARTESIAN_POINT('Ctrl Pts',(-10.0514428414943,136.156249999466,
-3.2659117547607));
#299382=CARTESIAN_POINT('Ctrl Pts',(-10.0514428414943,136.306249999465,
2.46189346052968E-15));
#299383=CARTESIAN_POINT('Ctrl Pts',(-10.0514428414943,136.456249999465,
3.26591175476071));
#299384=CARTESIAN_POINT('Ctrl Pts',(-8.13178807675728,136.606249999464,
5.90808986649102));
#299385=CARTESIAN_POINT('Ctrl Pts',(-6.2121333120203,136.756249999463,8.55026797822134));
#299386=CARTESIAN_POINT('Ctrl Pts',(-3.1060666560102,136.906249999463,9.5594902125713));
#299387=CARTESIAN_POINT('Ctrl Pts',(-8.94673003932553E-14,137.056249999462,
10.5687124469213));
#299388=CARTESIAN_POINT('Ctrl Pts',(3.10606665601002,137.206249999462,9.5594902125713));
#299389=CARTESIAN_POINT('Ctrl Pts',(6.21213331202012,137.356249999461,8.55026797822134));
#299390=CARTESIAN_POINT('Ctrl Pts',(8.1317880767571,137.50624999946,5.90808986649102));
#299391=CARTESIAN_POINT('Ctrl Pts',(10.0514428414941,137.65624999946,3.2659117547607));
#299392=CARTESIAN_POINT('Ctrl Pts',(10.0514428414941,137.806249999459,-1.23094673026484E-15));
#299393=CARTESIAN_POINT('Ctrl Pts',(10.0514428414941,137.956249999459,-3.26591175476071));
#299394=CARTESIAN_POINT('Ctrl Pts',(8.1317880767571,138.106249999458,-5.90808986649102));
#299395=CARTESIAN_POINT('Ctrl Pts',(6.21213331202012,138.256249999457,-8.55026797822134));
#299396=CARTESIAN_POINT('Ctrl Pts',(3.10606665601001,138.406249999457,-9.5594902125713));
#299397=CARTESIAN_POINT('Ctrl Pts',(-9.29197430029324E-14,138.556249999456,
-10.5687124469213));
#299398=CARTESIAN_POINT('Ctrl Pts',(-3.1060666560102,138.706249999456,-9.5594902125713));
#299399=CARTESIAN_POINT('Ctrl Pts',(-6.21213331202031,138.856249999455,
-8.55026797822134));
#299400=CARTESIAN_POINT('Ctrl Pts',(-8.13178807675728,139.006249999454,
-5.90808986649102));
#299401=CARTESIAN_POINT('Ctrl Pts',(-10.0514428414943,139.156249999454,
-3.2659117547607));
#299402=CARTESIAN_POINT('Ctrl Pts',(-10.0514428414943,139.306249999453,
2.46189346052968E-15));
#299403=CARTESIAN_POINT('Ctrl Pts',(-10.0514428414943,139.456249999453,
3.26591175476071));
#299404=CARTESIAN_POINT('Ctrl Pts',(-8.13178807675728,139.606249999452,
5.90808986649102));
#299405=CARTESIAN_POINT('Ctrl Pts',(-6.21213331202031,139.756249999451,
8.55026797822134));
#299406=CARTESIAN_POINT('Ctrl Pts',(-3.1060666560102,139.906249999451,9.5594902125713));
#299407=CARTESIAN_POINT('Ctrl Pts',(-9.11950096649171E-14,140.05624999945,
10.5687124469213));
#299408=CARTESIAN_POINT('Ctrl Pts',(3.10606665601002,140.20624999945,9.5594902125713));
#299409=CARTESIAN_POINT('Ctrl Pts',(6.21213331202012,140.356249999449,8.55026797822134));
#299410=CARTESIAN_POINT('Ctrl Pts',(8.1317880767571,140.506249999448,5.90808986649102));
#299411=CARTESIAN_POINT('Ctrl Pts',(10.0514428414941,140.656249999448,3.2659117547607));
#299412=CARTESIAN_POINT('Ctrl Pts',(10.0514428414941,140.806249999447,-1.23094673026484E-15));
#299413=CARTESIAN_POINT('Ctrl Pts',(10.0514428414941,140.956249999447,-3.26591175476071));
#299414=CARTESIAN_POINT('Ctrl Pts',(8.1317880767571,141.106249999446,-5.90808986649102));
#299415=CARTESIAN_POINT('Ctrl Pts',(6.21213331202012,141.256249999445,-8.55026797822134));
#299416=CARTESIAN_POINT('Ctrl Pts',(3.10606665601001,141.406249999445,-9.5594902125713));
#299417=CARTESIAN_POINT('Ctrl Pts',(-9.46474522745942E-14,141.556249999444,
-10.5687124469213));
#299418=CARTESIAN_POINT('Ctrl Pts',(-3.1060666560102,141.706249999444,-9.5594902125713));
#299419=CARTESIAN_POINT('Ctrl Pts',(-6.21213331202031,141.856249999443,
-8.55026797822134));
#299420=CARTESIAN_POINT('Ctrl Pts',(-8.13178807675729,142.006249999442,
-5.90808986649102));
#299421=CARTESIAN_POINT('Ctrl Pts',(-10.0514428414943,142.156249999442,
-3.2659117547607));
#299422=CARTESIAN_POINT('Ctrl Pts',(-10.0514428414943,142.306249999441,
2.46189346052968E-15));
#299423=CARTESIAN_POINT('Ctrl Pts',(-10.0514428414943,142.456249999441,
3.26591175476071));
#299424=CARTESIAN_POINT('Ctrl Pts',(-8.13178807675729,142.60624999944,5.90808986649102));
#299425=CARTESIAN_POINT('Ctrl Pts',(-6.21213331202031,142.756249999439,
8.55026797822134));
#299426=CARTESIAN_POINT('Ctrl Pts',(-3.1060666560102,142.906249999439,9.5594902125713));
#299427=CARTESIAN_POINT('Ctrl Pts',(-9.29227189365789E-14,143.056249999438,
10.5687124469213));
#299428=CARTESIAN_POINT('Ctrl Pts',(3.10606665601001,143.206249999438,9.5594902125713));
#299429=CARTESIAN_POINT('Ctrl Pts',(6.21213331202012,143.356249999437,8.55026797822134));
#299430=CARTESIAN_POINT('Ctrl Pts',(8.1317880767571,143.506249999436,5.90808986649102));
#299431=CARTESIAN_POINT('Ctrl Pts',(10.0514428414941,143.656249999436,3.2659117547607));
#299432=CARTESIAN_POINT('Ctrl Pts',(10.0514428414941,143.806249999435,-1.23094673026484E-15));
#299433=CARTESIAN_POINT('Ctrl Pts',(10.0514428414941,143.956249999435,-3.26591175476071));
#299434=CARTESIAN_POINT('Ctrl Pts',(8.1317880767571,144.106249999434,-5.90808986649102));
#299435=CARTESIAN_POINT('Ctrl Pts',(6.21213331202012,144.256249999433,-8.55026797822134));
#299436=CARTESIAN_POINT('Ctrl Pts',(3.10606665601001,144.406249999433,-9.5594902125713));
#299437=CARTESIAN_POINT('Ctrl Pts',(-9.63751615462561E-14,144.556249999432,
-10.5687124469213));
#299438=CARTESIAN_POINT('Ctrl Pts',(-3.1060666560102,144.706249999432,-9.5594902125713));
#299439=CARTESIAN_POINT('Ctrl Pts',(-6.21213331202031,144.856249999431,
-8.55026797822134));
#299440=CARTESIAN_POINT('Ctrl Pts',(-8.13178807675729,145.00624999943,-5.90808986649102));
#299441=CARTESIAN_POINT('Ctrl Pts',(-10.0514428414943,145.15624999943,-3.2659117547607));
#299442=CARTESIAN_POINT('Ctrl Pts',(-10.0514428414943,145.306249999429,
2.46189346052968E-15));
#299443=CARTESIAN_POINT('Ctrl Pts',(-10.0514428414943,145.456249999429,
3.26591175476071));
#299444=CARTESIAN_POINT('Ctrl Pts',(-8.13178807675729,145.606249999428,
5.90808986649102));
#299445=CARTESIAN_POINT('Ctrl Pts',(-6.21213331202031,145.756249999427,
8.55026797822134));
#299446=CARTESIAN_POINT('Ctrl Pts',(-3.1060666560102,145.906249999427,9.5594902125713));
#299447=CARTESIAN_POINT('Ctrl Pts',(-9.46504282082408E-14,146.056249999426,
10.5687124469213));
#299448=CARTESIAN_POINT('Ctrl Pts',(3.10606665601001,146.206249999426,9.5594902125713));
#299449=CARTESIAN_POINT('Ctrl Pts',(6.21213331202012,146.356249999425,8.55026797822134));
#299450=CARTESIAN_POINT('Ctrl Pts',(8.13178807675709,146.506249999424,5.90808986649102));
#299451=CARTESIAN_POINT('Ctrl Pts',(10.0514428414941,146.656249999424,3.2659117547607));
#299452=CARTESIAN_POINT('Ctrl Pts',(10.0514428414941,146.806249999423,-1.23094673026484E-15));
#299453=CARTESIAN_POINT('Ctrl Pts',(10.0514428414941,146.956249999423,-3.26591175476071));
#299454=CARTESIAN_POINT('Ctrl Pts',(8.13178807675709,147.106249999422,-5.90808986649102));
#299455=CARTESIAN_POINT('Ctrl Pts',(6.21213331202012,147.256249999421,-8.55026797822134));
#299456=CARTESIAN_POINT('Ctrl Pts',(3.10606665601001,147.406249999421,-9.5594902125713));
#299457=CARTESIAN_POINT('Ctrl Pts',(-9.81028708179179E-14,147.55624999942,
-10.5687124469213));
#299458=CARTESIAN_POINT('Ctrl Pts',(-3.10606665601021,147.70624999942,-9.5594902125713));
#299459=CARTESIAN_POINT('Ctrl Pts',(-6.21213331202032,147.856249999419,
-8.55026797822134));
#299460=CARTESIAN_POINT('Ctrl Pts',(-8.13178807675729,148.006249999418,
-5.90808986649102));
#299461=CARTESIAN_POINT('Ctrl Pts',(-10.0514428414943,148.156249999418,
-3.2659117547607));
#299462=CARTESIAN_POINT('Ctrl Pts',(-10.0514428414943,148.306249999417,
2.46189346052968E-15));
#299463=CARTESIAN_POINT('Ctrl Pts',(-10.0514428414943,148.456249999417,
3.26591175476071));
#299464=CARTESIAN_POINT('Ctrl Pts',(-8.13178807675729,148.606249999416,
5.90808986649102));
#299465=CARTESIAN_POINT('Ctrl Pts',(-6.21213331202031,148.756249999415,
8.55026797822134));
#299466=CARTESIAN_POINT('Ctrl Pts',(-3.1060666560102,148.906249999415,9.5594902125713));
#299467=CARTESIAN_POINT('Ctrl Pts',(-9.63781374799026E-14,149.056249999414,
10.5687124469213));
#299468=CARTESIAN_POINT('Ctrl Pts',(3.10606665601001,149.206249999414,9.5594902125713));
#299469=CARTESIAN_POINT('Ctrl Pts',(6.21213331202012,149.356249999413,8.55026797822134));
#299470=CARTESIAN_POINT('Ctrl Pts',(8.13178807675709,149.506249999412,5.90808986649102));
#299471=CARTESIAN_POINT('Ctrl Pts',(10.0514428414941,149.656249999412,3.2659117547607));
#299472=CARTESIAN_POINT('Ctrl Pts',(10.0514428414941,149.806249999411,-1.23094673026484E-15));
#299473=CARTESIAN_POINT('Ctrl Pts',(10.0514428414941,149.956249999411,-3.26591175476071));
#299474=CARTESIAN_POINT('Ctrl Pts',(8.13178807675709,150.10624999941,-5.90808986649102));
#299475=CARTESIAN_POINT('Ctrl Pts',(6.21213331202012,150.256249999409,-8.55026797822134));
#299476=CARTESIAN_POINT('Ctrl Pts',(3.10606665601001,150.406249999409,-9.5594902125713));
#299477=CARTESIAN_POINT('Ctrl Pts',(-9.98305800895797E-14,150.556249999408,
-10.5687124469213));
#299478=CARTESIAN_POINT('Ctrl Pts',(-3.10606665601021,150.706249999408,
-9.5594902125713));
#299479=CARTESIAN_POINT('Ctrl Pts',(-6.21213331202032,150.856249999407,
-8.55026797822134));
#299480=CARTESIAN_POINT('Ctrl Pts',(-8.13178807675729,151.006249999406,
-5.90808986649102));
#299481=CARTESIAN_POINT('Ctrl Pts',(-10.0514428414943,151.156249999406,
-3.2659117547607));
#299482=CARTESIAN_POINT('Ctrl Pts',(-10.0514428414943,151.306249999405,
2.46189346052968E-15));
#299483=CARTESIAN_POINT('Ctrl Pts',(-10.0514428414943,151.456249999405,
3.26591175476071));
#299484=CARTESIAN_POINT('Ctrl Pts',(-8.13178807675729,151.606249999404,
5.90808986649102));
#299485=CARTESIAN_POINT('Ctrl Pts',(-6.21213331202032,151.756249999403,
8.55026797822134));
#299486=CARTESIAN_POINT('Ctrl Pts',(-3.10606665601021,151.906249999403,
9.5594902125713));
#299487=CARTESIAN_POINT('Ctrl Pts',(-9.81058467515645E-14,152.056249999402,
10.5687124469213));
#299488=CARTESIAN_POINT('Ctrl Pts',(3.10606665601001,152.206249999402,9.5594902125713));
#299489=CARTESIAN_POINT('Ctrl Pts',(6.21213331202012,152.356249999401,8.55026797822134));
#299490=CARTESIAN_POINT('Ctrl Pts',(8.13178807675709,152.5062499994,5.90808986649102));
#299491=CARTESIAN_POINT('Ctrl Pts',(10.0514428414941,152.6562499994,3.2659117547607));
#299492=CARTESIAN_POINT('Ctrl Pts',(10.0514428414941,152.806249999399,-1.23094673026484E-15));
#299493=CARTESIAN_POINT('Ctrl Pts',(10.0514428414941,152.956249999399,-3.26591175476071));
#299494=CARTESIAN_POINT('Ctrl Pts',(8.13178807675709,153.106249999398,-5.90808986649102));
#299495=CARTESIAN_POINT('Ctrl Pts',(6.21213331202012,153.256249999397,-8.55026797822134));
#299496=CARTESIAN_POINT('Ctrl Pts',(3.10606665601001,153.406249999397,-9.5594902125713));
#299497=CARTESIAN_POINT('Ctrl Pts',(-1.01558289361242E-13,153.556249999396,
-10.5687124469213));
#299498=CARTESIAN_POINT('Ctrl Pts',(-3.10606665601021,153.706249999396,
-9.5594902125713));
#299499=CARTESIAN_POINT('Ctrl Pts',(-12.1623797632097,-0.474999999988005,
2.97892388940585E-15));
#299500=CARTESIAN_POINT('Ctrl Pts',(-12.1623797632096,-0.324999999988605,
3.95179673813133));
#299501=CARTESIAN_POINT('Ctrl Pts',(-9.83957192047856,-0.174999999989203,
7.14886745759505));
#299502=CARTESIAN_POINT('Ctrl Pts',(-7.51676407774747,-0.0249999999898023,
10.3459381770588));
#299503=CARTESIAN_POINT('Ctrl Pts',(-3.75838203887374,0.1250000000096,11.5671105274568));
#299504=CARTESIAN_POINT('Ctrl Pts',(-1.02868273148643E-14,0.275000000009002,
12.7882828778549));
#299505=CARTESIAN_POINT('Ctrl Pts',(3.75838203887372,0.425000000008404,
11.5671105274568));
#299506=CARTESIAN_POINT('Ctrl Pts',(7.51676407774745,0.575000000007806,
10.3459381770588));
#299507=CARTESIAN_POINT('Ctrl Pts',(9.83957192047854,0.725000000007208,
7.14886745759505));
#299508=CARTESIAN_POINT('Ctrl Pts',(12.1623797632096,0.875000000006609,
3.95179673813132));
#299509=CARTESIAN_POINT('Ctrl Pts',(12.1623797632096,1.02500000000601,-1.48946194470292E-15));
#299510=CARTESIAN_POINT('Ctrl Pts',(12.1623797632096,1.17500000000541,-3.95179673813132));
#299511=CARTESIAN_POINT('Ctrl Pts',(9.83957192047853,1.32500000000481,-7.14886745759505));
#299512=CARTESIAN_POINT('Ctrl Pts',(7.51676407774744,1.47500000000421,-10.3459381770588));
#299513=CARTESIAN_POINT('Ctrl Pts',(3.75838203887371,1.6250000000036,-11.5671105274568));
#299514=CARTESIAN_POINT('Ctrl Pts',(-1.42829078892864E-14,1.775000000003,
-12.7882828778549));
#299515=CARTESIAN_POINT('Ctrl Pts',(-3.75838203887374,1.9250000000024,-11.5671105274568));
#299516=CARTESIAN_POINT('Ctrl Pts',(-7.51676407774747,2.0750000000018,-10.3459381770588));
#299517=CARTESIAN_POINT('Ctrl Pts',(-9.83957192047856,2.2250000000012,-7.14886745759505));
#299518=CARTESIAN_POINT('Ctrl Pts',(-12.1623797632097,2.37500000000059,
-3.95179673813132));
#299519=CARTESIAN_POINT('Ctrl Pts',(-12.1623797632097,2.525,2.97892388940585E-15));
#299520=CARTESIAN_POINT('Ctrl Pts',(-12.1623797632097,2.6749999999994,3.95179673813133));
#299521=CARTESIAN_POINT('Ctrl Pts',(-9.83957192047856,2.8249999999988,7.14886745759505));
#299522=CARTESIAN_POINT('Ctrl Pts',(-7.51676407774747,2.9749999999982,10.3459381770588));
#299523=CARTESIAN_POINT('Ctrl Pts',(-3.75838203887374,3.1249999999976,11.5671105274568));
#299524=CARTESIAN_POINT('Ctrl Pts',(-1.20145365865262E-14,3.274999999997,
12.7882828778549));
#299525=CARTESIAN_POINT('Ctrl Pts',(3.75838203887372,3.4249999999964,11.5671105274568));
#299526=CARTESIAN_POINT('Ctrl Pts',(7.51676407774744,3.57499999999581,10.3459381770588));
#299527=CARTESIAN_POINT('Ctrl Pts',(9.83957192047853,3.72499999999521,7.14886745759505));
#299528=CARTESIAN_POINT('Ctrl Pts',(12.1623797632096,3.87499999999461,3.95179673813132));
#299529=CARTESIAN_POINT('Ctrl Pts',(12.1623797632096,4.02499999999401,-1.48946194470292E-15));
#299530=CARTESIAN_POINT('Ctrl Pts',(12.1623797632096,4.17499999999341,-3.95179673813132));
#299531=CARTESIAN_POINT('Ctrl Pts',(9.83957192047853,4.32499999999281,-7.14886745759505));
#299532=CARTESIAN_POINT('Ctrl Pts',(7.51676407774744,4.47499999999221,-10.3459381770588));
#299533=CARTESIAN_POINT('Ctrl Pts',(3.75838203887371,4.6249999999916,-11.5671105274568));
#299534=CARTESIAN_POINT('Ctrl Pts',(-1.60106171609483E-14,4.774999999991,
-12.7882828778549));
#299535=CARTESIAN_POINT('Ctrl Pts',(-3.75838203887374,4.9249999999904,-11.5671105274568));
#299536=CARTESIAN_POINT('Ctrl Pts',(-7.51676407774747,5.0749999999898,-10.3459381770588));
#299537=CARTESIAN_POINT('Ctrl Pts',(-9.83957192047857,5.2249999999892,-7.14886745759505));
#299538=CARTESIAN_POINT('Ctrl Pts',(-12.1623797632097,5.3749999999886,-3.95179673813132));
#299539=CARTESIAN_POINT('Ctrl Pts',(-12.1623797632097,5.52499999998799,
2.97892388940585E-15));
#299540=CARTESIAN_POINT('Ctrl Pts',(-12.1623797632097,5.6749999999874,3.95179673813133));
#299541=CARTESIAN_POINT('Ctrl Pts',(-9.83957192047857,5.8249999999868,7.14886745759505));
#299542=CARTESIAN_POINT('Ctrl Pts',(-7.51676407774747,5.9749999999862,10.3459381770588));
#299543=CARTESIAN_POINT('Ctrl Pts',(-3.75838203887374,6.1249999999856,11.5671105274568));
#299544=CARTESIAN_POINT('Ctrl Pts',(-1.3742245858188E-14,6.274999999985,
12.7882828778549));
#299545=CARTESIAN_POINT('Ctrl Pts',(3.75838203887371,6.4249999999844,11.5671105274568));
#299546=CARTESIAN_POINT('Ctrl Pts',(7.51676407774744,6.57499999998381,10.3459381770588));
#299547=CARTESIAN_POINT('Ctrl Pts',(9.83957192047853,6.72499999998321,7.14886745759505));
#299548=CARTESIAN_POINT('Ctrl Pts',(12.1623797632096,6.87499999998261,3.95179673813132));
#299549=CARTESIAN_POINT('Ctrl Pts',(12.1623797632096,7.02499999998201,-1.48946194470292E-15));
#299550=CARTESIAN_POINT('Ctrl Pts',(12.1623797632096,7.17499999998141,-3.95179673813132));
#299551=CARTESIAN_POINT('Ctrl Pts',(9.83957192047853,7.32499999998081,-7.14886745759505));
#299552=CARTESIAN_POINT('Ctrl Pts',(7.51676407774744,7.47499999998021,-10.3459381770588));
#299553=CARTESIAN_POINT('Ctrl Pts',(3.75838203887371,7.6249999999796,-11.5671105274568));
#299554=CARTESIAN_POINT('Ctrl Pts',(-1.77383264326101E-14,7.774999999979,
-12.7882828778549));
#299555=CARTESIAN_POINT('Ctrl Pts',(-3.75838203887375,7.9249999999784,-11.5671105274568));
#299556=CARTESIAN_POINT('Ctrl Pts',(-7.51676407774747,8.0749999999778,-10.3459381770588));
#299557=CARTESIAN_POINT('Ctrl Pts',(-9.83957192047857,8.2249999999772,-7.14886745759505));
#299558=CARTESIAN_POINT('Ctrl Pts',(-12.1623797632097,8.3749999999766,-3.95179673813132));
#299559=CARTESIAN_POINT('Ctrl Pts',(-12.1623797632097,8.52499999997599,
2.97892388940585E-15));
#299560=CARTESIAN_POINT('Ctrl Pts',(-12.1623797632097,8.6749999999754,3.95179673813133));
#299561=CARTESIAN_POINT('Ctrl Pts',(-9.83957192047857,8.8249999999748,7.14886745759505));
#299562=CARTESIAN_POINT('Ctrl Pts',(-7.51676407774747,8.9749999999742,10.3459381770588));
#299563=CARTESIAN_POINT('Ctrl Pts',(-3.75838203887374,9.1249999999736,11.5671105274568));
#299564=CARTESIAN_POINT('Ctrl Pts',(-1.54699551298498E-14,9.274999999973,
12.7882828778549));
#299565=CARTESIAN_POINT('Ctrl Pts',(3.75838203887371,9.4249999999724,11.5671105274568));
#299566=CARTESIAN_POINT('Ctrl Pts',(7.51676407774744,9.57499999997181,10.3459381770588));
#299567=CARTESIAN_POINT('Ctrl Pts',(9.83957192047853,9.72499999997121,7.14886745759505));
#299568=CARTESIAN_POINT('Ctrl Pts',(12.1623797632096,9.87499999997061,3.95179673813132));
#299569=CARTESIAN_POINT('Ctrl Pts',(12.1623797632096,10.02499999997,-1.48946194470292E-15));
#299570=CARTESIAN_POINT('Ctrl Pts',(12.1623797632096,10.1749999999694,-3.95179673813132));
#299571=CARTESIAN_POINT('Ctrl Pts',(9.83957192047853,10.3249999999688,-7.14886745759505));
#299572=CARTESIAN_POINT('Ctrl Pts',(7.51676407774744,10.4749999999682,-10.3459381770588));
#299573=CARTESIAN_POINT('Ctrl Pts',(3.75838203887371,10.6249999999676,-11.5671105274568));
#299574=CARTESIAN_POINT('Ctrl Pts',(-1.9466035704272E-14,10.774999999967,
-12.7882828778549));
#299575=CARTESIAN_POINT('Ctrl Pts',(-3.75838203887375,10.9249999999664,
-11.5671105274568));
#299576=CARTESIAN_POINT('Ctrl Pts',(-7.51676407774748,11.0749999999658,
-10.3459381770588));
#299577=CARTESIAN_POINT('Ctrl Pts',(-9.83957192047857,11.2249999999652,
-7.14886745759505));
#299578=CARTESIAN_POINT('Ctrl Pts',(-12.1623797632097,11.3749999999646,
-3.95179673813132));
#299579=CARTESIAN_POINT('Ctrl Pts',(-12.1623797632097,11.524999999964,2.97892388940585E-15));
#299580=CARTESIAN_POINT('Ctrl Pts',(-12.1623797632097,11.6749999999634,
3.95179673813133));
#299581=CARTESIAN_POINT('Ctrl Pts',(-9.83957192047857,11.8249999999628,
7.14886745759505));
#299582=CARTESIAN_POINT('Ctrl Pts',(-7.51676407774747,11.9749999999622,
10.3459381770588));
#299583=CARTESIAN_POINT('Ctrl Pts',(-3.75838203887375,12.1249999999616,
11.5671105274568));
#299584=CARTESIAN_POINT('Ctrl Pts',(-1.71976644015117E-14,12.274999999961,
12.7882828778549));
#299585=CARTESIAN_POINT('Ctrl Pts',(3.75838203887371,12.4249999999604,11.5671105274568));
#299586=CARTESIAN_POINT('Ctrl Pts',(7.51676407774744,12.5749999999598,10.3459381770588));
#299587=CARTESIAN_POINT('Ctrl Pts',(9.83957192047853,12.7249999999592,7.14886745759505));
#299588=CARTESIAN_POINT('Ctrl Pts',(12.1623797632096,12.8749999999586,3.95179673813132));
#299589=CARTESIAN_POINT('Ctrl Pts',(12.1623797632096,13.024999999958,-1.48946194470292E-15));
#299590=CARTESIAN_POINT('Ctrl Pts',(12.1623797632096,13.1749999999574,-3.95179673813132));
#299591=CARTESIAN_POINT('Ctrl Pts',(9.83957192047853,13.3249999999568,-7.14886745759505));
#299592=CARTESIAN_POINT('Ctrl Pts',(7.51676407774743,13.4749999999562,-10.3459381770588));
#299593=CARTESIAN_POINT('Ctrl Pts',(3.75838203887371,13.6249999999556,-11.5671105274568));
#299594=CARTESIAN_POINT('Ctrl Pts',(-2.11937449759338E-14,13.774999999955,
-12.7882828778549));
#299595=CARTESIAN_POINT('Ctrl Pts',(-3.75838203887375,13.9249999999544,
-11.5671105274568));
#299596=CARTESIAN_POINT('Ctrl Pts',(-7.51676407774748,14.0749999999538,
-10.3459381770588));
#299597=CARTESIAN_POINT('Ctrl Pts',(-9.83957192047857,14.2249999999532,
-7.14886745759505));
#299598=CARTESIAN_POINT('Ctrl Pts',(-12.1623797632097,14.3749999999526,
-3.95179673813132));
#299599=CARTESIAN_POINT('Ctrl Pts',(-12.1623797632097,14.524999999952,2.97892388940585E-15));
#299600=CARTESIAN_POINT('Ctrl Pts',(-12.1623797632097,14.6749999999514,
3.95179673813133));
#299601=CARTESIAN_POINT('Ctrl Pts',(-9.83957192047857,14.8249999999508,
7.14886745759505));
#299602=CARTESIAN_POINT('Ctrl Pts',(-7.51676407774747,14.9749999999502,
10.3459381770588));
#299603=CARTESIAN_POINT('Ctrl Pts',(-3.75838203887375,15.1249999999496,
11.5671105274568));
#299604=CARTESIAN_POINT('Ctrl Pts',(-1.89253736731735E-14,15.274999999949,
12.7882828778549));
#299605=CARTESIAN_POINT('Ctrl Pts',(3.75838203887371,15.4249999999484,11.5671105274568));
#299606=CARTESIAN_POINT('Ctrl Pts',(7.51676407774744,15.5749999999478,10.3459381770588));
#299607=CARTESIAN_POINT('Ctrl Pts',(9.83957192047853,15.7249999999472,7.14886745759505));
#299608=CARTESIAN_POINT('Ctrl Pts',(12.1623797632096,15.8749999999466,3.95179673813132));
#299609=CARTESIAN_POINT('Ctrl Pts',(12.1623797632096,16.024999999946,-1.48946194470292E-15));
#299610=CARTESIAN_POINT('Ctrl Pts',(12.1623797632096,16.1749999999454,-3.95179673813132));
#299611=CARTESIAN_POINT('Ctrl Pts',(9.83957192047852,16.3249999999448,-7.14886745759505));
#299612=CARTESIAN_POINT('Ctrl Pts',(7.51676407774743,16.4749999999442,-10.3459381770588));
#299613=CARTESIAN_POINT('Ctrl Pts',(3.7583820388737,16.6249999999436,-11.5671105274568));
#299614=CARTESIAN_POINT('Ctrl Pts',(-2.29214542475956E-14,16.774999999943,
-12.7882828778549));
#299615=CARTESIAN_POINT('Ctrl Pts',(-3.75838203887375,16.9249999999424,
-11.5671105274568));
#299616=CARTESIAN_POINT('Ctrl Pts',(-7.51676407774748,17.0749999999418,
-10.3459381770588));
#299617=CARTESIAN_POINT('Ctrl Pts',(-9.83957192047857,17.2249999999412,
-7.14886745759505));
#299618=CARTESIAN_POINT('Ctrl Pts',(-12.1623797632097,17.3749999999406,
-3.95179673813132));
#299619=CARTESIAN_POINT('Ctrl Pts',(-12.1623797632097,17.52499999994,2.97892388940585E-15));
#299620=CARTESIAN_POINT('Ctrl Pts',(-12.1623797632097,17.6749999999394,
3.95179673813133));
#299621=CARTESIAN_POINT('Ctrl Pts',(-9.83957192047857,17.8249999999388,
7.14886745759505));
#299622=CARTESIAN_POINT('Ctrl Pts',(-7.51676407774748,17.9749999999382,
10.3459381770588));
#299623=CARTESIAN_POINT('Ctrl Pts',(-3.75838203887375,18.1249999999376,
11.5671105274568));
#299624=CARTESIAN_POINT('Ctrl Pts',(-2.06530829448354E-14,18.274999999937,
12.7882828778549));
#299625=CARTESIAN_POINT('Ctrl Pts',(3.75838203887371,18.4249999999364,11.5671105274568));
#299626=CARTESIAN_POINT('Ctrl Pts',(7.51676407774743,18.5749999999358,10.3459381770588));
#299627=CARTESIAN_POINT('Ctrl Pts',(9.83957192047852,18.7249999999352,7.14886745759505));
#299628=CARTESIAN_POINT('Ctrl Pts',(12.1623797632096,18.8749999999346,3.95179673813132));
#299629=CARTESIAN_POINT('Ctrl Pts',(12.1623797632096,19.024999999934,-1.48946194470292E-15));
#299630=CARTESIAN_POINT('Ctrl Pts',(12.1623797632096,19.1749999999334,-3.95179673813132));
#299631=CARTESIAN_POINT('Ctrl Pts',(9.83957192047852,19.3249999999328,-7.14886745759505));
#299632=CARTESIAN_POINT('Ctrl Pts',(7.51676407774743,19.4749999999322,-10.3459381770588));
#299633=CARTESIAN_POINT('Ctrl Pts',(3.7583820388737,19.6249999999316,-11.5671105274568));
#299634=CARTESIAN_POINT('Ctrl Pts',(-2.46491635192575E-14,19.774999999931,
-12.7882828778549));
#299635=CARTESIAN_POINT('Ctrl Pts',(-3.75838203887375,19.9249999999304,
-11.5671105274568));
#299636=CARTESIAN_POINT('Ctrl Pts',(-7.51676407774748,20.0749999999298,
-10.3459381770588));
#299637=CARTESIAN_POINT('Ctrl Pts',(-9.83957192047857,20.2249999999292,
-7.14886745759505));
#299638=CARTESIAN_POINT('Ctrl Pts',(-12.1623797632097,20.3749999999286,
-3.95179673813132));
#299639=CARTESIAN_POINT('Ctrl Pts',(-12.1623797632097,20.524999999928,2.97892388940585E-15));
#299640=CARTESIAN_POINT('Ctrl Pts',(-12.1623797632097,20.6749999999274,
3.95179673813133));
#299641=CARTESIAN_POINT('Ctrl Pts',(-9.83957192047857,20.8249999999268,
7.14886745759505));
#299642=CARTESIAN_POINT('Ctrl Pts',(-7.51676407774748,20.9749999999262,
10.3459381770588));
#299643=CARTESIAN_POINT('Ctrl Pts',(-3.75838203887375,21.1249999999256,
11.5671105274568));
#299644=CARTESIAN_POINT('Ctrl Pts',(-2.23807922164972E-14,21.274999999925,
12.7882828778549));
#299645=CARTESIAN_POINT('Ctrl Pts',(3.7583820388737,21.4249999999244,11.5671105274568));
#299646=CARTESIAN_POINT('Ctrl Pts',(7.51676407774743,21.5749999999238,10.3459381770588));
#299647=CARTESIAN_POINT('Ctrl Pts',(9.83957192047852,21.7249999999232,7.14886745759505));
#299648=CARTESIAN_POINT('Ctrl Pts',(12.1623797632096,21.8749999999226,3.95179673813132));
#299649=CARTESIAN_POINT('Ctrl Pts',(12.1623797632096,22.024999999922,-1.48946194470292E-15));
#299650=CARTESIAN_POINT('Ctrl Pts',(12.1623797632096,22.1749999999214,-3.95179673813132));
#299651=CARTESIAN_POINT('Ctrl Pts',(9.83957192047852,22.3249999999208,-7.14886745759505));
#299652=CARTESIAN_POINT('Ctrl Pts',(7.51676407774743,22.4749999999202,-10.3459381770588));
#299653=CARTESIAN_POINT('Ctrl Pts',(3.7583820388737,22.6249999999196,-11.5671105274568));
#299654=CARTESIAN_POINT('Ctrl Pts',(-2.63768727909193E-14,22.774999999919,
-12.7882828778549));
#299655=CARTESIAN_POINT('Ctrl Pts',(-3.75838203887375,22.9249999999184,
-11.5671105274568));
#299656=CARTESIAN_POINT('Ctrl Pts',(-7.51676407774748,23.0749999999178,
-10.3459381770588));
#299657=CARTESIAN_POINT('Ctrl Pts',(-9.83957192047857,23.2249999999172,
-7.14886745759505));
#299658=CARTESIAN_POINT('Ctrl Pts',(-12.1623797632097,23.3749999999166,
-3.95179673813132));
#299659=CARTESIAN_POINT('Ctrl Pts',(-12.1623797632097,23.524999999916,2.97892388940585E-15));
#299660=CARTESIAN_POINT('Ctrl Pts',(-12.1623797632097,23.6749999999154,
3.95179673813133));
#299661=CARTESIAN_POINT('Ctrl Pts',(-9.83957192047857,23.8249999999148,
7.14886745759505));
#299662=CARTESIAN_POINT('Ctrl Pts',(-7.51676407774748,23.9749999999142,
10.3459381770588));
#299663=CARTESIAN_POINT('Ctrl Pts',(-3.75838203887375,24.1249999999136,
11.5671105274568));
#299664=CARTESIAN_POINT('Ctrl Pts',(-2.4108501488159E-14,24.274999999913,
12.7882828778549));
#299665=CARTESIAN_POINT('Ctrl Pts',(3.7583820388737,24.4249999999124,11.5671105274568));
#299666=CARTESIAN_POINT('Ctrl Pts',(7.51676407774743,24.5749999999118,10.3459381770588));
#299667=CARTESIAN_POINT('Ctrl Pts',(9.83957192047852,24.7249999999112,7.14886745759505));
#299668=CARTESIAN_POINT('Ctrl Pts',(12.1623797632096,24.8749999999106,3.95179673813132));
#299669=CARTESIAN_POINT('Ctrl Pts',(12.1623797632096,25.02499999991,-1.48946194470292E-15));
#299670=CARTESIAN_POINT('Ctrl Pts',(12.1623797632096,25.1749999999094,-3.95179673813132));
#299671=CARTESIAN_POINT('Ctrl Pts',(9.83957192047852,25.3249999999088,-7.14886745759505));
#299672=CARTESIAN_POINT('Ctrl Pts',(7.51676407774743,25.4749999999082,-10.3459381770588));
#299673=CARTESIAN_POINT('Ctrl Pts',(3.7583820388737,25.6249999999076,-11.5671105274568));
#299674=CARTESIAN_POINT('Ctrl Pts',(-2.81045820625811E-14,25.774999999907,
-12.7882828778549));
#299675=CARTESIAN_POINT('Ctrl Pts',(-3.75838203887376,25.9249999999064,
-11.5671105274568));
#299676=CARTESIAN_POINT('Ctrl Pts',(-7.51676407774749,26.0749999999058,
-10.3459381770588));
#299677=CARTESIAN_POINT('Ctrl Pts',(-9.83957192047857,26.2249999999052,
-7.14886745759505));
#299678=CARTESIAN_POINT('Ctrl Pts',(-12.1623797632097,26.3749999999046,
-3.95179673813132));
#299679=CARTESIAN_POINT('Ctrl Pts',(-12.1623797632097,26.524999999904,2.97892388940585E-15));
#299680=CARTESIAN_POINT('Ctrl Pts',(-12.1623797632097,26.6749999999034,
3.95179673813133));
#299681=CARTESIAN_POINT('Ctrl Pts',(-9.83957192047857,26.8249999999028,
7.14886745759505));
#299682=CARTESIAN_POINT('Ctrl Pts',(-7.51676407774748,26.9749999999022,
10.3459381770588));
#299683=CARTESIAN_POINT('Ctrl Pts',(-3.75838203887375,27.1249999999016,
11.5671105274568));
#299684=CARTESIAN_POINT('Ctrl Pts',(-2.58362107598209E-14,27.274999999901,
12.7882828778549));
#299685=CARTESIAN_POINT('Ctrl Pts',(3.7583820388737,27.4249999999004,11.5671105274568));
#299686=CARTESIAN_POINT('Ctrl Pts',(7.51676407774743,27.5749999998998,10.3459381770588));
#299687=CARTESIAN_POINT('Ctrl Pts',(9.83957192047852,27.7249999998992,7.14886745759505));
#299688=CARTESIAN_POINT('Ctrl Pts',(12.1623797632096,27.8749999998986,3.95179673813132));
#299689=CARTESIAN_POINT('Ctrl Pts',(12.1623797632096,28.024999999898,-1.48946194470292E-15));
#299690=CARTESIAN_POINT('Ctrl Pts',(12.1623797632096,28.1749999998974,-3.95179673813132));
#299691=CARTESIAN_POINT('Ctrl Pts',(9.83957192047852,28.3249999998968,-7.14886745759505));
#299692=CARTESIAN_POINT('Ctrl Pts',(7.51676407774743,28.4749999998962,-10.3459381770588));
#299693=CARTESIAN_POINT('Ctrl Pts',(3.7583820388737,28.6249999998956,-11.5671105274568));
#299694=CARTESIAN_POINT('Ctrl Pts',(-2.9832291334243E-14,28.774999999895,
-12.7882828778549));
#299695=CARTESIAN_POINT('Ctrl Pts',(-3.75838203887376,28.9249999998944,
-11.5671105274568));
#299696=CARTESIAN_POINT('Ctrl Pts',(-7.51676407774749,29.0749999998938,
-10.3459381770588));
#299697=CARTESIAN_POINT('Ctrl Pts',(-9.83957192047858,29.2249999998932,
-7.14886745759505));
#299698=CARTESIAN_POINT('Ctrl Pts',(-12.1623797632097,29.3749999998926,
-3.95179673813132));
#299699=CARTESIAN_POINT('Ctrl Pts',(-12.1623797632097,29.524999999892,2.97892388940585E-15));
#299700=CARTESIAN_POINT('Ctrl Pts',(-12.1623797632097,29.6749999998914,
3.95179673813133));
#299701=CARTESIAN_POINT('Ctrl Pts',(-9.83957192047858,29.8249999998908,
7.14886745759505));
#299702=CARTESIAN_POINT('Ctrl Pts',(-7.51676407774748,29.9749999998902,
10.3459381770588));
#299703=CARTESIAN_POINT('Ctrl Pts',(-3.75838203887376,30.1249999998896,
11.5671105274568));
#299704=CARTESIAN_POINT('Ctrl Pts',(-2.75639200314827E-14,30.274999999889,
12.7882828778549));
#299705=CARTESIAN_POINT('Ctrl Pts',(3.7583820388737,30.4249999998884,11.5671105274568));
#299706=CARTESIAN_POINT('Ctrl Pts',(7.51676407774743,30.5749999998878,10.3459381770588));
#299707=CARTESIAN_POINT('Ctrl Pts',(9.83957192047852,30.7249999998872,7.14886745759505));
#299708=CARTESIAN_POINT('Ctrl Pts',(12.1623797632096,30.8749999998866,3.95179673813132));
#299709=CARTESIAN_POINT('Ctrl Pts',(12.1623797632096,31.024999999886,-1.48946194470292E-15));
#299710=CARTESIAN_POINT('Ctrl Pts',(12.1623797632096,31.1749999998854,-3.95179673813132));
#299711=CARTESIAN_POINT('Ctrl Pts',(9.83957192047852,31.3249999998848,-7.14886745759505));
#299712=CARTESIAN_POINT('Ctrl Pts',(7.51676407774742,31.4749999998842,-10.3459381770588));
#299713=CARTESIAN_POINT('Ctrl Pts',(3.7583820388737,31.6249999998836,-11.5671105274568));
#299714=CARTESIAN_POINT('Ctrl Pts',(-3.15600006059048E-14,31.774999999883,
-12.7882828778549));
#299715=CARTESIAN_POINT('Ctrl Pts',(-3.75838203887376,31.9249999998824,
-11.5671105274568));
#299716=CARTESIAN_POINT('Ctrl Pts',(-7.51676407774749,32.0749999998818,
-10.3459381770588));
#299717=CARTESIAN_POINT('Ctrl Pts',(-9.83957192047858,32.2249999998812,
-7.14886745759505));
#299718=CARTESIAN_POINT('Ctrl Pts',(-12.1623797632097,32.3749999998806,
-3.95179673813132));
#299719=CARTESIAN_POINT('Ctrl Pts',(-12.1623797632097,32.52499999988,2.97892388940585E-15));
#299720=CARTESIAN_POINT('Ctrl Pts',(-12.1623797632097,32.6749999998794,
3.95179673813133));
#299721=CARTESIAN_POINT('Ctrl Pts',(-9.83957192047858,32.8249999998788,
7.14886745759505));
#299722=CARTESIAN_POINT('Ctrl Pts',(-7.51676407774749,32.9749999998782,
10.3459381770588));
#299723=CARTESIAN_POINT('Ctrl Pts',(-3.75838203887376,33.1249999998776,
11.5671105274568));
#299724=CARTESIAN_POINT('Ctrl Pts',(-2.92916293031446E-14,33.274999999877,
12.7882828778549));
#299725=CARTESIAN_POINT('Ctrl Pts',(3.7583820388737,33.4249999998764,11.5671105274568));
#299726=CARTESIAN_POINT('Ctrl Pts',(7.51676407774743,33.5749999998758,10.3459381770588));
#299727=CARTESIAN_POINT('Ctrl Pts',(9.83957192047852,33.7249999998752,7.14886745759505));
#299728=CARTESIAN_POINT('Ctrl Pts',(12.1623797632096,33.8749999998746,3.95179673813132));
#299729=CARTESIAN_POINT('Ctrl Pts',(12.1623797632096,34.024999999874,-1.48946194470292E-15));
#299730=CARTESIAN_POINT('Ctrl Pts',(12.1623797632096,34.1749999998734,-3.95179673813132));
#299731=CARTESIAN_POINT('Ctrl Pts',(9.83957192047851,34.3249999998728,-7.14886745759505));
#299732=CARTESIAN_POINT('Ctrl Pts',(7.51676407774742,34.4749999998722,-10.3459381770588));
#299733=CARTESIAN_POINT('Ctrl Pts',(3.7583820388737,34.6249999998716,-11.5671105274568));
#299734=CARTESIAN_POINT('Ctrl Pts',(-3.32877098775667E-14,34.774999999871,
-12.7882828778549));
#299735=CARTESIAN_POINT('Ctrl Pts',(-3.75838203887376,34.9249999998704,
-11.5671105274568));
#299736=CARTESIAN_POINT('Ctrl Pts',(-7.51676407774749,35.0749999998698,
-10.3459381770588));
#299737=CARTESIAN_POINT('Ctrl Pts',(-9.83957192047858,35.2249999998692,
-7.14886745759505));
#299738=CARTESIAN_POINT('Ctrl Pts',(-12.1623797632097,35.3749999998686,
-3.95179673813132));
#299739=CARTESIAN_POINT('Ctrl Pts',(-12.1623797632097,35.524999999868,2.97892388940585E-15));
#299740=CARTESIAN_POINT('Ctrl Pts',(-12.1623797632097,35.6749999998674,
3.95179673813133));
#299741=CARTESIAN_POINT('Ctrl Pts',(-9.83957192047858,35.8249999998668,
7.14886745759505));
#299742=CARTESIAN_POINT('Ctrl Pts',(-7.51676407774749,35.9749999998662,
10.3459381770588));
#299743=CARTESIAN_POINT('Ctrl Pts',(-3.75838203887376,36.1249999998656,
11.5671105274568));
#299744=CARTESIAN_POINT('Ctrl Pts',(-3.10193385748064E-14,36.274999999865,
12.7882828778549));
#299745=CARTESIAN_POINT('Ctrl Pts',(3.7583820388737,36.4249999998644,11.5671105274568));
#299746=CARTESIAN_POINT('Ctrl Pts',(7.51676407774742,36.5749999998638,10.3459381770588));
#299747=CARTESIAN_POINT('Ctrl Pts',(9.83957192047851,36.7249999998632,7.14886745759505));
#299748=CARTESIAN_POINT('Ctrl Pts',(12.1623797632096,36.8749999998626,3.95179673813132));
#299749=CARTESIAN_POINT('Ctrl Pts',(12.1623797632096,37.024999999862,-1.48946194470292E-15));
#299750=CARTESIAN_POINT('Ctrl Pts',(12.1623797632096,37.1749999998614,-3.95179673813132));
#299751=CARTESIAN_POINT('Ctrl Pts',(9.83957192047851,37.3249999998608,-7.14886745759505));
#299752=CARTESIAN_POINT('Ctrl Pts',(7.51676407774742,37.4749999998602,-10.3459381770588));
#299753=CARTESIAN_POINT('Ctrl Pts',(3.75838203887369,37.6249999998596,-11.5671105274568));
#299754=CARTESIAN_POINT('Ctrl Pts',(-3.50154191492285E-14,37.774999999859,
-12.7882828778549));
#299755=CARTESIAN_POINT('Ctrl Pts',(-3.75838203887376,37.9249999998584,
-11.5671105274568));
#299756=CARTESIAN_POINT('Ctrl Pts',(-7.51676407774749,38.0749999998578,
-10.3459381770588));
#299757=CARTESIAN_POINT('Ctrl Pts',(-9.83957192047858,38.2249999998572,
-7.14886745759505));
#299758=CARTESIAN_POINT('Ctrl Pts',(-12.1623797632097,38.3749999998566,
-3.95179673813132));
#299759=CARTESIAN_POINT('Ctrl Pts',(-12.1623797632097,38.524999999856,2.97892388940585E-15));
#299760=CARTESIAN_POINT('Ctrl Pts',(-12.1623797632097,38.6749999998554,
3.95179673813133));
#299761=CARTESIAN_POINT('Ctrl Pts',(-9.83957192047858,38.8249999998548,
7.14886745759505));
#299762=CARTESIAN_POINT('Ctrl Pts',(-7.51676407774749,38.9749999998542,
10.3459381770588));
#299763=CARTESIAN_POINT('Ctrl Pts',(-3.75838203887376,39.1249999998536,
11.5671105274568));
#299764=CARTESIAN_POINT('Ctrl Pts',(-3.27470478464682E-14,39.274999999853,
12.7882828778549));
#299765=CARTESIAN_POINT('Ctrl Pts',(3.7583820388737,39.4249999998524,11.5671105274568));
#299766=CARTESIAN_POINT('Ctrl Pts',(7.51676407774742,39.5749999998518,10.3459381770588));
#299767=CARTESIAN_POINT('Ctrl Pts',(9.83957192047851,39.7249999998512,7.14886745759505));
#299768=CARTESIAN_POINT('Ctrl Pts',(12.1623797632096,39.8749999998506,3.95179673813132));
#299769=CARTESIAN_POINT('Ctrl Pts',(12.1623797632096,40.02499999985,-1.48946194470292E-15));
#299770=CARTESIAN_POINT('Ctrl Pts',(12.1623797632096,40.1749999998494,-3.95179673813132));
#299771=CARTESIAN_POINT('Ctrl Pts',(9.83957192047851,40.3249999998488,-7.14886745759505));
#299772=CARTESIAN_POINT('Ctrl Pts',(7.51676407774742,40.4749999998482,-10.3459381770588));
#299773=CARTESIAN_POINT('Ctrl Pts',(3.75838203887369,40.6249999998476,-11.5671105274568));
#299774=CARTESIAN_POINT('Ctrl Pts',(-3.67431284208903E-14,40.774999999847,
-12.7882828778549));
#299775=CARTESIAN_POINT('Ctrl Pts',(-3.75838203887376,40.9249999998464,
-11.5671105274568));
#299776=CARTESIAN_POINT('Ctrl Pts',(-7.51676407774749,41.0749999998458,
-10.3459381770588));
#299777=CARTESIAN_POINT('Ctrl Pts',(-9.83957192047858,41.2249999998452,
-7.14886745759505));
#299778=CARTESIAN_POINT('Ctrl Pts',(-12.1623797632097,41.3749999998446,
-3.95179673813132));
#299779=CARTESIAN_POINT('Ctrl Pts',(-12.1623797632097,41.524999999844,2.97892388940585E-15));
#299780=CARTESIAN_POINT('Ctrl Pts',(-12.1623797632097,41.6749999998434,
3.95179673813133));
#299781=CARTESIAN_POINT('Ctrl Pts',(-9.83957192047858,41.8249999998428,
7.14886745759505));
#299782=CARTESIAN_POINT('Ctrl Pts',(-7.51676407774749,41.9749999998422,
10.3459381770588));
#299783=CARTESIAN_POINT('Ctrl Pts',(-3.75838203887376,42.1249999998416,
11.5671105274568));
#299784=CARTESIAN_POINT('Ctrl Pts',(-3.44747571181301E-14,42.274999999841,
12.7882828778549));
#299785=CARTESIAN_POINT('Ctrl Pts',(3.75838203887369,42.4249999998404,11.5671105274568));
#299786=CARTESIAN_POINT('Ctrl Pts',(7.51676407774742,42.5749999998398,10.3459381770588));
#299787=CARTESIAN_POINT('Ctrl Pts',(9.83957192047851,42.7249999998392,7.14886745759505));
#299788=CARTESIAN_POINT('Ctrl Pts',(12.1623797632096,42.8749999998386,3.95179673813132));
#299789=CARTESIAN_POINT('Ctrl Pts',(12.1623797632096,43.024999999838,-1.48946194470292E-15));
#299790=CARTESIAN_POINT('Ctrl Pts',(12.1623797632096,43.1749999998374,-3.95179673813132));
#299791=CARTESIAN_POINT('Ctrl Pts',(9.83957192047851,43.3249999998368,-7.14886745759505));
#299792=CARTESIAN_POINT('Ctrl Pts',(7.51676407774742,43.4749999998362,-10.3459381770588));
#299793=CARTESIAN_POINT('Ctrl Pts',(3.75838203887369,43.6249999998356,-11.5671105274568));
#299794=CARTESIAN_POINT('Ctrl Pts',(-3.84708376925522E-14,43.774999999835,
-12.7882828778549));
#299795=CARTESIAN_POINT('Ctrl Pts',(-3.75838203887377,43.9249999998344,
-11.5671105274568));
#299796=CARTESIAN_POINT('Ctrl Pts',(-7.51676407774749,44.0749999998338,
-10.3459381770588));
#299797=CARTESIAN_POINT('Ctrl Pts',(-9.83957192047859,44.2249999998332,
-7.14886745759505));
#299798=CARTESIAN_POINT('Ctrl Pts',(-12.1623797632097,44.3749999998326,
-3.95179673813132));
#299799=CARTESIAN_POINT('Ctrl Pts',(-12.1623797632097,44.524999999832,2.97892388940585E-15));
#299800=CARTESIAN_POINT('Ctrl Pts',(-12.1623797632097,44.6749999998314,
3.95179673813133));
#299801=CARTESIAN_POINT('Ctrl Pts',(-9.83957192047859,44.8249999998308,
7.14886745759505));
#299802=CARTESIAN_POINT('Ctrl Pts',(-7.51676407774749,44.9749999998302,
10.3459381770588));
#299803=CARTESIAN_POINT('Ctrl Pts',(-3.75838203887376,45.1249999998296,
11.5671105274568));
#299804=CARTESIAN_POINT('Ctrl Pts',(-3.62024663897919E-14,45.274999999829,
12.7882828778549));
#299805=CARTESIAN_POINT('Ctrl Pts',(3.75838203887369,45.4249999998284,11.5671105274568));
#299806=CARTESIAN_POINT('Ctrl Pts',(7.51676407774742,45.5749999998278,10.3459381770588));
#299807=CARTESIAN_POINT('Ctrl Pts',(9.83957192047851,45.7249999998272,7.14886745759505));
#299808=CARTESIAN_POINT('Ctrl Pts',(12.1623797632096,45.8749999998266,3.95179673813132));
#299809=CARTESIAN_POINT('Ctrl Pts',(12.1623797632096,46.024999999826,-1.48946194470292E-15));
#299810=CARTESIAN_POINT('Ctrl Pts',(12.1623797632096,46.1749999998254,-3.95179673813132));
#299811=CARTESIAN_POINT('Ctrl Pts',(9.83957192047851,46.3249999998248,-7.14886745759505));
#299812=CARTESIAN_POINT('Ctrl Pts',(7.51676407774742,46.4749999998242,-10.3459381770588));
#299813=CARTESIAN_POINT('Ctrl Pts',(3.75838203887369,46.6249999998236,-11.5671105274568));
#299814=CARTESIAN_POINT('Ctrl Pts',(-4.0198546964214E-14,46.774999999823,
-12.7882828778549));
#299815=CARTESIAN_POINT('Ctrl Pts',(-3.75838203887377,46.9249999998224,
-11.5671105274568));
#299816=CARTESIAN_POINT('Ctrl Pts',(-7.5167640777475,47.0749999998218,-10.3459381770588));
#299817=CARTESIAN_POINT('Ctrl Pts',(-9.83957192047859,47.2249999998212,
-7.14886745759505));
#299818=CARTESIAN_POINT('Ctrl Pts',(-12.1623797632097,47.3749999998206,
-3.95179673813132));
#299819=CARTESIAN_POINT('Ctrl Pts',(-12.1623797632097,47.52499999982,2.97892388940585E-15));
#299820=CARTESIAN_POINT('Ctrl Pts',(-12.1623797632097,47.6749999998194,
3.95179673813133));
#299821=CARTESIAN_POINT('Ctrl Pts',(-9.83957192047859,47.8249999998188,
7.14886745759505));
#299822=CARTESIAN_POINT('Ctrl Pts',(-7.51676407774749,47.9749999998182,
10.3459381770588));
#299823=CARTESIAN_POINT('Ctrl Pts',(-3.75838203887377,48.1249999998176,
11.5671105274568));
#299824=CARTESIAN_POINT('Ctrl Pts',(-3.79301756614538E-14,48.274999999817,
12.7882828778549));
#299825=CARTESIAN_POINT('Ctrl Pts',(3.75838203887369,48.4249999998164,11.5671105274568));
#299826=CARTESIAN_POINT('Ctrl Pts',(7.51676407774742,48.5749999998158,10.3459381770588));
#299827=CARTESIAN_POINT('Ctrl Pts',(9.83957192047851,48.7249999998152,7.14886745759505));
#299828=CARTESIAN_POINT('Ctrl Pts',(12.1623797632096,48.8749999998146,3.95179673813132));
#299829=CARTESIAN_POINT('Ctrl Pts',(12.1623797632096,49.024999999814,-1.48946194470292E-15));
#299830=CARTESIAN_POINT('Ctrl Pts',(12.1623797632096,49.1749999998134,-3.95179673813132));
#299831=CARTESIAN_POINT('Ctrl Pts',(9.83957192047851,49.3249999998128,-7.14886745759505));
#299832=CARTESIAN_POINT('Ctrl Pts',(7.51676407774741,49.4749999998122,-10.3459381770588));
#299833=CARTESIAN_POINT('Ctrl Pts',(3.75838203887369,49.6249999998116,-11.5671105274568));
#299834=CARTESIAN_POINT('Ctrl Pts',(-4.19262562358759E-14,49.774999999811,
-12.7882828778549));
#299835=CARTESIAN_POINT('Ctrl Pts',(-3.75838203887377,49.9249999998104,
-11.5671105274568));
#299836=CARTESIAN_POINT('Ctrl Pts',(-7.5167640777475,50.0749999998098,-10.3459381770588));
#299837=CARTESIAN_POINT('Ctrl Pts',(-9.83957192047859,50.2249999998092,
-7.14886745759505));
#299838=CARTESIAN_POINT('Ctrl Pts',(-12.1623797632097,50.3749999998086,
-3.95179673813132));
#299839=CARTESIAN_POINT('Ctrl Pts',(-12.1623797632097,50.524999999808,2.97892388940585E-15));
#299840=CARTESIAN_POINT('Ctrl Pts',(-12.1623797632097,50.6749999998074,
3.95179673813133));
#299841=CARTESIAN_POINT('Ctrl Pts',(-9.83957192047859,50.8249999998068,
7.14886745759505));
#299842=CARTESIAN_POINT('Ctrl Pts',(-7.51676407774749,50.9749999998062,
10.3459381770588));
#299843=CARTESIAN_POINT('Ctrl Pts',(-3.75838203887377,51.1249999998056,
11.5671105274568));
#299844=CARTESIAN_POINT('Ctrl Pts',(-3.96578849331156E-14,51.274999999805,
12.7882828778549));
#299845=CARTESIAN_POINT('Ctrl Pts',(3.75838203887369,51.4249999998044,11.5671105274568));
#299846=CARTESIAN_POINT('Ctrl Pts',(7.51676407774742,51.5749999998038,10.3459381770588));
#299847=CARTESIAN_POINT('Ctrl Pts',(9.83957192047851,51.7249999998032,7.14886745759505));
#299848=CARTESIAN_POINT('Ctrl Pts',(12.1623797632096,51.8749999998026,3.95179673813132));
#299849=CARTESIAN_POINT('Ctrl Pts',(12.1623797632096,52.024999999802,-1.48946194470292E-15));
#299850=CARTESIAN_POINT('Ctrl Pts',(12.1623797632096,52.1749999998014,-3.95179673813132));
#299851=CARTESIAN_POINT('Ctrl Pts',(9.8395719204785,52.3249999998008,-7.14886745759505));
#299852=CARTESIAN_POINT('Ctrl Pts',(7.51676407774741,52.4749999998002,-10.3459381770588));
#299853=CARTESIAN_POINT('Ctrl Pts',(3.75838203887368,52.6249999997996,-11.5671105274568));
#299854=CARTESIAN_POINT('Ctrl Pts',(-4.36539655075377E-14,52.774999999799,
-12.7882828778549));
#299855=CARTESIAN_POINT('Ctrl Pts',(-3.75838203887377,52.9249999997984,
-11.5671105274568));
#299856=CARTESIAN_POINT('Ctrl Pts',(-7.5167640777475,53.0749999997978,-10.3459381770588));
#299857=CARTESIAN_POINT('Ctrl Pts',(-9.83957192047859,53.2249999997972,
-7.14886745759505));
#299858=CARTESIAN_POINT('Ctrl Pts',(-12.1623797632097,53.3749999997966,
-3.95179673813132));
#299859=CARTESIAN_POINT('Ctrl Pts',(-12.1623797632097,53.524999999796,2.97892388940585E-15));
#299860=CARTESIAN_POINT('Ctrl Pts',(-12.1623797632097,53.6749999997954,
3.95179673813133));
#299861=CARTESIAN_POINT('Ctrl Pts',(-9.83957192047859,53.8249999997948,
7.14886745759505));
#299862=CARTESIAN_POINT('Ctrl Pts',(-7.5167640777475,53.9749999997942,10.3459381770588));
#299863=CARTESIAN_POINT('Ctrl Pts',(-3.75838203887377,54.1249999997936,
11.5671105274568));
#299864=CARTESIAN_POINT('Ctrl Pts',(-4.13855942047774E-14,54.274999999793,
12.7882828778549));
#299865=CARTESIAN_POINT('Ctrl Pts',(3.75838203887369,54.4249999997924,11.5671105274568));
#299866=CARTESIAN_POINT('Ctrl Pts',(7.51676407774741,54.5749999997918,10.3459381770588));
#299867=CARTESIAN_POINT('Ctrl Pts',(9.8395719204785,54.7249999997912,7.14886745759505));
#299868=CARTESIAN_POINT('Ctrl Pts',(12.1623797632096,54.8749999997906,3.95179673813132));
#299869=CARTESIAN_POINT('Ctrl Pts',(12.1623797632096,55.02499999979,-1.48946194470292E-15));
#299870=CARTESIAN_POINT('Ctrl Pts',(12.1623797632096,55.1749999997894,-3.95179673813132));
#299871=CARTESIAN_POINT('Ctrl Pts',(9.8395719204785,55.3249999997888,-7.14886745759505));
#299872=CARTESIAN_POINT('Ctrl Pts',(7.51676407774741,55.4749999997882,-10.3459381770588));
#299873=CARTESIAN_POINT('Ctrl Pts',(3.75838203887368,55.6249999997876,-11.5671105274568));
#299874=CARTESIAN_POINT('Ctrl Pts',(-4.53816747791995E-14,55.774999999787,
-12.7882828778549));
#299875=CARTESIAN_POINT('Ctrl Pts',(-3.75838203887377,55.9249999997864,
-11.5671105274568));
#299876=CARTESIAN_POINT('Ctrl Pts',(-7.5167640777475,56.0749999997858,-10.3459381770588));
#299877=CARTESIAN_POINT('Ctrl Pts',(-9.83957192047859,56.2249999997852,
-7.14886745759505));
#299878=CARTESIAN_POINT('Ctrl Pts',(-12.1623797632097,56.3749999997846,
-3.95179673813132));
#299879=CARTESIAN_POINT('Ctrl Pts',(-12.1623797632097,56.524999999784,2.97892388940585E-15));
#299880=CARTESIAN_POINT('Ctrl Pts',(-12.1623797632097,56.6749999997834,
3.95179673813133));
#299881=CARTESIAN_POINT('Ctrl Pts',(-9.83957192047859,56.8249999997828,
7.14886745759505));
#299882=CARTESIAN_POINT('Ctrl Pts',(-7.5167640777475,56.9749999997822,10.3459381770588));
#299883=CARTESIAN_POINT('Ctrl Pts',(-3.75838203887377,57.1249999997816,
11.5671105274568));
#299884=CARTESIAN_POINT('Ctrl Pts',(-4.31133034764393E-14,57.274999999781,
12.7882828778549));
#299885=CARTESIAN_POINT('Ctrl Pts',(3.75838203887368,57.4249999997804,11.5671105274568));
#299886=CARTESIAN_POINT('Ctrl Pts',(7.51676407774741,57.5749999997798,10.3459381770588));
#299887=CARTESIAN_POINT('Ctrl Pts',(9.8395719204785,57.7249999997792,7.14886745759505));
#299888=CARTESIAN_POINT('Ctrl Pts',(12.1623797632096,57.8749999997786,3.95179673813132));
#299889=CARTESIAN_POINT('Ctrl Pts',(12.1623797632096,58.024999999778,-1.48946194470292E-15));
#299890=CARTESIAN_POINT('Ctrl Pts',(12.1623797632096,58.1749999997774,-3.95179673813132));
#299891=CARTESIAN_POINT('Ctrl Pts',(9.8395719204785,58.3249999997768,-7.14886745759505));
#299892=CARTESIAN_POINT('Ctrl Pts',(7.51676407774741,58.4749999997762,-10.3459381770588));
#299893=CARTESIAN_POINT('Ctrl Pts',(3.75838203887368,58.6249999997756,-11.5671105274568));
#299894=CARTESIAN_POINT('Ctrl Pts',(-4.71093840508614E-14,58.774999999775,
-12.7882828778549));
#299895=CARTESIAN_POINT('Ctrl Pts',(-3.75838203887377,58.9249999997744,
-11.5671105274568));
#299896=CARTESIAN_POINT('Ctrl Pts',(-7.5167640777475,59.0749999997738,-10.3459381770588));
#299897=CARTESIAN_POINT('Ctrl Pts',(-9.83957192047859,59.2249999997732,
-7.14886745759505));
#299898=CARTESIAN_POINT('Ctrl Pts',(-12.1623797632097,59.3749999997726,
-3.95179673813132));
#299899=CARTESIAN_POINT('Ctrl Pts',(-12.1623797632097,59.524999999772,2.97892388940585E-15));
#299900=CARTESIAN_POINT('Ctrl Pts',(-12.1623797632097,59.6749999997714,
3.95179673813133));
#299901=CARTESIAN_POINT('Ctrl Pts',(-9.83957192047859,59.8249999997708,
7.14886745759505));
#299902=CARTESIAN_POINT('Ctrl Pts',(-7.5167640777475,59.9749999997702,10.3459381770588));
#299903=CARTESIAN_POINT('Ctrl Pts',(-3.75838203887377,60.1249999997696,
11.5671105274568));
#299904=CARTESIAN_POINT('Ctrl Pts',(-4.48410127481011E-14,60.274999999769,
12.7882828778549));
#299905=CARTESIAN_POINT('Ctrl Pts',(3.75838203887368,60.4249999997684,11.5671105274568));
#299906=CARTESIAN_POINT('Ctrl Pts',(7.51676407774741,60.5749999997678,10.3459381770588));
#299907=CARTESIAN_POINT('Ctrl Pts',(9.8395719204785,60.7249999997672,7.14886745759505));
#299908=CARTESIAN_POINT('Ctrl Pts',(12.1623797632096,60.8749999997666,3.95179673813132));
#299909=CARTESIAN_POINT('Ctrl Pts',(12.1623797632096,61.024999999766,-1.48946194470292E-15));
#299910=CARTESIAN_POINT('Ctrl Pts',(12.1623797632096,61.1749999997654,-3.95179673813132));
#299911=CARTESIAN_POINT('Ctrl Pts',(9.8395719204785,61.3249999997648,-7.14886745759505));
#299912=CARTESIAN_POINT('Ctrl Pts',(7.51676407774741,61.4749999997642,-10.3459381770588));
#299913=CARTESIAN_POINT('Ctrl Pts',(3.75838203887368,61.6249999997636,-11.5671105274568));
#299914=CARTESIAN_POINT('Ctrl Pts',(-4.88370933225232E-14,61.774999999763,
-12.7882828778549));
#299915=CARTESIAN_POINT('Ctrl Pts',(-3.75838203887378,61.9249999997624,
-11.5671105274568));
#299916=CARTESIAN_POINT('Ctrl Pts',(-7.5167640777475,62.0749999997618,-10.3459381770588));
#299917=CARTESIAN_POINT('Ctrl Pts',(-9.8395719204786,62.2249999997612,-7.14886745759505));
#299918=CARTESIAN_POINT('Ctrl Pts',(-12.1623797632097,62.3749999997606,
-3.95179673813132));
#299919=CARTESIAN_POINT('Ctrl Pts',(-12.1623797632097,62.52499999976,2.97892388940585E-15));
#299920=CARTESIAN_POINT('Ctrl Pts',(-12.1623797632097,62.6749999997594,
3.95179673813133));
#299921=CARTESIAN_POINT('Ctrl Pts',(-9.8395719204786,62.8249999997588,7.14886745759505));
#299922=CARTESIAN_POINT('Ctrl Pts',(-7.5167640777475,62.9749999997582,10.3459381770588));
#299923=CARTESIAN_POINT('Ctrl Pts',(-3.75838203887377,63.1249999997576,
11.5671105274568));
#299924=CARTESIAN_POINT('Ctrl Pts',(-4.6568722019763E-14,63.274999999757,
12.7882828778549));
#299925=CARTESIAN_POINT('Ctrl Pts',(3.75838203887368,63.4249999997564,11.5671105274568));
#299926=CARTESIAN_POINT('Ctrl Pts',(7.51676407774741,63.5749999997558,10.3459381770588));
#299927=CARTESIAN_POINT('Ctrl Pts',(9.8395719204785,63.7249999997552,7.14886745759505));
#299928=CARTESIAN_POINT('Ctrl Pts',(12.1623797632096,63.8749999997546,3.95179673813132));
#299929=CARTESIAN_POINT('Ctrl Pts',(12.1623797632096,64.024999999754,-1.48946194470292E-15));
#299930=CARTESIAN_POINT('Ctrl Pts',(12.1623797632096,64.1749999997534,-3.95179673813132));
#299931=CARTESIAN_POINT('Ctrl Pts',(9.8395719204785,64.3249999997528,-7.14886745759505));
#299932=CARTESIAN_POINT('Ctrl Pts',(7.5167640777474,64.4749999997522,-10.3459381770588));
#299933=CARTESIAN_POINT('Ctrl Pts',(3.75838203887368,64.6249999997516,-11.5671105274568));
#299934=CARTESIAN_POINT('Ctrl Pts',(-5.05648025941851E-14,64.774999999751,
-12.7882828778549));
#299935=CARTESIAN_POINT('Ctrl Pts',(-3.75838203887378,64.9249999997504,
-11.5671105274568));
#299936=CARTESIAN_POINT('Ctrl Pts',(-7.51676407774751,65.0749999997498,
-10.3459381770588));
#299937=CARTESIAN_POINT('Ctrl Pts',(-9.8395719204786,65.2249999997492,-7.14886745759505));
#299938=CARTESIAN_POINT('Ctrl Pts',(-12.1623797632097,65.3749999997486,
-3.95179673813132));
#299939=CARTESIAN_POINT('Ctrl Pts',(-12.1623797632097,65.524999999748,2.97892388940585E-15));
#299940=CARTESIAN_POINT('Ctrl Pts',(-12.1623797632097,65.6749999997474,
3.95179673813133));
#299941=CARTESIAN_POINT('Ctrl Pts',(-9.8395719204786,65.8249999997468,7.14886745759505));
#299942=CARTESIAN_POINT('Ctrl Pts',(-7.5167640777475,65.9749999997462,10.3459381770588));
#299943=CARTESIAN_POINT('Ctrl Pts',(-3.75838203887378,66.1249999997456,
11.5671105274568));
#299944=CARTESIAN_POINT('Ctrl Pts',(-4.82964312914248E-14,66.274999999745,
12.7882828778549));
#299945=CARTESIAN_POINT('Ctrl Pts',(3.75838203887368,66.4249999997444,11.5671105274568));
#299946=CARTESIAN_POINT('Ctrl Pts',(7.51676407774741,66.5749999997438,10.3459381770588));
#299947=CARTESIAN_POINT('Ctrl Pts',(9.8395719204785,66.7249999997432,7.14886745759505));
#299948=CARTESIAN_POINT('Ctrl Pts',(12.1623797632096,66.8749999997426,3.95179673813132));
#299949=CARTESIAN_POINT('Ctrl Pts',(12.1623797632096,67.024999999742,-1.48946194470292E-15));
#299950=CARTESIAN_POINT('Ctrl Pts',(12.1623797632096,67.1749999997414,-3.95179673813132));
#299951=CARTESIAN_POINT('Ctrl Pts',(9.8395719204785,67.3249999997408,-7.14886745759505));
#299952=CARTESIAN_POINT('Ctrl Pts',(7.5167640777474,67.4749999997402,-10.3459381770588));
#299953=CARTESIAN_POINT('Ctrl Pts',(3.75838203887368,67.6249999997396,-11.5671105274568));
#299954=CARTESIAN_POINT('Ctrl Pts',(-5.22925118658469E-14,67.774999999739,
-12.7882828778549));
#299955=CARTESIAN_POINT('Ctrl Pts',(-3.75838203887378,67.9249999997384,
-11.5671105274568));
#299956=CARTESIAN_POINT('Ctrl Pts',(-7.51676407774751,68.0749999997378,
-10.3459381770588));
#299957=CARTESIAN_POINT('Ctrl Pts',(-9.8395719204786,68.2249999997372,-7.14886745759505));
#299958=CARTESIAN_POINT('Ctrl Pts',(-12.1623797632097,68.3749999997366,
-3.95179673813132));
#299959=CARTESIAN_POINT('Ctrl Pts',(-12.1623797632097,68.524999999736,2.97892388940585E-15));
#299960=CARTESIAN_POINT('Ctrl Pts',(-12.1623797632097,68.6749999997354,
3.95179673813133));
#299961=CARTESIAN_POINT('Ctrl Pts',(-9.8395719204786,68.8249999997348,7.14886745759505));
#299962=CARTESIAN_POINT('Ctrl Pts',(-7.51676407774751,68.9749999997342,
10.3459381770588));
#299963=CARTESIAN_POINT('Ctrl Pts',(-3.75838203887378,69.1249999997336,
11.5671105274568));
#299964=CARTESIAN_POINT('Ctrl Pts',(-5.00241405630866E-14,69.274999999733,
12.7882828778549));
#299965=CARTESIAN_POINT('Ctrl Pts',(3.75838203887368,69.4249999997324,11.5671105274568));
#299966=CARTESIAN_POINT('Ctrl Pts',(7.5167640777474,69.5749999997318,10.3459381770588));
#299967=CARTESIAN_POINT('Ctrl Pts',(9.8395719204785,69.7249999997312,7.14886745759505));
#299968=CARTESIAN_POINT('Ctrl Pts',(12.1623797632096,69.8749999997306,3.95179673813132));
#299969=CARTESIAN_POINT('Ctrl Pts',(12.1623797632096,70.02499999973,-1.48946194470292E-15));
#299970=CARTESIAN_POINT('Ctrl Pts',(12.1623797632096,70.1749999997294,-3.95179673813132));
#299971=CARTESIAN_POINT('Ctrl Pts',(9.83957192047849,70.3249999997288,-7.14886745759505));
#299972=CARTESIAN_POINT('Ctrl Pts',(7.5167640777474,70.4749999997282,-10.3459381770588));
#299973=CARTESIAN_POINT('Ctrl Pts',(3.75838203887367,70.6249999997276,-11.5671105274568));
#299974=CARTESIAN_POINT('Ctrl Pts',(-5.40202211375087E-14,70.774999999727,
-12.7882828778549));
#299975=CARTESIAN_POINT('Ctrl Pts',(-3.75838203887378,70.9249999997264,
-11.5671105274568));
#299976=CARTESIAN_POINT('Ctrl Pts',(-7.51676407774751,71.0749999997258,
-10.3459381770588));
#299977=CARTESIAN_POINT('Ctrl Pts',(-9.8395719204786,71.2249999997252,-7.14886745759505));
#299978=CARTESIAN_POINT('Ctrl Pts',(-12.1623797632097,71.3749999997246,
-3.95179673813132));
#299979=CARTESIAN_POINT('Ctrl Pts',(-12.1623797632097,71.524999999724,2.97892388940585E-15));
#299980=CARTESIAN_POINT('Ctrl Pts',(-12.1623797632097,71.6749999997234,
3.95179673813133));
#299981=CARTESIAN_POINT('Ctrl Pts',(-9.8395719204786,71.8249999997228,7.14886745759505));
#299982=CARTESIAN_POINT('Ctrl Pts',(-7.51676407774751,71.9749999997222,
10.3459381770588));
#299983=CARTESIAN_POINT('Ctrl Pts',(-3.75838203887378,72.1249999997216,
11.5671105274568));
#299984=CARTESIAN_POINT('Ctrl Pts',(-5.17518498347485E-14,72.274999999721,
12.7882828778549));
#299985=CARTESIAN_POINT('Ctrl Pts',(3.75838203887368,72.4249999997204,11.5671105274568));
#299986=CARTESIAN_POINT('Ctrl Pts',(7.5167640777474,72.5749999997198,10.3459381770588));
#299987=CARTESIAN_POINT('Ctrl Pts',(9.83957192047849,72.7249999997192,7.14886745759505));
#299988=CARTESIAN_POINT('Ctrl Pts',(12.1623797632096,72.8749999997186,3.95179673813132));
#299989=CARTESIAN_POINT('Ctrl Pts',(12.1623797632096,73.024999999718,-1.48946194470292E-15));
#299990=CARTESIAN_POINT('Ctrl Pts',(12.1623797632096,73.1749999997174,-3.95179673813132));
#299991=CARTESIAN_POINT('Ctrl Pts',(9.83957192047849,73.3249999997168,-7.14886745759505));
#299992=CARTESIAN_POINT('Ctrl Pts',(7.5167640777474,73.4749999997162,-10.3459381770588));
#299993=CARTESIAN_POINT('Ctrl Pts',(3.75838203887367,73.6249999997156,-11.5671105274568));
#299994=CARTESIAN_POINT('Ctrl Pts',(-5.57479304091706E-14,73.774999999715,
-12.7882828778549));
#299995=CARTESIAN_POINT('Ctrl Pts',(-3.75838203887378,73.9249999997144,
-11.5671105274568));
#299996=CARTESIAN_POINT('Ctrl Pts',(-7.51676407774751,74.0749999997138,
-10.3459381770588));
#299997=CARTESIAN_POINT('Ctrl Pts',(-9.8395719204786,74.2249999997132,-7.14886745759505));
#299998=CARTESIAN_POINT('Ctrl Pts',(-12.1623797632097,74.3749999997126,
-3.95179673813132));
#299999=CARTESIAN_POINT('Ctrl Pts',(-12.1623797632097,74.524999999712,2.97892388940585E-15));
#300000=CARTESIAN_POINT('Ctrl Pts',(-12.1623797632097,74.6749999997114,
3.95179673813133));
#300001=CARTESIAN_POINT('Ctrl Pts',(-9.8395719204786,74.8249999997108,7.14886745759505));
#300002=CARTESIAN_POINT('Ctrl Pts',(-7.51676407774751,74.9749999997102,
10.3459381770588));
#300003=CARTESIAN_POINT('Ctrl Pts',(-3.75838203887378,75.1249999997096,
11.5671105274568));
#300004=CARTESIAN_POINT('Ctrl Pts',(-5.34795591064103E-14,75.274999999709,
12.7882828778549));
#300005=CARTESIAN_POINT('Ctrl Pts',(3.75838203887367,75.4249999997084,11.5671105274568));
#300006=CARTESIAN_POINT('Ctrl Pts',(7.5167640777474,75.5749999997078,10.3459381770588));
#300007=CARTESIAN_POINT('Ctrl Pts',(9.83957192047849,75.7249999997072,7.14886745759505));
#300008=CARTESIAN_POINT('Ctrl Pts',(12.1623797632096,75.8749999997066,3.95179673813132));
#300009=CARTESIAN_POINT('Ctrl Pts',(12.1623797632096,76.024999999706,-1.48946194470292E-15));
#300010=CARTESIAN_POINT('Ctrl Pts',(12.1623797632096,76.1749999997054,-3.95179673813132));
#300011=CARTESIAN_POINT('Ctrl Pts',(9.83957192047849,76.3249999997048,-7.14886745759505));
#300012=CARTESIAN_POINT('Ctrl Pts',(7.5167640777474,76.4749999997042,-10.3459381770588));
#300013=CARTESIAN_POINT('Ctrl Pts',(3.75838203887367,76.6249999997036,-11.5671105274568));
#300014=CARTESIAN_POINT('Ctrl Pts',(-5.74756396808324E-14,76.774999999703,
-12.7882828778549));
#300015=CARTESIAN_POINT('Ctrl Pts',(-3.75838203887379,76.9249999997024,
-11.5671105274568));
#300016=CARTESIAN_POINT('Ctrl Pts',(-7.51676407774751,77.0749999997018,
-10.3459381770588));
#300017=CARTESIAN_POINT('Ctrl Pts',(-9.8395719204786,77.2249999997012,-7.14886745759505));
#300018=CARTESIAN_POINT('Ctrl Pts',(-12.1623797632097,77.3749999997006,
-3.95179673813132));
#300019=CARTESIAN_POINT('Ctrl Pts',(-12.1623797632097,77.5249999997,2.97892388940585E-15));
#300020=CARTESIAN_POINT('Ctrl Pts',(-12.1623797632097,77.6749999996994,
3.95179673813133));
#300021=CARTESIAN_POINT('Ctrl Pts',(-9.8395719204786,77.8249999996988,7.14886745759505));
#300022=CARTESIAN_POINT('Ctrl Pts',(-7.51676407774751,77.9749999996982,
10.3459381770588));
#300023=CARTESIAN_POINT('Ctrl Pts',(-3.75838203887378,78.1249999996976,
11.5671105274568));
#300024=CARTESIAN_POINT('Ctrl Pts',(-5.52072683780721E-14,78.274999999697,
12.7882828778549));
#300025=CARTESIAN_POINT('Ctrl Pts',(3.75838203887367,78.4249999996964,11.5671105274568));
#300026=CARTESIAN_POINT('Ctrl Pts',(7.5167640777474,78.5749999996958,10.3459381770588));
#300027=CARTESIAN_POINT('Ctrl Pts',(9.83957192047849,78.7249999996952,7.14886745759505));
#300028=CARTESIAN_POINT('Ctrl Pts',(12.1623797632096,78.8749999996946,3.95179673813132));
#300029=CARTESIAN_POINT('Ctrl Pts',(12.1623797632096,79.024999999694,-1.48946194470292E-15));
#300030=CARTESIAN_POINT('Ctrl Pts',(12.1623797632096,79.1749999996934,-3.95179673813132));
#300031=CARTESIAN_POINT('Ctrl Pts',(9.83957192047849,79.3249999996928,-7.14886745759505));
#300032=CARTESIAN_POINT('Ctrl Pts',(7.5167640777474,79.4749999996922,-10.3459381770588));
#300033=CARTESIAN_POINT('Ctrl Pts',(3.75838203887367,79.6249999996916,-11.5671105274568));
#300034=CARTESIAN_POINT('Ctrl Pts',(-5.92033489524943E-14,79.774999999691,
-12.7882828778549));
#300035=CARTESIAN_POINT('Ctrl Pts',(-3.75838203887379,79.9249999996904,
-11.5671105274568));
#300036=CARTESIAN_POINT('Ctrl Pts',(-7.51676407774751,80.0749999996898,
-10.3459381770588));
#300037=CARTESIAN_POINT('Ctrl Pts',(-9.83957192047861,80.2249999996892,
-7.14886745759505));
#300038=CARTESIAN_POINT('Ctrl Pts',(-12.1623797632097,80.3749999996886,
-3.95179673813132));
#300039=CARTESIAN_POINT('Ctrl Pts',(-12.1623797632097,80.524999999688,2.97892388940585E-15));
#300040=CARTESIAN_POINT('Ctrl Pts',(-12.1623797632097,80.6749999996874,
3.95179673813133));
#300041=CARTESIAN_POINT('Ctrl Pts',(-9.83957192047861,80.8249999996868,
7.14886745759505));
#300042=CARTESIAN_POINT('Ctrl Pts',(-7.51676407774751,80.9749999996862,
10.3459381770588));
#300043=CARTESIAN_POINT('Ctrl Pts',(-3.75838203887378,81.1249999996856,
11.5671105274568));
#300044=CARTESIAN_POINT('Ctrl Pts',(-5.6934977649734E-14,81.274999999685,
12.7882828778549));
#300045=CARTESIAN_POINT('Ctrl Pts',(3.75838203887367,81.4249999996844,11.5671105274568));
#300046=CARTESIAN_POINT('Ctrl Pts',(7.5167640777474,81.5749999996838,10.3459381770588));
#300047=CARTESIAN_POINT('Ctrl Pts',(9.83957192047849,81.7249999996832,7.14886745759505));
#300048=CARTESIAN_POINT('Ctrl Pts',(12.1623797632096,81.8749999996826,3.95179673813132));
#300049=CARTESIAN_POINT('Ctrl Pts',(12.1623797632096,82.024999999682,-1.48946194470292E-15));
#300050=CARTESIAN_POINT('Ctrl Pts',(12.1623797632096,82.1749999996814,-3.95179673813132));
#300051=CARTESIAN_POINT('Ctrl Pts',(9.83957192047849,82.3249999996808,-7.14886745759505));
#300052=CARTESIAN_POINT('Ctrl Pts',(7.5167640777474,82.4749999996802,-10.3459381770588));
#300053=CARTESIAN_POINT('Ctrl Pts',(3.75838203887367,82.6249999996796,-11.5671105274568));
#300054=CARTESIAN_POINT('Ctrl Pts',(-6.09310582241561E-14,82.774999999679,
-12.7882828778549));
#300055=CARTESIAN_POINT('Ctrl Pts',(-3.75838203887379,82.9249999996784,
-11.5671105274568));
#300056=CARTESIAN_POINT('Ctrl Pts',(-7.51676407774752,83.0749999996778,
-10.3459381770588));
#300057=CARTESIAN_POINT('Ctrl Pts',(-9.83957192047861,83.2249999996772,
-7.14886745759505));
#300058=CARTESIAN_POINT('Ctrl Pts',(-12.1623797632097,83.3749999996766,
-3.95179673813132));
#300059=CARTESIAN_POINT('Ctrl Pts',(-12.1623797632097,83.524999999676,2.97892388940585E-15));
#300060=CARTESIAN_POINT('Ctrl Pts',(-12.1623797632097,83.6749999996754,
3.95179673813133));
#300061=CARTESIAN_POINT('Ctrl Pts',(-9.83957192047861,83.8249999996748,
7.14886745759505));
#300062=CARTESIAN_POINT('Ctrl Pts',(-7.51676407774751,83.9749999996742,
10.3459381770588));
#300063=CARTESIAN_POINT('Ctrl Pts',(-3.75838203887379,84.1249999996736,
11.5671105274568));
#300064=CARTESIAN_POINT('Ctrl Pts',(-5.86626869213958E-14,84.274999999673,
12.7882828778549));
#300065=CARTESIAN_POINT('Ctrl Pts',(3.75838203887367,84.4249999996724,11.5671105274568));
#300066=CARTESIAN_POINT('Ctrl Pts',(7.5167640777474,84.5749999996718,10.3459381770588));
#300067=CARTESIAN_POINT('Ctrl Pts',(9.83957192047849,84.7249999996712,7.14886745759505));
#300068=CARTESIAN_POINT('Ctrl Pts',(12.1623797632096,84.8749999996706,3.95179673813132));
#300069=CARTESIAN_POINT('Ctrl Pts',(12.1623797632096,85.02499999967,-1.48946194470292E-15));
#300070=CARTESIAN_POINT('Ctrl Pts',(12.1623797632096,85.1749999996694,-3.95179673813132));
#300071=CARTESIAN_POINT('Ctrl Pts',(9.83957192047849,85.3249999996688,-7.14886745759505));
#300072=CARTESIAN_POINT('Ctrl Pts',(7.51676407774739,85.4749999996682,-10.3459381770588));
#300073=CARTESIAN_POINT('Ctrl Pts',(3.75838203887367,85.6249999996676,-11.5671105274568));
#300074=CARTESIAN_POINT('Ctrl Pts',(-6.26587674958179E-14,85.774999999667,
-12.7882828778549));
#300075=CARTESIAN_POINT('Ctrl Pts',(-3.75838203887379,85.9249999996664,
-11.5671105274568));
#300076=CARTESIAN_POINT('Ctrl Pts',(-7.51676407774752,86.0749999996658,
-10.3459381770588));
#300077=CARTESIAN_POINT('Ctrl Pts',(-9.83957192047861,86.2249999996652,
-7.14886745759505));
#300078=CARTESIAN_POINT('Ctrl Pts',(-12.1623797632097,86.3749999996646,
-3.95179673813132));
#300079=CARTESIAN_POINT('Ctrl Pts',(-12.1623797632097,86.524999999664,2.97892388940585E-15));
#300080=CARTESIAN_POINT('Ctrl Pts',(-12.1623797632097,86.6749999996634,
3.95179673813133));
#300081=CARTESIAN_POINT('Ctrl Pts',(-9.83957192047861,86.8249999996628,
7.14886745759505));
#300082=CARTESIAN_POINT('Ctrl Pts',(-7.51676407774752,86.9749999996622,
10.3459381770588));
#300083=CARTESIAN_POINT('Ctrl Pts',(-3.75838203887379,87.1249999996616,
11.5671105274568));
#300084=CARTESIAN_POINT('Ctrl Pts',(-6.03903961930577E-14,87.274999999661,
12.7882828778549));
#300085=CARTESIAN_POINT('Ctrl Pts',(3.75838203887367,87.4249999996604,11.5671105274568));
#300086=CARTESIAN_POINT('Ctrl Pts',(7.5167640777474,87.5749999996598,10.3459381770588));
#300087=CARTESIAN_POINT('Ctrl Pts',(9.83957192047849,87.7249999996592,7.14886745759505));
#300088=CARTESIAN_POINT('Ctrl Pts',(12.1623797632096,87.8749999996586,3.95179673813132));
#300089=CARTESIAN_POINT('Ctrl Pts',(12.1623797632096,88.024999999658,-1.48946194470292E-15));
#300090=CARTESIAN_POINT('Ctrl Pts',(12.1623797632096,88.1749999996574,-3.95179673813132));
#300091=CARTESIAN_POINT('Ctrl Pts',(9.83957192047849,88.3249999996568,-7.14886745759505));
#300092=CARTESIAN_POINT('Ctrl Pts',(7.51676407774739,88.4749999996562,-10.3459381770588));
#300093=CARTESIAN_POINT('Ctrl Pts',(3.75838203887366,88.6249999996556,-11.5671105274568));
#300094=CARTESIAN_POINT('Ctrl Pts',(-6.43864767674798E-14,88.774999999655,
-12.7882828778549));
#300095=CARTESIAN_POINT('Ctrl Pts',(-3.75838203887379,88.9249999996544,
-11.5671105274568));
#300096=CARTESIAN_POINT('Ctrl Pts',(-7.51676407774752,89.0749999996538,
-10.3459381770588));
#300097=CARTESIAN_POINT('Ctrl Pts',(-9.83957192047861,89.2249999996532,
-7.14886745759505));
#300098=CARTESIAN_POINT('Ctrl Pts',(-12.1623797632097,89.3749999996526,
-3.95179673813132));
#300099=CARTESIAN_POINT('Ctrl Pts',(-12.1623797632097,89.524999999652,2.97892388940585E-15));
#300100=CARTESIAN_POINT('Ctrl Pts',(-12.1623797632097,89.6749999996514,
3.95179673813133));
#300101=CARTESIAN_POINT('Ctrl Pts',(-9.83957192047861,89.8249999996508,
7.14886745759505));
#300102=CARTESIAN_POINT('Ctrl Pts',(-7.51676407774752,89.9749999996502,
10.3459381770588));
#300103=CARTESIAN_POINT('Ctrl Pts',(-3.75838203887379,90.1249999996496,
11.5671105274568));
#300104=CARTESIAN_POINT('Ctrl Pts',(-6.21181054647195E-14,90.274999999649,
12.7882828778549));
#300105=CARTESIAN_POINT('Ctrl Pts',(3.75838203887366,90.4249999996484,11.5671105274568));
#300106=CARTESIAN_POINT('Ctrl Pts',(7.51676407774739,90.5749999996478,10.3459381770588));
#300107=CARTESIAN_POINT('Ctrl Pts',(9.83957192047848,90.7249999996472,7.14886745759505));
#300108=CARTESIAN_POINT('Ctrl Pts',(12.1623797632096,90.8749999996466,3.95179673813132));
#300109=CARTESIAN_POINT('Ctrl Pts',(12.1623797632096,91.024999999646,-1.48946194470292E-15));
#300110=CARTESIAN_POINT('Ctrl Pts',(12.1623797632096,91.1749999996454,-3.95179673813132));
#300111=CARTESIAN_POINT('Ctrl Pts',(9.83957192047848,91.3249999996448,-7.14886745759505));
#300112=CARTESIAN_POINT('Ctrl Pts',(7.51676407774739,91.4749999996442,-10.3459381770588));
#300113=CARTESIAN_POINT('Ctrl Pts',(3.75838203887366,91.6249999996436,-11.5671105274568));
#300114=CARTESIAN_POINT('Ctrl Pts',(-6.61141860391416E-14,91.774999999643,
-12.7882828778549));
#300115=CARTESIAN_POINT('Ctrl Pts',(-3.75838203887379,91.9249999996424,
-11.5671105274568));
#300116=CARTESIAN_POINT('Ctrl Pts',(-7.51676407774752,92.0749999996418,
-10.3459381770588));
#300117=CARTESIAN_POINT('Ctrl Pts',(-9.83957192047861,92.2249999996412,
-7.14886745759505));
#300118=CARTESIAN_POINT('Ctrl Pts',(-12.1623797632097,92.3749999996406,
-3.95179673813132));
#300119=CARTESIAN_POINT('Ctrl Pts',(-12.1623797632097,92.52499999964,2.97892388940585E-15));
#300120=CARTESIAN_POINT('Ctrl Pts',(-12.1623797632097,92.6749999996394,
3.95179673813133));
#300121=CARTESIAN_POINT('Ctrl Pts',(-9.83957192047861,92.8249999996388,
7.14886745759505));
#300122=CARTESIAN_POINT('Ctrl Pts',(-7.51676407774752,92.9749999996382,
10.3459381770588));
#300123=CARTESIAN_POINT('Ctrl Pts',(-3.75838203887379,93.1249999996376,
11.5671105274568));
#300124=CARTESIAN_POINT('Ctrl Pts',(-6.38458147363813E-14,93.274999999637,
12.7882828778549));
#300125=CARTESIAN_POINT('Ctrl Pts',(3.75838203887366,93.4249999996364,11.5671105274568));
#300126=CARTESIAN_POINT('Ctrl Pts',(7.51676407774739,93.5749999996358,10.3459381770588));
#300127=CARTESIAN_POINT('Ctrl Pts',(9.83957192047848,93.7249999996352,7.14886745759505));
#300128=CARTESIAN_POINT('Ctrl Pts',(12.1623797632096,93.8749999996346,3.95179673813132));
#300129=CARTESIAN_POINT('Ctrl Pts',(12.1623797632096,94.024999999634,-1.48946194470292E-15));
#300130=CARTESIAN_POINT('Ctrl Pts',(12.1623797632096,94.1749999996334,-3.95179673813132));
#300131=CARTESIAN_POINT('Ctrl Pts',(9.83957192047848,94.3249999996328,-7.14886745759505));
#300132=CARTESIAN_POINT('Ctrl Pts',(7.51676407774739,94.4749999996322,-10.3459381770588));
#300133=CARTESIAN_POINT('Ctrl Pts',(3.75838203887366,94.6249999996316,-11.5671105274568));
#300134=CARTESIAN_POINT('Ctrl Pts',(-6.78418953108034E-14,94.774999999631,
-12.7882828778549));
#300135=CARTESIAN_POINT('Ctrl Pts',(-3.7583820388738,94.9249999996304,-11.5671105274568));
#300136=CARTESIAN_POINT('Ctrl Pts',(-7.51676407774752,95.0749999996298,
-10.3459381770588));
#300137=CARTESIAN_POINT('Ctrl Pts',(-9.83957192047862,95.2249999996292,
-7.14886745759505));
#300138=CARTESIAN_POINT('Ctrl Pts',(-12.1623797632097,95.3749999996286,
-3.95179673813132));
#300139=CARTESIAN_POINT('Ctrl Pts',(-12.1623797632097,95.524999999628,2.97892388940585E-15));
#300140=CARTESIAN_POINT('Ctrl Pts',(-12.1623797632097,95.6749999996274,
3.95179673813133));
#300141=CARTESIAN_POINT('Ctrl Pts',(-9.83957192047862,95.8249999996268,
7.14886745759505));
#300142=CARTESIAN_POINT('Ctrl Pts',(-7.51676407774752,95.9749999996262,
10.3459381770588));
#300143=CARTESIAN_POINT('Ctrl Pts',(-3.75838203887379,96.1249999996256,
11.5671105274568));
#300144=CARTESIAN_POINT('Ctrl Pts',(-6.55735240080432E-14,96.274999999625,
12.7882828778549));
#300145=CARTESIAN_POINT('Ctrl Pts',(3.75838203887366,96.4249999996244,11.5671105274568));
#300146=CARTESIAN_POINT('Ctrl Pts',(7.51676407774739,96.5749999996238,10.3459381770588));
#300147=CARTESIAN_POINT('Ctrl Pts',(9.83957192047848,96.7249999996232,7.14886745759505));
#300148=CARTESIAN_POINT('Ctrl Pts',(12.1623797632096,96.8749999996226,3.95179673813132));
#300149=CARTESIAN_POINT('Ctrl Pts',(12.1623797632096,97.024999999622,-1.48946194470292E-15));
#300150=CARTESIAN_POINT('Ctrl Pts',(12.1623797632096,97.1749999996214,-3.95179673813132));
#300151=CARTESIAN_POINT('Ctrl Pts',(9.83957192047848,97.3249999996208,-7.14886745759505));
#300152=CARTESIAN_POINT('Ctrl Pts',(7.51676407774739,97.4749999996202,-10.3459381770588));
#300153=CARTESIAN_POINT('Ctrl Pts',(3.75838203887366,97.6249999996196,-11.5671105274568));
#300154=CARTESIAN_POINT('Ctrl Pts',(-6.95696045824653E-14,97.774999999619,
-12.7882828778549));
#300155=CARTESIAN_POINT('Ctrl Pts',(-3.7583820388738,97.9249999996184,-11.5671105274568));
#300156=CARTESIAN_POINT('Ctrl Pts',(-7.51676407774752,98.0749999996178,
-10.3459381770588));
#300157=CARTESIAN_POINT('Ctrl Pts',(-9.83957192047862,98.2249999996172,
-7.14886745759505));
#300158=CARTESIAN_POINT('Ctrl Pts',(-12.1623797632097,98.3749999996166,
-3.95179673813132));
#300159=CARTESIAN_POINT('Ctrl Pts',(-12.1623797632097,98.524999999616,2.97892388940585E-15));
#300160=CARTESIAN_POINT('Ctrl Pts',(-12.1623797632097,98.6749999996154,
3.95179673813133));
#300161=CARTESIAN_POINT('Ctrl Pts',(-9.83957192047862,98.8249999996148,
7.14886745759505));
#300162=CARTESIAN_POINT('Ctrl Pts',(-7.51676407774752,98.9749999996142,
10.3459381770588));
#300163=CARTESIAN_POINT('Ctrl Pts',(-3.7583820388738,99.1249999996136,11.5671105274568));
#300164=CARTESIAN_POINT('Ctrl Pts',(-6.7301233279705E-14,99.274999999613,
12.7882828778549));
#300165=CARTESIAN_POINT('Ctrl Pts',(3.75838203887366,99.4249999996124,11.5671105274568));
#300166=CARTESIAN_POINT('Ctrl Pts',(7.51676407774739,99.5749999996118,10.3459381770588));
#300167=CARTESIAN_POINT('Ctrl Pts',(9.83957192047848,99.7249999996112,7.14886745759505));
#300168=CARTESIAN_POINT('Ctrl Pts',(12.1623797632096,99.8749999996106,3.95179673813132));
#300169=CARTESIAN_POINT('Ctrl Pts',(12.1623797632096,100.02499999961,-1.48946194470292E-15));
#300170=CARTESIAN_POINT('Ctrl Pts',(12.1623797632096,100.174999999609,-3.95179673813132));
#300171=CARTESIAN_POINT('Ctrl Pts',(9.83957192047848,100.324999999609,-7.14886745759505));
#300172=CARTESIAN_POINT('Ctrl Pts',(7.51676407774738,100.474999999608,-10.3459381770588));
#300173=CARTESIAN_POINT('Ctrl Pts',(3.75838203887366,100.624999999608,-11.5671105274568));
#300174=CARTESIAN_POINT('Ctrl Pts',(-7.12973138541271E-14,100.774999999607,
-12.7882828778549));
#300175=CARTESIAN_POINT('Ctrl Pts',(-3.7583820388738,100.924999999606,-11.5671105274568));
#300176=CARTESIAN_POINT('Ctrl Pts',(-7.51676407774753,101.074999999606,
-10.3459381770588));
#300177=CARTESIAN_POINT('Ctrl Pts',(-9.83957192047862,101.224999999605,
-7.14886745759505));
#300178=CARTESIAN_POINT('Ctrl Pts',(-12.1623797632097,101.374999999605,
-3.95179673813132));
#300179=CARTESIAN_POINT('Ctrl Pts',(-12.1623797632097,101.524999999604,
2.97892388940585E-15));
#300180=CARTESIAN_POINT('Ctrl Pts',(-12.1623797632097,101.674999999603,
3.95179673813133));
#300181=CARTESIAN_POINT('Ctrl Pts',(-9.83957192047862,101.824999999603,
7.14886745759505));
#300182=CARTESIAN_POINT('Ctrl Pts',(-7.51676407774752,101.974999999602,
10.3459381770588));
#300183=CARTESIAN_POINT('Ctrl Pts',(-3.7583820388738,102.124999999602,11.5671105274568));
#300184=CARTESIAN_POINT('Ctrl Pts',(-6.90289425513669E-14,102.274999999601,
12.7882828778549));
#300185=CARTESIAN_POINT('Ctrl Pts',(3.75838203887366,102.4249999996,11.5671105274568));
#300186=CARTESIAN_POINT('Ctrl Pts',(7.51676407774739,102.5749999996,10.3459381770588));
#300187=CARTESIAN_POINT('Ctrl Pts',(9.83957192047848,102.724999999599,7.14886745759505));
#300188=CARTESIAN_POINT('Ctrl Pts',(12.1623797632096,102.874999999599,3.95179673813132));
#300189=CARTESIAN_POINT('Ctrl Pts',(12.1623797632096,103.024999999598,-1.48946194470292E-15));
#300190=CARTESIAN_POINT('Ctrl Pts',(12.1623797632096,103.174999999597,-3.95179673813132));
#300191=CARTESIAN_POINT('Ctrl Pts',(9.83957192047848,103.324999999597,-7.14886745759505));
#300192=CARTESIAN_POINT('Ctrl Pts',(7.51676407774738,103.474999999596,-10.3459381770588));
#300193=CARTESIAN_POINT('Ctrl Pts',(3.75838203887366,103.624999999596,-11.5671105274568));
#300194=CARTESIAN_POINT('Ctrl Pts',(-7.3025023125789E-14,103.774999999595,
-12.7882828778549));
#300195=CARTESIAN_POINT('Ctrl Pts',(-3.7583820388738,103.924999999594,-11.5671105274568));
#300196=CARTESIAN_POINT('Ctrl Pts',(-7.51676407774753,104.074999999594,
-10.3459381770588));
#300197=CARTESIAN_POINT('Ctrl Pts',(-9.83957192047862,104.224999999593,
-7.14886745759505));
#300198=CARTESIAN_POINT('Ctrl Pts',(-12.1623797632097,104.374999999593,
-3.95179673813132));
#300199=CARTESIAN_POINT('Ctrl Pts',(-12.1623797632097,104.524999999592,
2.97892388940585E-15));
#300200=CARTESIAN_POINT('Ctrl Pts',(-12.1623797632097,104.674999999591,
3.95179673813133));
#300201=CARTESIAN_POINT('Ctrl Pts',(-9.83957192047862,104.824999999591,
7.14886745759505));
#300202=CARTESIAN_POINT('Ctrl Pts',(-7.51676407774753,104.97499999959,10.3459381770588));
#300203=CARTESIAN_POINT('Ctrl Pts',(-3.7583820388738,105.12499999959,11.5671105274568));
#300204=CARTESIAN_POINT('Ctrl Pts',(-7.07566518230287E-14,105.274999999589,
12.7882828778549));
#300205=CARTESIAN_POINT('Ctrl Pts',(3.75838203887366,105.424999999588,11.5671105274568));
#300206=CARTESIAN_POINT('Ctrl Pts',(7.51676407774738,105.574999999588,10.3459381770588));
#300207=CARTESIAN_POINT('Ctrl Pts',(9.83957192047848,105.724999999587,7.14886745759505));
#300208=CARTESIAN_POINT('Ctrl Pts',(12.1623797632096,105.874999999587,3.95179673813132));
#300209=CARTESIAN_POINT('Ctrl Pts',(12.1623797632096,106.024999999586,-1.48946194470292E-15));
#300210=CARTESIAN_POINT('Ctrl Pts',(12.1623797632096,106.174999999585,-3.95179673813132));
#300211=CARTESIAN_POINT('Ctrl Pts',(9.83957192047848,106.324999999585,-7.14886745759505));
#300212=CARTESIAN_POINT('Ctrl Pts',(7.51676407774738,106.474999999584,-10.3459381770588));
#300213=CARTESIAN_POINT('Ctrl Pts',(3.75838203887365,106.624999999584,-11.5671105274568));
#300214=CARTESIAN_POINT('Ctrl Pts',(-7.47527323974508E-14,106.774999999583,
-12.7882828778549));
#300215=CARTESIAN_POINT('Ctrl Pts',(-3.7583820388738,106.924999999582,-11.5671105274568));
#300216=CARTESIAN_POINT('Ctrl Pts',(-7.51676407774753,107.074999999582,
-10.3459381770588));
#300217=CARTESIAN_POINT('Ctrl Pts',(-9.83957192047862,107.224999999581,
-7.14886745759505));
#300218=CARTESIAN_POINT('Ctrl Pts',(-12.1623797632097,107.374999999581,
-3.95179673813132));
#300219=CARTESIAN_POINT('Ctrl Pts',(-12.1623797632097,107.52499999958,2.97892388940585E-15));
#300220=CARTESIAN_POINT('Ctrl Pts',(-12.1623797632097,107.674999999579,
3.95179673813133));
#300221=CARTESIAN_POINT('Ctrl Pts',(-9.83957192047862,107.824999999579,
7.14886745759505));
#300222=CARTESIAN_POINT('Ctrl Pts',(-7.51676407774753,107.974999999578,
10.3459381770588));
#300223=CARTESIAN_POINT('Ctrl Pts',(-3.7583820388738,108.124999999578,11.5671105274568));
#300224=CARTESIAN_POINT('Ctrl Pts',(-7.24843610946905E-14,108.274999999577,
12.7882828778549));
#300225=CARTESIAN_POINT('Ctrl Pts',(3.75838203887366,108.424999999576,11.5671105274568));
#300226=CARTESIAN_POINT('Ctrl Pts',(7.51676407774738,108.574999999576,10.3459381770588));
#300227=CARTESIAN_POINT('Ctrl Pts',(9.83957192047847,108.724999999575,7.14886745759505));
#300228=CARTESIAN_POINT('Ctrl Pts',(12.1623797632096,108.874999999575,3.95179673813132));
#300229=CARTESIAN_POINT('Ctrl Pts',(12.1623797632096,109.024999999574,-1.48946194470292E-15));
#300230=CARTESIAN_POINT('Ctrl Pts',(12.1623797632096,109.174999999573,-3.95179673813132));
#300231=CARTESIAN_POINT('Ctrl Pts',(9.83957192047847,109.324999999573,-7.14886745759505));
#300232=CARTESIAN_POINT('Ctrl Pts',(7.51676407774738,109.474999999572,-10.3459381770588));
#300233=CARTESIAN_POINT('Ctrl Pts',(3.75838203887365,109.624999999572,-11.5671105274568));
#300234=CARTESIAN_POINT('Ctrl Pts',(-7.64804416691126E-14,109.774999999571,
-12.7882828778549));
#300235=CARTESIAN_POINT('Ctrl Pts',(-3.7583820388738,109.92499999957,-11.5671105274568));
#300236=CARTESIAN_POINT('Ctrl Pts',(-7.51676407774753,110.07499999957,-10.3459381770588));
#300237=CARTESIAN_POINT('Ctrl Pts',(-9.83957192047862,110.224999999569,
-7.14886745759505));
#300238=CARTESIAN_POINT('Ctrl Pts',(-12.1623797632097,110.374999999569,
-3.95179673813132));
#300239=CARTESIAN_POINT('Ctrl Pts',(-12.1623797632097,110.524999999568,
2.97892388940585E-15));
#300240=CARTESIAN_POINT('Ctrl Pts',(-12.1623797632097,110.674999999567,
3.95179673813133));
#300241=CARTESIAN_POINT('Ctrl Pts',(-9.83957192047862,110.824999999567,
7.14886745759505));
#300242=CARTESIAN_POINT('Ctrl Pts',(-7.51676407774753,110.974999999566,
10.3459381770588));
#300243=CARTESIAN_POINT('Ctrl Pts',(-3.7583820388738,111.124999999566,11.5671105274568));
#300244=CARTESIAN_POINT('Ctrl Pts',(-7.42120703663524E-14,111.274999999565,
12.7882828778549));
#300245=CARTESIAN_POINT('Ctrl Pts',(3.75838203887365,111.424999999564,11.5671105274568));
#300246=CARTESIAN_POINT('Ctrl Pts',(7.51676407774738,111.574999999564,10.3459381770588));
#300247=CARTESIAN_POINT('Ctrl Pts',(9.83957192047847,111.724999999563,7.14886745759505));
#300248=CARTESIAN_POINT('Ctrl Pts',(12.1623797632096,111.874999999563,3.95179673813132));
#300249=CARTESIAN_POINT('Ctrl Pts',(12.1623797632096,112.024999999562,-1.48946194470292E-15));
#300250=CARTESIAN_POINT('Ctrl Pts',(12.1623797632096,112.174999999561,-3.95179673813132));
#300251=CARTESIAN_POINT('Ctrl Pts',(9.83957192047847,112.324999999561,-7.14886745759505));
#300252=CARTESIAN_POINT('Ctrl Pts',(7.51676407774738,112.47499999956,-10.3459381770588));
#300253=CARTESIAN_POINT('Ctrl Pts',(3.75838203887365,112.62499999956,-11.5671105274568));
#300254=CARTESIAN_POINT('Ctrl Pts',(-7.82081509407745E-14,112.774999999559,
-12.7882828778549));
#300255=CARTESIAN_POINT('Ctrl Pts',(-3.75838203887381,112.924999999558,
-11.5671105274568));
#300256=CARTESIAN_POINT('Ctrl Pts',(-7.51676407774753,113.074999999558,
-10.3459381770588));
#300257=CARTESIAN_POINT('Ctrl Pts',(-9.83957192047863,113.224999999557,
-7.14886745759505));
#300258=CARTESIAN_POINT('Ctrl Pts',(-12.1623797632097,113.374999999557,
-3.95179673813132));
#300259=CARTESIAN_POINT('Ctrl Pts',(-12.1623797632097,113.524999999556,
2.97892388940585E-15));
#300260=CARTESIAN_POINT('Ctrl Pts',(-12.1623797632097,113.674999999555,
3.95179673813133));
#300261=CARTESIAN_POINT('Ctrl Pts',(-9.83957192047863,113.824999999555,
7.14886745759505));
#300262=CARTESIAN_POINT('Ctrl Pts',(-7.51676407774753,113.974999999554,
10.3459381770588));
#300263=CARTESIAN_POINT('Ctrl Pts',(-3.7583820388738,114.124999999554,11.5671105274568));
#300264=CARTESIAN_POINT('Ctrl Pts',(-7.59397796380142E-14,114.274999999553,
12.7882828778549));
#300265=CARTESIAN_POINT('Ctrl Pts',(3.75838203887365,114.424999999552,11.5671105274568));
#300266=CARTESIAN_POINT('Ctrl Pts',(7.51676407774738,114.574999999552,10.3459381770588));
#300267=CARTESIAN_POINT('Ctrl Pts',(9.83957192047847,114.724999999551,7.14886745759505));
#300268=CARTESIAN_POINT('Ctrl Pts',(12.1623797632096,114.874999999551,3.95179673813132));
#300269=CARTESIAN_POINT('Ctrl Pts',(12.1623797632096,115.02499999955,-1.48946194470292E-15));
#300270=CARTESIAN_POINT('Ctrl Pts',(12.1623797632096,115.174999999549,-3.95179673813132));
#300271=CARTESIAN_POINT('Ctrl Pts',(9.83957192047847,115.324999999549,-7.14886745759505));
#300272=CARTESIAN_POINT('Ctrl Pts',(7.51676407774738,115.474999999548,-10.3459381770588));
#300273=CARTESIAN_POINT('Ctrl Pts',(3.75838203887365,115.624999999548,-11.5671105274568));
#300274=CARTESIAN_POINT('Ctrl Pts',(-7.99358602124363E-14,115.774999999547,
-12.7882828778549));
#300275=CARTESIAN_POINT('Ctrl Pts',(-3.75838203887381,115.924999999546,
-11.5671105274568));
#300276=CARTESIAN_POINT('Ctrl Pts',(-7.51676407774754,116.074999999546,
-10.3459381770588));
#300277=CARTESIAN_POINT('Ctrl Pts',(-9.83957192047863,116.224999999545,
-7.14886745759505));
#300278=CARTESIAN_POINT('Ctrl Pts',(-12.1623797632097,116.374999999545,
-3.95179673813132));
#300279=CARTESIAN_POINT('Ctrl Pts',(-12.1623797632097,116.524999999544,
2.97892388940585E-15));
#300280=CARTESIAN_POINT('Ctrl Pts',(-12.1623797632097,116.674999999543,
3.95179673813133));
#300281=CARTESIAN_POINT('Ctrl Pts',(-9.83957192047863,116.824999999543,
7.14886745759505));
#300282=CARTESIAN_POINT('Ctrl Pts',(-7.51676407774753,116.974999999542,
10.3459381770588));
#300283=CARTESIAN_POINT('Ctrl Pts',(-3.75838203887381,117.124999999542,
11.5671105274568));
#300284=CARTESIAN_POINT('Ctrl Pts',(-7.76674889096761E-14,117.274999999541,
12.7882828778549));
#300285=CARTESIAN_POINT('Ctrl Pts',(3.75838203887365,117.42499999954,11.5671105274568));
#300286=CARTESIAN_POINT('Ctrl Pts',(7.51676407774738,117.57499999954,10.3459381770588));
#300287=CARTESIAN_POINT('Ctrl Pts',(9.83957192047847,117.724999999539,7.14886745759505));
#300288=CARTESIAN_POINT('Ctrl Pts',(12.1623797632096,117.874999999539,3.95179673813132));
#300289=CARTESIAN_POINT('Ctrl Pts',(12.1623797632096,118.024999999538,-1.48946194470292E-15));
#300290=CARTESIAN_POINT('Ctrl Pts',(12.1623797632096,118.174999999537,-3.95179673813132));
#300291=CARTESIAN_POINT('Ctrl Pts',(9.83957192047847,118.324999999537,-7.14886745759505));
#300292=CARTESIAN_POINT('Ctrl Pts',(7.51676407774737,118.474999999536,-10.3459381770588));
#300293=CARTESIAN_POINT('Ctrl Pts',(3.75838203887365,118.624999999536,-11.5671105274568));
#300294=CARTESIAN_POINT('Ctrl Pts',(-8.16635694840981E-14,118.774999999535,
-12.7882828778549));
#300295=CARTESIAN_POINT('Ctrl Pts',(-3.75838203887381,118.924999999534,
-11.5671105274568));
#300296=CARTESIAN_POINT('Ctrl Pts',(-7.51676407774754,119.074999999534,
-10.3459381770588));
#300297=CARTESIAN_POINT('Ctrl Pts',(-9.83957192047863,119.224999999533,
-7.14886745759505));
#300298=CARTESIAN_POINT('Ctrl Pts',(-12.1623797632097,119.374999999533,
-3.95179673813132));
#300299=CARTESIAN_POINT('Ctrl Pts',(-12.1623797632097,119.524999999532,
2.97892388940585E-15));
#300300=CARTESIAN_POINT('Ctrl Pts',(-12.1623797632097,119.674999999531,
3.95179673813133));
#300301=CARTESIAN_POINT('Ctrl Pts',(-9.83957192047863,119.824999999531,
7.14886745759505));
#300302=CARTESIAN_POINT('Ctrl Pts',(-7.51676407774754,119.97499999953,10.3459381770588));
#300303=CARTESIAN_POINT('Ctrl Pts',(-3.75838203887381,120.12499999953,11.5671105274568));
#300304=CARTESIAN_POINT('Ctrl Pts',(-7.93951981813379E-14,120.274999999529,
12.7882828778549));
#300305=CARTESIAN_POINT('Ctrl Pts',(3.75838203887365,120.424999999528,11.5671105274568));
#300306=CARTESIAN_POINT('Ctrl Pts',(7.51676407774738,120.574999999528,10.3459381770588));
#300307=CARTESIAN_POINT('Ctrl Pts',(9.83957192047847,120.724999999527,7.14886745759505));
#300308=CARTESIAN_POINT('Ctrl Pts',(12.1623797632096,120.874999999527,3.95179673813132));
#300309=CARTESIAN_POINT('Ctrl Pts',(12.1623797632096,121.024999999526,-1.48946194470292E-15));
#300310=CARTESIAN_POINT('Ctrl Pts',(12.1623797632096,121.174999999525,-3.95179673813132));
#300311=CARTESIAN_POINT('Ctrl Pts',(9.83957192047847,121.324999999525,-7.14886745759505));
#300312=CARTESIAN_POINT('Ctrl Pts',(7.51676407774737,121.474999999524,-10.3459381770588));
#300313=CARTESIAN_POINT('Ctrl Pts',(3.75838203887364,121.624999999524,-11.5671105274568));
#300314=CARTESIAN_POINT('Ctrl Pts',(-8.339127875576E-14,121.774999999523,
-12.7882828778549));
#300315=CARTESIAN_POINT('Ctrl Pts',(-3.75838203887381,121.924999999522,
-11.5671105274568));
#300316=CARTESIAN_POINT('Ctrl Pts',(-7.51676407774754,122.074999999522,
-10.3459381770588));
#300317=CARTESIAN_POINT('Ctrl Pts',(-9.83957192047863,122.224999999521,
-7.14886745759505));
#300318=CARTESIAN_POINT('Ctrl Pts',(-12.1623797632097,122.374999999521,
-3.95179673813132));
#300319=CARTESIAN_POINT('Ctrl Pts',(-12.1623797632097,122.52499999952,2.97892388940585E-15));
#300320=CARTESIAN_POINT('Ctrl Pts',(-12.1623797632097,122.674999999519,
3.95179673813133));
#300321=CARTESIAN_POINT('Ctrl Pts',(-9.83957192047863,122.824999999519,
7.14886745759505));
#300322=CARTESIAN_POINT('Ctrl Pts',(-7.51676407774754,122.974999999518,
10.3459381770588));
#300323=CARTESIAN_POINT('Ctrl Pts',(-3.75838203887381,123.124999999518,
11.5671105274568));
#300324=CARTESIAN_POINT('Ctrl Pts',(-8.11229074529997E-14,123.274999999517,
12.7882828778549));
#300325=CARTESIAN_POINT('Ctrl Pts',(3.75838203887365,123.424999999516,11.5671105274568));
#300326=CARTESIAN_POINT('Ctrl Pts',(7.51676407774737,123.574999999516,10.3459381770588));
#300327=CARTESIAN_POINT('Ctrl Pts',(9.83957192047846,123.724999999515,7.14886745759505));
#300328=CARTESIAN_POINT('Ctrl Pts',(12.1623797632096,123.874999999515,3.95179673813132));
#300329=CARTESIAN_POINT('Ctrl Pts',(12.1623797632096,124.024999999514,-1.48946194470292E-15));
#300330=CARTESIAN_POINT('Ctrl Pts',(12.1623797632096,124.174999999513,-3.95179673813132));
#300331=CARTESIAN_POINT('Ctrl Pts',(9.83957192047846,124.324999999513,-7.14886745759505));
#300332=CARTESIAN_POINT('Ctrl Pts',(7.51676407774737,124.474999999512,-10.3459381770588));
#300333=CARTESIAN_POINT('Ctrl Pts',(3.75838203887364,124.624999999512,-11.5671105274568));
#300334=CARTESIAN_POINT('Ctrl Pts',(-8.51189880274219E-14,124.774999999511,
-12.7882828778549));
#300335=CARTESIAN_POINT('Ctrl Pts',(-3.75838203887381,124.92499999951,-11.5671105274568));
#300336=CARTESIAN_POINT('Ctrl Pts',(-7.51676407774754,125.07499999951,-10.3459381770588));
#300337=CARTESIAN_POINT('Ctrl Pts',(-9.83957192047863,125.224999999509,
-7.14886745759505));
#300338=CARTESIAN_POINT('Ctrl Pts',(-12.1623797632097,125.374999999509,
-3.95179673813132));
#300339=CARTESIAN_POINT('Ctrl Pts',(-12.1623797632097,125.524999999508,
2.97892388940585E-15));
#300340=CARTESIAN_POINT('Ctrl Pts',(-12.1623797632097,125.674999999507,
3.95179673813133));
#300341=CARTESIAN_POINT('Ctrl Pts',(-9.83957192047863,125.824999999507,
7.14886745759505));
#300342=CARTESIAN_POINT('Ctrl Pts',(-7.51676407774754,125.974999999506,
10.3459381770588));
#300343=CARTESIAN_POINT('Ctrl Pts',(-3.75838203887381,126.124999999506,
11.5671105274568));
#300344=CARTESIAN_POINT('Ctrl Pts',(-8.28506167246616E-14,126.274999999505,
12.7882828778549));
#300345=CARTESIAN_POINT('Ctrl Pts',(3.75838203887364,126.424999999504,11.5671105274568));
#300346=CARTESIAN_POINT('Ctrl Pts',(7.51676407774737,126.574999999504,10.3459381770588));
#300347=CARTESIAN_POINT('Ctrl Pts',(9.83957192047846,126.724999999503,7.14886745759505));
#300348=CARTESIAN_POINT('Ctrl Pts',(12.1623797632096,126.874999999503,3.95179673813132));
#300349=CARTESIAN_POINT('Ctrl Pts',(12.1623797632096,127.024999999502,-1.48946194470292E-15));
#300350=CARTESIAN_POINT('Ctrl Pts',(12.1623797632096,127.174999999501,-3.95179673813132));
#300351=CARTESIAN_POINT('Ctrl Pts',(9.83957192047846,127.324999999501,-7.14886745759505));
#300352=CARTESIAN_POINT('Ctrl Pts',(7.51676407774737,127.4749999995,-10.3459381770588));
#300353=CARTESIAN_POINT('Ctrl Pts',(3.75838203887364,127.6249999995,-11.5671105274568));
#300354=CARTESIAN_POINT('Ctrl Pts',(-8.68466972990837E-14,127.774999999499,
-12.7882828778549));
#300355=CARTESIAN_POINT('Ctrl Pts',(-3.75838203887381,127.924999999498,
-11.5671105274568));
#300356=CARTESIAN_POINT('Ctrl Pts',(-7.51676407774754,128.074999999498,
-10.3459381770588));
#300357=CARTESIAN_POINT('Ctrl Pts',(-9.83957192047864,128.224999999497,
-7.14886745759505));
#300358=CARTESIAN_POINT('Ctrl Pts',(-12.1623797632097,128.374999999497,
-3.95179673813132));
#300359=CARTESIAN_POINT('Ctrl Pts',(-12.1623797632097,128.524999999496,
2.97892388940585E-15));
#300360=CARTESIAN_POINT('Ctrl Pts',(-12.1623797632097,128.674999999495,
3.95179673813133));
#300361=CARTESIAN_POINT('Ctrl Pts',(-9.83957192047864,128.824999999495,
7.14886745759505));
#300362=CARTESIAN_POINT('Ctrl Pts',(-7.51676407774754,128.974999999494,
10.3459381770588));
#300363=CARTESIAN_POINT('Ctrl Pts',(-3.75838203887381,129.124999999494,
11.5671105274568));
#300364=CARTESIAN_POINT('Ctrl Pts',(-8.45783259963234E-14,129.274999999493,
12.7882828778549));
#300365=CARTESIAN_POINT('Ctrl Pts',(3.75838203887364,129.424999999492,11.5671105274568));
#300366=CARTESIAN_POINT('Ctrl Pts',(7.51676407774737,129.574999999492,10.3459381770588));
#300367=CARTESIAN_POINT('Ctrl Pts',(9.83957192047846,129.724999999491,7.14886745759505));
#300368=CARTESIAN_POINT('Ctrl Pts',(12.1623797632096,129.874999999491,3.95179673813132));
#300369=CARTESIAN_POINT('Ctrl Pts',(12.1623797632096,130.02499999949,-1.48946194470292E-15));
#300370=CARTESIAN_POINT('Ctrl Pts',(12.1623797632096,130.174999999489,-3.95179673813132));
#300371=CARTESIAN_POINT('Ctrl Pts',(9.83957192047846,130.324999999489,-7.14886745759505));
#300372=CARTESIAN_POINT('Ctrl Pts',(7.51676407774737,130.474999999488,-10.3459381770588));
#300373=CARTESIAN_POINT('Ctrl Pts',(3.75838203887364,130.624999999488,-11.5671105274568));
#300374=CARTESIAN_POINT('Ctrl Pts',(-8.85744065707455E-14,130.774999999487,
-12.7882828778549));
#300375=CARTESIAN_POINT('Ctrl Pts',(-3.75838203887382,130.924999999486,
-11.5671105274568));
#300376=CARTESIAN_POINT('Ctrl Pts',(-7.51676407774754,131.074999999486,
-10.3459381770588));
#300377=CARTESIAN_POINT('Ctrl Pts',(-9.83957192047864,131.224999999485,
-7.14886745759505));
#300378=CARTESIAN_POINT('Ctrl Pts',(-12.1623797632097,131.374999999485,
-3.95179673813132));
#300379=CARTESIAN_POINT('Ctrl Pts',(-12.1623797632097,131.524999999484,
2.97892388940585E-15));
#300380=CARTESIAN_POINT('Ctrl Pts',(-12.1623797632097,131.674999999483,
3.95179673813133));
#300381=CARTESIAN_POINT('Ctrl Pts',(-9.83957192047864,131.824999999483,
7.14886745759505));
#300382=CARTESIAN_POINT('Ctrl Pts',(-7.51676407774754,131.974999999482,
10.3459381770588));
#300383=CARTESIAN_POINT('Ctrl Pts',(-3.75838203887381,132.124999999482,
11.5671105274568));
#300384=CARTESIAN_POINT('Ctrl Pts',(-8.63060352679853E-14,132.274999999481,
12.7882828778549));
#300385=CARTESIAN_POINT('Ctrl Pts',(3.75838203887364,132.42499999948,11.5671105274568));
#300386=CARTESIAN_POINT('Ctrl Pts',(7.51676407774737,132.57499999948,10.3459381770588));
#300387=CARTESIAN_POINT('Ctrl Pts',(9.83957192047846,132.724999999479,7.14886745759505));
#300388=CARTESIAN_POINT('Ctrl Pts',(12.1623797632096,132.874999999479,3.95179673813132));
#300389=CARTESIAN_POINT('Ctrl Pts',(12.1623797632096,133.024999999478,-1.48946194470292E-15));
#300390=CARTESIAN_POINT('Ctrl Pts',(12.1623797632096,133.174999999477,-3.95179673813132));
#300391=CARTESIAN_POINT('Ctrl Pts',(9.83957192047846,133.324999999477,-7.14886745759505));
#300392=CARTESIAN_POINT('Ctrl Pts',(7.51676407774736,133.474999999476,-10.3459381770588));
#300393=CARTESIAN_POINT('Ctrl Pts',(3.75838203887364,133.624999999476,-11.5671105274568));
#300394=CARTESIAN_POINT('Ctrl Pts',(-9.03021158424074E-14,133.774999999475,
-12.7882828778549));
#300395=CARTESIAN_POINT('Ctrl Pts',(-3.75838203887382,133.924999999474,
-11.5671105274568));
#300396=CARTESIAN_POINT('Ctrl Pts',(-7.51676407774755,134.074999999474,
-10.3459381770588));
#300397=CARTESIAN_POINT('Ctrl Pts',(-9.83957192047864,134.224999999473,
-7.14886745759505));
#300398=CARTESIAN_POINT('Ctrl Pts',(-12.1623797632097,134.374999999473,
-3.95179673813132));
#300399=CARTESIAN_POINT('Ctrl Pts',(-12.1623797632097,134.524999999472,
2.97892388940585E-15));
#300400=CARTESIAN_POINT('Ctrl Pts',(-12.1623797632097,134.674999999471,
3.95179673813133));
#300401=CARTESIAN_POINT('Ctrl Pts',(-9.83957192047864,134.824999999471,
7.14886745759505));
#300402=CARTESIAN_POINT('Ctrl Pts',(-7.51676407774754,134.97499999947,10.3459381770588));
#300403=CARTESIAN_POINT('Ctrl Pts',(-3.75838203887382,135.12499999947,11.5671105274568));
#300404=CARTESIAN_POINT('Ctrl Pts',(-8.80337445396471E-14,135.274999999469,
12.7882828778549));
#300405=CARTESIAN_POINT('Ctrl Pts',(3.75838203887364,135.424999999468,11.5671105274568));
#300406=CARTESIAN_POINT('Ctrl Pts',(7.51676407774737,135.574999999468,10.3459381770588));
#300407=CARTESIAN_POINT('Ctrl Pts',(9.83957192047846,135.724999999467,7.14886745759505));
#300408=CARTESIAN_POINT('Ctrl Pts',(12.1623797632096,135.874999999467,3.95179673813132));
#300409=CARTESIAN_POINT('Ctrl Pts',(12.1623797632096,136.024999999466,-1.48946194470292E-15));
#300410=CARTESIAN_POINT('Ctrl Pts',(12.1623797632095,136.174999999465,-3.95179673813132));
#300411=CARTESIAN_POINT('Ctrl Pts',(9.83957192047846,136.324999999465,-7.14886745759505));
#300412=CARTESIAN_POINT('Ctrl Pts',(7.51676407774736,136.474999999464,-10.3459381770588));
#300413=CARTESIAN_POINT('Ctrl Pts',(3.75838203887364,136.624999999464,-11.5671105274568));
#300414=CARTESIAN_POINT('Ctrl Pts',(-9.20298251140692E-14,136.774999999463,
-12.7882828778549));
#300415=CARTESIAN_POINT('Ctrl Pts',(-3.75838203887382,136.924999999462,
-11.5671105274568));
#300416=CARTESIAN_POINT('Ctrl Pts',(-7.51676407774755,137.074999999462,
-10.3459381770588));
#300417=CARTESIAN_POINT('Ctrl Pts',(-9.83957192047864,137.224999999461,
-7.14886745759505));
#300418=CARTESIAN_POINT('Ctrl Pts',(-12.1623797632097,137.374999999461,
-3.95179673813132));
#300419=CARTESIAN_POINT('Ctrl Pts',(-12.1623797632097,137.52499999946,2.97892388940585E-15));
#300420=CARTESIAN_POINT('Ctrl Pts',(-12.1623797632097,137.674999999459,
3.95179673813133));
#300421=CARTESIAN_POINT('Ctrl Pts',(-9.83957192047864,137.824999999459,
7.14886745759505));
#300422=CARTESIAN_POINT('Ctrl Pts',(-7.51676407774755,137.974999999458,
10.3459381770588));
#300423=CARTESIAN_POINT('Ctrl Pts',(-3.75838203887382,138.124999999458,
11.5671105274568));
#300424=CARTESIAN_POINT('Ctrl Pts',(-8.97614538113089E-14,138.274999999457,
12.7882828778549));
#300425=CARTESIAN_POINT('Ctrl Pts',(3.75838203887364,138.424999999456,11.5671105274568));
#300426=CARTESIAN_POINT('Ctrl Pts',(7.51676407774736,138.574999999456,10.3459381770588));
#300427=CARTESIAN_POINT('Ctrl Pts',(9.83957192047846,138.724999999455,7.14886745759505));
#300428=CARTESIAN_POINT('Ctrl Pts',(12.1623797632096,138.874999999455,3.95179673813132));
#300429=CARTESIAN_POINT('Ctrl Pts',(12.1623797632096,139.024999999454,-1.48946194470292E-15));
#300430=CARTESIAN_POINT('Ctrl Pts',(12.1623797632095,139.174999999453,-3.95179673813132));
#300431=CARTESIAN_POINT('Ctrl Pts',(9.83957192047846,139.324999999453,-7.14886745759505));
#300432=CARTESIAN_POINT('Ctrl Pts',(7.51676407774736,139.474999999452,-10.3459381770588));
#300433=CARTESIAN_POINT('Ctrl Pts',(3.75838203887363,139.624999999452,-11.5671105274568));
#300434=CARTESIAN_POINT('Ctrl Pts',(-9.3757534385731E-14,139.774999999451,
-12.7882828778549));
#300435=CARTESIAN_POINT('Ctrl Pts',(-3.75838203887382,139.92499999945,-11.5671105274568));
#300436=CARTESIAN_POINT('Ctrl Pts',(-7.51676407774755,140.07499999945,-10.3459381770588));
#300437=CARTESIAN_POINT('Ctrl Pts',(-9.83957192047864,140.224999999449,
-7.14886745759505));
#300438=CARTESIAN_POINT('Ctrl Pts',(-12.1623797632097,140.374999999449,
-3.95179673813132));
#300439=CARTESIAN_POINT('Ctrl Pts',(-12.1623797632097,140.524999999448,
2.97892388940585E-15));
#300440=CARTESIAN_POINT('Ctrl Pts',(-12.1623797632097,140.674999999447,
3.95179673813133));
#300441=CARTESIAN_POINT('Ctrl Pts',(-9.83957192047864,140.824999999447,
7.14886745759505));
#300442=CARTESIAN_POINT('Ctrl Pts',(-7.51676407774755,140.974999999446,
10.3459381770588));
#300443=CARTESIAN_POINT('Ctrl Pts',(-3.75838203887382,141.124999999446,
11.5671105274568));
#300444=CARTESIAN_POINT('Ctrl Pts',(-9.14891630829708E-14,141.274999999445,
12.7882828778549));
#300445=CARTESIAN_POINT('Ctrl Pts',(3.75838203887364,141.424999999444,11.5671105274568));
#300446=CARTESIAN_POINT('Ctrl Pts',(7.51676407774736,141.574999999444,10.3459381770588));
#300447=CARTESIAN_POINT('Ctrl Pts',(9.83957192047845,141.724999999443,7.14886745759505));
#300448=CARTESIAN_POINT('Ctrl Pts',(12.1623797632095,141.874999999443,3.95179673813132));
#300449=CARTESIAN_POINT('Ctrl Pts',(12.1623797632095,142.024999999442,-1.48946194470292E-15));
#300450=CARTESIAN_POINT('Ctrl Pts',(12.1623797632095,142.174999999441,-3.95179673813132));
#300451=CARTESIAN_POINT('Ctrl Pts',(9.83957192047845,142.324999999441,-7.14886745759505));
#300452=CARTESIAN_POINT('Ctrl Pts',(7.51676407774736,142.47499999944,-10.3459381770588));
#300453=CARTESIAN_POINT('Ctrl Pts',(3.75838203887363,142.62499999944,-11.5671105274568));
#300454=CARTESIAN_POINT('Ctrl Pts',(-9.54852436573929E-14,142.774999999439,
-12.7882828778549));
#300455=CARTESIAN_POINT('Ctrl Pts',(-3.75838203887382,142.924999999438,
-11.5671105274568));
#300456=CARTESIAN_POINT('Ctrl Pts',(-7.51676407774755,143.074999999438,
-10.3459381770588));
#300457=CARTESIAN_POINT('Ctrl Pts',(-9.83957192047864,143.224999999437,
-7.14886745759505));
#300458=CARTESIAN_POINT('Ctrl Pts',(-12.1623797632097,143.374999999437,
-3.95179673813132));
#300459=CARTESIAN_POINT('Ctrl Pts',(-12.1623797632097,143.524999999436,
2.97892388940585E-15));
#300460=CARTESIAN_POINT('Ctrl Pts',(-12.1623797632097,143.674999999435,
3.95179673813133));
#300461=CARTESIAN_POINT('Ctrl Pts',(-9.83957192047864,143.824999999435,
7.14886745759505));
#300462=CARTESIAN_POINT('Ctrl Pts',(-7.51676407774755,143.974999999434,
10.3459381770588));
#300463=CARTESIAN_POINT('Ctrl Pts',(-3.75838203887382,144.124999999434,
11.5671105274568));
#300464=CARTESIAN_POINT('Ctrl Pts',(-9.32168723546326E-14,144.274999999433,
12.7882828778549));
#300465=CARTESIAN_POINT('Ctrl Pts',(3.75838203887363,144.424999999432,11.5671105274568));
#300466=CARTESIAN_POINT('Ctrl Pts',(7.51676407774736,144.574999999432,10.3459381770588));
#300467=CARTESIAN_POINT('Ctrl Pts',(9.83957192047845,144.724999999431,7.14886745759505));
#300468=CARTESIAN_POINT('Ctrl Pts',(12.1623797632095,144.874999999431,3.95179673813132));
#300469=CARTESIAN_POINT('Ctrl Pts',(12.1623797632095,145.02499999943,-1.48946194470292E-15));
#300470=CARTESIAN_POINT('Ctrl Pts',(12.1623797632095,145.174999999429,-3.95179673813132));
#300471=CARTESIAN_POINT('Ctrl Pts',(9.83957192047845,145.324999999429,-7.14886745759505));
#300472=CARTESIAN_POINT('Ctrl Pts',(7.51676407774736,145.474999999428,-10.3459381770588));
#300473=CARTESIAN_POINT('Ctrl Pts',(3.75838203887363,145.624999999428,-11.5671105274568));
#300474=CARTESIAN_POINT('Ctrl Pts',(-9.72129529290547E-14,145.774999999427,
-12.7882828778549));
#300475=CARTESIAN_POINT('Ctrl Pts',(-3.75838203887382,145.924999999426,
-11.5671105274568));
#300476=CARTESIAN_POINT('Ctrl Pts',(-7.51676407774755,146.074999999426,
-10.3459381770588));
#300477=CARTESIAN_POINT('Ctrl Pts',(-9.83957192047865,146.224999999425,
-7.14886745759505));
#300478=CARTESIAN_POINT('Ctrl Pts',(-12.1623797632097,146.374999999425,
-3.95179673813132));
#300479=CARTESIAN_POINT('Ctrl Pts',(-12.1623797632097,146.524999999424,
2.97892388940585E-15));
#300480=CARTESIAN_POINT('Ctrl Pts',(-12.1623797632097,146.674999999423,
3.95179673813133));
#300481=CARTESIAN_POINT('Ctrl Pts',(-9.83957192047865,146.824999999423,
7.14886745759505));
#300482=CARTESIAN_POINT('Ctrl Pts',(-7.51676407774755,146.974999999422,
10.3459381770588));
#300483=CARTESIAN_POINT('Ctrl Pts',(-3.75838203887382,147.124999999422,
11.5671105274568));
#300484=CARTESIAN_POINT('Ctrl Pts',(-9.49445816262944E-14,147.274999999421,
12.7882828778549));
#300485=CARTESIAN_POINT('Ctrl Pts',(3.75838203887363,147.42499999942,11.5671105274568));
#300486=CARTESIAN_POINT('Ctrl Pts',(7.51676407774736,147.57499999942,10.3459381770588));
#300487=CARTESIAN_POINT('Ctrl Pts',(9.83957192047845,147.724999999419,7.14886745759505));
#300488=CARTESIAN_POINT('Ctrl Pts',(12.1623797632095,147.874999999419,3.95179673813132));
#300489=CARTESIAN_POINT('Ctrl Pts',(12.1623797632095,148.024999999418,-1.48946194470292E-15));
#300490=CARTESIAN_POINT('Ctrl Pts',(12.1623797632095,148.174999999417,-3.95179673813132));
#300491=CARTESIAN_POINT('Ctrl Pts',(9.83957192047845,148.324999999417,-7.14886745759505));
#300492=CARTESIAN_POINT('Ctrl Pts',(7.51676407774736,148.474999999416,-10.3459381770588));
#300493=CARTESIAN_POINT('Ctrl Pts',(3.75838203887363,148.624999999416,-11.5671105274568));
#300494=CARTESIAN_POINT('Ctrl Pts',(-9.89406622007166E-14,148.774999999415,
-12.7882828778549));
#300495=CARTESIAN_POINT('Ctrl Pts',(-3.75838203887383,148.924999999414,
-11.5671105274568));
#300496=CARTESIAN_POINT('Ctrl Pts',(-7.51676407774756,149.074999999414,
-10.3459381770588));
#300497=CARTESIAN_POINT('Ctrl Pts',(-9.83957192047865,149.224999999413,
-7.14886745759505));
#300498=CARTESIAN_POINT('Ctrl Pts',(-12.1623797632097,149.374999999413,
-3.95179673813132));
#300499=CARTESIAN_POINT('Ctrl Pts',(-12.1623797632097,149.524999999412,
2.97892388940585E-15));
#300500=CARTESIAN_POINT('Ctrl Pts',(-12.1623797632097,149.674999999411,
3.95179673813133));
#300501=CARTESIAN_POINT('Ctrl Pts',(-9.83957192047865,149.824999999411,
7.14886745759505));
#300502=CARTESIAN_POINT('Ctrl Pts',(-7.51676407774755,149.97499999941,10.3459381770588));
#300503=CARTESIAN_POINT('Ctrl Pts',(-3.75838203887382,150.12499999941,11.5671105274568));
#300504=CARTESIAN_POINT('Ctrl Pts',(-9.66722908979563E-14,150.274999999409,
12.7882828778549));
#300505=CARTESIAN_POINT('Ctrl Pts',(3.75838203887363,150.424999999408,11.5671105274568));
#300506=CARTESIAN_POINT('Ctrl Pts',(7.51676407774736,150.574999999408,10.3459381770588));
#300507=CARTESIAN_POINT('Ctrl Pts',(9.83957192047845,150.724999999407,7.14886745759505));
#300508=CARTESIAN_POINT('Ctrl Pts',(12.1623797632095,150.874999999407,3.95179673813132));
#300509=CARTESIAN_POINT('Ctrl Pts',(12.1623797632095,151.024999999406,-1.48946194470292E-15));
#300510=CARTESIAN_POINT('Ctrl Pts',(12.1623797632095,151.174999999405,-3.95179673813132));
#300511=CARTESIAN_POINT('Ctrl Pts',(9.83957192047845,151.324999999405,-7.14886745759505));
#300512=CARTESIAN_POINT('Ctrl Pts',(7.51676407774736,151.474999999404,-10.3459381770588));
#300513=CARTESIAN_POINT('Ctrl Pts',(3.75838203887363,151.624999999404,-11.5671105274568));
#300514=CARTESIAN_POINT('Ctrl Pts',(-1.00668371472378E-13,151.774999999403,
-12.7882828778549));
#300515=CARTESIAN_POINT('Ctrl Pts',(-3.75838203887383,151.924999999402,
-11.5671105274568));
#300516=CARTESIAN_POINT('Ctrl Pts',(-7.51676407774756,152.074999999402,
-10.3459381770588));
#300517=CARTESIAN_POINT('Ctrl Pts',(-9.83957192047865,152.224999999401,
-7.14886745759505));
#300518=CARTESIAN_POINT('Ctrl Pts',(-12.1623797632097,152.374999999401,
-3.95179673813132));
#300519=CARTESIAN_POINT('Ctrl Pts',(-12.1623797632097,152.5249999994,2.97892388940585E-15));
#300520=CARTESIAN_POINT('Ctrl Pts',(-12.1623797632097,152.674999999399,
3.95179673813133));
#300521=CARTESIAN_POINT('Ctrl Pts',(-9.83957192047865,152.824999999399,
7.14886745759505));
#300522=CARTESIAN_POINT('Ctrl Pts',(-7.51676407774756,152.974999999398,
10.3459381770588));
#300523=CARTESIAN_POINT('Ctrl Pts',(-3.75838203887383,153.124999999398,
11.5671105274568));
#300524=CARTESIAN_POINT('Ctrl Pts',(-9.84000001696181E-14,153.274999999397,
12.7882828778549));
#300525=CARTESIAN_POINT('Ctrl Pts',(3.75838203887363,153.424999999396,11.5671105274568));
#300526=CARTESIAN_POINT('Ctrl Pts',(7.51676407774736,153.574999999396,10.3459381770588));
#300527=CARTESIAN_POINT('Ctrl Pts',(9.83957192047845,153.724999999395,7.14886745759505));
#300528=CARTESIAN_POINT('Ctrl Pts',(12.1623797632095,153.874999999395,3.95179673813132));
#300529=CARTESIAN_POINT('Ctrl Pts',(12.1623797632095,154.024999999394,-1.48946194470292E-15));
#300530=CARTESIAN_POINT('Ctrl Pts',(12.1623797632095,154.174999999393,-3.95179673813132));
#300531=CARTESIAN_POINT('Ctrl Pts',(9.83957192047845,154.324999999393,-7.14886745759505));
#300532=CARTESIAN_POINT('Ctrl Pts',(7.51676407774735,154.474999999392,-10.3459381770588));
#300533=CARTESIAN_POINT('Ctrl Pts',(3.75838203887363,154.624999999392,-11.5671105274568));
#300534=CARTESIAN_POINT('Ctrl Pts',(-1.0239608074404E-13,154.774999999391,
-12.7882828778549));
#300535=CARTESIAN_POINT('Ctrl Pts',(-3.75838203887383,154.92499999939,-11.5671105274568));
#300536=CARTESIAN_POINT('Ctrl Pts',(10.0514428414941,59.8062499997713,-1.23094673026484E-15));
#300537=CARTESIAN_POINT('Ctrl Pts',(10.0514428414941,59.9562499997706,-3.26591175476071));
#300538=CARTESIAN_POINT('Ctrl Pts',(8.13178807675714,60.10624999977,-5.90808986649102));
#300539=CARTESIAN_POINT('Ctrl Pts',(7.55384587767069,60.1514098542684,-6.70355906039096));
#300540=CARTESIAN_POINT('Ctrl Pts',(6.83270577527258,60.1985571585059,-7.37194919844001));
#300541=CARTESIAN_POINT('Ctrl Pts',(-12.1623797632103,-3.28749999997638,
2.97892388940601E-15));
#300542=CARTESIAN_POINT('Ctrl Pts',(-12.1623797632103,-3.13749999997698,
3.95179673813154));
#300543=CARTESIAN_POINT('Ctrl Pts',(-9.83957192047908,-2.98749999997758,
7.14886745759543));
#300544=CARTESIAN_POINT('Ctrl Pts',(-7.51676407774787,-2.83749999997817,
10.3459381770593));
#300545=CARTESIAN_POINT('Ctrl Pts',(-3.75838203887394,-2.68749999997877,
11.5671105274575));
#300546=CARTESIAN_POINT('Ctrl Pts',(-8.66709987268145E-15,-2.53749999997937,
12.7882828778556));
#300547=CARTESIAN_POINT('Ctrl Pts',(3.75838203887392,-2.38749999997997,
11.5671105274575));
#300548=CARTESIAN_POINT('Ctrl Pts',(7.51676407774785,-2.23749999998057,
10.3459381770593));
#300549=CARTESIAN_POINT('Ctrl Pts',(9.83957192047906,-2.08749999998117,
7.14886745759543));
#300550=CARTESIAN_POINT('Ctrl Pts',(12.1623797632103,-1.93749999998176,
3.95179673813153));
#300551=CARTESIAN_POINT('Ctrl Pts',(12.1623797632103,-1.78749999998236,
-1.489461944703E-15));
#300552=CARTESIAN_POINT('Ctrl Pts',(12.1623797632103,-1.63749999998296,
-3.95179673813154));
#300553=CARTESIAN_POINT('Ctrl Pts',(9.83957192047906,-1.48749999998357,
-7.14886745759543));
#300554=CARTESIAN_POINT('Ctrl Pts',(7.51676407774784,-1.33749999998417,
-10.3459381770593));
#300555=CARTESIAN_POINT('Ctrl Pts',(3.75838203887392,-1.18749999998477,
-11.5671105274575));
#300556=CARTESIAN_POINT('Ctrl Pts',(-1.26631804471037E-14,-1.03749999998537,
-12.7882828778556));
#300557=CARTESIAN_POINT('Ctrl Pts',(-3.75838203887394,-0.887499999985973,
-11.5671105274575));
#300558=CARTESIAN_POINT('Ctrl Pts',(-7.51676407774787,-0.737499999986575,
-10.3459381770593));
#300559=CARTESIAN_POINT('Ctrl Pts',(-9.83957192047909,-0.587499999987176,
-7.14886745759543));
#300560=CARTESIAN_POINT('Ctrl Pts',(-12.1623797632103,-0.437499999987778,
-3.95179673813153));
#300561=CARTESIAN_POINT('Ctrl Pts',(-12.1623797632103,-0.287499999988378,
2.97892388940601E-15));
#300562=CARTESIAN_POINT('Ctrl Pts',(-12.1623797632103,-0.137499999988978,
3.95179673813154));
#300563=CARTESIAN_POINT('Ctrl Pts',(-9.83957192047909,0.0125000000104236,
7.14886745759543));
#300564=CARTESIAN_POINT('Ctrl Pts',(-7.51676407774787,0.162500000009825,
10.3459381770593));
#300565=CARTESIAN_POINT('Ctrl Pts',(-3.75838203887394,0.312500000009227,
11.5671105274575));
#300566=CARTESIAN_POINT('Ctrl Pts',(-1.03948091443433E-14,0.462500000008629,
12.7882828778556));
#300567=CARTESIAN_POINT('Ctrl Pts',(3.75838203887392,0.612500000008031,
11.5671105274575));
#300568=CARTESIAN_POINT('Ctrl Pts',(7.51676407774785,0.762500000007433,
10.3459381770593));
#300569=CARTESIAN_POINT('Ctrl Pts',(9.83957192047906,0.912500000006835,
7.14886745759543));
#300570=CARTESIAN_POINT('Ctrl Pts',(12.1623797632103,1.06250000000624,3.95179673813153));
#300571=CARTESIAN_POINT('Ctrl Pts',(12.1623797632103,1.21250000000564,-1.489461944703E-15));
#300572=CARTESIAN_POINT('Ctrl Pts',(12.1623797632103,1.36250000000504,-3.95179673813154));
#300573=CARTESIAN_POINT('Ctrl Pts',(9.83957192047906,1.51250000000444,-7.14886745759543));
#300574=CARTESIAN_POINT('Ctrl Pts',(7.51676407774784,1.66250000000383,-10.3459381770593));
#300575=CARTESIAN_POINT('Ctrl Pts',(3.75838203887391,1.81250000000323,-11.5671105274575));
#300576=CARTESIAN_POINT('Ctrl Pts',(-1.43908897187656E-14,1.96250000000263,
-12.7882828778556));
#300577=CARTESIAN_POINT('Ctrl Pts',(-3.75838203887394,2.11250000000203,
-11.5671105274575));
#300578=CARTESIAN_POINT('Ctrl Pts',(-7.51676407774787,2.26250000000143,
-10.3459381770593));
#300579=CARTESIAN_POINT('Ctrl Pts',(-9.83957192047909,2.41250000000082,
-7.14886745759543));
#300580=CARTESIAN_POINT('Ctrl Pts',(-12.1623797632103,2.56250000000022,
-3.95179673813153));
#300581=CARTESIAN_POINT('Ctrl Pts',(-12.1623797632103,2.71249999999962,
2.97892388940601E-15));
#300582=CARTESIAN_POINT('Ctrl Pts',(-12.1623797632103,2.86249999999902,
3.95179673813154));
#300583=CARTESIAN_POINT('Ctrl Pts',(-9.83957192047909,3.01249999999842,
7.14886745759543));
#300584=CARTESIAN_POINT('Ctrl Pts',(-7.51676407774787,3.16249999999782,
10.3459381770593));
#300585=CARTESIAN_POINT('Ctrl Pts',(-3.75838203887394,3.31249999999723,
11.5671105274575));
#300586=CARTESIAN_POINT('Ctrl Pts',(-1.21225184160051E-14,3.46249999999663,
12.7882828778556));
#300587=CARTESIAN_POINT('Ctrl Pts',(3.75838203887392,3.61249999999603,11.5671105274575));
#300588=CARTESIAN_POINT('Ctrl Pts',(7.51676407774784,3.76249999999543,10.3459381770593));
#300589=CARTESIAN_POINT('Ctrl Pts',(9.83957192047906,3.91249999999483,7.14886745759543));
#300590=CARTESIAN_POINT('Ctrl Pts',(12.1623797632103,4.06249999999424,3.95179673813153));
#300591=CARTESIAN_POINT('Ctrl Pts',(12.1623797632103,4.21249999999364,-1.489461944703E-15));
#300592=CARTESIAN_POINT('Ctrl Pts',(12.1623797632103,4.36249999999303,-3.95179673813154));
#300593=CARTESIAN_POINT('Ctrl Pts',(9.83957192047906,4.51249999999243,-7.14886745759543));
#300594=CARTESIAN_POINT('Ctrl Pts',(7.51676407774784,4.66249999999183,-10.3459381770593));
#300595=CARTESIAN_POINT('Ctrl Pts',(3.75838203887391,4.81249999999123,-11.5671105274575));
#300596=CARTESIAN_POINT('Ctrl Pts',(-1.61185989904274E-14,4.96249999999063,
-12.7882828778556));
#300597=CARTESIAN_POINT('Ctrl Pts',(-3.75838203887394,5.11249999999003,
-11.5671105274575));
#300598=CARTESIAN_POINT('Ctrl Pts',(-7.51676407774788,5.26249999998942,
-10.3459381770593));
#300599=CARTESIAN_POINT('Ctrl Pts',(-9.83957192047909,5.41249999998882,
-7.14886745759543));
#300600=CARTESIAN_POINT('Ctrl Pts',(-12.1623797632103,5.56249999998822,
-3.95179673813153));
#300601=CARTESIAN_POINT('Ctrl Pts',(-12.1623797632103,5.71249999998762,
2.97892388940601E-15));
#300602=CARTESIAN_POINT('Ctrl Pts',(-12.1623797632103,5.86249999998702,
3.95179673813154));
#300603=CARTESIAN_POINT('Ctrl Pts',(-9.83957192047909,6.01249999998642,
7.14886745759543));
#300604=CARTESIAN_POINT('Ctrl Pts',(-7.51676407774787,6.16249999998582,
10.3459381770593));
#300605=CARTESIAN_POINT('Ctrl Pts',(-3.75838203887394,6.31249999998523,
11.5671105274575));
#300606=CARTESIAN_POINT('Ctrl Pts',(-1.3850227687667E-14,6.46249999998463,
12.7882828778556));
#300607=CARTESIAN_POINT('Ctrl Pts',(3.75838203887392,6.61249999998403,11.5671105274575));
#300608=CARTESIAN_POINT('Ctrl Pts',(7.51676407774784,6.76249999998343,10.3459381770593));
#300609=CARTESIAN_POINT('Ctrl Pts',(9.83957192047906,6.91249999998283,7.14886745759543));
#300610=CARTESIAN_POINT('Ctrl Pts',(12.1623797632103,7.06249999998224,3.95179673813153));
#300611=CARTESIAN_POINT('Ctrl Pts',(12.1623797632103,7.21249999998164,-1.489461944703E-15));
#300612=CARTESIAN_POINT('Ctrl Pts',(12.1623797632103,7.36249999998104,-3.95179673813154));
#300613=CARTESIAN_POINT('Ctrl Pts',(9.83957192047906,7.51249999998044,-7.14886745759543));
#300614=CARTESIAN_POINT('Ctrl Pts',(7.51676407774784,7.66249999997983,-10.3459381770593));
#300615=CARTESIAN_POINT('Ctrl Pts',(3.75838203887391,7.81249999997923,-11.5671105274575));
#300616=CARTESIAN_POINT('Ctrl Pts',(-1.78463082620892E-14,7.96249999997863,
-12.7882828778556));
#300617=CARTESIAN_POINT('Ctrl Pts',(-3.75838203887395,8.11249999997803,
-11.5671105274575));
#300618=CARTESIAN_POINT('Ctrl Pts',(-7.51676407774788,8.26249999997743,
-10.3459381770593));
#300619=CARTESIAN_POINT('Ctrl Pts',(-9.83957192047909,8.41249999997682,
-7.14886745759543));
#300620=CARTESIAN_POINT('Ctrl Pts',(-12.1623797632103,8.56249999997622,
-3.95179673813153));
#300621=CARTESIAN_POINT('Ctrl Pts',(-12.1623797632103,8.71249999997562,
2.97892388940601E-15));
#300622=CARTESIAN_POINT('Ctrl Pts',(-12.1623797632103,8.86249999997502,
3.95179673813154));
#300623=CARTESIAN_POINT('Ctrl Pts',(-9.83957192047909,9.01249999997442,
7.14886745759543));
#300624=CARTESIAN_POINT('Ctrl Pts',(-7.51676407774787,9.16249999997382,
10.3459381770593));
#300625=CARTESIAN_POINT('Ctrl Pts',(-3.75838203887394,9.31249999997323,
11.5671105274575));
#300626=CARTESIAN_POINT('Ctrl Pts',(-1.55779369593288E-14,9.46249999997263,
12.7882828778556));
#300627=CARTESIAN_POINT('Ctrl Pts',(3.75838203887391,9.61249999997203,11.5671105274575));
#300628=CARTESIAN_POINT('Ctrl Pts',(7.51676407774784,9.76249999997144,10.3459381770593));
#300629=CARTESIAN_POINT('Ctrl Pts',(9.83957192047906,9.91249999997084,7.14886745759543));
#300630=CARTESIAN_POINT('Ctrl Pts',(12.1623797632103,10.0624999999702,3.95179673813153));
#300631=CARTESIAN_POINT('Ctrl Pts',(12.1623797632103,10.2124999999696,-1.489461944703E-15));
#300632=CARTESIAN_POINT('Ctrl Pts',(12.1623797632103,10.362499999969,-3.95179673813154));
#300633=CARTESIAN_POINT('Ctrl Pts',(9.83957192047905,10.5124999999684,-7.14886745759543));
#300634=CARTESIAN_POINT('Ctrl Pts',(7.51676407774784,10.6624999999678,-10.3459381770593));
#300635=CARTESIAN_POINT('Ctrl Pts',(3.75838203887391,10.8124999999672,-11.5671105274575));
#300636=CARTESIAN_POINT('Ctrl Pts',(-1.95740175337511E-14,10.9624999999666,
-12.7882828778556));
#300637=CARTESIAN_POINT('Ctrl Pts',(-3.75838203887395,11.112499999966,-11.5671105274575));
#300638=CARTESIAN_POINT('Ctrl Pts',(-7.51676407774788,11.2624999999654,
-10.3459381770593));
#300639=CARTESIAN_POINT('Ctrl Pts',(-9.83957192047909,11.4124999999648,
-7.14886745759543));
#300640=CARTESIAN_POINT('Ctrl Pts',(-12.1623797632103,11.5624999999642,
-3.95179673813153));
#300641=CARTESIAN_POINT('Ctrl Pts',(-12.1623797632103,11.7124999999636,
2.97892388940601E-15));
#300642=CARTESIAN_POINT('Ctrl Pts',(-12.1623797632103,11.862499999963,3.95179673813154));
#300643=CARTESIAN_POINT('Ctrl Pts',(-9.83957192047909,12.0124999999624,
7.14886745759543));
#300644=CARTESIAN_POINT('Ctrl Pts',(-7.51676407774788,12.1624999999618,
10.3459381770593));
#300645=CARTESIAN_POINT('Ctrl Pts',(-3.75838203887395,12.3124999999612,
11.5671105274575));
#300646=CARTESIAN_POINT('Ctrl Pts',(-1.73056462309906E-14,12.4624999999606,
12.7882828778556));
#300647=CARTESIAN_POINT('Ctrl Pts',(3.75838203887391,12.61249999996,11.5671105274575));
#300648=CARTESIAN_POINT('Ctrl Pts',(7.51676407774784,12.7624999999594,10.3459381770593));
#300649=CARTESIAN_POINT('Ctrl Pts',(9.83957192047906,12.9124999999588,7.14886745759543));
#300650=CARTESIAN_POINT('Ctrl Pts',(12.1623797632103,13.0624999999582,3.95179673813153));
#300651=CARTESIAN_POINT('Ctrl Pts',(12.1623797632103,13.2124999999576,-1.489461944703E-15));
#300652=CARTESIAN_POINT('Ctrl Pts',(12.1623797632103,13.362499999957,-3.95179673813154));
#300653=CARTESIAN_POINT('Ctrl Pts',(9.83957192047905,13.5124999999564,-7.14886745759543));
#300654=CARTESIAN_POINT('Ctrl Pts',(7.51676407774784,13.6624999999558,-10.3459381770593));
#300655=CARTESIAN_POINT('Ctrl Pts',(3.75838203887391,13.8124999999552,-11.5671105274575));
#300656=CARTESIAN_POINT('Ctrl Pts',(-2.13017268054129E-14,13.9624999999546,
-12.7882828778556));
#300657=CARTESIAN_POINT('Ctrl Pts',(-3.75838203887395,14.112499999954,-11.5671105274575));
#300658=CARTESIAN_POINT('Ctrl Pts',(-7.51676407774788,14.2624999999534,
-10.3459381770593));
#300659=CARTESIAN_POINT('Ctrl Pts',(-9.8395719204791,14.4124999999528,-7.14886745759543));
#300660=CARTESIAN_POINT('Ctrl Pts',(-12.1623797632103,14.5624999999522,
-3.95179673813153));
#300661=CARTESIAN_POINT('Ctrl Pts',(-12.1623797632103,14.7124999999516,
2.97892388940601E-15));
#300662=CARTESIAN_POINT('Ctrl Pts',(-12.1623797632103,14.862499999951,3.95179673813154));
#300663=CARTESIAN_POINT('Ctrl Pts',(-9.83957192047909,15.0124999999504,
7.14886745759543));
#300664=CARTESIAN_POINT('Ctrl Pts',(-7.51676407774788,15.1624999999498,
10.3459381770593));
#300665=CARTESIAN_POINT('Ctrl Pts',(-3.75838203887395,15.3124999999492,
11.5671105274575));
#300666=CARTESIAN_POINT('Ctrl Pts',(-1.90333555026525E-14,15.4624999999486,
12.7882828778556));
#300667=CARTESIAN_POINT('Ctrl Pts',(3.75838203887391,15.612499999948,11.5671105274575));
#300668=CARTESIAN_POINT('Ctrl Pts',(7.51676407774784,15.7624999999474,10.3459381770593));
#300669=CARTESIAN_POINT('Ctrl Pts',(9.83957192047905,15.9124999999468,7.14886745759543));
#300670=CARTESIAN_POINT('Ctrl Pts',(12.1623797632103,16.0624999999462,3.95179673813153));
#300671=CARTESIAN_POINT('Ctrl Pts',(12.1623797632103,16.2124999999456,-1.489461944703E-15));
#300672=CARTESIAN_POINT('Ctrl Pts',(12.1623797632103,16.362499999945,-3.95179673813154));
#300673=CARTESIAN_POINT('Ctrl Pts',(9.83957192047905,16.5124999999444,-7.14886745759543));
#300674=CARTESIAN_POINT('Ctrl Pts',(7.51676407774784,16.6624999999438,-10.3459381770593));
#300675=CARTESIAN_POINT('Ctrl Pts',(3.75838203887391,16.8124999999432,-11.5671105274575));
#300676=CARTESIAN_POINT('Ctrl Pts',(-2.30294360770748E-14,16.9624999999426,
-12.7882828778556));
#300677=CARTESIAN_POINT('Ctrl Pts',(-3.75838203887395,17.112499999942,-11.5671105274575));
#300678=CARTESIAN_POINT('Ctrl Pts',(-7.51676407774788,17.2624999999414,
-10.3459381770593));
#300679=CARTESIAN_POINT('Ctrl Pts',(-9.8395719204791,17.4124999999408,-7.14886745759543));
#300680=CARTESIAN_POINT('Ctrl Pts',(-12.1623797632103,17.5624999999402,
-3.95179673813153));
#300681=CARTESIAN_POINT('Ctrl Pts',(-12.1623797632103,17.7124999999396,
2.97892388940601E-15));
#300682=CARTESIAN_POINT('Ctrl Pts',(-12.1623797632103,17.862499999939,3.95179673813154));
#300683=CARTESIAN_POINT('Ctrl Pts',(-9.8395719204791,18.0124999999384,7.14886745759543));
#300684=CARTESIAN_POINT('Ctrl Pts',(-7.51676407774788,18.1624999999378,
10.3459381770593));
#300685=CARTESIAN_POINT('Ctrl Pts',(-3.75838203887395,18.3124999999372,
11.5671105274575));
#300686=CARTESIAN_POINT('Ctrl Pts',(-2.07610647743143E-14,18.4624999999366,
12.7882828778556));
#300687=CARTESIAN_POINT('Ctrl Pts',(3.75838203887391,18.612499999936,11.5671105274575));
#300688=CARTESIAN_POINT('Ctrl Pts',(7.51676407774784,18.7624999999354,10.3459381770593));
#300689=CARTESIAN_POINT('Ctrl Pts',(9.83957192047905,18.9124999999348,7.14886745759543));
#300690=CARTESIAN_POINT('Ctrl Pts',(12.1623797632103,19.0624999999342,3.95179673813153));
#300691=CARTESIAN_POINT('Ctrl Pts',(12.1623797632103,19.2124999999336,-1.489461944703E-15));
#300692=CARTESIAN_POINT('Ctrl Pts',(12.1623797632103,19.362499999933,-3.95179673813154));
#300693=CARTESIAN_POINT('Ctrl Pts',(9.83957192047905,19.5124999999324,-7.14886745759543));
#300694=CARTESIAN_POINT('Ctrl Pts',(7.51676407774784,19.6624999999318,-10.3459381770593));
#300695=CARTESIAN_POINT('Ctrl Pts',(3.7583820388739,19.8124999999312,-11.5671105274575));
#300696=CARTESIAN_POINT('Ctrl Pts',(-2.47571453487366E-14,19.9624999999306,
-12.7882828778556));
#300697=CARTESIAN_POINT('Ctrl Pts',(-3.75838203887395,20.11249999993,-11.5671105274575));
#300698=CARTESIAN_POINT('Ctrl Pts',(-7.51676407774788,20.2624999999294,
-10.3459381770593));
#300699=CARTESIAN_POINT('Ctrl Pts',(-9.8395719204791,20.4124999999288,-7.14886745759543));
#300700=CARTESIAN_POINT('Ctrl Pts',(-12.1623797632103,20.5624999999282,
-3.95179673813153));
#300701=CARTESIAN_POINT('Ctrl Pts',(-12.1623797632103,20.7124999999276,
2.97892388940601E-15));
#300702=CARTESIAN_POINT('Ctrl Pts',(-12.1623797632103,20.862499999927,3.95179673813154));
#300703=CARTESIAN_POINT('Ctrl Pts',(-9.8395719204791,21.0124999999264,7.14886745759543));
#300704=CARTESIAN_POINT('Ctrl Pts',(-7.51676407774788,21.1624999999258,
10.3459381770593));
#300705=CARTESIAN_POINT('Ctrl Pts',(-3.75838203887395,21.3124999999252,
11.5671105274575));
#300706=CARTESIAN_POINT('Ctrl Pts',(-2.24887740459762E-14,21.4624999999246,
12.7882828778556));
#300707=CARTESIAN_POINT('Ctrl Pts',(3.75838203887391,21.612499999924,11.5671105274575));
#300708=CARTESIAN_POINT('Ctrl Pts',(7.51676407774784,21.7624999999234,10.3459381770593));
#300709=CARTESIAN_POINT('Ctrl Pts',(9.83957192047905,21.9124999999228,7.14886745759543));
#300710=CARTESIAN_POINT('Ctrl Pts',(12.1623797632103,22.0624999999222,3.95179673813153));
#300711=CARTESIAN_POINT('Ctrl Pts',(12.1623797632103,22.2124999999216,-1.489461944703E-15));
#300712=CARTESIAN_POINT('Ctrl Pts',(12.1623797632103,22.362499999921,-3.95179673813154));
#300713=CARTESIAN_POINT('Ctrl Pts',(9.83957192047905,22.5124999999204,-7.14886745759543));
#300714=CARTESIAN_POINT('Ctrl Pts',(7.51676407774783,22.6624999999198,-10.3459381770593));
#300715=CARTESIAN_POINT('Ctrl Pts',(3.7583820388739,22.8124999999192,-11.5671105274575));
#300716=CARTESIAN_POINT('Ctrl Pts',(-2.64848546203984E-14,22.9624999999186,
-12.7882828778556));
#300717=CARTESIAN_POINT('Ctrl Pts',(-3.75838203887396,23.112499999918,-11.5671105274575));
#300718=CARTESIAN_POINT('Ctrl Pts',(-7.51676407774788,23.2624999999174,
-10.3459381770593));
#300719=CARTESIAN_POINT('Ctrl Pts',(-9.8395719204791,23.4124999999168,-7.14886745759543));
#300720=CARTESIAN_POINT('Ctrl Pts',(-12.1623797632103,23.5624999999162,
-3.95179673813153));
#300721=CARTESIAN_POINT('Ctrl Pts',(-12.1623797632103,23.7124999999156,
2.97892388940601E-15));
#300722=CARTESIAN_POINT('Ctrl Pts',(-12.1623797632103,23.862499999915,3.95179673813154));
#300723=CARTESIAN_POINT('Ctrl Pts',(-9.8395719204791,24.0124999999144,7.14886745759543));
#300724=CARTESIAN_POINT('Ctrl Pts',(-7.51676407774788,24.1624999999138,
10.3459381770593));
#300725=CARTESIAN_POINT('Ctrl Pts',(-3.75838203887395,24.3124999999132,
11.5671105274575));
#300726=CARTESIAN_POINT('Ctrl Pts',(-2.4216483317638E-14,24.4624999999126,
12.7882828778556));
#300727=CARTESIAN_POINT('Ctrl Pts',(3.7583820388739,24.612499999912,11.5671105274575));
#300728=CARTESIAN_POINT('Ctrl Pts',(7.51676407774783,24.7624999999114,10.3459381770593));
#300729=CARTESIAN_POINT('Ctrl Pts',(9.83957192047905,24.9124999999108,7.14886745759543));
#300730=CARTESIAN_POINT('Ctrl Pts',(12.1623797632103,25.0624999999102,3.95179673813153));
#300731=CARTESIAN_POINT('Ctrl Pts',(12.1623797632103,25.2124999999096,-1.489461944703E-15));
#300732=CARTESIAN_POINT('Ctrl Pts',(12.1623797632103,25.362499999909,-3.95179673813154));
#300733=CARTESIAN_POINT('Ctrl Pts',(9.83957192047905,25.5124999999084,-7.14886745759543));
#300734=CARTESIAN_POINT('Ctrl Pts',(7.51676407774783,25.6624999999078,-10.3459381770593));
#300735=CARTESIAN_POINT('Ctrl Pts',(3.7583820388739,25.8124999999072,-11.5671105274575));
#300736=CARTESIAN_POINT('Ctrl Pts',(-2.82125638920603E-14,25.9624999999066,
-12.7882828778556));
#300737=CARTESIAN_POINT('Ctrl Pts',(-3.75838203887396,26.112499999906,-11.5671105274575));
#300738=CARTESIAN_POINT('Ctrl Pts',(-7.51676407774788,26.2624999999054,
-10.3459381770593));
#300739=CARTESIAN_POINT('Ctrl Pts',(-9.8395719204791,26.4124999999048,-7.14886745759543));
#300740=CARTESIAN_POINT('Ctrl Pts',(-12.1623797632103,26.5624999999042,
-3.95179673813153));
#300741=CARTESIAN_POINT('Ctrl Pts',(-12.1623797632103,26.7124999999036,
2.97892388940601E-15));
#300742=CARTESIAN_POINT('Ctrl Pts',(-12.1623797632103,26.862499999903,3.95179673813154));
#300743=CARTESIAN_POINT('Ctrl Pts',(-9.8395719204791,27.0124999999024,7.14886745759543));
#300744=CARTESIAN_POINT('Ctrl Pts',(-7.51676407774788,27.1624999999018,
10.3459381770593));
#300745=CARTESIAN_POINT('Ctrl Pts',(-3.75838203887396,27.3124999999012,
11.5671105274575));
#300746=CARTESIAN_POINT('Ctrl Pts',(-2.59441925892998E-14,27.4624999999006,
12.7882828778556));
#300747=CARTESIAN_POINT('Ctrl Pts',(3.7583820388739,27.6124999999,11.5671105274575));
#300748=CARTESIAN_POINT('Ctrl Pts',(7.51676407774783,27.7624999998994,10.3459381770593));
#300749=CARTESIAN_POINT('Ctrl Pts',(9.83957192047905,27.9124999998988,7.14886745759543));
#300750=CARTESIAN_POINT('Ctrl Pts',(12.1623797632103,28.0624999998982,3.95179673813153));
#300751=CARTESIAN_POINT('Ctrl Pts',(12.1623797632103,28.2124999998976,-1.489461944703E-15));
#300752=CARTESIAN_POINT('Ctrl Pts',(12.1623797632103,28.362499999897,-3.95179673813154));
#300753=CARTESIAN_POINT('Ctrl Pts',(9.83957192047905,28.5124999998964,-7.14886745759543));
#300754=CARTESIAN_POINT('Ctrl Pts',(7.51676407774783,28.6624999998958,-10.3459381770593));
#300755=CARTESIAN_POINT('Ctrl Pts',(3.7583820388739,28.8124999998952,-11.5671105274575));
#300756=CARTESIAN_POINT('Ctrl Pts',(-2.99402731637221E-14,28.9624999998946,
-12.7882828778556));
#300757=CARTESIAN_POINT('Ctrl Pts',(-3.75838203887396,29.112499999894,-11.5671105274575));
#300758=CARTESIAN_POINT('Ctrl Pts',(-7.51676407774789,29.2624999998934,
-10.3459381770593));
#300759=CARTESIAN_POINT('Ctrl Pts',(-9.8395719204791,29.4124999998928,-7.14886745759543));
#300760=CARTESIAN_POINT('Ctrl Pts',(-12.1623797632103,29.5624999998922,
-3.95179673813153));
#300761=CARTESIAN_POINT('Ctrl Pts',(-12.1623797632103,29.7124999998916,
2.97892388940601E-15));
#300762=CARTESIAN_POINT('Ctrl Pts',(-12.1623797632103,29.862499999891,3.95179673813154));
#300763=CARTESIAN_POINT('Ctrl Pts',(-9.8395719204791,30.0124999998904,7.14886745759543));
#300764=CARTESIAN_POINT('Ctrl Pts',(-7.51676407774788,30.1624999998898,
10.3459381770593));
#300765=CARTESIAN_POINT('Ctrl Pts',(-3.75838203887396,30.3124999998892,
11.5671105274575));
#300766=CARTESIAN_POINT('Ctrl Pts',(-2.76719018609617E-14,30.4624999998886,
12.7882828778556));
#300767=CARTESIAN_POINT('Ctrl Pts',(3.7583820388739,30.612499999888,11.5671105274575));
#300768=CARTESIAN_POINT('Ctrl Pts',(7.51676407774783,30.7624999998874,10.3459381770593));
#300769=CARTESIAN_POINT('Ctrl Pts',(9.83957192047905,30.9124999998868,7.14886745759543));
#300770=CARTESIAN_POINT('Ctrl Pts',(12.1623797632103,31.0624999998862,3.95179673813153));
#300771=CARTESIAN_POINT('Ctrl Pts',(12.1623797632103,31.2124999998856,-1.489461944703E-15));
#300772=CARTESIAN_POINT('Ctrl Pts',(12.1623797632103,31.362499999885,-3.95179673813154));
#300773=CARTESIAN_POINT('Ctrl Pts',(9.83957192047904,31.5124999998844,-7.14886745759543));
#300774=CARTESIAN_POINT('Ctrl Pts',(7.51676407774783,31.6624999998838,-10.3459381770593));
#300775=CARTESIAN_POINT('Ctrl Pts',(3.7583820388739,31.8124999998832,-11.5671105274575));
#300776=CARTESIAN_POINT('Ctrl Pts',(-3.16679824353839E-14,31.9624999998826,
-12.7882828778556));
#300777=CARTESIAN_POINT('Ctrl Pts',(-3.75838203887396,32.112499999882,-11.5671105274575));
#300778=CARTESIAN_POINT('Ctrl Pts',(-7.51676407774789,32.2624999998814,
-10.3459381770593));
#300779=CARTESIAN_POINT('Ctrl Pts',(-9.83957192047911,32.4124999998808,
-7.14886745759543));
#300780=CARTESIAN_POINT('Ctrl Pts',(-12.1623797632103,32.5624999998802,
-3.95179673813153));
#300781=CARTESIAN_POINT('Ctrl Pts',(-12.1623797632103,32.7124999998796,
2.97892388940601E-15));
#300782=CARTESIAN_POINT('Ctrl Pts',(-12.1623797632103,32.862499999879,3.95179673813154));
#300783=CARTESIAN_POINT('Ctrl Pts',(-9.8395719204791,33.0124999998784,7.14886745759543));
#300784=CARTESIAN_POINT('Ctrl Pts',(-7.51676407774789,33.1624999998778,
10.3459381770593));
#300785=CARTESIAN_POINT('Ctrl Pts',(-3.75838203887396,33.3124999998772,
11.5671105274575));
#300786=CARTESIAN_POINT('Ctrl Pts',(-2.93996111326235E-14,33.4624999998766,
12.7882828778556));
#300787=CARTESIAN_POINT('Ctrl Pts',(3.7583820388739,33.612499999876,11.5671105274575));
#300788=CARTESIAN_POINT('Ctrl Pts',(7.51676407774783,33.7624999998754,10.3459381770593));
#300789=CARTESIAN_POINT('Ctrl Pts',(9.83957192047905,33.9124999998748,7.14886745759543));
#300790=CARTESIAN_POINT('Ctrl Pts',(12.1623797632103,34.0624999998742,3.95179673813153));
#300791=CARTESIAN_POINT('Ctrl Pts',(12.1623797632103,34.2124999998736,-1.489461944703E-15));
#300792=CARTESIAN_POINT('Ctrl Pts',(12.1623797632103,34.362499999873,-3.95179673813154));
#300793=CARTESIAN_POINT('Ctrl Pts',(9.83957192047904,34.5124999998724,-7.14886745759543));
#300794=CARTESIAN_POINT('Ctrl Pts',(7.51676407774783,34.6624999998718,-10.3459381770593));
#300795=CARTESIAN_POINT('Ctrl Pts',(3.7583820388739,34.8124999998712,-11.5671105274575));
#300796=CARTESIAN_POINT('Ctrl Pts',(-3.33956917070458E-14,34.9624999998706,
-12.7882828778556));
#300797=CARTESIAN_POINT('Ctrl Pts',(-3.75838203887396,35.11249999987,-11.5671105274575));
#300798=CARTESIAN_POINT('Ctrl Pts',(-7.51676407774789,35.2624999998694,
-10.3459381770593));
#300799=CARTESIAN_POINT('Ctrl Pts',(-9.83957192047911,35.4124999998688,
-7.14886745759543));
#300800=CARTESIAN_POINT('Ctrl Pts',(-12.1623797632103,35.5624999998682,
-3.95179673813153));
#300801=CARTESIAN_POINT('Ctrl Pts',(-12.1623797632103,35.7124999998676,
2.97892388940601E-15));
#300802=CARTESIAN_POINT('Ctrl Pts',(-12.1623797632103,35.862499999867,3.95179673813154));
#300803=CARTESIAN_POINT('Ctrl Pts',(-9.83957192047911,36.0124999998664,
7.14886745759543));
#300804=CARTESIAN_POINT('Ctrl Pts',(-7.51676407774789,36.1624999998658,
10.3459381770593));
#300805=CARTESIAN_POINT('Ctrl Pts',(-3.75838203887396,36.3124999998652,
11.5671105274575));
#300806=CARTESIAN_POINT('Ctrl Pts',(-3.11273204042854E-14,36.4624999998646,
12.7882828778556));
#300807=CARTESIAN_POINT('Ctrl Pts',(3.7583820388739,36.612499999864,11.5671105274575));
#300808=CARTESIAN_POINT('Ctrl Pts',(7.51676407774783,36.7624999998634,10.3459381770593));
#300809=CARTESIAN_POINT('Ctrl Pts',(9.83957192047904,36.9124999998628,7.14886745759543));
#300810=CARTESIAN_POINT('Ctrl Pts',(12.1623797632103,37.0624999998622,3.95179673813153));
#300811=CARTESIAN_POINT('Ctrl Pts',(12.1623797632103,37.2124999998616,-1.489461944703E-15));
#300812=CARTESIAN_POINT('Ctrl Pts',(12.1623797632103,37.362499999861,-3.95179673813154));
#300813=CARTESIAN_POINT('Ctrl Pts',(9.83957192047904,37.5124999998604,-7.14886745759543));
#300814=CARTESIAN_POINT('Ctrl Pts',(7.51676407774782,37.6624999998598,-10.3459381770593));
#300815=CARTESIAN_POINT('Ctrl Pts',(3.75838203887389,37.8124999998592,-11.5671105274575));
#300816=CARTESIAN_POINT('Ctrl Pts',(-3.51234009787076E-14,37.9624999998586,
-12.7882828778556));
#300817=CARTESIAN_POINT('Ctrl Pts',(-3.75838203887396,38.112499999858,-11.5671105274575));
#300818=CARTESIAN_POINT('Ctrl Pts',(-7.51676407774789,38.2624999998574,
-10.3459381770593));
#300819=CARTESIAN_POINT('Ctrl Pts',(-9.83957192047911,38.4124999998568,
-7.14886745759543));
#300820=CARTESIAN_POINT('Ctrl Pts',(-12.1623797632103,38.5624999998562,
-3.95179673813153));
#300821=CARTESIAN_POINT('Ctrl Pts',(-12.1623797632103,38.7124999998556,
2.97892388940601E-15));
#300822=CARTESIAN_POINT('Ctrl Pts',(-12.1623797632103,38.862499999855,3.95179673813154));
#300823=CARTESIAN_POINT('Ctrl Pts',(-9.83957192047911,39.0124999998544,
7.14886745759543));
#300824=CARTESIAN_POINT('Ctrl Pts',(-7.51676407774789,39.1624999998538,
10.3459381770593));
#300825=CARTESIAN_POINT('Ctrl Pts',(-3.75838203887396,39.3124999998532,
11.5671105274575));
#300826=CARTESIAN_POINT('Ctrl Pts',(-3.28550296759472E-14,39.4624999998526,
12.7882828778556));
#300827=CARTESIAN_POINT('Ctrl Pts',(3.7583820388739,39.612499999852,11.5671105274575));
#300828=CARTESIAN_POINT('Ctrl Pts',(7.51676407774782,39.7624999998514,10.3459381770593));
#300829=CARTESIAN_POINT('Ctrl Pts',(9.83957192047904,39.9124999998508,7.14886745759543));
#300830=CARTESIAN_POINT('Ctrl Pts',(12.1623797632103,40.0624999998502,3.95179673813153));
#300831=CARTESIAN_POINT('Ctrl Pts',(12.1623797632103,40.2124999998496,-1.489461944703E-15));
#300832=CARTESIAN_POINT('Ctrl Pts',(12.1623797632103,40.362499999849,-3.95179673813154));
#300833=CARTESIAN_POINT('Ctrl Pts',(9.83957192047904,40.5124999998484,-7.14886745759543));
#300834=CARTESIAN_POINT('Ctrl Pts',(7.51676407774782,40.6624999998478,-10.3459381770593));
#300835=CARTESIAN_POINT('Ctrl Pts',(3.75838203887389,40.8124999998472,-11.5671105274575));
#300836=CARTESIAN_POINT('Ctrl Pts',(-3.68511102503695E-14,40.9624999998466,
-12.7882828778556));
#300837=CARTESIAN_POINT('Ctrl Pts',(-3.75838203887397,41.112499999846,-11.5671105274575));
#300838=CARTESIAN_POINT('Ctrl Pts',(-7.51676407774789,41.2624999998454,
-10.3459381770593));
#300839=CARTESIAN_POINT('Ctrl Pts',(-9.83957192047911,41.4124999998448,
-7.14886745759543));
#300840=CARTESIAN_POINT('Ctrl Pts',(-12.1623797632103,41.5624999998442,
-3.95179673813153));
#300841=CARTESIAN_POINT('Ctrl Pts',(-12.1623797632103,41.7124999998436,
2.97892388940601E-15));
#300842=CARTESIAN_POINT('Ctrl Pts',(-12.1623797632103,41.862499999843,3.95179673813154));
#300843=CARTESIAN_POINT('Ctrl Pts',(-9.83957192047911,42.0124999998424,
7.14886745759543));
#300844=CARTESIAN_POINT('Ctrl Pts',(-7.51676407774789,42.1624999998418,
10.3459381770593));
#300845=CARTESIAN_POINT('Ctrl Pts',(-3.75838203887396,42.3124999998412,
11.5671105274575));
#300846=CARTESIAN_POINT('Ctrl Pts',(-3.4582738947609E-14,42.4624999998406,
12.7882828778556));
#300847=CARTESIAN_POINT('Ctrl Pts',(3.75838203887389,42.61249999984,11.5671105274575));
#300848=CARTESIAN_POINT('Ctrl Pts',(7.51676407774782,42.7624999998394,10.3459381770593));
#300849=CARTESIAN_POINT('Ctrl Pts',(9.83957192047904,42.9124999998388,7.14886745759543));
#300850=CARTESIAN_POINT('Ctrl Pts',(12.1623797632103,43.0624999998382,3.95179673813153));
#300851=CARTESIAN_POINT('Ctrl Pts',(12.1623797632103,43.2124999998376,-1.489461944703E-15));
#300852=CARTESIAN_POINT('Ctrl Pts',(12.1623797632103,43.362499999837,-3.95179673813154));
#300853=CARTESIAN_POINT('Ctrl Pts',(9.83957192047903,43.5124999998364,-7.14886745759543));
#300854=CARTESIAN_POINT('Ctrl Pts',(7.51676407774782,43.6624999998358,-10.3459381770593));
#300855=CARTESIAN_POINT('Ctrl Pts',(3.75838203887389,43.8124999998352,-11.5671105274575));
#300856=CARTESIAN_POINT('Ctrl Pts',(-3.85788195220313E-14,43.9624999998346,
-12.7882828778556));
#300857=CARTESIAN_POINT('Ctrl Pts',(-3.75838203887397,44.112499999834,-11.5671105274575));
#300858=CARTESIAN_POINT('Ctrl Pts',(-7.5167640777479,44.2624999998334,-10.3459381770593));
#300859=CARTESIAN_POINT('Ctrl Pts',(-9.83957192047911,44.4124999998328,
-7.14886745759543));
#300860=CARTESIAN_POINT('Ctrl Pts',(-12.1623797632103,44.5624999998322,
-3.95179673813153));
#300861=CARTESIAN_POINT('Ctrl Pts',(-12.1623797632103,44.7124999998316,
2.97892388940601E-15));
#300862=CARTESIAN_POINT('Ctrl Pts',(-12.1623797632103,44.862499999831,3.95179673813154));
#300863=CARTESIAN_POINT('Ctrl Pts',(-9.83957192047911,45.0124999998304,
7.14886745759543));
#300864=CARTESIAN_POINT('Ctrl Pts',(-7.51676407774789,45.1624999998298,
10.3459381770593));
#300865=CARTESIAN_POINT('Ctrl Pts',(-3.75838203887397,45.3124999998292,
11.5671105274575));
#300866=CARTESIAN_POINT('Ctrl Pts',(-3.63104482192709E-14,45.4624999998286,
12.7882828778556));
#300867=CARTESIAN_POINT('Ctrl Pts',(3.75838203887389,45.612499999828,11.5671105274575));
#300868=CARTESIAN_POINT('Ctrl Pts',(7.51676407774782,45.7624999998274,10.3459381770593));
#300869=CARTESIAN_POINT('Ctrl Pts',(9.83957192047904,45.9124999998268,7.14886745759543));
#300870=CARTESIAN_POINT('Ctrl Pts',(12.1623797632103,46.0624999998262,3.95179673813153));
#300871=CARTESIAN_POINT('Ctrl Pts',(12.1623797632103,46.2124999998256,-1.489461944703E-15));
#300872=CARTESIAN_POINT('Ctrl Pts',(12.1623797632103,46.362499999825,-3.95179673813154));
#300873=CARTESIAN_POINT('Ctrl Pts',(9.83957192047903,46.5124999998244,-7.14886745759543));
#300874=CARTESIAN_POINT('Ctrl Pts',(7.51676407774782,46.6624999998238,-10.3459381770593));
#300875=CARTESIAN_POINT('Ctrl Pts',(3.75838203887389,46.8124999998232,-11.5671105274575));
#300876=CARTESIAN_POINT('Ctrl Pts',(-4.03065287936931E-14,46.9624999998226,
-12.7882828778556));
#300877=CARTESIAN_POINT('Ctrl Pts',(-3.75838203887397,47.112499999822,-11.5671105274575));
#300878=CARTESIAN_POINT('Ctrl Pts',(-7.5167640777479,47.2624999998214,-10.3459381770593));
#300879=CARTESIAN_POINT('Ctrl Pts',(-9.83957192047912,47.4124999998208,
-7.14886745759543));
#300880=CARTESIAN_POINT('Ctrl Pts',(-12.1623797632103,47.5624999998202,
-3.95179673813153));
#300881=CARTESIAN_POINT('Ctrl Pts',(-12.1623797632103,47.7124999998196,
2.97892388940601E-15));
#300882=CARTESIAN_POINT('Ctrl Pts',(-12.1623797632103,47.862499999819,3.95179673813154));
#300883=CARTESIAN_POINT('Ctrl Pts',(-9.83957192047911,48.0124999998184,
7.14886745759543));
#300884=CARTESIAN_POINT('Ctrl Pts',(-7.51676407774789,48.1624999998178,
10.3459381770593));
#300885=CARTESIAN_POINT('Ctrl Pts',(-3.75838203887397,48.3124999998172,
11.5671105274575));
#300886=CARTESIAN_POINT('Ctrl Pts',(-3.80381574909327E-14,48.4624999998166,
12.7882828778556));
#300887=CARTESIAN_POINT('Ctrl Pts',(3.75838203887389,48.612499999816,11.5671105274575));
#300888=CARTESIAN_POINT('Ctrl Pts',(7.51676407774782,48.7624999998154,10.3459381770593));
#300889=CARTESIAN_POINT('Ctrl Pts',(9.83957192047903,48.9124999998148,7.14886745759543));
#300890=CARTESIAN_POINT('Ctrl Pts',(12.1623797632103,49.0624999998142,3.95179673813153));
#300891=CARTESIAN_POINT('Ctrl Pts',(12.1623797632103,49.2124999998136,-1.489461944703E-15));
#300892=CARTESIAN_POINT('Ctrl Pts',(12.1623797632103,49.362499999813,-3.95179673813154));
#300893=CARTESIAN_POINT('Ctrl Pts',(9.83957192047903,49.5124999998124,-7.14886745759543));
#300894=CARTESIAN_POINT('Ctrl Pts',(7.51676407774782,49.6624999998118,-10.3459381770593));
#300895=CARTESIAN_POINT('Ctrl Pts',(3.75838203887389,49.8124999998112,-11.5671105274575));
#300896=CARTESIAN_POINT('Ctrl Pts',(-4.2034238065355E-14,49.9624999998106,
-12.7882828778556));
#300897=CARTESIAN_POINT('Ctrl Pts',(-3.75838203887397,50.11249999981,-11.5671105274575));
#300898=CARTESIAN_POINT('Ctrl Pts',(-7.5167640777479,50.2624999998094,-10.3459381770593));
#300899=CARTESIAN_POINT('Ctrl Pts',(-9.83957192047912,50.4124999998088,
-7.14886745759543));
#300900=CARTESIAN_POINT('Ctrl Pts',(-12.1623797632103,50.5624999998082,
-3.95179673813153));
#300901=CARTESIAN_POINT('Ctrl Pts',(-12.1623797632103,50.7124999998076,
2.97892388940601E-15));
#300902=CARTESIAN_POINT('Ctrl Pts',(-12.1623797632103,50.862499999807,3.95179673813154));
#300903=CARTESIAN_POINT('Ctrl Pts',(-9.83957192047912,51.0124999998064,
7.14886745759543));
#300904=CARTESIAN_POINT('Ctrl Pts',(-7.5167640777479,51.1624999998058,10.3459381770593));
#300905=CARTESIAN_POINT('Ctrl Pts',(-3.75838203887397,51.3124999998052,
11.5671105274575));
#300906=CARTESIAN_POINT('Ctrl Pts',(-3.97658667625946E-14,51.4624999998046,
12.7882828778556));
#300907=CARTESIAN_POINT('Ctrl Pts',(3.75838203887389,51.612499999804,11.5671105274575));
#300908=CARTESIAN_POINT('Ctrl Pts',(7.51676407774782,51.7624999998034,10.3459381770593));
#300909=CARTESIAN_POINT('Ctrl Pts',(9.83957192047903,51.9124999998028,7.14886745759543));
#300910=CARTESIAN_POINT('Ctrl Pts',(12.1623797632103,52.0624999998022,3.95179673813153));
#300911=CARTESIAN_POINT('Ctrl Pts',(12.1623797632103,52.2124999998016,-1.489461944703E-15));
#300912=CARTESIAN_POINT('Ctrl Pts',(12.1623797632103,52.362499999801,-3.95179673813154));
#300913=CARTESIAN_POINT('Ctrl Pts',(9.83957192047903,52.5124999998004,-7.14886745759543));
#300914=CARTESIAN_POINT('Ctrl Pts',(7.51676407774781,52.6624999997998,-10.3459381770593));
#300915=CARTESIAN_POINT('Ctrl Pts',(3.75838203887388,52.8124999997992,-11.5671105274575));
#300916=CARTESIAN_POINT('Ctrl Pts',(-4.37619473370168E-14,52.9624999997986,
-12.7882828778556));
#300917=CARTESIAN_POINT('Ctrl Pts',(-3.75838203887397,53.112499999798,-11.5671105274575));
#300918=CARTESIAN_POINT('Ctrl Pts',(-7.5167640777479,53.2624999997974,-10.3459381770593));
#300919=CARTESIAN_POINT('Ctrl Pts',(-9.83957192047912,53.4124999997968,
-7.14886745759543));
#300920=CARTESIAN_POINT('Ctrl Pts',(-12.1623797632103,53.5624999997962,
-3.95179673813153));
#300921=CARTESIAN_POINT('Ctrl Pts',(-12.1623797632103,53.7124999997956,
2.97892388940601E-15));
#300922=CARTESIAN_POINT('Ctrl Pts',(-12.1623797632103,53.862499999795,3.95179673813154));
#300923=CARTESIAN_POINT('Ctrl Pts',(-9.83957192047912,54.0124999997944,
7.14886745759543));
#300924=CARTESIAN_POINT('Ctrl Pts',(-7.5167640777479,54.1624999997938,10.3459381770593));
#300925=CARTESIAN_POINT('Ctrl Pts',(-3.75838203887397,54.3124999997932,
11.5671105274575));
#300926=CARTESIAN_POINT('Ctrl Pts',(-4.14935760342564E-14,54.4624999997926,
12.7882828778556));
#300927=CARTESIAN_POINT('Ctrl Pts',(3.75838203887389,54.612499999792,11.5671105274575));
#300928=CARTESIAN_POINT('Ctrl Pts',(7.51676407774782,54.7624999997914,10.3459381770593));
#300929=CARTESIAN_POINT('Ctrl Pts',(9.83957192047903,54.9124999997908,7.14886745759543));
#300930=CARTESIAN_POINT('Ctrl Pts',(12.1623797632103,55.0624999997902,3.95179673813153));
#300931=CARTESIAN_POINT('Ctrl Pts',(12.1623797632103,55.2124999997896,-1.489461944703E-15));
#300932=CARTESIAN_POINT('Ctrl Pts',(12.1623797632103,55.362499999789,-3.95179673813154));
#300933=CARTESIAN_POINT('Ctrl Pts',(9.83957192047903,55.5124999997884,-7.14886745759543));
#300934=CARTESIAN_POINT('Ctrl Pts',(7.51676407774781,55.6624999997878,-10.3459381770593));
#300935=CARTESIAN_POINT('Ctrl Pts',(3.75838203887388,55.8124999997872,-11.5671105274575));
#300936=CARTESIAN_POINT('Ctrl Pts',(-4.54896566086787E-14,55.9624999997866,
-12.7882828778556));
#300937=CARTESIAN_POINT('Ctrl Pts',(-3.75838203887397,56.112499999786,-11.5671105274575));
#300938=CARTESIAN_POINT('Ctrl Pts',(-7.5167640777479,56.2624999997854,-10.3459381770593));
#300939=CARTESIAN_POINT('Ctrl Pts',(-9.83957192047912,56.4124999997848,
-7.14886745759543));
#300940=CARTESIAN_POINT('Ctrl Pts',(-12.1623797632103,56.5624999997842,
-3.95179673813153));
#300941=CARTESIAN_POINT('Ctrl Pts',(-12.1623797632103,56.7124999997836,
2.97892388940601E-15));
#300942=CARTESIAN_POINT('Ctrl Pts',(-12.1623797632103,56.862499999783,3.95179673813154));
#300943=CARTESIAN_POINT('Ctrl Pts',(-9.83957192047912,57.0124999997824,
7.14886745759543));
#300944=CARTESIAN_POINT('Ctrl Pts',(-7.5167640777479,57.1624999997818,10.3459381770593));
#300945=CARTESIAN_POINT('Ctrl Pts',(-3.75838203887397,57.3124999997812,
11.5671105274575));
#300946=CARTESIAN_POINT('Ctrl Pts',(-4.32212853059182E-14,57.4624999997806,
12.7882828778556));
#300947=CARTESIAN_POINT('Ctrl Pts',(3.75838203887389,57.61249999978,11.5671105274575));
#300948=CARTESIAN_POINT('Ctrl Pts',(7.51676407774781,57.7624999997794,10.3459381770593));
#300949=CARTESIAN_POINT('Ctrl Pts',(9.83957192047903,57.9124999997788,7.14886745759543));
#300950=CARTESIAN_POINT('Ctrl Pts',(12.1623797632103,58.0624999997782,3.95179673813153));
#300951=CARTESIAN_POINT('Ctrl Pts',(12.1623797632102,58.2124999997776,-1.489461944703E-15));
#300952=CARTESIAN_POINT('Ctrl Pts',(12.1623797632102,58.362499999777,-3.95179673813154));
#300953=CARTESIAN_POINT('Ctrl Pts',(9.83957192047903,58.5124999997764,-7.14886745759543));
#300954=CARTESIAN_POINT('Ctrl Pts',(7.51676407774781,58.6624999997758,-10.3459381770593));
#300955=CARTESIAN_POINT('Ctrl Pts',(3.75838203887388,58.8124999997752,-11.5671105274575));
#300956=CARTESIAN_POINT('Ctrl Pts',(-4.72173658803405E-14,58.9624999997746,
-12.7882828778556));
#300957=CARTESIAN_POINT('Ctrl Pts',(-3.75838203887398,59.112499999774,-11.5671105274575));
#300958=CARTESIAN_POINT('Ctrl Pts',(-7.51676407774791,59.2624999997734,
-10.3459381770593));
#300959=CARTESIAN_POINT('Ctrl Pts',(-9.83957192047912,59.4124999997728,
-7.14886745759543));
#300960=CARTESIAN_POINT('Ctrl Pts',(-12.1623797632103,59.5624999997722,
-3.95179673813153));
#300961=CARTESIAN_POINT('Ctrl Pts',(-12.1623797632103,59.7124999997716,
2.97892388940601E-15));
#300962=CARTESIAN_POINT('Ctrl Pts',(-12.1623797632103,59.862499999771,3.95179673813154));
#300963=CARTESIAN_POINT('Ctrl Pts',(-9.83957192047912,60.0124999997704,
7.14886745759543));
#300964=CARTESIAN_POINT('Ctrl Pts',(-7.5167640777479,60.1624999997698,10.3459381770593));
#300965=CARTESIAN_POINT('Ctrl Pts',(-3.75838203887397,60.3124999997692,
11.5671105274575));
#300966=CARTESIAN_POINT('Ctrl Pts',(-4.49489945775801E-14,60.4624999997686,
12.7882828778556));
#300967=CARTESIAN_POINT('Ctrl Pts',(3.75838203887388,60.612499999768,11.5671105274575));
#300968=CARTESIAN_POINT('Ctrl Pts',(7.51676407774781,60.7624999997674,10.3459381770593));
#300969=CARTESIAN_POINT('Ctrl Pts',(9.83957192047903,60.9124999997668,7.14886745759543));
#300970=CARTESIAN_POINT('Ctrl Pts',(12.1623797632103,61.0624999997662,3.95179673813153));
#300971=CARTESIAN_POINT('Ctrl Pts',(12.1623797632102,61.2124999997656,-1.489461944703E-15));
#300972=CARTESIAN_POINT('Ctrl Pts',(12.1623797632102,61.362499999765,-3.95179673813154));
#300973=CARTESIAN_POINT('Ctrl Pts',(9.83957192047902,61.5124999997644,-7.14886745759543));
#300974=CARTESIAN_POINT('Ctrl Pts',(7.51676407774781,61.6624999997638,-10.3459381770593));
#300975=CARTESIAN_POINT('Ctrl Pts',(3.75838203887388,61.8124999997632,-11.5671105274575));
#300976=CARTESIAN_POINT('Ctrl Pts',(-4.89450751520023E-14,61.9624999997626,
-12.7882828778556));
#300977=CARTESIAN_POINT('Ctrl Pts',(-3.75838203887398,62.112499999762,-11.5671105274575));
#300978=CARTESIAN_POINT('Ctrl Pts',(-7.51676407774791,62.2624999997614,
-10.3459381770593));
#300979=CARTESIAN_POINT('Ctrl Pts',(-9.83957192047912,62.4124999997608,
-7.14886745759543));
#300980=CARTESIAN_POINT('Ctrl Pts',(-12.1623797632103,62.5624999997602,
-3.95179673813153));
#300981=CARTESIAN_POINT('Ctrl Pts',(-12.1623797632103,62.7124999997596,
2.97892388940601E-15));
#300982=CARTESIAN_POINT('Ctrl Pts',(-12.1623797632103,62.862499999759,3.95179673813154));
#300983=CARTESIAN_POINT('Ctrl Pts',(-9.83957192047912,63.0124999997584,
7.14886745759543));
#300984=CARTESIAN_POINT('Ctrl Pts',(-7.5167640777479,63.1624999997578,10.3459381770593));
#300985=CARTESIAN_POINT('Ctrl Pts',(-3.75838203887398,63.3124999997572,
11.5671105274575));
#300986=CARTESIAN_POINT('Ctrl Pts',(-4.66767038492419E-14,63.4624999997566,
12.7882828778556));
#300987=CARTESIAN_POINT('Ctrl Pts',(3.75838203887388,63.612499999756,11.5671105274575));
#300988=CARTESIAN_POINT('Ctrl Pts',(7.51676407774781,63.7624999997554,10.3459381770593));
#300989=CARTESIAN_POINT('Ctrl Pts',(9.83957192047903,63.9124999997548,7.14886745759543));
#300990=CARTESIAN_POINT('Ctrl Pts',(12.1623797632102,64.0624999997542,3.95179673813153));
#300991=CARTESIAN_POINT('Ctrl Pts',(12.1623797632102,64.2124999997536,-1.489461944703E-15));
#300992=CARTESIAN_POINT('Ctrl Pts',(12.1623797632102,64.362499999753,-3.95179673813154));
#300993=CARTESIAN_POINT('Ctrl Pts',(9.83957192047902,64.5124999997524,-7.14886745759543));
#300994=CARTESIAN_POINT('Ctrl Pts',(7.51676407774781,64.6624999997518,-10.3459381770593));
#300995=CARTESIAN_POINT('Ctrl Pts',(3.75838203887388,64.8124999997512,-11.5671105274575));
#300996=CARTESIAN_POINT('Ctrl Pts',(-5.06727844236642E-14,64.9624999997506,
-12.7882828778556));
#300997=CARTESIAN_POINT('Ctrl Pts',(-3.75838203887398,65.11249999975,-11.5671105274575));
#300998=CARTESIAN_POINT('Ctrl Pts',(-7.51676407774791,65.2624999997494,
-10.3459381770593));
#300999=CARTESIAN_POINT('Ctrl Pts',(-9.83957192047913,65.4124999997488,
-7.14886745759543));
#301000=CARTESIAN_POINT('Ctrl Pts',(-12.1623797632103,65.5624999997482,
-3.95179673813153));
#301001=CARTESIAN_POINT('Ctrl Pts',(-12.1623797632103,65.7124999997476,
2.97892388940601E-15));
#301002=CARTESIAN_POINT('Ctrl Pts',(-12.1623797632103,65.862499999747,3.95179673813154));
#301003=CARTESIAN_POINT('Ctrl Pts',(-9.83957192047912,66.0124999997464,
7.14886745759543));
#301004=CARTESIAN_POINT('Ctrl Pts',(-7.51676407774791,66.1624999997458,
10.3459381770593));
#301005=CARTESIAN_POINT('Ctrl Pts',(-3.75838203887398,66.3124999997452,
11.5671105274575));
#301006=CARTESIAN_POINT('Ctrl Pts',(-4.84044131209037E-14,66.4624999997446,
12.7882828778556));
#301007=CARTESIAN_POINT('Ctrl Pts',(3.75838203887388,66.612499999744,11.5671105274575));
#301008=CARTESIAN_POINT('Ctrl Pts',(7.51676407774781,66.7624999997434,10.3459381770593));
#301009=CARTESIAN_POINT('Ctrl Pts',(9.83957192047902,66.9124999997428,7.14886745759543));
#301010=CARTESIAN_POINT('Ctrl Pts',(12.1623797632102,67.0624999997422,3.95179673813153));
#301011=CARTESIAN_POINT('Ctrl Pts',(12.1623797632102,67.2124999997416,-1.489461944703E-15));
#301012=CARTESIAN_POINT('Ctrl Pts',(12.1623797632102,67.362499999741,-3.95179673813154));
#301013=CARTESIAN_POINT('Ctrl Pts',(9.83957192047902,67.5124999997404,-7.14886745759543));
#301014=CARTESIAN_POINT('Ctrl Pts',(7.51676407774781,67.6624999997398,-10.3459381770593));
#301015=CARTESIAN_POINT('Ctrl Pts',(3.75838203887388,67.8124999997392,-11.5671105274575));
#301016=CARTESIAN_POINT('Ctrl Pts',(-5.2400493695326E-14,67.9624999997386,
-12.7882828778556));
#301017=CARTESIAN_POINT('Ctrl Pts',(-3.75838203887398,68.112499999738,-11.5671105274575));
#301018=CARTESIAN_POINT('Ctrl Pts',(-7.51676407774791,68.2624999997374,
-10.3459381770593));
#301019=CARTESIAN_POINT('Ctrl Pts',(-9.83957192047913,68.4124999997368,
-7.14886745759543));
#301020=CARTESIAN_POINT('Ctrl Pts',(-12.1623797632103,68.5624999997362,
-3.95179673813153));
#301021=CARTESIAN_POINT('Ctrl Pts',(-12.1623797632103,68.7124999997356,
2.97892388940601E-15));
#301022=CARTESIAN_POINT('Ctrl Pts',(-12.1623797632103,68.862499999735,3.95179673813154));
#301023=CARTESIAN_POINT('Ctrl Pts',(-9.83957192047913,69.0124999997344,
7.14886745759543));
#301024=CARTESIAN_POINT('Ctrl Pts',(-7.51676407774791,69.1624999997338,
10.3459381770593));
#301025=CARTESIAN_POINT('Ctrl Pts',(-3.75838203887398,69.3124999997332,
11.5671105274575));
#301026=CARTESIAN_POINT('Ctrl Pts',(-5.01321223925656E-14,69.4624999997326,
12.7882828778556));
#301027=CARTESIAN_POINT('Ctrl Pts',(3.75838203887388,69.612499999732,11.5671105274575));
#301028=CARTESIAN_POINT('Ctrl Pts',(7.51676407774781,69.7624999997314,10.3459381770593));
#301029=CARTESIAN_POINT('Ctrl Pts',(9.83957192047902,69.9124999997308,7.14886745759543));
#301030=CARTESIAN_POINT('Ctrl Pts',(12.1623797632102,70.0624999997302,3.95179673813153));
#301031=CARTESIAN_POINT('Ctrl Pts',(12.1623797632102,70.2124999997296,-1.489461944703E-15));
#301032=CARTESIAN_POINT('Ctrl Pts',(12.1623797632102,70.362499999729,-3.95179673813154));
#301033=CARTESIAN_POINT('Ctrl Pts',(9.83957192047902,70.5124999997284,-7.14886745759543));
#301034=CARTESIAN_POINT('Ctrl Pts',(7.5167640777478,70.6624999997278,-10.3459381770593));
#301035=CARTESIAN_POINT('Ctrl Pts',(3.75838203887388,70.8124999997272,-11.5671105274575));
#301036=CARTESIAN_POINT('Ctrl Pts',(-5.41282029669879E-14,70.9624999997266,
-12.7882828778556));
#301037=CARTESIAN_POINT('Ctrl Pts',(-3.75838203887398,71.112499999726,-11.5671105274575));
#301038=CARTESIAN_POINT('Ctrl Pts',(-7.51676407774791,71.2624999997254,
-10.3459381770593));
#301039=CARTESIAN_POINT('Ctrl Pts',(-9.83957192047913,71.4124999997248,
-7.14886745759543));
#301040=CARTESIAN_POINT('Ctrl Pts',(-12.1623797632103,71.5624999997242,
-3.95179673813153));
#301041=CARTESIAN_POINT('Ctrl Pts',(-12.1623797632103,71.7124999997236,
2.97892388940601E-15));
#301042=CARTESIAN_POINT('Ctrl Pts',(-12.1623797632103,71.862499999723,3.95179673813154));
#301043=CARTESIAN_POINT('Ctrl Pts',(-9.83957192047913,72.0124999997224,
7.14886745759543));
#301044=CARTESIAN_POINT('Ctrl Pts',(-7.51676407774791,72.1624999997218,
10.3459381770593));
#301045=CARTESIAN_POINT('Ctrl Pts',(-3.75838203887398,72.3124999997212,
11.5671105274575));
#301046=CARTESIAN_POINT('Ctrl Pts',(-5.18598316642274E-14,72.4624999997206,
12.7882828778556));
#301047=CARTESIAN_POINT('Ctrl Pts',(3.75838203887388,72.61249999972,11.5671105274575));
#301048=CARTESIAN_POINT('Ctrl Pts',(7.51676407774781,72.7624999997194,10.3459381770593));
#301049=CARTESIAN_POINT('Ctrl Pts',(9.83957192047902,72.9124999997188,7.14886745759543));
#301050=CARTESIAN_POINT('Ctrl Pts',(12.1623797632102,73.0624999997182,3.95179673813153));
#301051=CARTESIAN_POINT('Ctrl Pts',(12.1623797632102,73.2124999997176,-1.489461944703E-15));
#301052=CARTESIAN_POINT('Ctrl Pts',(12.1623797632102,73.362499999717,-3.95179673813154));
#301053=CARTESIAN_POINT('Ctrl Pts',(9.83957192047902,73.5124999997164,-7.14886745759543));
#301054=CARTESIAN_POINT('Ctrl Pts',(7.5167640777478,73.6624999997158,-10.3459381770593));
#301055=CARTESIAN_POINT('Ctrl Pts',(3.75838203887387,73.8124999997152,-11.5671105274575));
#301056=CARTESIAN_POINT('Ctrl Pts',(-5.58559122386497E-14,73.9624999997146,
-12.7882828778556));
#301057=CARTESIAN_POINT('Ctrl Pts',(-3.75838203887398,74.112499999714,-11.5671105274575));
#301058=CARTESIAN_POINT('Ctrl Pts',(-7.51676407774791,74.2624999997134,
-10.3459381770593));
#301059=CARTESIAN_POINT('Ctrl Pts',(-9.83957192047913,74.4124999997128,
-7.14886745759543));
#301060=CARTESIAN_POINT('Ctrl Pts',(-12.1623797632103,74.5624999997122,
-3.95179673813153));
#301061=CARTESIAN_POINT('Ctrl Pts',(-12.1623797632103,74.7124999997116,
2.97892388940601E-15));
#301062=CARTESIAN_POINT('Ctrl Pts',(-12.1623797632103,74.862499999711,3.95179673813154));
#301063=CARTESIAN_POINT('Ctrl Pts',(-9.83957192047913,75.0124999997104,
7.14886745759543));
#301064=CARTESIAN_POINT('Ctrl Pts',(-7.51676407774791,75.1624999997098,
10.3459381770593));
#301065=CARTESIAN_POINT('Ctrl Pts',(-3.75838203887398,75.3124999997092,
11.5671105274575));
#301066=CARTESIAN_POINT('Ctrl Pts',(-5.35875409358893E-14,75.4624999997086,
12.7882828778556));
#301067=CARTESIAN_POINT('Ctrl Pts',(3.75838203887388,75.612499999708,11.5671105274575));
#301068=CARTESIAN_POINT('Ctrl Pts',(7.5167640777478,75.7624999997074,10.3459381770593));
#301069=CARTESIAN_POINT('Ctrl Pts',(9.83957192047902,75.9124999997068,7.14886745759543));
#301070=CARTESIAN_POINT('Ctrl Pts',(12.1623797632102,76.0624999997062,3.95179673813153));
#301071=CARTESIAN_POINT('Ctrl Pts',(12.1623797632102,76.2124999997056,-1.489461944703E-15));
#301072=CARTESIAN_POINT('Ctrl Pts',(12.1623797632102,76.362499999705,-3.95179673813154));
#301073=CARTESIAN_POINT('Ctrl Pts',(9.83957192047902,76.5124999997044,-7.14886745759543));
#301074=CARTESIAN_POINT('Ctrl Pts',(7.5167640777478,76.6624999997038,-10.3459381770593));
#301075=CARTESIAN_POINT('Ctrl Pts',(3.75838203887387,76.8124999997032,-11.5671105274575));
#301076=CARTESIAN_POINT('Ctrl Pts',(-5.75836215103115E-14,76.9624999997026,
-12.7882828778556));
#301077=CARTESIAN_POINT('Ctrl Pts',(-3.75838203887399,77.112499999702,-11.5671105274575));
#301078=CARTESIAN_POINT('Ctrl Pts',(-7.51676407774791,77.2624999997014,
-10.3459381770593));
#301079=CARTESIAN_POINT('Ctrl Pts',(-9.83957192047913,77.4124999997008,
-7.14886745759543));
#301080=CARTESIAN_POINT('Ctrl Pts',(-12.1623797632103,77.5624999997002,
-3.95179673813153));
#301081=CARTESIAN_POINT('Ctrl Pts',(-12.1623797632103,77.7124999996996,
2.97892388940601E-15));
#301082=CARTESIAN_POINT('Ctrl Pts',(-12.1623797632103,77.862499999699,3.95179673813154));
#301083=CARTESIAN_POINT('Ctrl Pts',(-9.83957192047913,78.0124999996984,
7.14886745759543));
#301084=CARTESIAN_POINT('Ctrl Pts',(-7.51676407774791,78.1624999996978,
10.3459381770593));
#301085=CARTESIAN_POINT('Ctrl Pts',(-3.75838203887398,78.3124999996972,
11.5671105274575));
#301086=CARTESIAN_POINT('Ctrl Pts',(-5.53152502075511E-14,78.4624999996966,
12.7882828778556));
#301087=CARTESIAN_POINT('Ctrl Pts',(3.75838203887387,78.612499999696,11.5671105274575));
#301088=CARTESIAN_POINT('Ctrl Pts',(7.5167640777478,78.7624999996954,10.3459381770593));
#301089=CARTESIAN_POINT('Ctrl Pts',(9.83957192047902,78.9124999996948,7.14886745759543));
#301090=CARTESIAN_POINT('Ctrl Pts',(12.1623797632102,79.0624999996942,3.95179673813153));
#301091=CARTESIAN_POINT('Ctrl Pts',(12.1623797632102,79.2124999996936,-1.489461944703E-15));
#301092=CARTESIAN_POINT('Ctrl Pts',(12.1623797632102,79.362499999693,-3.95179673813154));
#301093=CARTESIAN_POINT('Ctrl Pts',(9.83957192047902,79.5124999996924,-7.14886745759543));
#301094=CARTESIAN_POINT('Ctrl Pts',(7.5167640777478,79.6624999996918,-10.3459381770593));
#301095=CARTESIAN_POINT('Ctrl Pts',(3.75838203887387,79.8124999996912,-11.5671105274575));
#301096=CARTESIAN_POINT('Ctrl Pts',(-5.93113307819734E-14,79.9624999996906,
-12.7882828778556));
#301097=CARTESIAN_POINT('Ctrl Pts',(-3.75838203887399,80.11249999969,-11.5671105274575));
#301098=CARTESIAN_POINT('Ctrl Pts',(-7.51676407774791,80.2624999996894,
-10.3459381770593));
#301099=CARTESIAN_POINT('Ctrl Pts',(-9.83957192047913,80.4124999996888,
-7.14886745759543));
#301100=CARTESIAN_POINT('Ctrl Pts',(-12.1623797632104,80.5624999996882,
-3.95179673813153));
#301101=CARTESIAN_POINT('Ctrl Pts',(-12.1623797632104,80.7124999996876,
2.97892388940601E-15));
#301102=CARTESIAN_POINT('Ctrl Pts',(-12.1623797632104,80.862499999687,3.95179673813154));
#301103=CARTESIAN_POINT('Ctrl Pts',(-9.83957192047913,81.0124999996864,
7.14886745759543));
#301104=CARTESIAN_POINT('Ctrl Pts',(-7.51676407774791,81.1624999996858,
10.3459381770593));
#301105=CARTESIAN_POINT('Ctrl Pts',(-3.75838203887399,81.3124999996852,
11.5671105274575));
#301106=CARTESIAN_POINT('Ctrl Pts',(-5.70429594792129E-14,81.4624999996846,
12.7882828778556));
#301107=CARTESIAN_POINT('Ctrl Pts',(3.75838203887387,81.612499999684,11.5671105274575));
#301108=CARTESIAN_POINT('Ctrl Pts',(7.5167640777478,81.7624999996834,10.3459381770593));
#301109=CARTESIAN_POINT('Ctrl Pts',(9.83957192047902,81.9124999996828,7.14886745759543));
#301110=CARTESIAN_POINT('Ctrl Pts',(12.1623797632102,82.0624999996822,3.95179673813153));
#301111=CARTESIAN_POINT('Ctrl Pts',(12.1623797632102,82.2124999996816,-1.489461944703E-15));
#301112=CARTESIAN_POINT('Ctrl Pts',(12.1623797632102,82.362499999681,-3.95179673813154));
#301113=CARTESIAN_POINT('Ctrl Pts',(9.83957192047902,82.5124999996804,-7.14886745759543));
#301114=CARTESIAN_POINT('Ctrl Pts',(7.5167640777478,82.6624999996798,-10.3459381770593));
#301115=CARTESIAN_POINT('Ctrl Pts',(3.75838203887387,82.8124999996792,-11.5671105274575));
#301116=CARTESIAN_POINT('Ctrl Pts',(-6.10390400536352E-14,82.9624999996786,
-12.7882828778556));
#301117=CARTESIAN_POINT('Ctrl Pts',(-3.75838203887399,83.112499999678,-11.5671105274575));
#301118=CARTESIAN_POINT('Ctrl Pts',(-7.51676407774792,83.2624999996774,
-10.3459381770593));
#301119=CARTESIAN_POINT('Ctrl Pts',(-9.83957192047914,83.4124999996768,
-7.14886745759543));
#301120=CARTESIAN_POINT('Ctrl Pts',(-12.1623797632104,83.5624999996762,
-3.95179673813153));
#301121=CARTESIAN_POINT('Ctrl Pts',(-12.1623797632104,83.7124999996756,
2.97892388940601E-15));
#301122=CARTESIAN_POINT('Ctrl Pts',(-12.1623797632104,83.862499999675,3.95179673813154));
#301123=CARTESIAN_POINT('Ctrl Pts',(-9.83957192047913,84.0124999996744,
7.14886745759543));
#301124=CARTESIAN_POINT('Ctrl Pts',(-7.51676407774791,84.1624999996738,
10.3459381770593));
#301125=CARTESIAN_POINT('Ctrl Pts',(-3.75838203887399,84.3124999996732,
11.5671105274575));
#301126=CARTESIAN_POINT('Ctrl Pts',(-5.87706687508748E-14,84.4624999996726,
12.7882828778556));
#301127=CARTESIAN_POINT('Ctrl Pts',(3.75838203887387,84.6124999996721,11.5671105274575));
#301128=CARTESIAN_POINT('Ctrl Pts',(7.5167640777478,84.7624999996714,10.3459381770593));
#301129=CARTESIAN_POINT('Ctrl Pts',(9.83957192047902,84.9124999996708,7.14886745759543));
#301130=CARTESIAN_POINT('Ctrl Pts',(12.1623797632102,85.0624999996702,3.95179673813153));
#301131=CARTESIAN_POINT('Ctrl Pts',(12.1623797632102,85.2124999996696,-1.489461944703E-15));
#301132=CARTESIAN_POINT('Ctrl Pts',(12.1623797632102,85.362499999669,-3.95179673813154));
#301133=CARTESIAN_POINT('Ctrl Pts',(9.83957192047901,85.5124999996684,-7.14886745759543));
#301134=CARTESIAN_POINT('Ctrl Pts',(7.5167640777478,85.6624999996678,-10.3459381770593));
#301135=CARTESIAN_POINT('Ctrl Pts',(3.75838203887387,85.8124999996672,-11.5671105274575));
#301136=CARTESIAN_POINT('Ctrl Pts',(-6.27667493252971E-14,85.9624999996666,
-12.7882828778556));
#301137=CARTESIAN_POINT('Ctrl Pts',(-3.75838203887399,86.112499999666,-11.5671105274575));
#301138=CARTESIAN_POINT('Ctrl Pts',(-7.51676407774792,86.2624999996654,
-10.3459381770593));
#301139=CARTESIAN_POINT('Ctrl Pts',(-9.83957192047914,86.4124999996648,
-7.14886745759543));
#301140=CARTESIAN_POINT('Ctrl Pts',(-12.1623797632104,86.5624999996642,
-3.95179673813153));
#301141=CARTESIAN_POINT('Ctrl Pts',(-12.1623797632104,86.7124999996636,
2.97892388940601E-15));
#301142=CARTESIAN_POINT('Ctrl Pts',(-12.1623797632104,86.862499999663,3.95179673813154));
#301143=CARTESIAN_POINT('Ctrl Pts',(-9.83957192047914,87.0124999996624,
7.14886745759543));
#301144=CARTESIAN_POINT('Ctrl Pts',(-7.51676407774792,87.1624999996618,
10.3459381770593));
#301145=CARTESIAN_POINT('Ctrl Pts',(-3.75838203887399,87.3124999996612,
11.5671105274575));
#301146=CARTESIAN_POINT('Ctrl Pts',(-6.04983780225366E-14,87.4624999996606,
12.7882828778556));
#301147=CARTESIAN_POINT('Ctrl Pts',(3.75838203887387,87.61249999966,11.5671105274575));
#301148=CARTESIAN_POINT('Ctrl Pts',(7.5167640777478,87.7624999996594,10.3459381770593));
#301149=CARTESIAN_POINT('Ctrl Pts',(9.83957192047901,87.9124999996588,7.14886745759543));
#301150=CARTESIAN_POINT('Ctrl Pts',(12.1623797632102,88.0624999996582,3.95179673813153));
#301151=CARTESIAN_POINT('Ctrl Pts',(12.1623797632102,88.2124999996576,-1.489461944703E-15));
#301152=CARTESIAN_POINT('Ctrl Pts',(12.1623797632102,88.362499999657,-3.95179673813154));
#301153=CARTESIAN_POINT('Ctrl Pts',(9.83957192047901,88.5124999996564,-7.14886745759543));
#301154=CARTESIAN_POINT('Ctrl Pts',(7.51676407774779,88.6624999996558,-10.3459381770593));
#301155=CARTESIAN_POINT('Ctrl Pts',(3.75838203887386,88.8124999996552,-11.5671105274575));
#301156=CARTESIAN_POINT('Ctrl Pts',(-6.44944585969589E-14,88.9624999996546,
-12.7882828778556));
#301157=CARTESIAN_POINT('Ctrl Pts',(-3.75838203887399,89.112499999654,-11.5671105274575));
#301158=CARTESIAN_POINT('Ctrl Pts',(-7.51676407774792,89.2624999996534,
-10.3459381770593));
#301159=CARTESIAN_POINT('Ctrl Pts',(-9.83957192047914,89.4124999996528,
-7.14886745759543));
#301160=CARTESIAN_POINT('Ctrl Pts',(-12.1623797632104,89.5624999996522,
-3.95179673813153));
#301161=CARTESIAN_POINT('Ctrl Pts',(-12.1623797632104,89.7124999996516,
2.97892388940601E-15));
#301162=CARTESIAN_POINT('Ctrl Pts',(-12.1623797632104,89.862499999651,3.95179673813154));
#301163=CARTESIAN_POINT('Ctrl Pts',(-9.83957192047914,90.0124999996504,
7.14886745759543));
#301164=CARTESIAN_POINT('Ctrl Pts',(-7.51676407774792,90.1624999996498,
10.3459381770593));
#301165=CARTESIAN_POINT('Ctrl Pts',(-3.75838203887399,90.3124999996492,
11.5671105274575));
#301166=CARTESIAN_POINT('Ctrl Pts',(-6.22260872941985E-14,90.4624999996486,
12.7882828778556));
#301167=CARTESIAN_POINT('Ctrl Pts',(3.75838203887387,90.612499999648,11.5671105274575));
#301168=CARTESIAN_POINT('Ctrl Pts',(7.5167640777478,90.7624999996474,10.3459381770593));
#301169=CARTESIAN_POINT('Ctrl Pts',(9.83957192047901,90.9124999996468,7.14886745759543));
#301170=CARTESIAN_POINT('Ctrl Pts',(12.1623797632102,91.0624999996462,3.95179673813153));
#301171=CARTESIAN_POINT('Ctrl Pts',(12.1623797632102,91.2124999996456,-1.489461944703E-15));
#301172=CARTESIAN_POINT('Ctrl Pts',(12.1623797632102,91.362499999645,-3.95179673813154));
#301173=CARTESIAN_POINT('Ctrl Pts',(9.83957192047901,91.5124999996444,-7.14886745759543));
#301174=CARTESIAN_POINT('Ctrl Pts',(7.51676407774779,91.6624999996438,-10.3459381770593));
#301175=CARTESIAN_POINT('Ctrl Pts',(3.75838203887386,91.8124999996432,-11.5671105274575));
#301176=CARTESIAN_POINT('Ctrl Pts',(-6.62221678686207E-14,91.9624999996426,
-12.7882828778556));
#301177=CARTESIAN_POINT('Ctrl Pts',(-3.75838203887399,92.112499999642,-11.5671105274575));
#301178=CARTESIAN_POINT('Ctrl Pts',(-7.51676407774792,92.2624999996414,
-10.3459381770593));
#301179=CARTESIAN_POINT('Ctrl Pts',(-9.83957192047914,92.4124999996408,
-7.14886745759543));
#301180=CARTESIAN_POINT('Ctrl Pts',(-12.1623797632104,92.5624999996402,
-3.95179673813153));
#301181=CARTESIAN_POINT('Ctrl Pts',(-12.1623797632104,92.7124999996396,
2.97892388940601E-15));
#301182=CARTESIAN_POINT('Ctrl Pts',(-12.1623797632104,92.862499999639,3.95179673813154));
#301183=CARTESIAN_POINT('Ctrl Pts',(-9.83957192047914,93.0124999996384,
7.14886745759543));
#301184=CARTESIAN_POINT('Ctrl Pts',(-7.51676407774792,93.1624999996378,
10.3459381770593));
#301185=CARTESIAN_POINT('Ctrl Pts',(-3.75838203887399,93.3124999996372,
11.5671105274575));
#301186=CARTESIAN_POINT('Ctrl Pts',(-6.39537965658603E-14,93.4624999996366,
12.7882828778556));
#301187=CARTESIAN_POINT('Ctrl Pts',(3.75838203887386,93.612499999636,11.5671105274575));
#301188=CARTESIAN_POINT('Ctrl Pts',(7.51676407774779,93.7624999996354,10.3459381770593));
#301189=CARTESIAN_POINT('Ctrl Pts',(9.83957192047901,93.9124999996348,7.14886745759543));
#301190=CARTESIAN_POINT('Ctrl Pts',(12.1623797632102,94.0624999996342,3.95179673813153));
#301191=CARTESIAN_POINT('Ctrl Pts',(12.1623797632102,94.2124999996336,-1.489461944703E-15));
#301192=CARTESIAN_POINT('Ctrl Pts',(12.1623797632102,94.362499999633,-3.95179673813154));
#301193=CARTESIAN_POINT('Ctrl Pts',(9.83957192047901,94.5124999996324,-7.14886745759543));
#301194=CARTESIAN_POINT('Ctrl Pts',(7.51676407774779,94.6624999996318,-10.3459381770593));
#301195=CARTESIAN_POINT('Ctrl Pts',(3.75838203887386,94.8124999996312,-11.5671105274575));
#301196=CARTESIAN_POINT('Ctrl Pts',(-6.79498771402825E-14,94.9624999996306,
-12.7882828778556));
#301197=CARTESIAN_POINT('Ctrl Pts',(-3.758382038874,95.11249999963,-11.5671105274575));
#301198=CARTESIAN_POINT('Ctrl Pts',(-7.51676407774792,95.2624999996294,
-10.3459381770593));
#301199=CARTESIAN_POINT('Ctrl Pts',(-9.83957192047914,95.4124999996288,
-7.14886745759543));
#301200=CARTESIAN_POINT('Ctrl Pts',(-12.1623797632104,95.5624999996282,
-3.95179673813153));
#301201=CARTESIAN_POINT('Ctrl Pts',(-12.1623797632104,95.7124999996276,
2.97892388940601E-15));
#301202=CARTESIAN_POINT('Ctrl Pts',(-12.1623797632104,95.862499999627,3.95179673813154));
#301203=CARTESIAN_POINT('Ctrl Pts',(-9.83957192047914,96.0124999996264,
7.14886745759543));
#301204=CARTESIAN_POINT('Ctrl Pts',(-7.51676407774792,96.1624999996258,
10.3459381770593));
#301205=CARTESIAN_POINT('Ctrl Pts',(-3.75838203887399,96.3124999996252,
11.5671105274575));
#301206=CARTESIAN_POINT('Ctrl Pts',(-6.56815058375222E-14,96.4624999996246,
12.7882828778556));
#301207=CARTESIAN_POINT('Ctrl Pts',(3.75838203887386,96.612499999624,11.5671105274575));
#301208=CARTESIAN_POINT('Ctrl Pts',(7.51676407774779,96.7624999996234,10.3459381770593));
#301209=CARTESIAN_POINT('Ctrl Pts',(9.83957192047901,96.9124999996228,7.14886745759543));
#301210=CARTESIAN_POINT('Ctrl Pts',(12.1623797632102,97.0624999996222,3.95179673813153));
#301211=CARTESIAN_POINT('Ctrl Pts',(12.1623797632102,97.2124999996216,-1.489461944703E-15));
#301212=CARTESIAN_POINT('Ctrl Pts',(12.1623797632102,97.3624999996211,-3.95179673813154));
#301213=CARTESIAN_POINT('Ctrl Pts',(9.83957192047901,97.5124999996204,-7.14886745759543));
#301214=CARTESIAN_POINT('Ctrl Pts',(7.51676407774779,97.6624999996198,-10.3459381770593));
#301215=CARTESIAN_POINT('Ctrl Pts',(3.75838203887386,97.8124999996192,-11.5671105274575));
#301216=CARTESIAN_POINT('Ctrl Pts',(-6.96775864119444E-14,97.9624999996187,
-12.7882828778556));
#301217=CARTESIAN_POINT('Ctrl Pts',(-3.758382038874,98.112499999618,-11.5671105274575));
#301218=CARTESIAN_POINT('Ctrl Pts',(-7.51676407774793,98.2624999996174,
-10.3459381770593));
#301219=CARTESIAN_POINT('Ctrl Pts',(-9.83957192047914,98.4124999996168,
-7.14886745759543));
#301220=CARTESIAN_POINT('Ctrl Pts',(-12.1623797632104,98.5624999996162,
-3.95179673813153));
#301221=CARTESIAN_POINT('Ctrl Pts',(-12.1623797632104,98.7124999996156,
2.97892388940601E-15));
#301222=CARTESIAN_POINT('Ctrl Pts',(-12.1623797632104,98.862499999615,3.95179673813154));
#301223=CARTESIAN_POINT('Ctrl Pts',(-9.83957192047914,99.0124999996144,
7.14886745759543));
#301224=CARTESIAN_POINT('Ctrl Pts',(-7.51676407774792,99.1624999996138,
10.3459381770593));
#301225=CARTESIAN_POINT('Ctrl Pts',(-3.758382038874,99.3124999996132,11.5671105274575));
#301226=CARTESIAN_POINT('Ctrl Pts',(-6.7409215109184E-14,99.4624999996126,
12.7882828778556));
#301227=CARTESIAN_POINT('Ctrl Pts',(3.75838203887386,99.612499999612,11.5671105274575));
#301228=CARTESIAN_POINT('Ctrl Pts',(7.51676407774779,99.7624999996114,10.3459381770593));
#301229=CARTESIAN_POINT('Ctrl Pts',(9.83957192047901,99.9124999996108,7.14886745759543));
#301230=CARTESIAN_POINT('Ctrl Pts',(12.1623797632102,100.06249999961,3.95179673813153));
#301231=CARTESIAN_POINT('Ctrl Pts',(12.1623797632102,100.21249999961,-1.489461944703E-15));
#301232=CARTESIAN_POINT('Ctrl Pts',(12.1623797632102,100.362499999609,-3.95179673813154));
#301233=CARTESIAN_POINT('Ctrl Pts',(9.839571920479,100.512499999608,-7.14886745759543));
#301234=CARTESIAN_POINT('Ctrl Pts',(7.51676407774779,100.662499999608,-10.3459381770593));
#301235=CARTESIAN_POINT('Ctrl Pts',(3.75838203887386,100.812499999607,-11.5671105274575));
#301236=CARTESIAN_POINT('Ctrl Pts',(-7.14052956836063E-14,100.962499999607,
-12.7882828778556));
#301237=CARTESIAN_POINT('Ctrl Pts',(-3.758382038874,101.112499999606,-11.5671105274575));
#301238=CARTESIAN_POINT('Ctrl Pts',(-7.51676407774793,101.262499999605,
-10.3459381770593));
#301239=CARTESIAN_POINT('Ctrl Pts',(-9.83957192047915,101.412499999605,
-7.14886745759543));
#301240=CARTESIAN_POINT('Ctrl Pts',(-12.1623797632104,101.562499999604,
-3.95179673813153));
#301241=CARTESIAN_POINT('Ctrl Pts',(-12.1623797632104,101.712499999604,
2.97892388940601E-15));
#301242=CARTESIAN_POINT('Ctrl Pts',(-12.1623797632104,101.862499999603,
3.95179673813154));
#301243=CARTESIAN_POINT('Ctrl Pts',(-9.83957192047914,102.012499999602,
7.14886745759543));
#301244=CARTESIAN_POINT('Ctrl Pts',(-7.51676407774793,102.162499999602,
10.3459381770593));
#301245=CARTESIAN_POINT('Ctrl Pts',(-3.758382038874,102.312499999601,11.5671105274575));
#301246=CARTESIAN_POINT('Ctrl Pts',(-6.91369243808458E-14,102.462499999601,
12.7882828778556));
#301247=CARTESIAN_POINT('Ctrl Pts',(3.75838203887386,102.6124999996,11.5671105274575));
#301248=CARTESIAN_POINT('Ctrl Pts',(7.51676407774779,102.762499999599,10.3459381770593));
#301249=CARTESIAN_POINT('Ctrl Pts',(9.839571920479,102.912499999599,7.14886745759543));
#301250=CARTESIAN_POINT('Ctrl Pts',(12.1623797632102,103.062499999598,3.95179673813153));
#301251=CARTESIAN_POINT('Ctrl Pts',(12.1623797632102,103.212499999598,-1.489461944703E-15));
#301252=CARTESIAN_POINT('Ctrl Pts',(12.1623797632102,103.362499999597,-3.95179673813154));
#301253=CARTESIAN_POINT('Ctrl Pts',(9.839571920479,103.512499999596,-7.14886745759543));
#301254=CARTESIAN_POINT('Ctrl Pts',(7.51676407774779,103.662499999596,-10.3459381770593));
#301255=CARTESIAN_POINT('Ctrl Pts',(3.75838203887386,103.812499999595,-11.5671105274575));
#301256=CARTESIAN_POINT('Ctrl Pts',(-7.31330049552681E-14,103.962499999595,
-12.7882828778556));
#301257=CARTESIAN_POINT('Ctrl Pts',(-3.758382038874,104.112499999594,-11.5671105274575));
#301258=CARTESIAN_POINT('Ctrl Pts',(-7.51676407774793,104.262499999593,
-10.3459381770593));
#301259=CARTESIAN_POINT('Ctrl Pts',(-9.83957192047915,104.412499999593,
-7.14886745759543));
#301260=CARTESIAN_POINT('Ctrl Pts',(-12.1623797632104,104.562499999592,
-3.95179673813153));
#301261=CARTESIAN_POINT('Ctrl Pts',(-12.1623797632104,104.712499999592,
2.97892388940601E-15));
#301262=CARTESIAN_POINT('Ctrl Pts',(-12.1623797632104,104.862499999591,
3.95179673813154));
#301263=CARTESIAN_POINT('Ctrl Pts',(-9.83957192047915,105.01249999959,7.14886745759543));
#301264=CARTESIAN_POINT('Ctrl Pts',(-7.51676407774793,105.16249999959,10.3459381770593));
#301265=CARTESIAN_POINT('Ctrl Pts',(-3.758382038874,105.312499999589,11.5671105274575));
#301266=CARTESIAN_POINT('Ctrl Pts',(-7.08646336525076E-14,105.462499999589,
12.7882828778556));
#301267=CARTESIAN_POINT('Ctrl Pts',(3.75838203887386,105.612499999588,11.5671105274575));
#301268=CARTESIAN_POINT('Ctrl Pts',(7.51676407774779,105.762499999587,10.3459381770593));
#301269=CARTESIAN_POINT('Ctrl Pts',(9.839571920479,105.912499999587,7.14886745759543));
#301270=CARTESIAN_POINT('Ctrl Pts',(12.1623797632102,106.062499999586,3.95179673813153));
#301271=CARTESIAN_POINT('Ctrl Pts',(12.1623797632102,106.212499999586,-1.489461944703E-15));
#301272=CARTESIAN_POINT('Ctrl Pts',(12.1623797632102,106.362499999585,-3.95179673813154));
#301273=CARTESIAN_POINT('Ctrl Pts',(9.839571920479,106.512499999584,-7.14886745759543));
#301274=CARTESIAN_POINT('Ctrl Pts',(7.51676407774778,106.662499999584,-10.3459381770593));
#301275=CARTESIAN_POINT('Ctrl Pts',(3.75838203887385,106.812499999583,-11.5671105274575));
#301276=CARTESIAN_POINT('Ctrl Pts',(-7.48607142269299E-14,106.962499999583,
-12.7882828778556));
#301277=CARTESIAN_POINT('Ctrl Pts',(-3.758382038874,107.112499999582,-11.5671105274575));
#301278=CARTESIAN_POINT('Ctrl Pts',(-7.51676407774793,107.262499999581,
-10.3459381770593));
#301279=CARTESIAN_POINT('Ctrl Pts',(-9.83957192047915,107.412499999581,
-7.14886745759543));
#301280=CARTESIAN_POINT('Ctrl Pts',(-12.1623797632104,107.56249999958,-3.95179673813153));
#301281=CARTESIAN_POINT('Ctrl Pts',(-12.1623797632104,107.71249999958,2.97892388940601E-15));
#301282=CARTESIAN_POINT('Ctrl Pts',(-12.1623797632104,107.862499999579,
3.95179673813154));
#301283=CARTESIAN_POINT('Ctrl Pts',(-9.83957192047915,108.012499999578,
7.14886745759543));
#301284=CARTESIAN_POINT('Ctrl Pts',(-7.51676407774793,108.162499999578,
10.3459381770593));
#301285=CARTESIAN_POINT('Ctrl Pts',(-3.758382038874,108.312499999577,11.5671105274575));
#301286=CARTESIAN_POINT('Ctrl Pts',(-7.25923429241695E-14,108.462499999577,
12.7882828778556));
#301287=CARTESIAN_POINT('Ctrl Pts',(3.75838203887386,108.612499999576,11.5671105274575));
#301288=CARTESIAN_POINT('Ctrl Pts',(7.51676407774779,108.762499999575,10.3459381770593));
#301289=CARTESIAN_POINT('Ctrl Pts',(9.839571920479,108.912499999575,7.14886745759543));
#301290=CARTESIAN_POINT('Ctrl Pts',(12.1623797632102,109.062499999574,3.95179673813153));
#301291=CARTESIAN_POINT('Ctrl Pts',(12.1623797632102,109.212499999574,-1.489461944703E-15));
#301292=CARTESIAN_POINT('Ctrl Pts',(12.1623797632102,109.362499999573,-3.95179673813154));
#301293=CARTESIAN_POINT('Ctrl Pts',(9.839571920479,109.512499999572,-7.14886745759543));
#301294=CARTESIAN_POINT('Ctrl Pts',(7.51676407774778,109.662499999572,-10.3459381770593));
#301295=CARTESIAN_POINT('Ctrl Pts',(3.75838203887385,109.812499999571,-11.5671105274575));
#301296=CARTESIAN_POINT('Ctrl Pts',(-7.65884234985918E-14,109.962499999571,
-12.7882828778556));
#301297=CARTESIAN_POINT('Ctrl Pts',(-3.75838203887401,110.11249999957,-11.5671105274575));
#301298=CARTESIAN_POINT('Ctrl Pts',(-7.51676407774793,110.262499999569,
-10.3459381770593));
#301299=CARTESIAN_POINT('Ctrl Pts',(-9.83957192047915,110.412499999569,
-7.14886745759543));
#301300=CARTESIAN_POINT('Ctrl Pts',(-12.1623797632104,110.562499999568,
-3.95179673813153));
#301301=CARTESIAN_POINT('Ctrl Pts',(-12.1623797632104,110.712499999568,
2.97892388940601E-15));
#301302=CARTESIAN_POINT('Ctrl Pts',(-12.1623797632104,110.862499999567,
3.95179673813154));
#301303=CARTESIAN_POINT('Ctrl Pts',(-9.83957192047915,111.012499999566,
7.14886745759543));
#301304=CARTESIAN_POINT('Ctrl Pts',(-7.51676407774793,111.162499999566,
10.3459381770593));
#301305=CARTESIAN_POINT('Ctrl Pts',(-3.758382038874,111.312499999565,11.5671105274575));
#301306=CARTESIAN_POINT('Ctrl Pts',(-7.43200521958313E-14,111.462499999565,
12.7882828778556));
#301307=CARTESIAN_POINT('Ctrl Pts',(3.75838203887385,111.612499999564,11.5671105274575));
#301308=CARTESIAN_POINT('Ctrl Pts',(7.51676407774778,111.762499999563,10.3459381770593));
#301309=CARTESIAN_POINT('Ctrl Pts',(9.839571920479,111.912499999563,7.14886745759543));
#301310=CARTESIAN_POINT('Ctrl Pts',(12.1623797632102,112.062499999562,3.95179673813153));
#301311=CARTESIAN_POINT('Ctrl Pts',(12.1623797632102,112.212499999562,-1.489461944703E-15));
#301312=CARTESIAN_POINT('Ctrl Pts',(12.1623797632102,112.362499999561,-3.95179673813154));
#301313=CARTESIAN_POINT('Ctrl Pts',(9.839571920479,112.51249999956,-7.14886745759543));
#301314=CARTESIAN_POINT('Ctrl Pts',(7.51676407774778,112.66249999956,-10.3459381770593));
#301315=CARTESIAN_POINT('Ctrl Pts',(3.75838203887385,112.812499999559,-11.5671105274575));
#301316=CARTESIAN_POINT('Ctrl Pts',(-7.83161327702536E-14,112.962499999559,
-12.7882828778556));
#301317=CARTESIAN_POINT('Ctrl Pts',(-3.75838203887401,113.112499999558,
-11.5671105274575));
#301318=CARTESIAN_POINT('Ctrl Pts',(-7.51676407774793,113.262499999557,
-10.3459381770593));
#301319=CARTESIAN_POINT('Ctrl Pts',(-9.83957192047915,113.412499999557,
-7.14886745759543));
#301320=CARTESIAN_POINT('Ctrl Pts',(-12.1623797632104,113.562499999556,
-3.95179673813153));
#301321=CARTESIAN_POINT('Ctrl Pts',(-12.1623797632104,113.712499999556,
2.97892388940601E-15));
#301322=CARTESIAN_POINT('Ctrl Pts',(-12.1623797632104,113.862499999555,
3.95179673813154));
#301323=CARTESIAN_POINT('Ctrl Pts',(-9.83957192047915,114.012499999554,
7.14886745759543));
#301324=CARTESIAN_POINT('Ctrl Pts',(-7.51676407774793,114.162499999554,
10.3459381770593));
#301325=CARTESIAN_POINT('Ctrl Pts',(-3.758382038874,114.312499999553,11.5671105274575));
#301326=CARTESIAN_POINT('Ctrl Pts',(-7.60477614674932E-14,114.462499999553,
12.7882828778556));
#301327=CARTESIAN_POINT('Ctrl Pts',(3.75838203887385,114.612499999552,11.5671105274575));
#301328=CARTESIAN_POINT('Ctrl Pts',(7.51676407774778,114.762499999551,10.3459381770593));
#301329=CARTESIAN_POINT('Ctrl Pts',(9.839571920479,114.912499999551,7.14886745759543));
#301330=CARTESIAN_POINT('Ctrl Pts',(12.1623797632102,115.06249999955,3.95179673813153));
#301331=CARTESIAN_POINT('Ctrl Pts',(12.1623797632102,115.21249999955,-1.489461944703E-15));
#301332=CARTESIAN_POINT('Ctrl Pts',(12.1623797632102,115.362499999549,-3.95179673813154));
#301333=CARTESIAN_POINT('Ctrl Pts',(9.839571920479,115.512499999548,-7.14886745759543));
#301334=CARTESIAN_POINT('Ctrl Pts',(7.51676407774778,115.662499999548,-10.3459381770593));
#301335=CARTESIAN_POINT('Ctrl Pts',(3.75838203887385,115.812499999547,-11.5671105274575));
#301336=CARTESIAN_POINT('Ctrl Pts',(-8.00438420419154E-14,115.962499999547,
-12.7882828778556));
#301337=CARTESIAN_POINT('Ctrl Pts',(-3.75838203887401,116.112499999546,
-11.5671105274575));
#301338=CARTESIAN_POINT('Ctrl Pts',(-7.51676407774794,116.262499999545,
-10.3459381770593));
#301339=CARTESIAN_POINT('Ctrl Pts',(-9.83957192047916,116.412499999545,
-7.14886745759543));
#301340=CARTESIAN_POINT('Ctrl Pts',(-12.1623797632104,116.562499999544,
-3.95179673813153));
#301341=CARTESIAN_POINT('Ctrl Pts',(-12.1623797632104,116.712499999544,
2.97892388940601E-15));
#301342=CARTESIAN_POINT('Ctrl Pts',(-12.1623797632104,116.862499999543,
3.95179673813154));
#301343=CARTESIAN_POINT('Ctrl Pts',(-9.83957192047915,117.012499999542,
7.14886745759543));
#301344=CARTESIAN_POINT('Ctrl Pts',(-7.51676407774793,117.162499999542,
10.3459381770593));
#301345=CARTESIAN_POINT('Ctrl Pts',(-3.75838203887401,117.312499999541,
11.5671105274575));
#301346=CARTESIAN_POINT('Ctrl Pts',(-7.7775470739155E-14,117.462499999541,
12.7882828778556));
#301347=CARTESIAN_POINT('Ctrl Pts',(3.75838203887385,117.61249999954,11.5671105274575));
#301348=CARTESIAN_POINT('Ctrl Pts',(7.51676407774778,117.762499999539,10.3459381770593));
#301349=CARTESIAN_POINT('Ctrl Pts',(9.839571920479,117.912499999539,7.14886745759543));
#301350=CARTESIAN_POINT('Ctrl Pts',(12.1623797632102,118.062499999538,3.95179673813153));
#301351=CARTESIAN_POINT('Ctrl Pts',(12.1623797632102,118.212499999538,-1.489461944703E-15));
#301352=CARTESIAN_POINT('Ctrl Pts',(12.1623797632102,118.362499999537,-3.95179673813154));
#301353=CARTESIAN_POINT('Ctrl Pts',(9.83957192047899,118.512499999536,-7.14886745759543));
#301354=CARTESIAN_POINT('Ctrl Pts',(7.51676407774778,118.662499999536,-10.3459381770593));
#301355=CARTESIAN_POINT('Ctrl Pts',(3.75838203887385,118.812499999535,-11.5671105274575));
#301356=CARTESIAN_POINT('Ctrl Pts',(-8.17715513135773E-14,118.962499999535,
-12.7882828778556));
#301357=CARTESIAN_POINT('Ctrl Pts',(-3.75838203887401,119.112499999534,
-11.5671105274575));
#301358=CARTESIAN_POINT('Ctrl Pts',(-7.51676407774794,119.262499999533,
-10.3459381770593));
#301359=CARTESIAN_POINT('Ctrl Pts',(-9.83957192047916,119.412499999533,
-7.14886745759543));
#301360=CARTESIAN_POINT('Ctrl Pts',(-12.1623797632104,119.562499999532,
-3.95179673813153));
#301361=CARTESIAN_POINT('Ctrl Pts',(-12.1623797632104,119.712499999532,
2.97892388940601E-15));
#301362=CARTESIAN_POINT('Ctrl Pts',(-12.1623797632104,119.862499999531,
3.95179673813154));
#301363=CARTESIAN_POINT('Ctrl Pts',(-9.83957192047916,120.01249999953,7.14886745759543));
#301364=CARTESIAN_POINT('Ctrl Pts',(-7.51676407774794,120.16249999953,10.3459381770593));
#301365=CARTESIAN_POINT('Ctrl Pts',(-3.75838203887401,120.312499999529,
11.5671105274575));
#301366=CARTESIAN_POINT('Ctrl Pts',(-7.95031800108169E-14,120.462499999529,
12.7882828778556));
#301367=CARTESIAN_POINT('Ctrl Pts',(3.75838203887385,120.612499999528,11.5671105274575));
#301368=CARTESIAN_POINT('Ctrl Pts',(7.51676407774778,120.762499999527,10.3459381770593));
#301369=CARTESIAN_POINT('Ctrl Pts',(9.83957192047899,120.912499999527,7.14886745759543));
#301370=CARTESIAN_POINT('Ctrl Pts',(12.1623797632102,121.062499999526,3.95179673813153));
#301371=CARTESIAN_POINT('Ctrl Pts',(12.1623797632102,121.212499999526,-1.489461944703E-15));
#301372=CARTESIAN_POINT('Ctrl Pts',(12.1623797632102,121.362499999525,-3.95179673813154));
#301373=CARTESIAN_POINT('Ctrl Pts',(9.83957192047899,121.512499999524,-7.14886745759543));
#301374=CARTESIAN_POINT('Ctrl Pts',(7.51676407774777,121.662499999524,-10.3459381770593));
#301375=CARTESIAN_POINT('Ctrl Pts',(3.75838203887385,121.812499999523,-11.5671105274575));
#301376=CARTESIAN_POINT('Ctrl Pts',(-8.34992605852391E-14,121.962499999523,
-12.7882828778556));
#301377=CARTESIAN_POINT('Ctrl Pts',(-3.75838203887401,122.112499999522,
-11.5671105274575));
#301378=CARTESIAN_POINT('Ctrl Pts',(-7.51676407774794,122.262499999521,
-10.3459381770593));
#301379=CARTESIAN_POINT('Ctrl Pts',(-9.83957192047916,122.412499999521,
-7.14886745759543));
#301380=CARTESIAN_POINT('Ctrl Pts',(-12.1623797632104,122.56249999952,-3.95179673813153));
#301381=CARTESIAN_POINT('Ctrl Pts',(-12.1623797632104,122.71249999952,2.97892388940601E-15));
#301382=CARTESIAN_POINT('Ctrl Pts',(-12.1623797632104,122.862499999519,
3.95179673813154));
#301383=CARTESIAN_POINT('Ctrl Pts',(-9.83957192047916,123.012499999518,
7.14886745759543));
#301384=CARTESIAN_POINT('Ctrl Pts',(-7.51676407774794,123.162499999518,
10.3459381770593));
#301385=CARTESIAN_POINT('Ctrl Pts',(-3.75838203887401,123.312499999517,
11.5671105274575));
#301386=CARTESIAN_POINT('Ctrl Pts',(-8.12308892824787E-14,123.462499999517,
12.7882828778556));
#301387=CARTESIAN_POINT('Ctrl Pts',(3.75838203887385,123.612499999516,11.5671105274575));
#301388=CARTESIAN_POINT('Ctrl Pts',(7.51676407774778,123.762499999515,10.3459381770593));
#301389=CARTESIAN_POINT('Ctrl Pts',(9.83957192047899,123.912499999515,7.14886745759543));
#301390=CARTESIAN_POINT('Ctrl Pts',(12.1623797632102,124.062499999514,3.95179673813153));
#301391=CARTESIAN_POINT('Ctrl Pts',(12.1623797632102,124.212499999514,-1.489461944703E-15));
#301392=CARTESIAN_POINT('Ctrl Pts',(12.1623797632102,124.362499999513,-3.95179673813154));
#301393=CARTESIAN_POINT('Ctrl Pts',(9.83957192047899,124.512499999512,-7.14886745759543));
#301394=CARTESIAN_POINT('Ctrl Pts',(7.51676407774777,124.662499999512,-10.3459381770593));
#301395=CARTESIAN_POINT('Ctrl Pts',(3.75838203887384,124.812499999511,-11.5671105274575));
#301396=CARTESIAN_POINT('Ctrl Pts',(-8.52269698569009E-14,124.962499999511,
-12.7882828778556));
#301397=CARTESIAN_POINT('Ctrl Pts',(-3.75838203887401,125.11249999951,-11.5671105274575));
#301398=CARTESIAN_POINT('Ctrl Pts',(-7.51676407774794,125.262499999509,
-10.3459381770593));
#301399=CARTESIAN_POINT('Ctrl Pts',(-9.83957192047916,125.412499999509,
-7.14886745759543));
#301400=CARTESIAN_POINT('Ctrl Pts',(-12.1623797632104,125.562499999508,
-3.95179673813153));
#301401=CARTESIAN_POINT('Ctrl Pts',(-12.1623797632104,125.712499999508,
2.97892388940601E-15));
#301402=CARTESIAN_POINT('Ctrl Pts',(-12.1623797632104,125.862499999507,
3.95179673813154));
#301403=CARTESIAN_POINT('Ctrl Pts',(-9.83957192047916,126.012499999506,
7.14886745759543));
#301404=CARTESIAN_POINT('Ctrl Pts',(-7.51676407774794,126.162499999506,
10.3459381770593));
#301405=CARTESIAN_POINT('Ctrl Pts',(-3.75838203887401,126.312499999505,
11.5671105274575));
#301406=CARTESIAN_POINT('Ctrl Pts',(-8.29585985541405E-14,126.462499999505,
12.7882828778556));
#301407=CARTESIAN_POINT('Ctrl Pts',(3.75838203887385,126.612499999504,11.5671105274575));
#301408=CARTESIAN_POINT('Ctrl Pts',(7.51676407774777,126.762499999503,10.3459381770593));
#301409=CARTESIAN_POINT('Ctrl Pts',(9.83957192047899,126.912499999503,7.14886745759543));
#301410=CARTESIAN_POINT('Ctrl Pts',(12.1623797632102,127.062499999502,3.95179673813153));
#301411=CARTESIAN_POINT('Ctrl Pts',(12.1623797632102,127.212499999502,-1.489461944703E-15));
#301412=CARTESIAN_POINT('Ctrl Pts',(12.1623797632102,127.362499999501,-3.95179673813154));
#301413=CARTESIAN_POINT('Ctrl Pts',(9.83957192047899,127.5124999995,-7.14886745759543));
#301414=CARTESIAN_POINT('Ctrl Pts',(7.51676407774777,127.6624999995,-10.3459381770593));
#301415=CARTESIAN_POINT('Ctrl Pts',(3.75838203887384,127.812499999499,-11.5671105274575));
#301416=CARTESIAN_POINT('Ctrl Pts',(-8.69546791285628E-14,127.962499999499,
-12.7882828778556));
#301417=CARTESIAN_POINT('Ctrl Pts',(-3.75838203887402,128.112499999498,
-11.5671105274575));
#301418=CARTESIAN_POINT('Ctrl Pts',(-7.51676407774795,128.262499999497,
-10.3459381770593));
#301419=CARTESIAN_POINT('Ctrl Pts',(-9.83957192047916,128.412499999497,
-7.14886745759543));
#301420=CARTESIAN_POINT('Ctrl Pts',(-12.1623797632104,128.562499999496,
-3.95179673813153));
#301421=CARTESIAN_POINT('Ctrl Pts',(-12.1623797632104,128.712499999496,
2.97892388940601E-15));
#301422=CARTESIAN_POINT('Ctrl Pts',(-12.1623797632104,128.862499999495,
3.95179673813154));
#301423=CARTESIAN_POINT('Ctrl Pts',(-9.83957192047916,129.012499999494,
7.14886745759543));
#301424=CARTESIAN_POINT('Ctrl Pts',(-7.51676407774794,129.162499999494,
10.3459381770593));
#301425=CARTESIAN_POINT('Ctrl Pts',(-3.75838203887401,129.312499999493,
11.5671105274575));
#301426=CARTESIAN_POINT('Ctrl Pts',(-8.46863078258024E-14,129.462499999493,
12.7882828778556));
#301427=CARTESIAN_POINT('Ctrl Pts',(3.75838203887384,129.612499999492,11.5671105274575));
#301428=CARTESIAN_POINT('Ctrl Pts',(7.51676407774777,129.762499999491,10.3459381770593));
#301429=CARTESIAN_POINT('Ctrl Pts',(9.83957192047899,129.912499999491,7.14886745759543));
#301430=CARTESIAN_POINT('Ctrl Pts',(12.1623797632102,130.06249999949,3.95179673813153));
#301431=CARTESIAN_POINT('Ctrl Pts',(12.1623797632102,130.21249999949,-1.489461944703E-15));
#301432=CARTESIAN_POINT('Ctrl Pts',(12.1623797632102,130.362499999489,-3.95179673813154));
#301433=CARTESIAN_POINT('Ctrl Pts',(9.83957192047899,130.512499999488,-7.14886745759543));
#301434=CARTESIAN_POINT('Ctrl Pts',(7.51676407774777,130.662499999488,-10.3459381770593));
#301435=CARTESIAN_POINT('Ctrl Pts',(3.75838203887384,130.812499999487,-11.5671105274575));
#301436=CARTESIAN_POINT('Ctrl Pts',(-8.86823884002247E-14,130.962499999487,
-12.7882828778556));
#301437=CARTESIAN_POINT('Ctrl Pts',(-3.75838203887402,131.112499999486,
-11.5671105274575));
#301438=CARTESIAN_POINT('Ctrl Pts',(-7.51676407774795,131.262499999485,
-10.3459381770593));
#301439=CARTESIAN_POINT('Ctrl Pts',(-9.83957192047916,131.412499999485,
-7.14886745759543));
#301440=CARTESIAN_POINT('Ctrl Pts',(-12.1623797632104,131.562499999484,
-3.95179673813153));
#301441=CARTESIAN_POINT('Ctrl Pts',(-12.1623797632104,131.712499999484,
2.97892388940601E-15));
#301442=CARTESIAN_POINT('Ctrl Pts',(-12.1623797632104,131.862499999483,
3.95179673813154));
#301443=CARTESIAN_POINT('Ctrl Pts',(-9.83957192047916,132.012499999482,
7.14886745759543));
#301444=CARTESIAN_POINT('Ctrl Pts',(-7.51676407774795,132.162499999482,
10.3459381770593));
#301445=CARTESIAN_POINT('Ctrl Pts',(-3.75838203887402,132.312499999481,
11.5671105274575));
#301446=CARTESIAN_POINT('Ctrl Pts',(-8.64140170974642E-14,132.462499999481,
12.7882828778556));
#301447=CARTESIAN_POINT('Ctrl Pts',(3.75838203887384,132.61249999948,11.5671105274575));
#301448=CARTESIAN_POINT('Ctrl Pts',(7.51676407774777,132.762499999479,10.3459381770593));
#301449=CARTESIAN_POINT('Ctrl Pts',(9.83957192047899,132.912499999479,7.14886745759543));
#301450=CARTESIAN_POINT('Ctrl Pts',(12.1623797632102,133.062499999478,3.95179673813153));
#301451=CARTESIAN_POINT('Ctrl Pts',(12.1623797632102,133.212499999478,-1.489461944703E-15));
#301452=CARTESIAN_POINT('Ctrl Pts',(12.1623797632102,133.362499999477,-3.95179673813154));
#301453=CARTESIAN_POINT('Ctrl Pts',(9.83957192047898,133.512499999476,-7.14886745759543));
#301454=CARTESIAN_POINT('Ctrl Pts',(7.51676407774777,133.662499999476,-10.3459381770593));
#301455=CARTESIAN_POINT('Ctrl Pts',(3.75838203887384,133.812499999475,-11.5671105274575));
#301456=CARTESIAN_POINT('Ctrl Pts',(-9.04100976718865E-14,133.962499999475,
-12.7882828778556));
#301457=CARTESIAN_POINT('Ctrl Pts',(-3.75838203887402,134.112499999474,
-11.5671105274575));
#301458=CARTESIAN_POINT('Ctrl Pts',(-7.51676407774795,134.262499999473,
-10.3459381770593));
#301459=CARTESIAN_POINT('Ctrl Pts',(-9.83957192047917,134.412499999473,
-7.14886745759543));
#301460=CARTESIAN_POINT('Ctrl Pts',(-12.1623797632104,134.562499999472,
-3.95179673813153));
#301461=CARTESIAN_POINT('Ctrl Pts',(-12.1623797632104,134.712499999472,
2.97892388940601E-15));
#301462=CARTESIAN_POINT('Ctrl Pts',(-12.1623797632104,134.862499999471,
3.95179673813154));
#301463=CARTESIAN_POINT('Ctrl Pts',(-9.83957192047916,135.01249999947,7.14886745759543));
#301464=CARTESIAN_POINT('Ctrl Pts',(-7.51676407774795,135.16249999947,10.3459381770593));
#301465=CARTESIAN_POINT('Ctrl Pts',(-3.75838203887402,135.312499999469,
11.5671105274575));
#301466=CARTESIAN_POINT('Ctrl Pts',(-8.8141726369126E-14,135.462499999469,
12.7882828778556));
#301467=CARTESIAN_POINT('Ctrl Pts',(3.75838203887384,135.612499999468,11.5671105274575));
#301468=CARTESIAN_POINT('Ctrl Pts',(7.51676407774777,135.762499999467,10.3459381770593));
#301469=CARTESIAN_POINT('Ctrl Pts',(9.83957192047898,135.912499999467,7.14886745759543));
#301470=CARTESIAN_POINT('Ctrl Pts',(12.1623797632102,136.062499999466,3.95179673813153));
#301471=CARTESIAN_POINT('Ctrl Pts',(12.1623797632102,136.212499999466,-1.489461944703E-15));
#301472=CARTESIAN_POINT('Ctrl Pts',(12.1623797632102,136.362499999465,-3.95179673813154));
#301473=CARTESIAN_POINT('Ctrl Pts',(9.83957192047898,136.512499999464,-7.14886745759543));
#301474=CARTESIAN_POINT('Ctrl Pts',(7.51676407774777,136.662499999464,-10.3459381770593));
#301475=CARTESIAN_POINT('Ctrl Pts',(3.75838203887384,136.812499999463,-11.5671105274575));
#301476=CARTESIAN_POINT('Ctrl Pts',(-9.21378069435483E-14,136.962499999463,
-12.7882828778556));
#301477=CARTESIAN_POINT('Ctrl Pts',(-3.75838203887402,137.112499999462,
-11.5671105274575));
#301478=CARTESIAN_POINT('Ctrl Pts',(-7.51676407774795,137.262499999461,
-10.3459381770593));
#301479=CARTESIAN_POINT('Ctrl Pts',(-9.83957192047917,137.412499999461,
-7.14886745759543));
#301480=CARTESIAN_POINT('Ctrl Pts',(-12.1623797632104,137.56249999946,-3.95179673813153));
#301481=CARTESIAN_POINT('Ctrl Pts',(-12.1623797632104,137.71249999946,2.97892388940601E-15));
#301482=CARTESIAN_POINT('Ctrl Pts',(-12.1623797632104,137.862499999459,
3.95179673813154));
#301483=CARTESIAN_POINT('Ctrl Pts',(-9.83957192047917,138.012499999458,
7.14886745759543));
#301484=CARTESIAN_POINT('Ctrl Pts',(-7.51676407774795,138.162499999458,
10.3459381770593));
#301485=CARTESIAN_POINT('Ctrl Pts',(-3.75838203887402,138.312499999457,
11.5671105274575));
#301486=CARTESIAN_POINT('Ctrl Pts',(-8.98694356407879E-14,138.462499999457,
12.7882828778556));
#301487=CARTESIAN_POINT('Ctrl Pts',(3.75838203887384,138.612499999456,11.5671105274575));
#301488=CARTESIAN_POINT('Ctrl Pts',(7.51676407774777,138.762499999455,10.3459381770593));
#301489=CARTESIAN_POINT('Ctrl Pts',(9.83957192047898,138.912499999455,7.14886745759543));
#301490=CARTESIAN_POINT('Ctrl Pts',(12.1623797632102,139.062499999454,3.95179673813153));
#301491=CARTESIAN_POINT('Ctrl Pts',(12.1623797632102,139.212499999454,-1.489461944703E-15));
#301492=CARTESIAN_POINT('Ctrl Pts',(12.1623797632102,139.362499999453,-3.95179673813154));
#301493=CARTESIAN_POINT('Ctrl Pts',(9.83957192047898,139.512499999452,-7.14886745759543));
#301494=CARTESIAN_POINT('Ctrl Pts',(7.51676407774776,139.662499999452,-10.3459381770593));
#301495=CARTESIAN_POINT('Ctrl Pts',(3.75838203887384,139.812499999451,-11.5671105274575));
#301496=CARTESIAN_POINT('Ctrl Pts',(-9.38655162152102E-14,139.962499999451,
-12.7882828778556));
#301497=CARTESIAN_POINT('Ctrl Pts',(-3.75838203887402,140.11249999945,-11.5671105274575));
#301498=CARTESIAN_POINT('Ctrl Pts',(-7.51676407774795,140.262499999449,
-10.3459381770593));
#301499=CARTESIAN_POINT('Ctrl Pts',(-9.83957192047917,140.412499999449,
-7.14886745759543));
#301500=CARTESIAN_POINT('Ctrl Pts',(-12.1623797632104,140.562499999448,
-3.95179673813153));
#301501=CARTESIAN_POINT('Ctrl Pts',(-12.1623797632104,140.712499999448,
2.97892388940601E-15));
#301502=CARTESIAN_POINT('Ctrl Pts',(-12.1623797632104,140.862499999447,
3.95179673813154));
#301503=CARTESIAN_POINT('Ctrl Pts',(-9.83957192047917,141.012499999446,
7.14886745759543));
#301504=CARTESIAN_POINT('Ctrl Pts',(-7.51676407774795,141.162499999446,
10.3459381770593));
#301505=CARTESIAN_POINT('Ctrl Pts',(-3.75838203887402,141.312499999445,
11.5671105274575));
#301506=CARTESIAN_POINT('Ctrl Pts',(-9.15971449124498E-14,141.462499999445,
12.7882828778556));
#301507=CARTESIAN_POINT('Ctrl Pts',(3.75838203887384,141.612499999444,11.5671105274575));
#301508=CARTESIAN_POINT('Ctrl Pts',(7.51676407774777,141.762499999443,10.3459381770593));
#301509=CARTESIAN_POINT('Ctrl Pts',(9.83957192047898,141.912499999443,7.14886745759543));
#301510=CARTESIAN_POINT('Ctrl Pts',(12.1623797632102,142.062499999442,3.95179673813153));
#301511=CARTESIAN_POINT('Ctrl Pts',(12.1623797632102,142.212499999442,-1.489461944703E-15));
#301512=CARTESIAN_POINT('Ctrl Pts',(12.1623797632102,142.362499999441,-3.95179673813154));
#301513=CARTESIAN_POINT('Ctrl Pts',(9.83957192047898,142.51249999944,-7.14886745759543));
#301514=CARTESIAN_POINT('Ctrl Pts',(7.51676407774776,142.66249999944,-10.3459381770593));
#301515=CARTESIAN_POINT('Ctrl Pts',(3.75838203887383,142.812499999439,-11.5671105274575));
#301516=CARTESIAN_POINT('Ctrl Pts',(-9.5593225486872E-14,142.962499999439,
-12.7882828778556));
#301517=CARTESIAN_POINT('Ctrl Pts',(-3.75838203887402,143.112499999438,
-11.5671105274575));
#301518=CARTESIAN_POINT('Ctrl Pts',(-7.51676407774795,143.262499999437,
-10.3459381770593));
#301519=CARTESIAN_POINT('Ctrl Pts',(-9.83957192047917,143.412499999437,
-7.14886745759543));
#301520=CARTESIAN_POINT('Ctrl Pts',(-12.1623797632104,143.562499999436,
-3.95179673813153));
#301521=CARTESIAN_POINT('Ctrl Pts',(-12.1623797632104,143.712499999436,
2.97892388940601E-15));
#301522=CARTESIAN_POINT('Ctrl Pts',(-12.1623797632104,143.862499999435,
3.95179673813154));
#301523=CARTESIAN_POINT('Ctrl Pts',(-9.83957192047917,144.012499999434,
7.14886745759543));
#301524=CARTESIAN_POINT('Ctrl Pts',(-7.51676407774795,144.162499999434,
10.3459381770593));
#301525=CARTESIAN_POINT('Ctrl Pts',(-3.75838203887402,144.312499999433,
11.5671105274575));
#301526=CARTESIAN_POINT('Ctrl Pts',(-9.33248541841116E-14,144.462499999433,
12.7882828778556));
#301527=CARTESIAN_POINT('Ctrl Pts',(3.75838203887384,144.612499999432,11.5671105274575));
#301528=CARTESIAN_POINT('Ctrl Pts',(7.51676407774776,144.762499999431,10.3459381770593));
#301529=CARTESIAN_POINT('Ctrl Pts',(9.83957192047898,144.912499999431,7.14886745759543));
#301530=CARTESIAN_POINT('Ctrl Pts',(12.1623797632102,145.06249999943,3.95179673813153));
#301531=CARTESIAN_POINT('Ctrl Pts',(12.1623797632102,145.21249999943,-1.489461944703E-15));
#301532=CARTESIAN_POINT('Ctrl Pts',(12.1623797632102,145.362499999429,-3.95179673813154));
#301533=CARTESIAN_POINT('Ctrl Pts',(9.83957192047898,145.512499999428,-7.14886745759543));
#301534=CARTESIAN_POINT('Ctrl Pts',(7.51676407774776,145.662499999428,-10.3459381770593));
#301535=CARTESIAN_POINT('Ctrl Pts',(3.75838203887383,145.812499999427,-11.5671105274575));
#301536=CARTESIAN_POINT('Ctrl Pts',(-9.73209347585338E-14,145.962499999427,
-12.7882828778556));
#301537=CARTESIAN_POINT('Ctrl Pts',(-3.75838203887403,146.112499999426,
-11.5671105274575));
#301538=CARTESIAN_POINT('Ctrl Pts',(-7.51676407774795,146.262499999425,
-10.3459381770593));
#301539=CARTESIAN_POINT('Ctrl Pts',(-9.83957192047917,146.412499999425,
-7.14886745759543));
#301540=CARTESIAN_POINT('Ctrl Pts',(-12.1623797632104,146.562499999424,
-3.95179673813153));
#301541=CARTESIAN_POINT('Ctrl Pts',(-12.1623797632104,146.712499999424,
2.97892388940601E-15));
#301542=CARTESIAN_POINT('Ctrl Pts',(-12.1623797632104,146.862499999423,
3.95179673813154));
#301543=CARTESIAN_POINT('Ctrl Pts',(-9.83957192047917,147.012499999422,
7.14886745759543));
#301544=CARTESIAN_POINT('Ctrl Pts',(-7.51676407774795,147.162499999422,
10.3459381770593));
#301545=CARTESIAN_POINT('Ctrl Pts',(-3.75838203887402,147.312499999421,
11.5671105274575));
#301546=CARTESIAN_POINT('Ctrl Pts',(-9.50525634557734E-14,147.462499999421,
12.7882828778556));
#301547=CARTESIAN_POINT('Ctrl Pts',(3.75838203887383,147.61249999942,11.5671105274575));
#301548=CARTESIAN_POINT('Ctrl Pts',(7.51676407774776,147.762499999419,10.3459381770593));
#301549=CARTESIAN_POINT('Ctrl Pts',(9.83957192047898,147.912499999419,7.14886745759543));
#301550=CARTESIAN_POINT('Ctrl Pts',(12.1623797632102,148.062499999418,3.95179673813153));
#301551=CARTESIAN_POINT('Ctrl Pts',(12.1623797632102,148.212499999418,-1.489461944703E-15));
#301552=CARTESIAN_POINT('Ctrl Pts',(12.1623797632102,148.362499999417,-3.95179673813154));
#301553=CARTESIAN_POINT('Ctrl Pts',(9.83957192047898,148.512499999416,-7.14886745759543));
#301554=CARTESIAN_POINT('Ctrl Pts',(7.51676407774776,148.662499999416,-10.3459381770593));
#301555=CARTESIAN_POINT('Ctrl Pts',(3.75838203887383,148.812499999415,-11.5671105274575));
#301556=CARTESIAN_POINT('Ctrl Pts',(-9.90486440301957E-14,148.962499999415,
-12.7882828778556));
#301557=CARTESIAN_POINT('Ctrl Pts',(-3.75838203887403,149.112499999414,
-11.5671105274575));
#301558=CARTESIAN_POINT('Ctrl Pts',(-7.51676407774795,149.262499999413,
-10.3459381770593));
#301559=CARTESIAN_POINT('Ctrl Pts',(-9.83957192047917,149.412499999413,
-7.14886745759543));
#301560=CARTESIAN_POINT('Ctrl Pts',(-12.1623797632104,149.562499999412,
-3.95179673813153));
#301561=CARTESIAN_POINT('Ctrl Pts',(-12.1623797632104,149.712499999412,
2.97892388940601E-15));
#301562=CARTESIAN_POINT('Ctrl Pts',(-12.1623797632104,149.862499999411,
3.95179673813154));
#301563=CARTESIAN_POINT('Ctrl Pts',(-9.83957192047917,150.01249999941,7.14886745759543));
#301564=CARTESIAN_POINT('Ctrl Pts',(-7.51676407774795,150.16249999941,10.3459381770593));
#301565=CARTESIAN_POINT('Ctrl Pts',(-3.75838203887403,150.312499999409,
11.5671105274575));
#301566=CARTESIAN_POINT('Ctrl Pts',(-9.67802727274353E-14,150.462499999409,
12.7882828778556));
#301567=CARTESIAN_POINT('Ctrl Pts',(3.75838203887383,150.612499999408,11.5671105274575));
#301568=CARTESIAN_POINT('Ctrl Pts',(7.51676407774776,150.762499999407,10.3459381770593));
#301569=CARTESIAN_POINT('Ctrl Pts',(9.83957192047898,150.912499999407,7.14886745759543));
#301570=CARTESIAN_POINT('Ctrl Pts',(12.1623797632102,151.062499999406,3.95179673813153));
#301571=CARTESIAN_POINT('Ctrl Pts',(12.1623797632102,151.212499999406,-1.489461944703E-15));
#301572=CARTESIAN_POINT('Ctrl Pts',(12.1623797632102,151.362499999405,-3.95179673813154));
#301573=CARTESIAN_POINT('Ctrl Pts',(9.83957192047897,151.512499999404,-7.14886745759543));
#301574=CARTESIAN_POINT('Ctrl Pts',(7.51676407774776,151.662499999404,-10.3459381770593));
#301575=CARTESIAN_POINT('Ctrl Pts',(3.75838203887383,151.812499999403,-11.5671105274575));
#301576=CARTESIAN_POINT('Ctrl Pts',(-1.00776353301858E-13,151.962499999403,
-12.7882828778556));
#301577=CARTESIAN_POINT('Ctrl Pts',(-3.75838203887403,152.112499999402,
-11.5671105274575));
#301578=CARTESIAN_POINT('Ctrl Pts',(-10.0514428414942,-2.06874999998125,
2.46189346052968E-15));
#301579=CARTESIAN_POINT('Ctrl Pts',(-10.0514428414942,-1.91874999998185,
3.26591175476071));
#301580=CARTESIAN_POINT('Ctrl Pts',(-8.1317880767572,-1.76874999998245,
5.90808986649102));
#301581=CARTESIAN_POINT('Ctrl Pts',(-6.21213331202023,-1.61874999998305,
8.55026797822134));
#301582=CARTESIAN_POINT('Ctrl Pts',(-3.10606665601012,-1.46874999998365,
9.5594902125713));
#301583=CARTESIAN_POINT('Ctrl Pts',(-9.77671023785295E-15,-1.31874999998425,
10.5687124469213));
#301584=CARTESIAN_POINT('Ctrl Pts',(3.1060666560101,-1.16874999998485,9.5594902125713));
#301585=CARTESIAN_POINT('Ctrl Pts',(6.21213331202021,-1.01874999998544,
8.55026797822134));
#301586=CARTESIAN_POINT('Ctrl Pts',(8.13178807675718,-0.868749999986043,
5.90808986649102));
#301587=CARTESIAN_POINT('Ctrl Pts',(10.0514428414942,-0.718749999986641,
3.2659117547607));
#301588=CARTESIAN_POINT('Ctrl Pts',(10.0514428414942,-0.568749999987242,
-1.23094673026484E-15));
#301589=CARTESIAN_POINT('Ctrl Pts',(10.0514428414942,-0.418749999987842,
-3.26591175476071));
#301590=CARTESIAN_POINT('Ctrl Pts',(8.13178807675718,-0.268749999988443,
-5.90808986649102));
#301591=CARTESIAN_POINT('Ctrl Pts',(6.2121333120202,-0.118749999989044,
-8.55026797822134));
#301592=CARTESIAN_POINT('Ctrl Pts',(3.10606665601009,0.0312500000103543,
-9.5594902125713));
#301593=CARTESIAN_POINT('Ctrl Pts',(-1.322915284753E-14,0.181250000009752,
-10.5687124469213));
#301594=CARTESIAN_POINT('Ctrl Pts',(-3.10606665601012,0.331250000009151,
-9.5594902125713));
#301595=CARTESIAN_POINT('Ctrl Pts',(-6.21213331202023,0.481250000008549,
-8.55026797822134));
#301596=CARTESIAN_POINT('Ctrl Pts',(-8.1317880767572,0.631250000007948,
-5.90808986649102));
#301597=CARTESIAN_POINT('Ctrl Pts',(-10.0514428414942,0.781250000007346,
-3.2659117547607));
#301598=CARTESIAN_POINT('Ctrl Pts',(-10.0514428414942,0.931250000006746,
2.46189346052968E-15));
#301599=CARTESIAN_POINT('Ctrl Pts',(-10.0514428414942,1.08125000000615,
3.26591175476071));
#301600=CARTESIAN_POINT('Ctrl Pts',(-8.1317880767572,1.23125000000555,5.90808986649102));
#301601=CARTESIAN_POINT('Ctrl Pts',(-6.21213331202023,1.38125000000495,
8.55026797822134));
#301602=CARTESIAN_POINT('Ctrl Pts',(-3.10606665601012,1.53125000000435,
9.5594902125713));
#301603=CARTESIAN_POINT('Ctrl Pts',(-1.15044195095148E-14,1.68125000000375,
10.5687124469213));
#301604=CARTESIAN_POINT('Ctrl Pts',(3.1060666560101,1.83125000000315,9.5594902125713));
#301605=CARTESIAN_POINT('Ctrl Pts',(6.2121333120202,1.98125000000256,8.55026797822134));
#301606=CARTESIAN_POINT('Ctrl Pts',(8.13178807675718,2.13125000000196,5.90808986649102));
#301607=CARTESIAN_POINT('Ctrl Pts',(10.0514428414942,2.28125000000136,3.2659117547607));
#301608=CARTESIAN_POINT('Ctrl Pts',(10.0514428414942,2.43125000000076,-1.23094673026484E-15));
#301609=CARTESIAN_POINT('Ctrl Pts',(10.0514428414942,2.58125000000016,-3.26591175476071));
#301610=CARTESIAN_POINT('Ctrl Pts',(8.13178807675718,2.73124999999956,-5.90808986649102));
#301611=CARTESIAN_POINT('Ctrl Pts',(6.2121333120202,2.88124999999896,-8.55026797822134));
#301612=CARTESIAN_POINT('Ctrl Pts',(3.10606665601009,3.03124999999835,-9.5594902125713));
#301613=CARTESIAN_POINT('Ctrl Pts',(-1.49568621191919E-14,3.18124999999775,
-10.5687124469213));
#301614=CARTESIAN_POINT('Ctrl Pts',(-3.10606665601012,3.33124999999715,
-9.5594902125713));
#301615=CARTESIAN_POINT('Ctrl Pts',(-6.21213331202023,3.48124999999655,
-8.55026797822134));
#301616=CARTESIAN_POINT('Ctrl Pts',(-8.13178807675721,3.63124999999595,
-5.90808986649102));
#301617=CARTESIAN_POINT('Ctrl Pts',(-10.0514428414942,3.78124999999535,
-3.2659117547607));
#301618=CARTESIAN_POINT('Ctrl Pts',(-10.0514428414942,3.93124999999475,
2.46189346052968E-15));
#301619=CARTESIAN_POINT('Ctrl Pts',(-10.0514428414942,4.08124999999415,
3.26591175476071));
#301620=CARTESIAN_POINT('Ctrl Pts',(-8.13178807675721,4.23124999999355,
5.90808986649102));
#301621=CARTESIAN_POINT('Ctrl Pts',(-6.21213331202023,4.38124999999295,
8.55026797822134));
#301622=CARTESIAN_POINT('Ctrl Pts',(-3.10606665601012,4.53124999999235,
9.5594902125713));
#301623=CARTESIAN_POINT('Ctrl Pts',(-1.32321287811766E-14,4.68124999999175,
10.5687124469213));
#301624=CARTESIAN_POINT('Ctrl Pts',(3.10606665601009,4.83124999999115,9.5594902125713));
#301625=CARTESIAN_POINT('Ctrl Pts',(6.2121333120202,4.98124999999055,8.55026797822134));
#301626=CARTESIAN_POINT('Ctrl Pts',(8.13178807675718,5.13124999998996,5.90808986649102));
#301627=CARTESIAN_POINT('Ctrl Pts',(10.0514428414942,5.28124999998936,3.2659117547607));
#301628=CARTESIAN_POINT('Ctrl Pts',(10.0514428414941,5.43124999998876,-1.23094673026484E-15));
#301629=CARTESIAN_POINT('Ctrl Pts',(10.0514428414941,5.58124999998816,-3.26591175476071));
#301630=CARTESIAN_POINT('Ctrl Pts',(8.13178807675717,5.73124999998756,-5.90808986649102));
#301631=CARTESIAN_POINT('Ctrl Pts',(6.2121333120202,5.88124999998695,-8.55026797822134));
#301632=CARTESIAN_POINT('Ctrl Pts',(3.10606665601009,6.03124999998635,-9.5594902125713));
#301633=CARTESIAN_POINT('Ctrl Pts',(-1.66845713908537E-14,6.18124999998575,
-10.5687124469213));
#301634=CARTESIAN_POINT('Ctrl Pts',(-3.10606665601012,6.33124999998515,
-9.5594902125713));
#301635=CARTESIAN_POINT('Ctrl Pts',(-6.21213331202023,6.48124999998455,
-8.55026797822134));
#301636=CARTESIAN_POINT('Ctrl Pts',(-8.13178807675721,6.63124999998395,
-5.90808986649102));
#301637=CARTESIAN_POINT('Ctrl Pts',(-10.0514428414942,6.78124999998335,
-3.2659117547607));
#301638=CARTESIAN_POINT('Ctrl Pts',(-10.0514428414942,6.93124999998275,
2.46189346052968E-15));
#301639=CARTESIAN_POINT('Ctrl Pts',(-10.0514428414942,7.08124999998215,
3.26591175476071));
#301640=CARTESIAN_POINT('Ctrl Pts',(-8.13178807675721,7.23124999998155,
5.90808986649102));
#301641=CARTESIAN_POINT('Ctrl Pts',(-6.21213331202023,7.38124999998095,
8.55026797822134));
#301642=CARTESIAN_POINT('Ctrl Pts',(-3.10606665601012,7.53124999998035,
9.5594902125713));
#301643=CARTESIAN_POINT('Ctrl Pts',(-1.49598380528385E-14,7.68124999997975,
10.5687124469213));
#301644=CARTESIAN_POINT('Ctrl Pts',(3.10606665601009,7.83124999997915,9.5594902125713));
#301645=CARTESIAN_POINT('Ctrl Pts',(6.2121333120202,7.98124999997856,8.55026797822134));
#301646=CARTESIAN_POINT('Ctrl Pts',(8.13178807675717,8.13124999997796,5.90808986649102));
#301647=CARTESIAN_POINT('Ctrl Pts',(10.0514428414942,8.28124999997736,3.2659117547607));
#301648=CARTESIAN_POINT('Ctrl Pts',(10.0514428414941,8.43124999997676,-1.23094673026484E-15));
#301649=CARTESIAN_POINT('Ctrl Pts',(10.0514428414941,8.58124999997616,-3.26591175476071));
#301650=CARTESIAN_POINT('Ctrl Pts',(8.13178807675717,8.73124999997556,-5.90808986649102));
#301651=CARTESIAN_POINT('Ctrl Pts',(6.2121333120202,8.88124999997496,-8.55026797822134));
#301652=CARTESIAN_POINT('Ctrl Pts',(3.10606665601009,9.03124999997436,-9.5594902125713));
#301653=CARTESIAN_POINT('Ctrl Pts',(-1.84122806625156E-14,9.18124999997375,
-10.5687124469213));
#301654=CARTESIAN_POINT('Ctrl Pts',(-3.10606665601013,9.33124999997315,
-9.5594902125713));
#301655=CARTESIAN_POINT('Ctrl Pts',(-6.21213331202023,9.48124999997255,
-8.55026797822134));
#301656=CARTESIAN_POINT('Ctrl Pts',(-8.13178807675721,9.63124999997195,
-5.90808986649102));
#301657=CARTESIAN_POINT('Ctrl Pts',(-10.0514428414942,9.78124999997135,
-3.2659117547607));
#301658=CARTESIAN_POINT('Ctrl Pts',(-10.0514428414942,9.93124999997075,
2.46189346052968E-15));
#301659=CARTESIAN_POINT('Ctrl Pts',(-10.0514428414942,10.0812499999701,
3.26591175476071));
#301660=CARTESIAN_POINT('Ctrl Pts',(-8.13178807675721,10.2312499999695,
5.90808986649102));
#301661=CARTESIAN_POINT('Ctrl Pts',(-6.21213331202023,10.3812499999689,
8.55026797822134));
#301662=CARTESIAN_POINT('Ctrl Pts',(-3.10606665601012,10.5312499999684,
9.5594902125713));
#301663=CARTESIAN_POINT('Ctrl Pts',(-1.66875473245003E-14,10.6812499999678,
10.5687124469213));
#301664=CARTESIAN_POINT('Ctrl Pts',(3.10606665601009,10.8312499999672,9.5594902125713));
#301665=CARTESIAN_POINT('Ctrl Pts',(6.2121333120202,10.9812499999666,8.55026797822134));
#301666=CARTESIAN_POINT('Ctrl Pts',(8.13178807675717,11.131249999966,5.90808986649102));
#301667=CARTESIAN_POINT('Ctrl Pts',(10.0514428414941,11.2812499999654,3.2659117547607));
#301668=CARTESIAN_POINT('Ctrl Pts',(10.0514428414941,11.4312499999648,-1.23094673026484E-15));
#301669=CARTESIAN_POINT('Ctrl Pts',(10.0514428414941,11.5812499999642,-3.26591175476071));
#301670=CARTESIAN_POINT('Ctrl Pts',(8.13178807675717,11.7312499999636,-5.90808986649102));
#301671=CARTESIAN_POINT('Ctrl Pts',(6.2121333120202,11.881249999963,-8.55026797822134));
#301672=CARTESIAN_POINT('Ctrl Pts',(3.10606665601009,12.0312499999624,-9.5594902125713));
#301673=CARTESIAN_POINT('Ctrl Pts',(-2.01399899341774E-14,12.1812499999618,
-10.5687124469213));
#301674=CARTESIAN_POINT('Ctrl Pts',(-3.10606665601013,12.3312499999612,
-9.5594902125713));
#301675=CARTESIAN_POINT('Ctrl Pts',(-6.21213331202024,12.4812499999605,
-8.55026797822134));
#301676=CARTESIAN_POINT('Ctrl Pts',(-8.13178807675721,12.6312499999599,
-5.90808986649102));
#301677=CARTESIAN_POINT('Ctrl Pts',(-10.0514428414942,12.7812499999593,
-3.2659117547607));
#301678=CARTESIAN_POINT('Ctrl Pts',(-10.0514428414942,12.9312499999587,
2.46189346052968E-15));
#301679=CARTESIAN_POINT('Ctrl Pts',(-10.0514428414942,13.0812499999581,
3.26591175476071));
#301680=CARTESIAN_POINT('Ctrl Pts',(-8.13178807675721,13.2312499999575,
5.90808986649102));
#301681=CARTESIAN_POINT('Ctrl Pts',(-6.21213331202023,13.3812499999569,
8.55026797822134));
#301682=CARTESIAN_POINT('Ctrl Pts',(-3.10606665601013,13.5312499999564,
9.5594902125713));
#301683=CARTESIAN_POINT('Ctrl Pts',(-1.84152565961621E-14,13.6812499999558,
10.5687124469213));
#301684=CARTESIAN_POINT('Ctrl Pts',(3.10606665601009,13.8312499999552,9.5594902125713));
#301685=CARTESIAN_POINT('Ctrl Pts',(6.2121333120202,13.9812499999546,8.55026797822134));
#301686=CARTESIAN_POINT('Ctrl Pts',(8.13178807675717,14.131249999954,5.90808986649102));
#301687=CARTESIAN_POINT('Ctrl Pts',(10.0514428414941,14.2812499999534,3.2659117547607));
#301688=CARTESIAN_POINT('Ctrl Pts',(10.0514428414941,14.4312499999528,-1.23094673026484E-15));
#301689=CARTESIAN_POINT('Ctrl Pts',(10.0514428414941,14.5812499999522,-3.26591175476071));
#301690=CARTESIAN_POINT('Ctrl Pts',(8.13178807675717,14.7312499999516,-5.90808986649102));
#301691=CARTESIAN_POINT('Ctrl Pts',(6.21213331202019,14.881249999951,-8.55026797822134));
#301692=CARTESIAN_POINT('Ctrl Pts',(3.10606665601009,15.0312499999504,-9.5594902125713));
#301693=CARTESIAN_POINT('Ctrl Pts',(-2.18676992058392E-14,15.1812499999498,
-10.5687124469213));
#301694=CARTESIAN_POINT('Ctrl Pts',(-3.10606665601013,15.3312499999492,
-9.5594902125713));
#301695=CARTESIAN_POINT('Ctrl Pts',(-6.21213331202024,15.4812499999485,
-8.55026797822134));
#301696=CARTESIAN_POINT('Ctrl Pts',(-8.13178807675721,15.6312499999479,
-5.90808986649102));
#301697=CARTESIAN_POINT('Ctrl Pts',(-10.0514428414942,15.7812499999473,
-3.2659117547607));
#301698=CARTESIAN_POINT('Ctrl Pts',(-10.0514428414942,15.9312499999467,
2.46189346052968E-15));
#301699=CARTESIAN_POINT('Ctrl Pts',(-10.0514428414942,16.0812499999461,
3.26591175476071));
#301700=CARTESIAN_POINT('Ctrl Pts',(-8.13178807675721,16.2312499999455,
5.90808986649102));
#301701=CARTESIAN_POINT('Ctrl Pts',(-6.21213331202024,16.3812499999449,
8.55026797822134));
#301702=CARTESIAN_POINT('Ctrl Pts',(-3.10606665601013,16.5312499999444,
9.5594902125713));
#301703=CARTESIAN_POINT('Ctrl Pts',(-2.0142965867824E-14,16.6812499999438,
10.5687124469213));
#301704=CARTESIAN_POINT('Ctrl Pts',(3.10606665601009,16.8312499999432,9.5594902125713));
#301705=CARTESIAN_POINT('Ctrl Pts',(6.21213331202019,16.9812499999426,8.55026797822134));
#301706=CARTESIAN_POINT('Ctrl Pts',(8.13178807675717,17.131249999942,5.90808986649102));
#301707=CARTESIAN_POINT('Ctrl Pts',(10.0514428414941,17.2812499999414,3.2659117547607));
#301708=CARTESIAN_POINT('Ctrl Pts',(10.0514428414941,17.4312499999408,-1.23094673026484E-15));
#301709=CARTESIAN_POINT('Ctrl Pts',(10.0514428414941,17.5812499999402,-3.26591175476071));
#301710=CARTESIAN_POINT('Ctrl Pts',(8.13178807675717,17.7312499999396,-5.90808986649102));
#301711=CARTESIAN_POINT('Ctrl Pts',(6.21213331202019,17.881249999939,-8.55026797822134));
#301712=CARTESIAN_POINT('Ctrl Pts',(3.10606665601008,18.0312499999384,-9.5594902125713));
#301713=CARTESIAN_POINT('Ctrl Pts',(-2.35954084775011E-14,18.1812499999378,
-10.5687124469213));
#301714=CARTESIAN_POINT('Ctrl Pts',(-3.10606665601013,18.3312499999371,
-9.5594902125713));
#301715=CARTESIAN_POINT('Ctrl Pts',(-6.21213331202024,18.4812499999365,
-8.55026797822134));
#301716=CARTESIAN_POINT('Ctrl Pts',(-8.13178807675721,18.6312499999359,
-5.90808986649102));
#301717=CARTESIAN_POINT('Ctrl Pts',(-10.0514428414942,18.7812499999353,
-3.2659117547607));
#301718=CARTESIAN_POINT('Ctrl Pts',(-10.0514428414942,18.9312499999347,
2.46189346052968E-15));
#301719=CARTESIAN_POINT('Ctrl Pts',(-10.0514428414942,19.0812499999341,
3.26591175476071));
#301720=CARTESIAN_POINT('Ctrl Pts',(-8.13178807675721,19.2312499999335,
5.90808986649102));
#301721=CARTESIAN_POINT('Ctrl Pts',(-6.21213331202024,19.381249999933,8.55026797822134));
#301722=CARTESIAN_POINT('Ctrl Pts',(-3.10606665601013,19.5312499999323,
9.5594902125713));
#301723=CARTESIAN_POINT('Ctrl Pts',(-2.18706751394858E-14,19.6812499999318,
10.5687124469213));
#301724=CARTESIAN_POINT('Ctrl Pts',(3.10606665601009,19.8312499999312,9.5594902125713));
#301725=CARTESIAN_POINT('Ctrl Pts',(6.21213331202019,19.9812499999306,8.55026797822134));
#301726=CARTESIAN_POINT('Ctrl Pts',(8.13178807675717,20.13124999993,5.90808986649102));
#301727=CARTESIAN_POINT('Ctrl Pts',(10.0514428414941,20.2812499999294,3.2659117547607));
#301728=CARTESIAN_POINT('Ctrl Pts',(10.0514428414941,20.4312499999288,-1.23094673026484E-15));
#301729=CARTESIAN_POINT('Ctrl Pts',(10.0514428414941,20.5812499999282,-3.26591175476071));
#301730=CARTESIAN_POINT('Ctrl Pts',(8.13178807675716,20.7312499999276,-5.90808986649102));
#301731=CARTESIAN_POINT('Ctrl Pts',(6.21213331202019,20.881249999927,-8.55026797822134));
#301732=CARTESIAN_POINT('Ctrl Pts',(3.10606665601008,21.0312499999264,-9.5594902125713));
#301733=CARTESIAN_POINT('Ctrl Pts',(-2.53231177491629E-14,21.1812499999258,
-10.5687124469213));
#301734=CARTESIAN_POINT('Ctrl Pts',(-3.10606665601013,21.3312499999251,
-9.5594902125713));
#301735=CARTESIAN_POINT('Ctrl Pts',(-6.21213331202024,21.4812499999245,
-8.55026797822134));
#301736=CARTESIAN_POINT('Ctrl Pts',(-8.13178807675722,21.6312499999239,
-5.90808986649102));
#301737=CARTESIAN_POINT('Ctrl Pts',(-10.0514428414942,21.7812499999233,
-3.2659117547607));
#301738=CARTESIAN_POINT('Ctrl Pts',(-10.0514428414942,21.9312499999227,
2.46189346052968E-15));
#301739=CARTESIAN_POINT('Ctrl Pts',(-10.0514428414942,22.0812499999221,
3.26591175476071));
#301740=CARTESIAN_POINT('Ctrl Pts',(-8.13178807675722,22.2312499999215,
5.90808986649102));
#301741=CARTESIAN_POINT('Ctrl Pts',(-6.21213331202024,22.3812499999209,
8.55026797822134));
#301742=CARTESIAN_POINT('Ctrl Pts',(-3.10606665601013,22.5312499999204,
9.5594902125713));
#301743=CARTESIAN_POINT('Ctrl Pts',(-2.35983844111477E-14,22.6812499999198,
10.5687124469213));
#301744=CARTESIAN_POINT('Ctrl Pts',(3.10606665601008,22.8312499999192,9.5594902125713));
#301745=CARTESIAN_POINT('Ctrl Pts',(6.21213331202019,22.9812499999186,8.55026797822134));
#301746=CARTESIAN_POINT('Ctrl Pts',(8.13178807675716,23.131249999918,5.90808986649102));
#301747=CARTESIAN_POINT('Ctrl Pts',(10.0514428414941,23.2812499999174,3.2659117547607));
#301748=CARTESIAN_POINT('Ctrl Pts',(10.0514428414941,23.4312499999168,-1.23094673026484E-15));
#301749=CARTESIAN_POINT('Ctrl Pts',(10.0514428414941,23.5812499999162,-3.26591175476071));
#301750=CARTESIAN_POINT('Ctrl Pts',(8.13178807675716,23.7312499999156,-5.90808986649102));
#301751=CARTESIAN_POINT('Ctrl Pts',(6.21213331202019,23.881249999915,-8.55026797822134));
#301752=CARTESIAN_POINT('Ctrl Pts',(3.10606665601008,24.0312499999144,-9.5594902125713));
#301753=CARTESIAN_POINT('Ctrl Pts',(-2.70508270208248E-14,24.1812499999138,
-10.5687124469213));
#301754=CARTESIAN_POINT('Ctrl Pts',(-3.10606665601014,24.3312499999131,
-9.5594902125713));
#301755=CARTESIAN_POINT('Ctrl Pts',(-6.21213331202024,24.4812499999125,
-8.55026797822134));
#301756=CARTESIAN_POINT('Ctrl Pts',(-8.13178807675722,24.6312499999119,
-5.90808986649102));
#301757=CARTESIAN_POINT('Ctrl Pts',(-10.0514428414942,24.7812499999113,
-3.2659117547607));
#301758=CARTESIAN_POINT('Ctrl Pts',(-10.0514428414942,24.9312499999107,
2.46189346052968E-15));
#301759=CARTESIAN_POINT('Ctrl Pts',(-10.0514428414942,25.0812499999101,
3.26591175476071));
#301760=CARTESIAN_POINT('Ctrl Pts',(-8.13178807675722,25.2312499999095,
5.90808986649102));
#301761=CARTESIAN_POINT('Ctrl Pts',(-6.21213331202024,25.381249999909,8.55026797822134));
#301762=CARTESIAN_POINT('Ctrl Pts',(-3.10606665601013,25.5312499999084,
9.5594902125713));
#301763=CARTESIAN_POINT('Ctrl Pts',(-2.53260936828095E-14,25.6812499999078,
10.5687124469213));
#301764=CARTESIAN_POINT('Ctrl Pts',(3.10606665601008,25.8312499999072,9.5594902125713));
#301765=CARTESIAN_POINT('Ctrl Pts',(6.21213331202019,25.9812499999066,8.55026797822134));
#301766=CARTESIAN_POINT('Ctrl Pts',(8.13178807675716,26.131249999906,5.90808986649102));
#301767=CARTESIAN_POINT('Ctrl Pts',(10.0514428414941,26.2812499999054,3.2659117547607));
#301768=CARTESIAN_POINT('Ctrl Pts',(10.0514428414941,26.4312499999048,-1.23094673026484E-15));
#301769=CARTESIAN_POINT('Ctrl Pts',(10.0514428414941,26.5812499999042,-3.26591175476071));
#301770=CARTESIAN_POINT('Ctrl Pts',(8.13178807675716,26.7312499999036,-5.90808986649102));
#301771=CARTESIAN_POINT('Ctrl Pts',(6.21213331202019,26.881249999903,-8.55026797822134));
#301772=CARTESIAN_POINT('Ctrl Pts',(3.10606665601008,27.0312499999024,-9.5594902125713));
#301773=CARTESIAN_POINT('Ctrl Pts',(-2.87785362924866E-14,27.1812499999018,
-10.5687124469213));
#301774=CARTESIAN_POINT('Ctrl Pts',(-3.10606665601014,27.3312499999011,
-9.5594902125713));
#301775=CARTESIAN_POINT('Ctrl Pts',(-6.21213331202024,27.4812499999005,
-8.55026797822134));
#301776=CARTESIAN_POINT('Ctrl Pts',(-8.13178807675722,27.6312499998999,
-5.90808986649102));
#301777=CARTESIAN_POINT('Ctrl Pts',(-10.0514428414942,27.7812499998993,
-3.2659117547607));
#301778=CARTESIAN_POINT('Ctrl Pts',(-10.0514428414942,27.9312499998987,
2.46189346052968E-15));
#301779=CARTESIAN_POINT('Ctrl Pts',(-10.0514428414942,28.0812499998981,
3.26591175476071));
#301780=CARTESIAN_POINT('Ctrl Pts',(-8.13178807675722,28.2312499998975,
5.90808986649102));
#301781=CARTESIAN_POINT('Ctrl Pts',(-6.21213331202024,28.3812499998969,
8.55026797822134));
#301782=CARTESIAN_POINT('Ctrl Pts',(-3.10606665601014,28.5312499998964,
9.5594902125713));
#301783=CARTESIAN_POINT('Ctrl Pts',(-2.70538029544713E-14,28.6812499998958,
10.5687124469213));
#301784=CARTESIAN_POINT('Ctrl Pts',(3.10606665601008,28.8312499998952,9.5594902125713));
#301785=CARTESIAN_POINT('Ctrl Pts',(6.21213331202019,28.9812499998946,8.55026797822134));
#301786=CARTESIAN_POINT('Ctrl Pts',(8.13178807675716,29.131249999894,5.90808986649102));
#301787=CARTESIAN_POINT('Ctrl Pts',(10.0514428414941,29.2812499998934,3.2659117547607));
#301788=CARTESIAN_POINT('Ctrl Pts',(10.0514428414941,29.4312499998928,-1.23094673026484E-15));
#301789=CARTESIAN_POINT('Ctrl Pts',(10.0514428414941,29.5812499998922,-3.26591175476071));
#301790=CARTESIAN_POINT('Ctrl Pts',(8.13178807675716,29.7312499998916,-5.90808986649102));
#301791=CARTESIAN_POINT('Ctrl Pts',(6.21213331202019,29.881249999891,-8.55026797822134));
#301792=CARTESIAN_POINT('Ctrl Pts',(3.10606665601008,30.0312499998904,-9.5594902125713));
#301793=CARTESIAN_POINT('Ctrl Pts',(-3.05062455641484E-14,30.1812499998898,
-10.5687124469213));
#301794=CARTESIAN_POINT('Ctrl Pts',(-3.10606665601014,30.3312499998892,
-9.5594902125713));
#301795=CARTESIAN_POINT('Ctrl Pts',(-6.21213331202025,30.4812499998885,
-8.55026797822134));
#301796=CARTESIAN_POINT('Ctrl Pts',(-8.13178807675722,30.6312499998879,
-5.90808986649102));
#301797=CARTESIAN_POINT('Ctrl Pts',(-10.0514428414942,30.7812499998873,
-3.2659117547607));
#301798=CARTESIAN_POINT('Ctrl Pts',(-10.0514428414942,30.9312499998867,
2.46189346052968E-15));
#301799=CARTESIAN_POINT('Ctrl Pts',(-10.0514428414942,31.0812499998861,
3.26591175476071));
#301800=CARTESIAN_POINT('Ctrl Pts',(-8.13178807675722,31.2312499998855,
5.90808986649102));
#301801=CARTESIAN_POINT('Ctrl Pts',(-6.21213331202024,31.381249999885,8.55026797822134));
#301802=CARTESIAN_POINT('Ctrl Pts',(-3.10606665601014,31.5312499998843,
9.5594902125713));
#301803=CARTESIAN_POINT('Ctrl Pts',(-2.87815122261332E-14,31.6812499998838,
10.5687124469213));
#301804=CARTESIAN_POINT('Ctrl Pts',(3.10606665601008,31.8312499998832,9.5594902125713));
#301805=CARTESIAN_POINT('Ctrl Pts',(6.21213331202019,31.9812499998826,8.55026797822134));
#301806=CARTESIAN_POINT('Ctrl Pts',(8.13178807675716,32.131249999882,5.90808986649102));
#301807=CARTESIAN_POINT('Ctrl Pts',(10.0514428414941,32.2812499998814,3.2659117547607));
#301808=CARTESIAN_POINT('Ctrl Pts',(10.0514428414941,32.4312499998808,-1.23094673026484E-15));
#301809=CARTESIAN_POINT('Ctrl Pts',(10.0514428414941,32.5812499998802,-3.26591175476071));
#301810=CARTESIAN_POINT('Ctrl Pts',(8.13178807675716,32.7312499998796,-5.90808986649102));
#301811=CARTESIAN_POINT('Ctrl Pts',(6.21213331202019,32.8812499998789,-8.55026797822134));
#301812=CARTESIAN_POINT('Ctrl Pts',(3.10606665601008,33.0312499998784,-9.5594902125713));
#301813=CARTESIAN_POINT('Ctrl Pts',(-3.22339548358103E-14,33.1812499998777,
-10.5687124469213));
#301814=CARTESIAN_POINT('Ctrl Pts',(-3.10606665601014,33.3312499998772,
-9.5594902125713));
#301815=CARTESIAN_POINT('Ctrl Pts',(-6.21213331202025,33.4812499998766,
-8.55026797822134));
#301816=CARTESIAN_POINT('Ctrl Pts',(-8.13178807675722,33.6312499998759,
-5.90808986649102));
#301817=CARTESIAN_POINT('Ctrl Pts',(-10.0514428414942,33.7812499998753,
-3.2659117547607));
#301818=CARTESIAN_POINT('Ctrl Pts',(-10.0514428414942,33.9312499998747,
2.46189346052968E-15));
#301819=CARTESIAN_POINT('Ctrl Pts',(-10.0514428414942,34.0812499998741,
3.26591175476071));
#301820=CARTESIAN_POINT('Ctrl Pts',(-8.13178807675722,34.2312499998735,
5.90808986649102));
#301821=CARTESIAN_POINT('Ctrl Pts',(-6.21213331202024,34.3812499998729,
8.55026797822134));
#301822=CARTESIAN_POINT('Ctrl Pts',(-3.10606665601014,34.5312499998724,
9.5594902125713));
#301823=CARTESIAN_POINT('Ctrl Pts',(-3.0509221497795E-14,34.6812499998718,
10.5687124469213));
#301824=CARTESIAN_POINT('Ctrl Pts',(3.10606665601008,34.8312499998712,9.5594902125713));
#301825=CARTESIAN_POINT('Ctrl Pts',(6.21213331202019,34.9812499998706,8.55026797822134));
#301826=CARTESIAN_POINT('Ctrl Pts',(8.13178807675716,35.13124999987,5.90808986649102));
#301827=CARTESIAN_POINT('Ctrl Pts',(10.0514428414941,35.2812499998694,3.2659117547607));
#301828=CARTESIAN_POINT('Ctrl Pts',(10.0514428414941,35.4312499998688,-1.23094673026484E-15));
#301829=CARTESIAN_POINT('Ctrl Pts',(10.0514428414941,35.5812499998682,-3.26591175476071));
#301830=CARTESIAN_POINT('Ctrl Pts',(8.13178807675716,35.7312499998676,-5.90808986649102));
#301831=CARTESIAN_POINT('Ctrl Pts',(6.21213331202018,35.881249999867,-8.55026797822134));
#301832=CARTESIAN_POINT('Ctrl Pts',(3.10606665601007,36.0312499998664,-9.5594902125713));
#301833=CARTESIAN_POINT('Ctrl Pts',(-3.39616641074721E-14,36.1812499998658,
-10.5687124469213));
#301834=CARTESIAN_POINT('Ctrl Pts',(-3.10606665601014,36.3312499998652,
-9.5594902125713));
#301835=CARTESIAN_POINT('Ctrl Pts',(-6.21213331202025,36.4812499998646,
-8.55026797822134));
#301836=CARTESIAN_POINT('Ctrl Pts',(-8.13178807675722,36.6312499998639,
-5.90808986649102));
#301837=CARTESIAN_POINT('Ctrl Pts',(-10.0514428414942,36.7812499998634,
-3.2659117547607));
#301838=CARTESIAN_POINT('Ctrl Pts',(-10.0514428414942,36.9312499998627,
2.46189346052968E-15));
#301839=CARTESIAN_POINT('Ctrl Pts',(-10.0514428414942,37.0812499998621,
3.26591175476071));
#301840=CARTESIAN_POINT('Ctrl Pts',(-8.13178807675722,37.2312499998615,
5.90808986649102));
#301841=CARTESIAN_POINT('Ctrl Pts',(-6.21213331202025,37.3812499998609,
8.55026797822134));
#301842=CARTESIAN_POINT('Ctrl Pts',(-3.10606665601014,37.5312499998603,
9.5594902125713));
#301843=CARTESIAN_POINT('Ctrl Pts',(-3.22369307694568E-14,37.6812499998598,
10.5687124469213));
#301844=CARTESIAN_POINT('Ctrl Pts',(3.10606665601008,37.8312499998592,9.5594902125713));
#301845=CARTESIAN_POINT('Ctrl Pts',(6.21213331202018,37.9812499998586,8.55026797822134));
#301846=CARTESIAN_POINT('Ctrl Pts',(8.13178807675716,38.131249999858,5.90808986649102));
#301847=CARTESIAN_POINT('Ctrl Pts',(10.0514428414941,38.2812499998574,3.2659117547607));
#301848=CARTESIAN_POINT('Ctrl Pts',(10.0514428414941,38.4312499998568,-1.23094673026484E-15));
#301849=CARTESIAN_POINT('Ctrl Pts',(10.0514428414941,38.5812499998562,-3.26591175476071));
#301850=CARTESIAN_POINT('Ctrl Pts',(8.13178807675715,38.7312499998556,-5.90808986649102));
#301851=CARTESIAN_POINT('Ctrl Pts',(6.21213331202018,38.881249999855,-8.55026797822134));
#301852=CARTESIAN_POINT('Ctrl Pts',(3.10606665601007,39.0312499998544,-9.5594902125713));
#301853=CARTESIAN_POINT('Ctrl Pts',(-3.5689373379134E-14,39.1812499998538,
-10.5687124469213));
#301854=CARTESIAN_POINT('Ctrl Pts',(-3.10606665601014,39.3312499998532,
-9.5594902125713));
#301855=CARTESIAN_POINT('Ctrl Pts',(-6.21213331202025,39.4812499998525,
-8.55026797822134));
#301856=CARTESIAN_POINT('Ctrl Pts',(-8.13178807675723,39.6312499998519,
-5.90808986649102));
#301857=CARTESIAN_POINT('Ctrl Pts',(-10.0514428414942,39.7812499998513,
-3.2659117547607));
#301858=CARTESIAN_POINT('Ctrl Pts',(-10.0514428414942,39.9312499998507,
2.46189346052968E-15));
#301859=CARTESIAN_POINT('Ctrl Pts',(-10.0514428414942,40.0812499998502,
3.26591175476071));
#301860=CARTESIAN_POINT('Ctrl Pts',(-8.13178807675723,40.2312499998495,
5.90808986649102));
#301861=CARTESIAN_POINT('Ctrl Pts',(-6.21213331202025,40.3812499998489,
8.55026797822134));
#301862=CARTESIAN_POINT('Ctrl Pts',(-3.10606665601014,40.5312499998483,
9.5594902125713));
#301863=CARTESIAN_POINT('Ctrl Pts',(-3.39646400411187E-14,40.6812499998478,
10.5687124469213));
#301864=CARTESIAN_POINT('Ctrl Pts',(3.10606665601007,40.8312499998472,9.5594902125713));
#301865=CARTESIAN_POINT('Ctrl Pts',(6.21213331202018,40.9812499998466,8.55026797822134));
#301866=CARTESIAN_POINT('Ctrl Pts',(8.13178807675715,41.131249999846,5.90808986649102));
#301867=CARTESIAN_POINT('Ctrl Pts',(10.0514428414941,41.2812499998454,3.2659117547607));
#301868=CARTESIAN_POINT('Ctrl Pts',(10.0514428414941,41.4312499998448,-1.23094673026484E-15));
#301869=CARTESIAN_POINT('Ctrl Pts',(10.0514428414941,41.5812499998442,-3.26591175476071));
#301870=CARTESIAN_POINT('Ctrl Pts',(8.13178807675715,41.7312499998436,-5.90808986649102));
#301871=CARTESIAN_POINT('Ctrl Pts',(6.21213331202018,41.881249999843,-8.55026797822134));
#301872=CARTESIAN_POINT('Ctrl Pts',(3.10606665601007,42.0312499998423,-9.5594902125713));
#301873=CARTESIAN_POINT('Ctrl Pts',(-3.74170826507958E-14,42.1812499998418,
-10.5687124469213));
#301874=CARTESIAN_POINT('Ctrl Pts',(-3.10606665601015,42.3312499998411,
-9.5594902125713));
#301875=CARTESIAN_POINT('Ctrl Pts',(-6.21213331202025,42.4812499998406,
-8.55026797822134));
#301876=CARTESIAN_POINT('Ctrl Pts',(-8.13178807675723,42.6312499998399,
-5.90808986649102));
#301877=CARTESIAN_POINT('Ctrl Pts',(-10.0514428414942,42.7812499998393,
-3.2659117547607));
#301878=CARTESIAN_POINT('Ctrl Pts',(-10.0514428414942,42.9312499998387,
2.46189346052968E-15));
#301879=CARTESIAN_POINT('Ctrl Pts',(-10.0514428414942,43.0812499998381,
3.26591175476071));
#301880=CARTESIAN_POINT('Ctrl Pts',(-8.13178807675723,43.2312499998375,
5.90808986649102));
#301881=CARTESIAN_POINT('Ctrl Pts',(-6.21213331202025,43.3812499998369,
8.55026797822134));
#301882=CARTESIAN_POINT('Ctrl Pts',(-3.10606665601014,43.5312499998363,
9.5594902125713));
#301883=CARTESIAN_POINT('Ctrl Pts',(-3.56923493127805E-14,43.6812499998357,
10.5687124469213));
#301884=CARTESIAN_POINT('Ctrl Pts',(3.10606665601007,43.8312499998352,9.5594902125713));
#301885=CARTESIAN_POINT('Ctrl Pts',(6.21213331202018,43.9812499998345,8.55026797822134));
#301886=CARTESIAN_POINT('Ctrl Pts',(8.13178807675715,44.131249999834,5.90808986649102));
#301887=CARTESIAN_POINT('Ctrl Pts',(10.0514428414941,44.2812499998334,3.2659117547607));
#301888=CARTESIAN_POINT('Ctrl Pts',(10.0514428414941,44.4312499998328,-1.23094673026484E-15));
#301889=CARTESIAN_POINT('Ctrl Pts',(10.0514428414941,44.5812499998322,-3.26591175476071));
#301890=CARTESIAN_POINT('Ctrl Pts',(8.13178807675715,44.7312499998316,-5.90808986649102));
#301891=CARTESIAN_POINT('Ctrl Pts',(6.21213331202018,44.881249999831,-8.55026797822134));
#301892=CARTESIAN_POINT('Ctrl Pts',(3.10606665601007,45.0312499998304,-9.5594902125713));
#301893=CARTESIAN_POINT('Ctrl Pts',(-3.91447919224576E-14,45.1812499998297,
-10.5687124469213));
#301894=CARTESIAN_POINT('Ctrl Pts',(-3.10606665601015,45.3312499998292,
-9.5594902125713));
#301895=CARTESIAN_POINT('Ctrl Pts',(-6.21213331202026,45.4812499998285,
-8.55026797822134));
#301896=CARTESIAN_POINT('Ctrl Pts',(-8.13178807675723,45.6312499998279,
-5.90808986649102));
#301897=CARTESIAN_POINT('Ctrl Pts',(-10.0514428414942,45.7812499998273,
-3.2659117547607));
#301898=CARTESIAN_POINT('Ctrl Pts',(-10.0514428414942,45.9312499998267,
2.46189346052968E-15));
#301899=CARTESIAN_POINT('Ctrl Pts',(-10.0514428414942,46.0812499998261,
3.26591175476071));
#301900=CARTESIAN_POINT('Ctrl Pts',(-8.13178807675723,46.2312499998255,
5.90808986649102));
#301901=CARTESIAN_POINT('Ctrl Pts',(-6.21213331202025,46.3812499998249,
8.55026797822134));
#301902=CARTESIAN_POINT('Ctrl Pts',(-3.10606665601015,46.5312499998244,
9.5594902125713));
#301903=CARTESIAN_POINT('Ctrl Pts',(-3.74200585844424E-14,46.6812499998238,
10.5687124469213));
#301904=CARTESIAN_POINT('Ctrl Pts',(3.10606665601007,46.8312499998232,9.5594902125713));
#301905=CARTESIAN_POINT('Ctrl Pts',(6.21213331202018,46.9812499998226,8.55026797822134));
#301906=CARTESIAN_POINT('Ctrl Pts',(8.13178807675715,47.131249999822,5.90808986649102));
#301907=CARTESIAN_POINT('Ctrl Pts',(10.0514428414941,47.2812499998214,3.2659117547607));
#301908=CARTESIAN_POINT('Ctrl Pts',(10.0514428414941,47.4312499998208,-1.23094673026484E-15));
#301909=CARTESIAN_POINT('Ctrl Pts',(10.0514428414941,47.5812499998202,-3.26591175476071));
#301910=CARTESIAN_POINT('Ctrl Pts',(8.13178807675715,47.7312499998196,-5.90808986649102));
#301911=CARTESIAN_POINT('Ctrl Pts',(6.21213331202017,47.881249999819,-8.55026797822134));
#301912=CARTESIAN_POINT('Ctrl Pts',(3.10606665601007,48.0312499998184,-9.5594902125713));
#301913=CARTESIAN_POINT('Ctrl Pts',(-4.08725011941195E-14,48.1812499998178,
-10.5687124469213));
#301914=CARTESIAN_POINT('Ctrl Pts',(-3.10606665601015,48.3312499998172,
-9.5594902125713));
#301915=CARTESIAN_POINT('Ctrl Pts',(-6.21213331202026,48.4812499998166,
-8.55026797822134));
#301916=CARTESIAN_POINT('Ctrl Pts',(-8.13178807675723,48.6312499998159,
-5.90808986649102));
#301917=CARTESIAN_POINT('Ctrl Pts',(-10.0514428414942,48.7812499998153,
-3.2659117547607));
#301918=CARTESIAN_POINT('Ctrl Pts',(-10.0514428414942,48.9312499998147,
2.46189346052968E-15));
#301919=CARTESIAN_POINT('Ctrl Pts',(-10.0514428414942,49.0812499998141,
3.26591175476071));
#301920=CARTESIAN_POINT('Ctrl Pts',(-8.13178807675723,49.2312499998135,
5.90808986649102));
#301921=CARTESIAN_POINT('Ctrl Pts',(-6.21213331202026,49.3812499998129,
8.55026797822134));
#301922=CARTESIAN_POINT('Ctrl Pts',(-3.10606665601015,49.5312499998124,
9.5594902125713));
#301923=CARTESIAN_POINT('Ctrl Pts',(-3.91477678561042E-14,49.6812499998117,
10.5687124469213));
#301924=CARTESIAN_POINT('Ctrl Pts',(3.10606665601007,49.8312499998111,9.5594902125713));
#301925=CARTESIAN_POINT('Ctrl Pts',(6.21213331202017,49.9812499998106,8.55026797822134));
#301926=CARTESIAN_POINT('Ctrl Pts',(8.13178807675715,50.13124999981,5.90808986649102));
#301927=CARTESIAN_POINT('Ctrl Pts',(10.0514428414941,50.2812499998094,3.2659117547607));
#301928=CARTESIAN_POINT('Ctrl Pts',(10.0514428414941,50.4312499998088,-1.23094673026484E-15));
#301929=CARTESIAN_POINT('Ctrl Pts',(10.0514428414941,50.5812499998082,-3.26591175476071));
#301930=CARTESIAN_POINT('Ctrl Pts',(8.13178807675715,50.7312499998076,-5.90808986649102));
#301931=CARTESIAN_POINT('Ctrl Pts',(6.21213331202017,50.881249999807,-8.55026797822134));
#301932=CARTESIAN_POINT('Ctrl Pts',(3.10606665601007,51.0312499998064,-9.5594902125713));
#301933=CARTESIAN_POINT('Ctrl Pts',(-4.26002104657813E-14,51.1812499998058,
-10.5687124469213));
#301934=CARTESIAN_POINT('Ctrl Pts',(-3.10606665601015,51.3312499998052,
-9.5594902125713));
#301935=CARTESIAN_POINT('Ctrl Pts',(-6.21213331202026,51.4812499998045,
-8.55026797822134));
#301936=CARTESIAN_POINT('Ctrl Pts',(-8.13178807675723,51.631249999804,-5.90808986649102));
#301937=CARTESIAN_POINT('Ctrl Pts',(-10.0514428414942,51.7812499998034,
-3.2659117547607));
#301938=CARTESIAN_POINT('Ctrl Pts',(-10.0514428414942,51.9312499998027,
2.46189346052968E-15));
#301939=CARTESIAN_POINT('Ctrl Pts',(-10.0514428414942,52.0812499998021,
3.26591175476071));
#301940=CARTESIAN_POINT('Ctrl Pts',(-8.13178807675723,52.2312499998015,
5.90808986649102));
#301941=CARTESIAN_POINT('Ctrl Pts',(-6.21213331202026,52.3812499998009,
8.55026797822134));
#301942=CARTESIAN_POINT('Ctrl Pts',(-3.10606665601015,52.5312499998004,
9.5594902125713));
#301943=CARTESIAN_POINT('Ctrl Pts',(-4.08754771277661E-14,52.6812499997998,
10.5687124469213));
#301944=CARTESIAN_POINT('Ctrl Pts',(3.10606665601007,52.8312499997991,9.5594902125713));
#301945=CARTESIAN_POINT('Ctrl Pts',(6.21213331202017,52.9812499997986,8.55026797822134));
#301946=CARTESIAN_POINT('Ctrl Pts',(8.13178807675715,53.131249999798,5.90808986649102));
#301947=CARTESIAN_POINT('Ctrl Pts',(10.0514428414941,53.2812499997974,3.2659117547607));
#301948=CARTESIAN_POINT('Ctrl Pts',(10.0514428414941,53.4312499997968,-1.23094673026484E-15));
#301949=CARTESIAN_POINT('Ctrl Pts',(10.0514428414941,53.5812499997962,-3.26591175476071));
#301950=CARTESIAN_POINT('Ctrl Pts',(8.13178807675714,53.7312499997956,-5.90808986649102));
#301951=CARTESIAN_POINT('Ctrl Pts',(6.21213331202017,53.881249999795,-8.55026797822134));
#301952=CARTESIAN_POINT('Ctrl Pts',(3.10606665601006,54.0312499997944,-9.5594902125713));
#301953=CARTESIAN_POINT('Ctrl Pts',(-4.43279197374432E-14,54.1812499997938,
-10.5687124469213));
#301954=CARTESIAN_POINT('Ctrl Pts',(-3.10606665601015,54.3312499997932,
-9.5594902125713));
#301955=CARTESIAN_POINT('Ctrl Pts',(-6.21213331202026,54.4812499997926,
-8.55026797822134));
#301956=CARTESIAN_POINT('Ctrl Pts',(-8.13178807675724,54.6312499997919,
-5.90808986649102));
#301957=CARTESIAN_POINT('Ctrl Pts',(-10.0514428414942,54.7812499997914,
-3.2659117547607));
#301958=CARTESIAN_POINT('Ctrl Pts',(-10.0514428414942,54.9312499997907,
2.46189346052968E-15));
#301959=CARTESIAN_POINT('Ctrl Pts',(-10.0514428414942,55.0812499997901,
3.26591175476071));
#301960=CARTESIAN_POINT('Ctrl Pts',(-8.13178807675724,55.2312499997895,
5.90808986649102));
#301961=CARTESIAN_POINT('Ctrl Pts',(-6.21213331202026,55.3812499997889,
8.55026797822134));
#301962=CARTESIAN_POINT('Ctrl Pts',(-3.10606665601015,55.5312499997884,
9.5594902125713));
#301963=CARTESIAN_POINT('Ctrl Pts',(-4.26031863994279E-14,55.6812499997877,
10.5687124469213));
#301964=CARTESIAN_POINT('Ctrl Pts',(3.10606665601006,55.8312499997871,9.5594902125713));
#301965=CARTESIAN_POINT('Ctrl Pts',(6.21213331202017,55.9812499997865,8.55026797822134));
#301966=CARTESIAN_POINT('Ctrl Pts',(8.13178807675714,56.131249999786,5.90808986649102));
#301967=CARTESIAN_POINT('Ctrl Pts',(10.0514428414941,56.2812499997854,3.2659117547607));
#301968=CARTESIAN_POINT('Ctrl Pts',(10.0514428414941,56.4312499997848,-1.23094673026484E-15));
#301969=CARTESIAN_POINT('Ctrl Pts',(10.0514428414941,56.5812499997842,-3.26591175476071));
#301970=CARTESIAN_POINT('Ctrl Pts',(8.13178807675714,56.7312499997836,-5.90808986649102));
#301971=CARTESIAN_POINT('Ctrl Pts',(6.21213331202017,56.881249999783,-8.55026797822134));
#301972=CARTESIAN_POINT('Ctrl Pts',(3.10606665601006,57.0312499997824,-9.5594902125713));
#301973=CARTESIAN_POINT('Ctrl Pts',(-4.6055629009105E-14,57.1812499997818,
-10.5687124469213));
#301974=CARTESIAN_POINT('Ctrl Pts',(-3.10606665601015,57.3312499997812,
-9.5594902125713));
#301975=CARTESIAN_POINT('Ctrl Pts',(-6.21213331202026,57.4812499997805,
-8.55026797822134));
#301976=CARTESIAN_POINT('Ctrl Pts',(-8.13178807675724,57.6312499997799,
-5.90808986649102));
#301977=CARTESIAN_POINT('Ctrl Pts',(-10.0514428414942,57.7812499997793,
-3.2659117547607));
#301978=CARTESIAN_POINT('Ctrl Pts',(-10.0514428414942,57.9312499997787,
2.46189346052968E-15));
#301979=CARTESIAN_POINT('Ctrl Pts',(-10.0514428414942,58.0812499997781,
3.26591175476071));
#301980=CARTESIAN_POINT('Ctrl Pts',(-8.13178807675724,58.2312499997775,
5.90808986649102));
#301981=CARTESIAN_POINT('Ctrl Pts',(-6.21213331202026,58.3812499997769,
8.55026797822134));
#301982=CARTESIAN_POINT('Ctrl Pts',(-3.10606665601015,58.5312499997763,
9.5594902125713));
#301983=CARTESIAN_POINT('Ctrl Pts',(-4.43308956710897E-14,58.6812499997758,
10.5687124469213));
#301984=CARTESIAN_POINT('Ctrl Pts',(3.10606665601006,58.8312499997751,9.5594902125713));
#301985=CARTESIAN_POINT('Ctrl Pts',(6.21213331202017,58.9812499997745,8.55026797822134));
#301986=CARTESIAN_POINT('Ctrl Pts',(8.13178807675714,59.131249999774,5.90808986649102));
#301987=CARTESIAN_POINT('Ctrl Pts',(10.0514428414941,59.2812499997734,3.2659117547607));
#301988=CARTESIAN_POINT('Ctrl Pts',(10.0514428414941,59.4312499997728,-1.23094673026484E-15));
#301989=CARTESIAN_POINT('Ctrl Pts',(10.0514428414941,59.5812499997722,-3.26591175476071));
#301990=CARTESIAN_POINT('Ctrl Pts',(8.13178807675714,59.7312499997716,-5.90808986649102));
#301991=CARTESIAN_POINT('Ctrl Pts',(6.21213331202017,59.881249999771,-8.55026797822134));
#301992=CARTESIAN_POINT('Ctrl Pts',(3.10606665601006,60.0312499997704,-9.5594902125713));
#301993=CARTESIAN_POINT('Ctrl Pts',(-4.77833382807668E-14,60.1812499997698,
-10.5687124469213));
#301994=CARTESIAN_POINT('Ctrl Pts',(-3.10606665601016,60.3312499997692,
-9.5594902125713));
#301995=CARTESIAN_POINT('Ctrl Pts',(-6.21213331202026,60.4812499997686,
-8.55026797822134));
#301996=CARTESIAN_POINT('Ctrl Pts',(-8.13178807675724,60.6312499997679,
-5.90808986649102));
#301997=CARTESIAN_POINT('Ctrl Pts',(-10.0514428414942,60.7812499997674,
-3.2659117547607));
#301998=CARTESIAN_POINT('Ctrl Pts',(-10.0514428414942,60.9312499997667,
2.46189346052968E-15));
#301999=CARTESIAN_POINT('Ctrl Pts',(-10.0514428414942,61.0812499997661,
3.26591175476071));
#302000=CARTESIAN_POINT('Ctrl Pts',(-8.13178807675724,61.2312499997655,
5.90808986649102));
#302001=CARTESIAN_POINT('Ctrl Pts',(-6.21213331202026,61.3812499997649,
8.55026797822134));
#302002=CARTESIAN_POINT('Ctrl Pts',(-3.10606665601015,61.5312499997643,
9.5594902125713));
#302003=CARTESIAN_POINT('Ctrl Pts',(-4.60586049427516E-14,61.6812499997638,
10.5687124469213));
#302004=CARTESIAN_POINT('Ctrl Pts',(3.10606665601006,61.8312499997632,9.5594902125713));
#302005=CARTESIAN_POINT('Ctrl Pts',(6.21213331202017,61.9812499997625,8.55026797822134));
#302006=CARTESIAN_POINT('Ctrl Pts',(8.13178807675714,62.131249999762,5.90808986649102));
#302007=CARTESIAN_POINT('Ctrl Pts',(10.0514428414941,62.2812499997614,3.2659117547607));
#302008=CARTESIAN_POINT('Ctrl Pts',(10.0514428414941,62.4312499997608,-1.23094673026484E-15));
#302009=CARTESIAN_POINT('Ctrl Pts',(10.0514428414941,62.5812499997602,-3.26591175476071));
#302010=CARTESIAN_POINT('Ctrl Pts',(8.13178807675714,62.7312499997596,-5.90808986649102));
#302011=CARTESIAN_POINT('Ctrl Pts',(6.21213331202017,62.881249999759,-8.55026797822134));
#302012=CARTESIAN_POINT('Ctrl Pts',(3.10606665601006,63.0312499997584,-9.5594902125713));
#302013=CARTESIAN_POINT('Ctrl Pts',(-4.95110475524287E-14,63.1812499997578,
-10.5687124469213));
#302014=CARTESIAN_POINT('Ctrl Pts',(-3.10606665601016,63.3312499997572,
-9.5594902125713));
#302015=CARTESIAN_POINT('Ctrl Pts',(-6.21213331202027,63.4812499997565,
-8.55026797822134));
#302016=CARTESIAN_POINT('Ctrl Pts',(-8.13178807675724,63.631249999756,-5.90808986649102));
#302017=CARTESIAN_POINT('Ctrl Pts',(-10.0514428414942,63.7812499997553,
-3.2659117547607));
#302018=CARTESIAN_POINT('Ctrl Pts',(-10.0514428414942,63.9312499997548,
2.46189346052968E-15));
#302019=CARTESIAN_POINT('Ctrl Pts',(-10.0514428414942,64.0812499997541,
3.26591175476071));
#302020=CARTESIAN_POINT('Ctrl Pts',(-8.13178807675724,64.2312499997535,
5.90808986649102));
#302021=CARTESIAN_POINT('Ctrl Pts',(-6.21213331202026,64.381249999753,8.55026797822134));
#302022=CARTESIAN_POINT('Ctrl Pts',(-3.10606665601016,64.5312499997523,
9.5594902125713));
#302023=CARTESIAN_POINT('Ctrl Pts',(-4.77863142144134E-14,64.6812499997518,
10.5687124469213));
#302024=CARTESIAN_POINT('Ctrl Pts',(3.10606665601006,64.8312499997512,9.5594902125713));
#302025=CARTESIAN_POINT('Ctrl Pts',(6.21213331202017,64.9812499997506,8.55026797822134));
#302026=CARTESIAN_POINT('Ctrl Pts',(8.13178807675714,65.13124999975,5.90808986649102));
#302027=CARTESIAN_POINT('Ctrl Pts',(10.0514428414941,65.2812499997493,3.2659117547607));
#302028=CARTESIAN_POINT('Ctrl Pts',(10.0514428414941,65.4312499997488,-1.23094673026484E-15));
#302029=CARTESIAN_POINT('Ctrl Pts',(10.0514428414941,65.5812499997482,-3.26591175476071));
#302030=CARTESIAN_POINT('Ctrl Pts',(8.13178807675714,65.7312499997475,-5.90808986649102));
#302031=CARTESIAN_POINT('Ctrl Pts',(6.21213331202016,65.881249999747,-8.55026797822134));
#302032=CARTESIAN_POINT('Ctrl Pts',(3.10606665601006,66.0312499997464,-9.5594902125713));
#302033=CARTESIAN_POINT('Ctrl Pts',(-5.12387568240905E-14,66.1812499997457,
-10.5687124469213));
#302034=CARTESIAN_POINT('Ctrl Pts',(-3.10606665601016,66.3312499997451,
-9.5594902125713));
#302035=CARTESIAN_POINT('Ctrl Pts',(-6.21213331202027,66.4812499997445,
-8.55026797822134));
#302036=CARTESIAN_POINT('Ctrl Pts',(-8.13178807675724,66.6312499997439,
-5.90808986649102));
#302037=CARTESIAN_POINT('Ctrl Pts',(-10.0514428414942,66.7812499997433,
-3.2659117547607));
#302038=CARTESIAN_POINT('Ctrl Pts',(-10.0514428414942,66.9312499997427,
2.46189346052968E-15));
#302039=CARTESIAN_POINT('Ctrl Pts',(-10.0514428414942,67.0812499997421,
3.26591175476071));
#302040=CARTESIAN_POINT('Ctrl Pts',(-8.13178807675724,67.2312499997416,
5.90808986649102));
#302041=CARTESIAN_POINT('Ctrl Pts',(-6.21213331202027,67.3812499997409,
8.55026797822134));
#302042=CARTESIAN_POINT('Ctrl Pts',(-3.10606665601016,67.5312499997404,
9.5594902125713));
#302043=CARTESIAN_POINT('Ctrl Pts',(-4.95140234860752E-14,67.6812499997397,
10.5687124469213));
#302044=CARTESIAN_POINT('Ctrl Pts',(3.10606665601006,67.8312499997391,9.5594902125713));
#302045=CARTESIAN_POINT('Ctrl Pts',(6.21213331202017,67.9812499997385,8.55026797822134));
#302046=CARTESIAN_POINT('Ctrl Pts',(8.13178807675714,68.1312499997379,5.90808986649102));
#302047=CARTESIAN_POINT('Ctrl Pts',(10.0514428414941,68.2812499997374,3.2659117547607));
#302048=CARTESIAN_POINT('Ctrl Pts',(10.0514428414941,68.4312499997367,-1.23094673026484E-15));
#302049=CARTESIAN_POINT('Ctrl Pts',(10.0514428414941,68.5812499997361,-3.26591175476071));
#302050=CARTESIAN_POINT('Ctrl Pts',(8.13178807675714,68.7312499997356,-5.90808986649102));
#302051=CARTESIAN_POINT('Ctrl Pts',(6.21213331202016,68.881249999735,-8.55026797822134));
#302052=CARTESIAN_POINT('Ctrl Pts',(3.10606665601006,69.0312499997344,-9.5594902125713));
#302053=CARTESIAN_POINT('Ctrl Pts',(-5.29664660957524E-14,69.1812499997337,
-10.5687124469213));
#302054=CARTESIAN_POINT('Ctrl Pts',(-3.10606665601016,69.3312499997332,
-9.5594902125713));
#302055=CARTESIAN_POINT('Ctrl Pts',(-6.21213331202027,69.4812499997326,
-8.55026797822134));
#302056=CARTESIAN_POINT('Ctrl Pts',(-8.13178807675724,69.6312499997319,
-5.90808986649102));
#302057=CARTESIAN_POINT('Ctrl Pts',(-10.0514428414942,69.7812499997313,
-3.2659117547607));
#302058=CARTESIAN_POINT('Ctrl Pts',(-10.0514428414942,69.9312499997307,
2.46189346052968E-15));
#302059=CARTESIAN_POINT('Ctrl Pts',(-10.0514428414942,70.0812499997301,
3.26591175476071));
#302060=CARTESIAN_POINT('Ctrl Pts',(-8.13178807675724,70.2312499997295,
5.90808986649102));
#302061=CARTESIAN_POINT('Ctrl Pts',(-6.21213331202027,70.3812499997289,
8.55026797822134));
#302062=CARTESIAN_POINT('Ctrl Pts',(-3.10606665601016,70.5312499997283,
9.5594902125713));
#302063=CARTESIAN_POINT('Ctrl Pts',(-5.12417327577371E-14,70.6812499997277,
10.5687124469213));
#302064=CARTESIAN_POINT('Ctrl Pts',(3.10606665601006,70.8312499997271,9.5594902125713));
#302065=CARTESIAN_POINT('Ctrl Pts',(6.21213331202016,70.9812499997265,8.55026797822134));
#302066=CARTESIAN_POINT('Ctrl Pts',(8.13178807675714,71.131249999726,5.90808986649102));
#302067=CARTESIAN_POINT('Ctrl Pts',(10.0514428414941,71.2812499997253,3.2659117547607));
#302068=CARTESIAN_POINT('Ctrl Pts',(10.0514428414941,71.4312499997248,-1.23094673026484E-15));
#302069=CARTESIAN_POINT('Ctrl Pts',(10.0514428414941,71.5812499997242,-3.26591175476071));
#302070=CARTESIAN_POINT('Ctrl Pts',(8.13178807675713,71.7312499997236,-5.90808986649102));
#302071=CARTESIAN_POINT('Ctrl Pts',(6.21213331202016,71.881249999723,-8.55026797822134));
#302072=CARTESIAN_POINT('Ctrl Pts',(3.10606665601005,72.0312499997223,-9.5594902125713));
#302073=CARTESIAN_POINT('Ctrl Pts',(-5.46941753674142E-14,72.1812499997217,
-10.5687124469213));
#302074=CARTESIAN_POINT('Ctrl Pts',(-3.10606665601016,72.3312499997212,
-9.5594902125713));
#302075=CARTESIAN_POINT('Ctrl Pts',(-6.21213331202027,72.4812499997205,
-8.55026797822134));
#302076=CARTESIAN_POINT('Ctrl Pts',(-8.13178807675725,72.63124999972,-5.90808986649102));
#302077=CARTESIAN_POINT('Ctrl Pts',(-10.0514428414942,72.7812499997193,
-3.2659117547607));
#302078=CARTESIAN_POINT('Ctrl Pts',(-10.0514428414942,72.9312499997187,
2.46189346052968E-15));
#302079=CARTESIAN_POINT('Ctrl Pts',(-10.0514428414942,73.0812499997181,
3.26591175476071));
#302080=CARTESIAN_POINT('Ctrl Pts',(-8.13178807675725,73.2312499997175,
5.90808986649102));
#302081=CARTESIAN_POINT('Ctrl Pts',(-6.21213331202027,73.381249999717,8.55026797822134));
#302082=CARTESIAN_POINT('Ctrl Pts',(-3.10606665601016,73.5312499997164,
9.5594902125713));
#302083=CARTESIAN_POINT('Ctrl Pts',(-5.29694420293989E-14,73.6812499997157,
10.5687124469213));
#302084=CARTESIAN_POINT('Ctrl Pts',(3.10606665601005,73.8312499997151,9.5594902125713));
#302085=CARTESIAN_POINT('Ctrl Pts',(6.21213331202016,73.9812499997146,8.55026797822134));
#302086=CARTESIAN_POINT('Ctrl Pts',(8.13178807675713,74.1312499997139,5.90808986649102));
#302087=CARTESIAN_POINT('Ctrl Pts',(10.0514428414941,74.2812499997134,3.2659117547607));
#302088=CARTESIAN_POINT('Ctrl Pts',(10.0514428414941,74.4312499997127,-1.23094673026484E-15));
#302089=CARTESIAN_POINT('Ctrl Pts',(10.0514428414941,74.5812499997122,-3.26591175476071));
#302090=CARTESIAN_POINT('Ctrl Pts',(8.13178807675713,74.7312499997116,-5.90808986649102));
#302091=CARTESIAN_POINT('Ctrl Pts',(6.21213331202016,74.8812499997109,-8.55026797822134));
#302092=CARTESIAN_POINT('Ctrl Pts',(3.10606665601005,75.0312499997104,-9.5594902125713));
#302093=CARTESIAN_POINT('Ctrl Pts',(-5.6421884639076E-14,75.1812499997098,
-10.5687124469213));
#302094=CARTESIAN_POINT('Ctrl Pts',(-3.10606665601016,75.3312499997092,
-9.5594902125713));
#302095=CARTESIAN_POINT('Ctrl Pts',(-6.21213331202027,75.4812499997086,
-8.55026797822134));
#302096=CARTESIAN_POINT('Ctrl Pts',(-8.13178807675725,75.6312499997079,
-5.90808986649102));
#302097=CARTESIAN_POINT('Ctrl Pts',(-10.0514428414942,75.7812499997073,
-3.2659117547607));
#302098=CARTESIAN_POINT('Ctrl Pts',(-10.0514428414942,75.9312499997068,
2.46189346052968E-15));
#302099=CARTESIAN_POINT('Ctrl Pts',(-10.0514428414942,76.0812499997061,
3.26591175476071));
#302100=CARTESIAN_POINT('Ctrl Pts',(-8.13178807675725,76.2312499997055,
5.90808986649102));
#302101=CARTESIAN_POINT('Ctrl Pts',(-6.21213331202027,76.3812499997049,
8.55026797822134));
#302102=CARTESIAN_POINT('Ctrl Pts',(-3.10606665601016,76.5312499997043,
9.5594902125713));
#302103=CARTESIAN_POINT('Ctrl Pts',(-5.46971513010608E-14,76.6812499997037,
10.5687124469213));
#302104=CARTESIAN_POINT('Ctrl Pts',(3.10606665601005,76.8312499997031,9.5594902125713));
#302105=CARTESIAN_POINT('Ctrl Pts',(6.21213331202016,76.9812499997025,8.55026797822134));
#302106=CARTESIAN_POINT('Ctrl Pts',(8.13178807675713,77.131249999702,5.90808986649102));
#302107=CARTESIAN_POINT('Ctrl Pts',(10.0514428414941,77.2812499997013,3.2659117547607));
#302108=CARTESIAN_POINT('Ctrl Pts',(10.0514428414941,77.4312499997008,-1.23094673026484E-15));
#302109=CARTESIAN_POINT('Ctrl Pts',(10.0514428414941,77.5812499997001,-3.26591175476071));
#302110=CARTESIAN_POINT('Ctrl Pts',(8.13178807675713,77.7312499996995,-5.90808986649102));
#302111=CARTESIAN_POINT('Ctrl Pts',(6.21213331202016,77.881249999699,-8.55026797822134));
#302112=CARTESIAN_POINT('Ctrl Pts',(3.10606665601005,78.0312499996984,-9.5594902125713));
#302113=CARTESIAN_POINT('Ctrl Pts',(-5.81495939107379E-14,78.1812499996978,
-10.5687124469213));
#302114=CARTESIAN_POINT('Ctrl Pts',(-3.10606665601017,78.3312499996971,
-9.5594902125713));
#302115=CARTESIAN_POINT('Ctrl Pts',(-6.21213331202028,78.4812499996966,
-8.55026797822134));
#302116=CARTESIAN_POINT('Ctrl Pts',(-8.13178807675725,78.631249999696,-5.90808986649102));
#302117=CARTESIAN_POINT('Ctrl Pts',(-10.0514428414942,78.7812499996954,
-3.2659117547607));
#302118=CARTESIAN_POINT('Ctrl Pts',(-10.0514428414942,78.9312499996948,
2.46189346052968E-15));
#302119=CARTESIAN_POINT('Ctrl Pts',(-10.0514428414942,79.0812499996942,
3.26591175476071));
#302120=CARTESIAN_POINT('Ctrl Pts',(-8.13178807675725,79.2312499996936,
5.90808986649102));
#302121=CARTESIAN_POINT('Ctrl Pts',(-6.21213331202027,79.381249999693,8.55026797822134));
#302122=CARTESIAN_POINT('Ctrl Pts',(-3.10606665601016,79.5312499996923,
9.5594902125713));
#302123=CARTESIAN_POINT('Ctrl Pts',(-5.64248605727226E-14,79.6812499996917,
10.5687124469213));
#302124=CARTESIAN_POINT('Ctrl Pts',(3.10606665601005,79.8312499996911,9.5594902125713));
#302125=CARTESIAN_POINT('Ctrl Pts',(6.21213331202016,79.9812499996905,8.55026797822134));
#302126=CARTESIAN_POINT('Ctrl Pts',(8.13178807675713,80.1312499996899,5.90808986649102));
#302127=CARTESIAN_POINT('Ctrl Pts',(10.0514428414941,80.2812499996894,3.2659117547607));
#302128=CARTESIAN_POINT('Ctrl Pts',(10.0514428414941,80.4312499996887,-1.23094673026484E-15));
#302129=CARTESIAN_POINT('Ctrl Pts',(10.0514428414941,80.5812499996882,-3.26591175476071));
#302130=CARTESIAN_POINT('Ctrl Pts',(8.13178807675713,80.7312499996875,-5.90808986649102));
#302131=CARTESIAN_POINT('Ctrl Pts',(6.21213331202016,80.881249999687,-8.55026797822134));
#302132=CARTESIAN_POINT('Ctrl Pts',(3.10606665601005,81.0312499996864,-9.5594902125713));
#302133=CARTESIAN_POINT('Ctrl Pts',(-5.98773031823997E-14,81.1812499996858,
-10.5687124469213));
#302134=CARTESIAN_POINT('Ctrl Pts',(-3.10606665601017,81.3312499996851,
-9.5594902125713));
#302135=CARTESIAN_POINT('Ctrl Pts',(-6.21213331202028,81.4812499996845,
-8.55026797822134));
#302136=CARTESIAN_POINT('Ctrl Pts',(-8.13178807675725,81.6312499996839,
-5.90808986649102));
#302137=CARTESIAN_POINT('Ctrl Pts',(-10.0514428414942,81.7812499996834,
-3.2659117547607));
#302138=CARTESIAN_POINT('Ctrl Pts',(-10.0514428414942,81.9312499996827,
2.46189346052968E-15));
#302139=CARTESIAN_POINT('Ctrl Pts',(-10.0514428414942,82.0812499996821,
3.26591175476071));
#302140=CARTESIAN_POINT('Ctrl Pts',(-8.13178807675725,82.2312499996816,
5.90808986649102));
#302141=CARTESIAN_POINT('Ctrl Pts',(-6.21213331202028,82.381249999681,8.55026797822134));
#302142=CARTESIAN_POINT('Ctrl Pts',(-3.10606665601017,82.5312499996804,
9.5594902125713));
#302143=CARTESIAN_POINT('Ctrl Pts',(-5.81525698443845E-14,82.6812499996797,
10.5687124469213));
#302144=CARTESIAN_POINT('Ctrl Pts',(3.10606665601005,82.8312499996792,9.5594902125713));
#302145=CARTESIAN_POINT('Ctrl Pts',(6.21213331202016,82.9812499996786,8.55026797822134));
#302146=CARTESIAN_POINT('Ctrl Pts',(8.13178807675713,83.131249999678,5.90808986649102));
#302147=CARTESIAN_POINT('Ctrl Pts',(10.0514428414941,83.2812499996773,3.2659117547607));
#302148=CARTESIAN_POINT('Ctrl Pts',(10.0514428414941,83.4312499996767,-1.23094673026484E-15));
#302149=CARTESIAN_POINT('Ctrl Pts',(10.0514428414941,83.5812499996761,-3.26591175476071));
#302150=CARTESIAN_POINT('Ctrl Pts',(8.13178807675713,83.7312499996756,-5.90808986649102));
#302151=CARTESIAN_POINT('Ctrl Pts',(6.21213331202016,83.8812499996749,-8.55026797822134));
#302152=CARTESIAN_POINT('Ctrl Pts',(3.10606665601005,84.0312499996743,-9.5594902125713));
#302153=CARTESIAN_POINT('Ctrl Pts',(-6.16050124540615E-14,84.1812499996738,
-10.5687124469213));
#302154=CARTESIAN_POINT('Ctrl Pts',(-3.10606665601017,84.3312499996732,
-9.5594902125713));
#302155=CARTESIAN_POINT('Ctrl Pts',(-6.21213331202028,84.4812499996725,
-8.55026797822134));
#302156=CARTESIAN_POINT('Ctrl Pts',(-8.13178807675725,84.631249999672,-5.90808986649102));
#302157=CARTESIAN_POINT('Ctrl Pts',(-10.0514428414942,84.7812499996714,
-3.2659117547607));
#302158=CARTESIAN_POINT('Ctrl Pts',(-10.0514428414942,84.9312499996708,
2.46189346052968E-15));
#302159=CARTESIAN_POINT('Ctrl Pts',(-10.0514428414942,85.0812499996701,
3.26591175476071));
#302160=CARTESIAN_POINT('Ctrl Pts',(-8.13178807675725,85.2312499996695,
5.90808986649102));
#302161=CARTESIAN_POINT('Ctrl Pts',(-6.21213331202028,85.381249999669,8.55026797822134));
#302162=CARTESIAN_POINT('Ctrl Pts',(-3.10606665601017,85.5312499996683,
9.5594902125713));
#302163=CARTESIAN_POINT('Ctrl Pts',(-5.98802791160463E-14,85.6812499996678,
10.5687124469213));
#302164=CARTESIAN_POINT('Ctrl Pts',(3.10606665601005,85.8312499996672,9.5594902125713));
#302165=CARTESIAN_POINT('Ctrl Pts',(6.21213331202016,85.9812499996666,8.55026797822134));
#302166=CARTESIAN_POINT('Ctrl Pts',(8.13178807675713,86.1312499996659,5.90808986649102));
#302167=CARTESIAN_POINT('Ctrl Pts',(10.0514428414941,86.2812499996653,3.2659117547607));
#302168=CARTESIAN_POINT('Ctrl Pts',(10.0514428414941,86.4312499996647,-1.23094673026484E-15));
#302169=CARTESIAN_POINT('Ctrl Pts',(10.0514428414941,86.5812499996642,-3.26591175476071));
#302170=CARTESIAN_POINT('Ctrl Pts',(8.13178807675713,86.7312499996635,-5.90808986649102));
#302171=CARTESIAN_POINT('Ctrl Pts',(6.21213331202015,86.8812499996629,-8.55026797822134));
#302172=CARTESIAN_POINT('Ctrl Pts',(3.10606665601004,87.0312499996624,-9.5594902125713));
#302173=CARTESIAN_POINT('Ctrl Pts',(-6.33327217257234E-14,87.1812499996618,
-10.5687124469213));
#302174=CARTESIAN_POINT('Ctrl Pts',(-3.10606665601017,87.3312499996611,
-9.5594902125713));
#302175=CARTESIAN_POINT('Ctrl Pts',(-6.21213331202028,87.4812499996605,
-8.55026797822134));
#302176=CARTESIAN_POINT('Ctrl Pts',(-8.13178807675726,87.6312499996599,
-5.90808986649102));
#302177=CARTESIAN_POINT('Ctrl Pts',(-10.0514428414942,87.7812499996594,
-3.2659117547607));
#302178=CARTESIAN_POINT('Ctrl Pts',(-10.0514428414942,87.9312499996587,
2.46189346052968E-15));
#302179=CARTESIAN_POINT('Ctrl Pts',(-10.0514428414942,88.0812499996581,
3.26591175476071));
#302180=CARTESIAN_POINT('Ctrl Pts',(-8.13178807675726,88.2312499996575,
5.90808986649102));
#302181=CARTESIAN_POINT('Ctrl Pts',(-6.21213331202028,88.3812499996569,
8.55026797822134));
#302182=CARTESIAN_POINT('Ctrl Pts',(-3.10606665601017,88.5312499996564,
9.5594902125713));
#302183=CARTESIAN_POINT('Ctrl Pts',(-6.16079883877081E-14,88.6812499996557,
10.5687124469213));
#302184=CARTESIAN_POINT('Ctrl Pts',(3.10606665601005,88.8312499996552,9.5594902125713));
#302185=CARTESIAN_POINT('Ctrl Pts',(6.21213331202016,88.9812499996546,8.55026797822134));
#302186=CARTESIAN_POINT('Ctrl Pts',(8.13178807675713,89.131249999654,5.90808986649102));
#302187=CARTESIAN_POINT('Ctrl Pts',(10.0514428414941,89.2812499996533,3.2659117547607));
#302188=CARTESIAN_POINT('Ctrl Pts',(10.0514428414941,89.4312499996527,-1.23094673026484E-15));
#302189=CARTESIAN_POINT('Ctrl Pts',(10.0514428414941,89.5812499996521,-3.26591175476071));
#302190=CARTESIAN_POINT('Ctrl Pts',(8.13178807675713,89.7312499996515,-5.90808986649102));
#302191=CARTESIAN_POINT('Ctrl Pts',(6.21213331202015,89.8812499996509,-8.55026797822134));
#302192=CARTESIAN_POINT('Ctrl Pts',(3.10606665601004,90.0312499996504,-9.5594902125713));
#302193=CARTESIAN_POINT('Ctrl Pts',(-6.50604309973852E-14,90.1812499996498,
-10.5687124469213));
#302194=CARTESIAN_POINT('Ctrl Pts',(-3.10606665601017,90.3312499996491,
-9.5594902125713));
#302195=CARTESIAN_POINT('Ctrl Pts',(-6.21213331202028,90.4812499996485,
-8.55026797822134));
#302196=CARTESIAN_POINT('Ctrl Pts',(-8.13178807675726,90.631249999648,-5.90808986649102));
#302197=CARTESIAN_POINT('Ctrl Pts',(-10.0514428414942,90.7812499996473,
-3.2659117547607));
#302198=CARTESIAN_POINT('Ctrl Pts',(-10.0514428414942,90.9312499996468,
2.46189346052968E-15));
#302199=CARTESIAN_POINT('Ctrl Pts',(-10.0514428414942,91.0812499996461,
3.26591175476071));
#302200=CARTESIAN_POINT('Ctrl Pts',(-8.13178807675726,91.2312499996455,
5.90808986649102));
#302201=CARTESIAN_POINT('Ctrl Pts',(-6.21213331202028,91.381249999645,8.55026797822134));
#302202=CARTESIAN_POINT('Ctrl Pts',(-3.10606665601017,91.5312499996443,
9.5594902125713));
#302203=CARTESIAN_POINT('Ctrl Pts',(-6.333569765937E-14,91.6812499996438,
10.5687124469213));
#302204=CARTESIAN_POINT('Ctrl Pts',(3.10606665601004,91.8312499996431,9.5594902125713));
#302205=CARTESIAN_POINT('Ctrl Pts',(6.21213331202015,91.9812499996426,8.55026797822134));
#302206=CARTESIAN_POINT('Ctrl Pts',(8.13178807675712,92.131249999642,5.90808986649102));
#302207=CARTESIAN_POINT('Ctrl Pts',(10.0514428414941,92.2812499996414,3.2659117547607));
#302208=CARTESIAN_POINT('Ctrl Pts',(10.0514428414941,92.4312499996408,-1.23094673026484E-15));
#302209=CARTESIAN_POINT('Ctrl Pts',(10.0514428414941,92.5812499996402,-3.26591175476071));
#302210=CARTESIAN_POINT('Ctrl Pts',(8.13178807675712,92.7312499996396,-5.90808986649102));
#302211=CARTESIAN_POINT('Ctrl Pts',(6.21213331202015,92.8812499996389,-8.55026797822134));
#302212=CARTESIAN_POINT('Ctrl Pts',(3.10606665601004,93.0312499996383,-9.5594902125713));
#302213=CARTESIAN_POINT('Ctrl Pts',(-6.67881402690471E-14,93.1812499996377,
-10.5687124469213));
#302214=CARTESIAN_POINT('Ctrl Pts',(-3.10606665601018,93.3312499996371,
-9.5594902125713));
#302215=CARTESIAN_POINT('Ctrl Pts',(-6.21213331202028,93.4812499996365,
-8.55026797822134));
#302216=CARTESIAN_POINT('Ctrl Pts',(-8.13178807675726,93.6312499996359,
-5.90808986649102));
#302217=CARTESIAN_POINT('Ctrl Pts',(-10.0514428414942,93.7812499996353,
-3.2659117547607));
#302218=CARTESIAN_POINT('Ctrl Pts',(-10.0514428414942,93.9312499996347,
2.46189346052968E-15));
#302219=CARTESIAN_POINT('Ctrl Pts',(-10.0514428414942,94.0812499996341,
3.26591175476071));
#302220=CARTESIAN_POINT('Ctrl Pts',(-8.13178807675726,94.2312499996335,
5.90808986649102));
#302221=CARTESIAN_POINT('Ctrl Pts',(-6.21213331202028,94.381249999633,8.55026797822134));
#302222=CARTESIAN_POINT('Ctrl Pts',(-3.10606665601017,94.5312499996324,
9.5594902125713));
#302223=CARTESIAN_POINT('Ctrl Pts',(-6.50634069310318E-14,94.6812499996317,
10.5687124469213));
#302224=CARTESIAN_POINT('Ctrl Pts',(3.10606665601004,94.8312499996312,9.5594902125713));
#302225=CARTESIAN_POINT('Ctrl Pts',(6.21213331202015,94.9812499996306,8.55026797822134));
#302226=CARTESIAN_POINT('Ctrl Pts',(8.13178807675712,95.13124999963,5.90808986649102));
#302227=CARTESIAN_POINT('Ctrl Pts',(10.0514428414941,95.2812499996293,3.2659117547607));
#302228=CARTESIAN_POINT('Ctrl Pts',(10.0514428414941,95.4312499996288,-1.23094673026484E-15));
#302229=CARTESIAN_POINT('Ctrl Pts',(10.0514428414941,95.5812499996282,-3.26591175476071));
#302230=CARTESIAN_POINT('Ctrl Pts',(8.13178807675712,95.7312499996276,-5.90808986649102));
#302231=CARTESIAN_POINT('Ctrl Pts',(6.21213331202015,95.8812499996269,-8.55026797822134));
#302232=CARTESIAN_POINT('Ctrl Pts',(3.10606665601004,96.0312499996264,-9.5594902125713));
#302233=CARTESIAN_POINT('Ctrl Pts',(-6.85158495407089E-14,96.1812499996257,
-10.5687124469213));
#302234=CARTESIAN_POINT('Ctrl Pts',(-3.10606665601018,96.3312499996252,
-9.5594902125713));
#302235=CARTESIAN_POINT('Ctrl Pts',(-6.21213331202028,96.4812499996245,
-8.55026797822134));
#302236=CARTESIAN_POINT('Ctrl Pts',(-8.13178807675726,96.6312499996239,
-5.90808986649102));
#302237=CARTESIAN_POINT('Ctrl Pts',(-10.0514428414942,96.7812499996234,
-3.2659117547607));
#302238=CARTESIAN_POINT('Ctrl Pts',(-10.0514428414942,96.9312499996227,
2.46189346052968E-15));
#302239=CARTESIAN_POINT('Ctrl Pts',(-10.0514428414942,97.0812499996221,
3.26591175476071));
#302240=CARTESIAN_POINT('Ctrl Pts',(-8.13178807675726,97.2312499996215,
5.90808986649102));
#302241=CARTESIAN_POINT('Ctrl Pts',(-6.21213331202028,97.381249999621,8.55026797822134));
#302242=CARTESIAN_POINT('Ctrl Pts',(-3.10606665601017,97.5312499996203,
9.5594902125713));
#302243=CARTESIAN_POINT('Ctrl Pts',(-6.67911162026936E-14,97.6812499996197,
10.5687124469213));
#302244=CARTESIAN_POINT('Ctrl Pts',(3.10606665601004,97.8312499996191,9.5594902125713));
#302245=CARTESIAN_POINT('Ctrl Pts',(6.21213331202015,97.9812499996186,8.55026797822134));
#302246=CARTESIAN_POINT('Ctrl Pts',(8.13178807675712,98.1312499996179,5.90808986649102));
#302247=CARTESIAN_POINT('Ctrl Pts',(10.0514428414941,98.2812499996173,3.2659117547607));
#302248=CARTESIAN_POINT('Ctrl Pts',(10.0514428414941,98.4312499996168,-1.23094673026484E-15));
#302249=CARTESIAN_POINT('Ctrl Pts',(10.0514428414941,98.5812499996162,-3.26591175476071));
#302250=CARTESIAN_POINT('Ctrl Pts',(8.13178807675712,98.7312499996156,-5.90808986649102));
#302251=CARTESIAN_POINT('Ctrl Pts',(6.21213331202015,98.8812499996149,-8.55026797822134));
#302252=CARTESIAN_POINT('Ctrl Pts',(3.10606665601004,99.0312499996143,-9.5594902125713));
#302253=CARTESIAN_POINT('Ctrl Pts',(-7.02435588123707E-14,99.1812499996138,
-10.5687124469213));
#302254=CARTESIAN_POINT('Ctrl Pts',(-3.10606665601018,99.3312499996131,
-9.5594902125713));
#302255=CARTESIAN_POINT('Ctrl Pts',(-6.21213331202028,99.4812499996125,
-8.55026797822134));
#302256=CARTESIAN_POINT('Ctrl Pts',(-8.13178807675726,99.631249999612,-5.90808986649102));
#302257=CARTESIAN_POINT('Ctrl Pts',(-10.0514428414942,99.7812499996113,
-3.2659117547607));
#302258=CARTESIAN_POINT('Ctrl Pts',(-10.0514428414942,99.9312499996108,
2.46189346052968E-15));
#302259=CARTESIAN_POINT('Ctrl Pts',(-10.0514428414942,100.08124999961,3.26591175476071));
#302260=CARTESIAN_POINT('Ctrl Pts',(-8.13178807675726,100.23124999961,5.90808986649102));
#302261=CARTESIAN_POINT('Ctrl Pts',(-6.21213331202028,100.381249999609,
8.55026797822134));
#302262=CARTESIAN_POINT('Ctrl Pts',(-3.10606665601018,100.531249999608,
9.5594902125713));
#302263=CARTESIAN_POINT('Ctrl Pts',(-6.85188254743555E-14,100.681249999608,
10.5687124469213));
#302264=CARTESIAN_POINT('Ctrl Pts',(3.10606665601004,100.831249999607,9.5594902125713));
#302265=CARTESIAN_POINT('Ctrl Pts',(6.21213331202015,100.981249999607,8.55026797822134));
#302266=CARTESIAN_POINT('Ctrl Pts',(8.13178807675712,101.131249999606,5.90808986649102));
#302267=CARTESIAN_POINT('Ctrl Pts',(10.0514428414941,101.281249999605,3.2659117547607));
#302268=CARTESIAN_POINT('Ctrl Pts',(10.0514428414941,101.431249999605,-1.23094673026484E-15));
#302269=CARTESIAN_POINT('Ctrl Pts',(10.0514428414941,101.581249999604,-3.26591175476071));
#302270=CARTESIAN_POINT('Ctrl Pts',(8.13178807675712,101.731249999604,-5.90808986649102));
#302271=CARTESIAN_POINT('Ctrl Pts',(6.21213331202014,101.881249999603,-8.55026797822134));
#302272=CARTESIAN_POINT('Ctrl Pts',(3.10606665601004,102.031249999602,-9.5594902125713));
#302273=CARTESIAN_POINT('Ctrl Pts',(-7.19712680840326E-14,102.181249999602,
-10.5687124469213));
#302274=CARTESIAN_POINT('Ctrl Pts',(-3.10606665601018,102.331249999601,
-9.5594902125713));
#302275=CARTESIAN_POINT('Ctrl Pts',(-6.21213331202029,102.481249999601,
-8.55026797822134));
#302276=CARTESIAN_POINT('Ctrl Pts',(-8.13178807675726,102.6312499996,-5.90808986649102));
#302277=CARTESIAN_POINT('Ctrl Pts',(-10.0514428414942,102.781249999599,
-3.2659117547607));
#302278=CARTESIAN_POINT('Ctrl Pts',(-10.0514428414942,102.931249999599,
2.46189346052968E-15));
#302279=CARTESIAN_POINT('Ctrl Pts',(-10.0514428414942,103.081249999598,
3.26591175476071));
#302280=CARTESIAN_POINT('Ctrl Pts',(-8.13178807675726,103.231249999598,
5.90808986649102));
#302281=CARTESIAN_POINT('Ctrl Pts',(-6.21213331202028,103.381249999597,
8.55026797822134));
#302282=CARTESIAN_POINT('Ctrl Pts',(-3.10606665601018,103.531249999596,
9.5594902125713));
#302283=CARTESIAN_POINT('Ctrl Pts',(-7.02465347460173E-14,103.681249999596,
10.5687124469213));
#302284=CARTESIAN_POINT('Ctrl Pts',(3.10606665601004,103.831249999595,9.5594902125713));
#302285=CARTESIAN_POINT('Ctrl Pts',(6.21213331202015,103.981249999595,8.55026797822134));
#302286=CARTESIAN_POINT('Ctrl Pts',(8.13178807675712,104.131249999594,5.90808986649102));
#302287=CARTESIAN_POINT('Ctrl Pts',(10.0514428414941,104.281249999593,3.2659117547607));
#302288=CARTESIAN_POINT('Ctrl Pts',(10.0514428414941,104.431249999593,-1.23094673026484E-15));
#302289=CARTESIAN_POINT('Ctrl Pts',(10.0514428414941,104.581249999592,-3.26591175476071));
#302290=CARTESIAN_POINT('Ctrl Pts',(8.13178807675712,104.731249999592,-5.90808986649102));
#302291=CARTESIAN_POINT('Ctrl Pts',(6.21213331202014,104.881249999591,-8.55026797822134));
#302292=CARTESIAN_POINT('Ctrl Pts',(3.10606665601003,105.03124999959,-9.5594902125713));
#302293=CARTESIAN_POINT('Ctrl Pts',(-7.36989773556944E-14,105.18124999959,
-10.5687124469213));
#302294=CARTESIAN_POINT('Ctrl Pts',(-3.10606665601018,105.331249999589,
-9.5594902125713));
#302295=CARTESIAN_POINT('Ctrl Pts',(-6.21213331202029,105.481249999589,
-8.55026797822134));
#302296=CARTESIAN_POINT('Ctrl Pts',(-8.13178807675726,105.631249999588,
-5.90808986649102));
#302297=CARTESIAN_POINT('Ctrl Pts',(-10.0514428414942,105.781249999587,
-3.2659117547607));
#302298=CARTESIAN_POINT('Ctrl Pts',(-10.0514428414942,105.931249999587,
2.46189346052968E-15));
#302299=CARTESIAN_POINT('Ctrl Pts',(-10.0514428414942,106.081249999586,
3.26591175476071));
#302300=CARTESIAN_POINT('Ctrl Pts',(-8.13178807675726,106.231249999586,
5.90808986649102));
#302301=CARTESIAN_POINT('Ctrl Pts',(-6.21213331202029,106.381249999585,
8.55026797822134));
#302302=CARTESIAN_POINT('Ctrl Pts',(-3.10606665601018,106.531249999584,
9.5594902125713));
#302303=CARTESIAN_POINT('Ctrl Pts',(-7.19742440176792E-14,106.681249999584,
10.5687124469213));
#302304=CARTESIAN_POINT('Ctrl Pts',(3.10606665601004,106.831249999583,9.5594902125713));
#302305=CARTESIAN_POINT('Ctrl Pts',(6.21213331202014,106.981249999583,8.55026797822134));
#302306=CARTESIAN_POINT('Ctrl Pts',(8.13178807675711,107.131249999582,5.90808986649102));
#302307=CARTESIAN_POINT('Ctrl Pts',(10.0514428414941,107.281249999581,3.2659117547607));
#302308=CARTESIAN_POINT('Ctrl Pts',(10.0514428414941,107.431249999581,-1.23094673026484E-15));
#302309=CARTESIAN_POINT('Ctrl Pts',(10.0514428414941,107.58124999958,-3.26591175476071));
#302310=CARTESIAN_POINT('Ctrl Pts',(8.13178807675711,107.73124999958,-5.90808986649102));
#302311=CARTESIAN_POINT('Ctrl Pts',(6.21213331202014,107.881249999579,-8.55026797822134));
#302312=CARTESIAN_POINT('Ctrl Pts',(3.10606665601003,108.031249999578,-9.5594902125713));
#302313=CARTESIAN_POINT('Ctrl Pts',(-7.54266866273562E-14,108.181249999578,
-10.5687124469213));
#302314=CARTESIAN_POINT('Ctrl Pts',(-3.10606665601018,108.331249999577,
-9.5594902125713));
#302315=CARTESIAN_POINT('Ctrl Pts',(-6.21213331202029,108.481249999577,
-8.55026797822134));
#302316=CARTESIAN_POINT('Ctrl Pts',(-8.13178807675727,108.631249999576,
-5.90808986649102));
#302317=CARTESIAN_POINT('Ctrl Pts',(-10.0514428414942,108.781249999575,
-3.2659117547607));
#302318=CARTESIAN_POINT('Ctrl Pts',(-10.0514428414942,108.931249999575,
2.46189346052968E-15));
#302319=CARTESIAN_POINT('Ctrl Pts',(-10.0514428414942,109.081249999574,
3.26591175476071));
#302320=CARTESIAN_POINT('Ctrl Pts',(-8.13178807675727,109.231249999574,
5.90808986649102));
#302321=CARTESIAN_POINT('Ctrl Pts',(-6.21213331202029,109.381249999573,
8.55026797822134));
#302322=CARTESIAN_POINT('Ctrl Pts',(-3.10606665601018,109.531249999572,
9.5594902125713));
#302323=CARTESIAN_POINT('Ctrl Pts',(-7.3701953289341E-14,109.681249999572,
10.5687124469213));
#302324=CARTESIAN_POINT('Ctrl Pts',(3.10606665601003,109.831249999571,9.5594902125713));
#302325=CARTESIAN_POINT('Ctrl Pts',(6.21213331202014,109.981249999571,8.55026797822134));
#302326=CARTESIAN_POINT('Ctrl Pts',(8.13178807675711,110.13124999957,5.90808986649102));
#302327=CARTESIAN_POINT('Ctrl Pts',(10.0514428414941,110.281249999569,3.2659117547607));
#302328=CARTESIAN_POINT('Ctrl Pts',(10.0514428414941,110.431249999569,-1.23094673026484E-15));
#302329=CARTESIAN_POINT('Ctrl Pts',(10.0514428414941,110.581249999568,-3.26591175476071));
#302330=CARTESIAN_POINT('Ctrl Pts',(8.13178807675711,110.731249999568,-5.90808986649102));
#302331=CARTESIAN_POINT('Ctrl Pts',(6.21213331202014,110.881249999567,-8.55026797822134));
#302332=CARTESIAN_POINT('Ctrl Pts',(3.10606665601003,111.031249999566,-9.5594902125713));
#302333=CARTESIAN_POINT('Ctrl Pts',(-7.71543958990181E-14,111.181249999566,
-10.5687124469213));
#302334=CARTESIAN_POINT('Ctrl Pts',(-3.10606665601019,111.331249999565,
-9.5594902125713));
#302335=CARTESIAN_POINT('Ctrl Pts',(-6.21213331202029,111.481249999565,
-8.55026797822134));
#302336=CARTESIAN_POINT('Ctrl Pts',(-8.13178807675727,111.631249999564,
-5.90808986649102));
#302337=CARTESIAN_POINT('Ctrl Pts',(-10.0514428414942,111.781249999563,
-3.2659117547607));
#302338=CARTESIAN_POINT('Ctrl Pts',(-10.0514428414942,111.931249999563,
2.46189346052968E-15));
#302339=CARTESIAN_POINT('Ctrl Pts',(-10.0514428414942,112.081249999562,
3.26591175476071));
#302340=CARTESIAN_POINT('Ctrl Pts',(-8.13178807675727,112.231249999562,
5.90808986649102));
#302341=CARTESIAN_POINT('Ctrl Pts',(-6.21213331202029,112.381249999561,
8.55026797822134));
#302342=CARTESIAN_POINT('Ctrl Pts',(-3.10606665601018,112.53124999956,9.5594902125713));
#302343=CARTESIAN_POINT('Ctrl Pts',(-7.54296625610028E-14,112.68124999956,
10.5687124469213));
#302344=CARTESIAN_POINT('Ctrl Pts',(3.10606665601003,112.831249999559,9.5594902125713));
#302345=CARTESIAN_POINT('Ctrl Pts',(6.21213331202014,112.981249999559,8.55026797822134));
#302346=CARTESIAN_POINT('Ctrl Pts',(8.13178807675711,113.131249999558,5.90808986649102));
#302347=CARTESIAN_POINT('Ctrl Pts',(10.0514428414941,113.281249999557,3.2659117547607));
#302348=CARTESIAN_POINT('Ctrl Pts',(10.0514428414941,113.431249999557,-1.23094673026484E-15));
#302349=CARTESIAN_POINT('Ctrl Pts',(10.0514428414941,113.581249999556,-3.26591175476071));
#302350=CARTESIAN_POINT('Ctrl Pts',(8.13178807675711,113.731249999556,-5.90808986649102));
#302351=CARTESIAN_POINT('Ctrl Pts',(6.21213331202014,113.881249999555,-8.55026797822134));
#302352=CARTESIAN_POINT('Ctrl Pts',(3.10606665601003,114.031249999554,-9.5594902125713));
#302353=CARTESIAN_POINT('Ctrl Pts',(-7.88821051706799E-14,114.181249999554,
-10.5687124469213));
#302354=CARTESIAN_POINT('Ctrl Pts',(-3.10606665601019,114.331249999553,
-9.5594902125713));
#302355=CARTESIAN_POINT('Ctrl Pts',(-6.2121333120203,114.481249999553,-8.55026797822134));
#302356=CARTESIAN_POINT('Ctrl Pts',(-8.13178807675727,114.631249999552,
-5.90808986649102));
#302357=CARTESIAN_POINT('Ctrl Pts',(-10.0514428414942,114.781249999551,
-3.2659117547607));
#302358=CARTESIAN_POINT('Ctrl Pts',(-10.0514428414942,114.931249999551,
2.46189346052968E-15));
#302359=CARTESIAN_POINT('Ctrl Pts',(-10.0514428414942,115.08124999955,3.26591175476071));
#302360=CARTESIAN_POINT('Ctrl Pts',(-8.13178807675727,115.23124999955,5.90808986649102));
#302361=CARTESIAN_POINT('Ctrl Pts',(-6.21213331202029,115.381249999549,
8.55026797822134));
#302362=CARTESIAN_POINT('Ctrl Pts',(-3.10606665601018,115.531249999548,
9.5594902125713));
#302363=CARTESIAN_POINT('Ctrl Pts',(-7.71573718326647E-14,115.681249999548,
10.5687124469213));
#302364=CARTESIAN_POINT('Ctrl Pts',(3.10606665601003,115.831249999547,9.5594902125713));
#302365=CARTESIAN_POINT('Ctrl Pts',(6.21213331202014,115.981249999547,8.55026797822134));
#302366=CARTESIAN_POINT('Ctrl Pts',(8.13178807675711,116.131249999546,5.90808986649102));
#302367=CARTESIAN_POINT('Ctrl Pts',(10.0514428414941,116.281249999545,3.2659117547607));
#302368=CARTESIAN_POINT('Ctrl Pts',(10.0514428414941,116.431249999545,-1.23094673026484E-15));
#302369=CARTESIAN_POINT('Ctrl Pts',(10.0514428414941,116.581249999544,-3.26591175476071));
#302370=CARTESIAN_POINT('Ctrl Pts',(8.13178807675711,116.731249999544,-5.90808986649102));
#302371=CARTESIAN_POINT('Ctrl Pts',(6.21213331202014,116.881249999543,-8.55026797822134));
#302372=CARTESIAN_POINT('Ctrl Pts',(3.10606665601003,117.031249999542,-9.5594902125713));
#302373=CARTESIAN_POINT('Ctrl Pts',(-8.06098144423418E-14,117.181249999542,
-10.5687124469213));
#302374=CARTESIAN_POINT('Ctrl Pts',(-3.10606665601019,117.331249999541,
-9.5594902125713));
#302375=CARTESIAN_POINT('Ctrl Pts',(-6.2121333120203,117.481249999541,-8.55026797822134));
#302376=CARTESIAN_POINT('Ctrl Pts',(-8.13178807675727,117.63124999954,-5.90808986649102));
#302377=CARTESIAN_POINT('Ctrl Pts',(-10.0514428414942,117.781249999539,
-3.2659117547607));
#302378=CARTESIAN_POINT('Ctrl Pts',(-10.0514428414942,117.931249999539,
2.46189346052968E-15));
#302379=CARTESIAN_POINT('Ctrl Pts',(-10.0514428414942,118.081249999538,
3.26591175476071));
#302380=CARTESIAN_POINT('Ctrl Pts',(-8.13178807675727,118.231249999538,
5.90808986649102));
#302381=CARTESIAN_POINT('Ctrl Pts',(-6.2121333120203,118.381249999537,8.55026797822134));
#302382=CARTESIAN_POINT('Ctrl Pts',(-3.10606665601019,118.531249999536,
9.5594902125713));
#302383=CARTESIAN_POINT('Ctrl Pts',(-7.88850811043265E-14,118.681249999536,
10.5687124469213));
#302384=CARTESIAN_POINT('Ctrl Pts',(3.10606665601003,118.831249999535,9.5594902125713));
#302385=CARTESIAN_POINT('Ctrl Pts',(6.21213331202014,118.981249999535,8.55026797822134));
#302386=CARTESIAN_POINT('Ctrl Pts',(8.13178807675711,119.131249999534,5.90808986649102));
#302387=CARTESIAN_POINT('Ctrl Pts',(10.0514428414941,119.281249999533,3.2659117547607));
#302388=CARTESIAN_POINT('Ctrl Pts',(10.0514428414941,119.431249999533,-1.23094673026484E-15));
#302389=CARTESIAN_POINT('Ctrl Pts',(10.0514428414941,119.581249999532,-3.26591175476071));
#302390=CARTESIAN_POINT('Ctrl Pts',(8.13178807675711,119.731249999532,-5.90808986649102));
#302391=CARTESIAN_POINT('Ctrl Pts',(6.21213331202013,119.881249999531,-8.55026797822134));
#302392=CARTESIAN_POINT('Ctrl Pts',(3.10606665601003,120.03124999953,-9.5594902125713));
#302393=CARTESIAN_POINT('Ctrl Pts',(-8.23375237140036E-14,120.18124999953,
-10.5687124469213));
#302394=CARTESIAN_POINT('Ctrl Pts',(-3.10606665601019,120.331249999529,
-9.5594902125713));
#302395=CARTESIAN_POINT('Ctrl Pts',(-6.2121333120203,120.481249999529,-8.55026797822134));
#302396=CARTESIAN_POINT('Ctrl Pts',(-8.13178807675727,120.631249999528,
-5.90808986649102));
#302397=CARTESIAN_POINT('Ctrl Pts',(-10.0514428414943,120.781249999527,
-3.2659117547607));
#302398=CARTESIAN_POINT('Ctrl Pts',(-10.0514428414943,120.931249999527,
2.46189346052968E-15));
#302399=CARTESIAN_POINT('Ctrl Pts',(-10.0514428414943,121.081249999526,
3.26591175476071));
#302400=CARTESIAN_POINT('Ctrl Pts',(-8.13178807675727,121.231249999526,
5.90808986649102));
#302401=CARTESIAN_POINT('Ctrl Pts',(-6.2121333120203,121.381249999525,8.55026797822134));
#302402=CARTESIAN_POINT('Ctrl Pts',(-3.10606665601019,121.531249999524,
9.5594902125713));
#302403=CARTESIAN_POINT('Ctrl Pts',(-8.06127903759884E-14,121.681249999524,
10.5687124469213));
#302404=CARTESIAN_POINT('Ctrl Pts',(3.10606665601003,121.831249999523,9.5594902125713));
#302405=CARTESIAN_POINT('Ctrl Pts',(6.21213331202014,121.981249999523,8.55026797822134));
#302406=CARTESIAN_POINT('Ctrl Pts',(8.13178807675711,122.131249999522,5.90808986649102));
#302407=CARTESIAN_POINT('Ctrl Pts',(10.0514428414941,122.281249999521,3.2659117547607));
#302408=CARTESIAN_POINT('Ctrl Pts',(10.0514428414941,122.431249999521,-1.23094673026484E-15));
#302409=CARTESIAN_POINT('Ctrl Pts',(10.0514428414941,122.58124999952,-3.26591175476071));
#302410=CARTESIAN_POINT('Ctrl Pts',(8.13178807675711,122.73124999952,-5.90808986649102));
#302411=CARTESIAN_POINT('Ctrl Pts',(6.21213331202013,122.881249999519,-8.55026797822134));
#302412=CARTESIAN_POINT('Ctrl Pts',(3.10606665601002,123.031249999518,-9.5594902125713));
#302413=CARTESIAN_POINT('Ctrl Pts',(-8.40652329856655E-14,123.181249999518,
-10.5687124469213));
#302414=CARTESIAN_POINT('Ctrl Pts',(-3.10606665601019,123.331249999517,
-9.5594902125713));
#302415=CARTESIAN_POINT('Ctrl Pts',(-6.2121333120203,123.481249999517,-8.55026797822134));
#302416=CARTESIAN_POINT('Ctrl Pts',(-8.13178807675727,123.631249999516,
-5.90808986649102));
#302417=CARTESIAN_POINT('Ctrl Pts',(-10.0514428414943,123.781249999515,
-3.2659117547607));
#302418=CARTESIAN_POINT('Ctrl Pts',(-10.0514428414943,123.931249999515,
2.46189346052968E-15));
#302419=CARTESIAN_POINT('Ctrl Pts',(-10.0514428414943,124.081249999514,
3.26591175476071));
#302420=CARTESIAN_POINT('Ctrl Pts',(-8.13178807675727,124.231249999514,
5.90808986649102));
#302421=CARTESIAN_POINT('Ctrl Pts',(-6.2121333120203,124.381249999513,8.55026797822134));
#302422=CARTESIAN_POINT('Ctrl Pts',(-3.10606665601019,124.531249999512,
9.5594902125713));
#302423=CARTESIAN_POINT('Ctrl Pts',(-8.23404996476502E-14,124.681249999512,
10.5687124469213));
#302424=CARTESIAN_POINT('Ctrl Pts',(3.10606665601002,124.831249999511,9.5594902125713));
#302425=CARTESIAN_POINT('Ctrl Pts',(6.21213331202013,124.981249999511,8.55026797822134));
#302426=CARTESIAN_POINT('Ctrl Pts',(8.13178807675711,125.13124999951,5.90808986649102));
#302427=CARTESIAN_POINT('Ctrl Pts',(10.0514428414941,125.281249999509,3.2659117547607));
#302428=CARTESIAN_POINT('Ctrl Pts',(10.0514428414941,125.431249999509,-1.23094673026484E-15));
#302429=CARTESIAN_POINT('Ctrl Pts',(10.0514428414941,125.581249999508,-3.26591175476071));
#302430=CARTESIAN_POINT('Ctrl Pts',(8.13178807675711,125.731249999508,-5.90808986649102));
#302431=CARTESIAN_POINT('Ctrl Pts',(6.21213331202013,125.881249999507,-8.55026797822134));
#302432=CARTESIAN_POINT('Ctrl Pts',(3.10606665601002,126.031249999506,-9.5594902125713));
#302433=CARTESIAN_POINT('Ctrl Pts',(-8.57929422573273E-14,126.181249999506,
-10.5687124469213));
#302434=CARTESIAN_POINT('Ctrl Pts',(-3.10606665601019,126.331249999505,
-9.5594902125713));
#302435=CARTESIAN_POINT('Ctrl Pts',(-6.2121333120203,126.481249999505,-8.55026797822134));
#302436=CARTESIAN_POINT('Ctrl Pts',(-8.13178807675728,126.631249999504,
-5.90808986649102));
#302437=CARTESIAN_POINT('Ctrl Pts',(-10.0514428414943,126.781249999503,
-3.2659117547607));
#302438=CARTESIAN_POINT('Ctrl Pts',(-10.0514428414943,126.931249999503,
2.46189346052968E-15));
#302439=CARTESIAN_POINT('Ctrl Pts',(-10.0514428414943,127.081249999502,
3.26591175476071));
#302440=CARTESIAN_POINT('Ctrl Pts',(-8.13178807675728,127.231249999502,
5.90808986649102));
#302441=CARTESIAN_POINT('Ctrl Pts',(-6.2121333120203,127.381249999501,8.55026797822134));
#302442=CARTESIAN_POINT('Ctrl Pts',(-3.10606665601019,127.5312499995,9.5594902125713));
#302443=CARTESIAN_POINT('Ctrl Pts',(-8.4068208919312E-14,127.6812499995,
10.5687124469213));
#302444=CARTESIAN_POINT('Ctrl Pts',(3.10606665601002,127.831249999499,9.5594902125713));
#302445=CARTESIAN_POINT('Ctrl Pts',(6.21213331202013,127.981249999499,8.55026797822134));
#302446=CARTESIAN_POINT('Ctrl Pts',(8.1317880767571,128.131249999498,5.90808986649102));
#302447=CARTESIAN_POINT('Ctrl Pts',(10.0514428414941,128.281249999497,3.2659117547607));
#302448=CARTESIAN_POINT('Ctrl Pts',(10.0514428414941,128.431249999497,-1.23094673026484E-15));
#302449=CARTESIAN_POINT('Ctrl Pts',(10.0514428414941,128.581249999496,-3.26591175476071));
#302450=CARTESIAN_POINT('Ctrl Pts',(8.1317880767571,128.731249999496,-5.90808986649102));
#302451=CARTESIAN_POINT('Ctrl Pts',(6.21213331202013,128.881249999495,-8.55026797822134));
#302452=CARTESIAN_POINT('Ctrl Pts',(3.10606665601002,129.031249999494,-9.5594902125713));
#302453=CARTESIAN_POINT('Ctrl Pts',(-8.75206515289892E-14,129.181249999494,
-10.5687124469213));
#302454=CARTESIAN_POINT('Ctrl Pts',(-3.1060666560102,129.331249999493,-9.5594902125713));
#302455=CARTESIAN_POINT('Ctrl Pts',(-6.2121333120203,129.481249999493,-8.55026797822134));
#302456=CARTESIAN_POINT('Ctrl Pts',(-8.13178807675728,129.631249999492,
-5.90808986649102));
#302457=CARTESIAN_POINT('Ctrl Pts',(-10.0514428414943,129.781249999491,
-3.2659117547607));
#302458=CARTESIAN_POINT('Ctrl Pts',(-10.0514428414943,129.931249999491,
2.46189346052968E-15));
#302459=CARTESIAN_POINT('Ctrl Pts',(-10.0514428414943,130.08124999949,3.26591175476071));
#302460=CARTESIAN_POINT('Ctrl Pts',(-8.13178807675728,130.23124999949,5.90808986649102));
#302461=CARTESIAN_POINT('Ctrl Pts',(-6.2121333120203,130.381249999489,8.55026797822134));
#302462=CARTESIAN_POINT('Ctrl Pts',(-3.10606665601019,130.531249999488,
9.5594902125713));
#302463=CARTESIAN_POINT('Ctrl Pts',(-8.57959181909739E-14,130.681249999488,
10.5687124469213));
#302464=CARTESIAN_POINT('Ctrl Pts',(3.10606665601002,130.831249999487,9.5594902125713));
#302465=CARTESIAN_POINT('Ctrl Pts',(6.21213331202013,130.981249999487,8.55026797822134));
#302466=CARTESIAN_POINT('Ctrl Pts',(8.1317880767571,131.131249999486,5.90808986649102));
#302467=CARTESIAN_POINT('Ctrl Pts',(10.0514428414941,131.281249999485,3.2659117547607));
#302468=CARTESIAN_POINT('Ctrl Pts',(10.0514428414941,131.431249999485,-1.23094673026484E-15));
#302469=CARTESIAN_POINT('Ctrl Pts',(10.0514428414941,131.581249999484,-3.26591175476071));
#302470=CARTESIAN_POINT('Ctrl Pts',(8.1317880767571,131.731249999484,-5.90808986649102));
#302471=CARTESIAN_POINT('Ctrl Pts',(6.21213331202012,131.881249999483,-8.55026797822134));
#302472=CARTESIAN_POINT('Ctrl Pts',(3.10606665601002,132.031249999482,-9.5594902125713));
#302473=CARTESIAN_POINT('Ctrl Pts',(-8.9248360800651E-14,132.181249999482,
-10.5687124469213));
#302474=CARTESIAN_POINT('Ctrl Pts',(-3.1060666560102,132.331249999481,-9.5594902125713));
#302475=CARTESIAN_POINT('Ctrl Pts',(-6.2121333120203,132.48124999948,-8.55026797822134));
#302476=CARTESIAN_POINT('Ctrl Pts',(-8.13178807675728,132.63124999948,-5.90808986649102));
#302477=CARTESIAN_POINT('Ctrl Pts',(-10.0514428414943,132.781249999479,
-3.2659117547607));
#302478=CARTESIAN_POINT('Ctrl Pts',(-10.0514428414943,132.931249999479,
2.46189346052968E-15));
#302479=CARTESIAN_POINT('Ctrl Pts',(-10.0514428414943,133.081249999478,
3.26591175476071));
#302480=CARTESIAN_POINT('Ctrl Pts',(-8.13178807675728,133.231249999478,
5.90808986649102));
#302481=CARTESIAN_POINT('Ctrl Pts',(-6.2121333120203,133.381249999477,8.55026797822134));
#302482=CARTESIAN_POINT('Ctrl Pts',(-3.1060666560102,133.531249999476,9.5594902125713));
#302483=CARTESIAN_POINT('Ctrl Pts',(-8.75236274626357E-14,133.681249999476,
10.5687124469213));
#302484=CARTESIAN_POINT('Ctrl Pts',(3.10606665601002,133.831249999475,9.5594902125713));
#302485=CARTESIAN_POINT('Ctrl Pts',(6.21213331202013,133.981249999475,8.55026797822134));
#302486=CARTESIAN_POINT('Ctrl Pts',(8.1317880767571,134.131249999474,5.90808986649102));
#302487=CARTESIAN_POINT('Ctrl Pts',(10.0514428414941,134.281249999473,3.2659117547607));
#302488=CARTESIAN_POINT('Ctrl Pts',(10.0514428414941,134.431249999473,-1.23094673026484E-15));
#302489=CARTESIAN_POINT('Ctrl Pts',(10.0514428414941,134.581249999472,-3.26591175476071));
#302490=CARTESIAN_POINT('Ctrl Pts',(8.1317880767571,134.731249999472,-5.90808986649102));
#302491=CARTESIAN_POINT('Ctrl Pts',(6.21213331202012,134.881249999471,-8.55026797822134));
#302492=CARTESIAN_POINT('Ctrl Pts',(3.10606665601002,135.03124999947,-9.5594902125713));
#302493=CARTESIAN_POINT('Ctrl Pts',(-9.09760700723128E-14,135.18124999947,
-10.5687124469213));
#302494=CARTESIAN_POINT('Ctrl Pts',(-3.1060666560102,135.331249999469,-9.5594902125713));
#302495=CARTESIAN_POINT('Ctrl Pts',(-6.21213331202031,135.481249999469,
-8.55026797822134));
#302496=CARTESIAN_POINT('Ctrl Pts',(-8.13178807675728,135.631249999468,
-5.90808986649102));
#302497=CARTESIAN_POINT('Ctrl Pts',(-10.0514428414943,135.781249999467,
-3.2659117547607));
#302498=CARTESIAN_POINT('Ctrl Pts',(-10.0514428414943,135.931249999467,
2.46189346052968E-15));
#302499=CARTESIAN_POINT('Ctrl Pts',(-10.0514428414943,136.081249999466,
3.26591175476071));
#302500=CARTESIAN_POINT('Ctrl Pts',(-8.13178807675728,136.231249999466,
5.90808986649102));
#302501=CARTESIAN_POINT('Ctrl Pts',(-6.2121333120203,136.381249999465,8.55026797822134));
#302502=CARTESIAN_POINT('Ctrl Pts',(-3.1060666560102,136.531249999464,9.5594902125713));
#302503=CARTESIAN_POINT('Ctrl Pts',(-8.92513367342975E-14,136.681249999464,
10.5687124469213));
#302504=CARTESIAN_POINT('Ctrl Pts',(3.10606665601002,136.831249999463,9.5594902125713));
#302505=CARTESIAN_POINT('Ctrl Pts',(6.21213331202012,136.981249999463,8.55026797822134));
#302506=CARTESIAN_POINT('Ctrl Pts',(8.1317880767571,137.131249999462,5.90808986649102));
#302507=CARTESIAN_POINT('Ctrl Pts',(10.0514428414941,137.281249999461,3.2659117547607));
#302508=CARTESIAN_POINT('Ctrl Pts',(10.0514428414941,137.431249999461,-1.23094673026484E-15));
#302509=CARTESIAN_POINT('Ctrl Pts',(10.0514428414941,137.58124999946,-3.26591175476071));
#302510=CARTESIAN_POINT('Ctrl Pts',(8.1317880767571,137.73124999946,-5.90808986649102));
#302511=CARTESIAN_POINT('Ctrl Pts',(6.21213331202012,137.881249999459,-8.55026797822134));
#302512=CARTESIAN_POINT('Ctrl Pts',(3.10606665601002,138.031249999458,-9.5594902125713));
#302513=CARTESIAN_POINT('Ctrl Pts',(-9.27037793439746E-14,138.181249999458,
-10.5687124469213));
#302514=CARTESIAN_POINT('Ctrl Pts',(-3.1060666560102,138.331249999457,-9.5594902125713));
#302515=CARTESIAN_POINT('Ctrl Pts',(-6.21213331202031,138.481249999456,
-8.55026797822134));
#302516=CARTESIAN_POINT('Ctrl Pts',(-8.13178807675728,138.631249999456,
-5.90808986649102));
#302517=CARTESIAN_POINT('Ctrl Pts',(-10.0514428414943,138.781249999455,
-3.2659117547607));
#302518=CARTESIAN_POINT('Ctrl Pts',(-10.0514428414943,138.931249999455,
2.46189346052968E-15));
#302519=CARTESIAN_POINT('Ctrl Pts',(-10.0514428414943,139.081249999454,
3.26591175476071));
#302520=CARTESIAN_POINT('Ctrl Pts',(-8.13178807675728,139.231249999454,
5.90808986649102));
#302521=CARTESIAN_POINT('Ctrl Pts',(-6.21213331202031,139.381249999453,
8.55026797822134));
#302522=CARTESIAN_POINT('Ctrl Pts',(-3.1060666560102,139.531249999452,9.5594902125713));
#302523=CARTESIAN_POINT('Ctrl Pts',(-9.09790460059594E-14,139.681249999452,
10.5687124469213));
#302524=CARTESIAN_POINT('Ctrl Pts',(3.10606665601002,139.831249999451,9.5594902125713));
#302525=CARTESIAN_POINT('Ctrl Pts',(6.21213331202012,139.981249999451,8.55026797822134));
#302526=CARTESIAN_POINT('Ctrl Pts',(8.1317880767571,140.13124999945,5.90808986649102));
#302527=CARTESIAN_POINT('Ctrl Pts',(10.0514428414941,140.281249999449,3.2659117547607));
#302528=CARTESIAN_POINT('Ctrl Pts',(10.0514428414941,140.431249999449,-1.23094673026484E-15));
#302529=CARTESIAN_POINT('Ctrl Pts',(10.0514428414941,140.581249999448,-3.26591175476071));
#302530=CARTESIAN_POINT('Ctrl Pts',(8.1317880767571,140.731249999448,-5.90808986649102));
#302531=CARTESIAN_POINT('Ctrl Pts',(6.21213331202012,140.881249999447,-8.55026797822134));
#302532=CARTESIAN_POINT('Ctrl Pts',(3.10606665601001,141.031249999446,-9.5594902125713));
#302533=CARTESIAN_POINT('Ctrl Pts',(-9.44314886156365E-14,141.181249999446,
-10.5687124469213));
#302534=CARTESIAN_POINT('Ctrl Pts',(-3.1060666560102,141.331249999445,-9.5594902125713));
#302535=CARTESIAN_POINT('Ctrl Pts',(-6.21213331202031,141.481249999445,
-8.55026797822134));
#302536=CARTESIAN_POINT('Ctrl Pts',(-8.13178807675729,141.631249999444,
-5.90808986649102));
#302537=CARTESIAN_POINT('Ctrl Pts',(-10.0514428414943,141.781249999443,
-3.2659117547607));
#302538=CARTESIAN_POINT('Ctrl Pts',(-10.0514428414943,141.931249999443,
2.46189346052968E-15));
#302539=CARTESIAN_POINT('Ctrl Pts',(-10.0514428414943,142.081249999442,
3.26591175476071));
#302540=CARTESIAN_POINT('Ctrl Pts',(-8.13178807675729,142.231249999442,
5.90808986649102));
#302541=CARTESIAN_POINT('Ctrl Pts',(-6.21213331202031,142.381249999441,
8.55026797822134));
#302542=CARTESIAN_POINT('Ctrl Pts',(-3.1060666560102,142.53124999944,9.5594902125713));
#302543=CARTESIAN_POINT('Ctrl Pts',(-9.27067552776212E-14,142.68124999944,
10.5687124469213));
#302544=CARTESIAN_POINT('Ctrl Pts',(3.10606665601001,142.831249999439,9.5594902125713));
#302545=CARTESIAN_POINT('Ctrl Pts',(6.21213331202012,142.981249999439,8.55026797822134));
#302546=CARTESIAN_POINT('Ctrl Pts',(8.1317880767571,143.131249999438,5.90808986649102));
#302547=CARTESIAN_POINT('Ctrl Pts',(10.0514428414941,143.281249999437,3.2659117547607));
#302548=CARTESIAN_POINT('Ctrl Pts',(10.0514428414941,143.431249999437,-1.23094673026484E-15));
#302549=CARTESIAN_POINT('Ctrl Pts',(10.0514428414941,143.581249999436,-3.26591175476071));
#302550=CARTESIAN_POINT('Ctrl Pts',(8.1317880767571,143.731249999436,-5.90808986649102));
#302551=CARTESIAN_POINT('Ctrl Pts',(6.21213331202012,143.881249999435,-8.55026797822134));
#302552=CARTESIAN_POINT('Ctrl Pts',(3.10606665601001,144.031249999434,-9.5594902125713));
#302553=CARTESIAN_POINT('Ctrl Pts',(-9.61591978872984E-14,144.181249999434,
-10.5687124469213));
#302554=CARTESIAN_POINT('Ctrl Pts',(-3.1060666560102,144.331249999433,-9.5594902125713));
#302555=CARTESIAN_POINT('Ctrl Pts',(-6.21213331202031,144.481249999432,
-8.55026797822134));
#302556=CARTESIAN_POINT('Ctrl Pts',(-8.13178807675729,144.631249999432,
-5.90808986649102));
#302557=CARTESIAN_POINT('Ctrl Pts',(-10.0514428414943,144.781249999431,
-3.2659117547607));
#302558=CARTESIAN_POINT('Ctrl Pts',(-10.0514428414943,144.931249999431,
2.46189346052968E-15));
#302559=CARTESIAN_POINT('Ctrl Pts',(-10.0514428414943,145.08124999943,3.26591175476071));
#302560=CARTESIAN_POINT('Ctrl Pts',(-8.13178807675729,145.23124999943,5.90808986649102));
#302561=CARTESIAN_POINT('Ctrl Pts',(-6.21213331202031,145.381249999429,
8.55026797822134));
#302562=CARTESIAN_POINT('Ctrl Pts',(-3.1060666560102,145.531249999428,9.5594902125713));
#302563=CARTESIAN_POINT('Ctrl Pts',(-9.44344645492831E-14,145.681249999428,
10.5687124469213));
#302564=CARTESIAN_POINT('Ctrl Pts',(3.10606665601001,145.831249999427,9.5594902125713));
#302565=CARTESIAN_POINT('Ctrl Pts',(6.21213331202012,145.981249999427,8.55026797822134));
#302566=CARTESIAN_POINT('Ctrl Pts',(8.13178807675709,146.131249999426,5.90808986649102));
#302567=CARTESIAN_POINT('Ctrl Pts',(10.0514428414941,146.281249999425,3.2659117547607));
#302568=CARTESIAN_POINT('Ctrl Pts',(10.0514428414941,146.431249999425,-1.23094673026484E-15));
#302569=CARTESIAN_POINT('Ctrl Pts',(10.0514428414941,146.581249999424,-3.26591175476071));
#302570=CARTESIAN_POINT('Ctrl Pts',(8.13178807675709,146.731249999424,-5.90808986649102));
#302571=CARTESIAN_POINT('Ctrl Pts',(6.21213331202012,146.881249999423,-8.55026797822134));
#302572=CARTESIAN_POINT('Ctrl Pts',(3.10606665601001,147.031249999422,-9.5594902125713));
#302573=CARTESIAN_POINT('Ctrl Pts',(-9.78869071589602E-14,147.181249999422,
-10.5687124469213));
#302574=CARTESIAN_POINT('Ctrl Pts',(-3.10606665601021,147.331249999421,
-9.5594902125713));
#302575=CARTESIAN_POINT('Ctrl Pts',(-6.21213331202032,147.481249999421,
-8.55026797822134));
#302576=CARTESIAN_POINT('Ctrl Pts',(-8.13178807675729,147.63124999942,-5.90808986649102));
#302577=CARTESIAN_POINT('Ctrl Pts',(-10.0514428414943,147.781249999419,
-3.2659117547607));
#302578=CARTESIAN_POINT('Ctrl Pts',(-10.0514428414943,147.931249999419,
2.46189346052968E-15));
#302579=CARTESIAN_POINT('Ctrl Pts',(-10.0514428414943,148.081249999418,
3.26591175476071));
#302580=CARTESIAN_POINT('Ctrl Pts',(-8.13178807675729,148.231249999418,
5.90808986649102));
#302581=CARTESIAN_POINT('Ctrl Pts',(-6.21213331202031,148.381249999417,
8.55026797822134));
#302582=CARTESIAN_POINT('Ctrl Pts',(-3.1060666560102,148.531249999416,9.5594902125713));
#302583=CARTESIAN_POINT('Ctrl Pts',(-9.61621738209449E-14,148.681249999416,
10.5687124469213));
#302584=CARTESIAN_POINT('Ctrl Pts',(3.10606665601001,148.831249999415,9.5594902125713));
#302585=CARTESIAN_POINT('Ctrl Pts',(6.21213331202012,148.981249999415,8.55026797822134));
#302586=CARTESIAN_POINT('Ctrl Pts',(8.13178807675709,149.131249999414,5.90808986649102));
#302587=CARTESIAN_POINT('Ctrl Pts',(10.0514428414941,149.281249999413,3.2659117547607));
#302588=CARTESIAN_POINT('Ctrl Pts',(10.0514428414941,149.431249999413,-1.23094673026484E-15));
#302589=CARTESIAN_POINT('Ctrl Pts',(10.0514428414941,149.581249999412,-3.26591175476071));
#302590=CARTESIAN_POINT('Ctrl Pts',(8.13178807675709,149.731249999412,-5.90808986649102));
#302591=CARTESIAN_POINT('Ctrl Pts',(6.21213331202012,149.881249999411,-8.55026797822134));
#302592=CARTESIAN_POINT('Ctrl Pts',(3.10606665601001,150.03124999941,-9.5594902125713));
#302593=CARTESIAN_POINT('Ctrl Pts',(-9.9614616430622E-14,150.18124999941,
-10.5687124469213));
#302594=CARTESIAN_POINT('Ctrl Pts',(-3.10606665601021,150.331249999409,
-9.5594902125713));
#302595=CARTESIAN_POINT('Ctrl Pts',(-6.21213331202032,150.481249999409,
-8.55026797822134));
#302596=CARTESIAN_POINT('Ctrl Pts',(-8.13178807675729,150.631249999408,
-5.90808986649102));
#302597=CARTESIAN_POINT('Ctrl Pts',(-10.0514428414943,150.781249999407,
-3.2659117547607));
#302598=CARTESIAN_POINT('Ctrl Pts',(-10.0514428414943,150.931249999407,
2.46189346052968E-15));
#302599=CARTESIAN_POINT('Ctrl Pts',(-10.0514428414943,151.081249999406,
3.26591175476071));
#302600=CARTESIAN_POINT('Ctrl Pts',(-8.13178807675729,151.231249999406,
5.90808986649102));
#302601=CARTESIAN_POINT('Ctrl Pts',(-6.21213331202032,151.381249999405,
8.55026797822134));
#302602=CARTESIAN_POINT('Ctrl Pts',(-3.10606665601021,151.531249999404,
9.5594902125713));
#302603=CARTESIAN_POINT('Ctrl Pts',(-9.78898830926068E-14,151.681249999404,
10.5687124469213));
#302604=CARTESIAN_POINT('Ctrl Pts',(3.10606665601001,151.831249999403,9.5594902125713));
#302605=CARTESIAN_POINT('Ctrl Pts',(6.21213331202012,151.981249999403,8.55026797822134));
#302606=CARTESIAN_POINT('Ctrl Pts',(8.13178807675709,152.131249999402,5.90808986649102));
#302607=CARTESIAN_POINT('Ctrl Pts',(10.0514428414941,152.281249999401,3.2659117547607));
#302608=CARTESIAN_POINT('Ctrl Pts',(10.0514428414941,152.431249999401,-1.23094673026484E-15));
#302609=CARTESIAN_POINT('Ctrl Pts',(10.0514428414941,152.5812499994,-3.26591175476071));
#302610=CARTESIAN_POINT('Ctrl Pts',(8.13178807675709,152.7312499994,-5.90808986649102));
#302611=CARTESIAN_POINT('Ctrl Pts',(6.21213331202012,152.881249999399,-8.55026797822134));
#302612=CARTESIAN_POINT('Ctrl Pts',(3.10606665601001,153.031249999398,-9.5594902125713));
#302613=CARTESIAN_POINT('Ctrl Pts',(-1.01342325702284E-13,153.181249999398,
-10.5687124469213));
#302614=CARTESIAN_POINT('Ctrl Pts',(-3.10606665601021,153.331249999397,
-9.5594902125713));
#302615=CARTESIAN_POINT('Ctrl Pts',(10.0514428414941,59.4312499997728,-1.23094673026484E-15));
#302616=CARTESIAN_POINT('Ctrl Pts',(10.0514428414941,59.5812499997722,-3.26591175476071));
#302617=CARTESIAN_POINT('Ctrl Pts',(8.13178807675714,59.7312499997716,-5.90808986649102));
#302618=CARTESIAN_POINT('Ctrl Pts',(6.21213331202017,59.881249999771,-8.55026797822134));
#302619=CARTESIAN_POINT('Ctrl Pts',(3.10606665601006,60.0312499997704,-9.5594902125713));
#302620=CARTESIAN_POINT('Ctrl Pts',(1.41674609610483,60.1128316630275,-10.1083837357357));
#302621=CARTESIAN_POINT('Ctrl Pts',(-0.358381257737887,60.1985571585059,
-10.0450518201713));
#302622=CARTESIAN_POINT('Origin',(-3.77475828372553E-14,-1.881249999982,
2.68644078414671E-15));
#302623=CARTESIAN_POINT('Origin',(0.,-21.2328125,0.));
#302624=CARTESIAN_POINT('',(-1.45809509523482E-16,-21.2328125,1.190625));
#302625=CARTESIAN_POINT('Origin',(0.,-21.2328125,0.));
#302626=CARTESIAN_POINT('',(-1.45809509523482E-16,-21.43125,1.190625));
#302627=CARTESIAN_POINT('',(-1.45809509523482E-16,-21.2328125,1.190625));
#302628=CARTESIAN_POINT('Origin',(0.,-21.43125,0.));
#302629=CARTESIAN_POINT('Origin',(-22.4506403026729,-21.2328125,22.4506403026729));
#302630=CARTESIAN_POINT('',(-22.4506403026729,-21.2328125,23.6412653026729));
#302631=CARTESIAN_POINT('Origin',(-22.4506403026729,-21.2328125,22.4506403026729));
#302632=CARTESIAN_POINT('',(-22.4506403026729,-21.43125,23.6412653026729));
#302633=CARTESIAN_POINT('',(-22.4506403026729,-21.2328125,23.6412653026729));
#302634=CARTESIAN_POINT('Origin',(-22.4506403026729,-21.43125,22.4506403026729));
#302635=CARTESIAN_POINT('Origin',(-31.75,-21.2328125,-6.93889390390723E-15));
#302636=CARTESIAN_POINT('',(-31.75,-21.2328125,1.19062499999999));
#302637=CARTESIAN_POINT('Origin',(-31.75,-21.2328125,-6.93889390390723E-15));
#302638=CARTESIAN_POINT('',(-31.75,-21.43125,1.19062499999999));
#302639=CARTESIAN_POINT('',(-31.75,-21.2328125,1.19062499999999));
#302640=CARTESIAN_POINT('Origin',(-31.75,-21.43125,-6.93889390390723E-15));
#302641=CARTESIAN_POINT('Origin',(-22.4506403026729,-21.2328125,-22.4506403026729));
#302642=CARTESIAN_POINT('',(-22.4506403026729,-21.2328125,-21.2600153026729));
#302643=CARTESIAN_POINT('Origin',(-22.4506403026729,-21.2328125,-22.4506403026729));
#302644=CARTESIAN_POINT('',(-22.4506403026729,-21.43125,-21.2600153026729));
#302645=CARTESIAN_POINT('',(-22.4506403026729,-21.2328125,-21.2600153026729));
#302646=CARTESIAN_POINT('Origin',(-22.4506403026729,-21.43125,-22.4506403026729));
#302647=CARTESIAN_POINT('Origin',(3.46944695195361E-15,-21.2328125,-31.75));
#302648=CARTESIAN_POINT('',(3.32363744243013E-15,-21.2328125,-30.559375));
#302649=CARTESIAN_POINT('Origin',(3.46944695195361E-15,-21.2328125,-31.75));
#302650=CARTESIAN_POINT('',(3.32363744243013E-15,-21.43125,-30.559375));
#302651=CARTESIAN_POINT('',(3.32363744243013E-15,-21.2328125,-30.559375));
#302652=CARTESIAN_POINT('Origin',(3.46944695195361E-15,-21.43125,-31.75));
#302653=CARTESIAN_POINT('Origin',(22.4506403026729,-21.2328125,-22.4506403026729));
#302654=CARTESIAN_POINT('',(22.4506403026729,-21.2328125,-21.2600153026729));
#302655=CARTESIAN_POINT('Origin',(22.4506403026729,-21.2328125,-22.4506403026729));
#302656=CARTESIAN_POINT('',(22.4506403026729,-21.43125,-21.2600153026729));
#302657=CARTESIAN_POINT('',(22.4506403026729,-21.2328125,-21.2600153026729));
#302658=CARTESIAN_POINT('Origin',(22.4506403026729,-21.43125,-22.4506403026729));
#302659=CARTESIAN_POINT('Origin',(31.75,-21.2328125,1.73472347597681E-15));
#302660=CARTESIAN_POINT('',(31.75,-21.2328125,1.190625));
#302661=CARTESIAN_POINT('Origin',(31.75,-21.2328125,1.73472347597681E-15));
#302662=CARTESIAN_POINT('',(31.75,-21.43125,1.190625));
#302663=CARTESIAN_POINT('',(31.75,-21.2328125,1.190625));
#302664=CARTESIAN_POINT('Origin',(31.75,-21.43125,1.73472347597681E-15));
#302665=CARTESIAN_POINT('Origin',(22.4506403026729,-21.2328125,22.4506403026729));
#302666=CARTESIAN_POINT('',(22.4506403026729,-21.2328125,23.6412653026729));
#302667=CARTESIAN_POINT('Origin',(22.4506403026729,-21.2328125,22.4506403026729));
#302668=CARTESIAN_POINT('',(22.4506403026729,-21.43125,23.6412653026729));
#302669=CARTESIAN_POINT('',(22.4506403026729,-21.2328125,23.6412653026729));
#302670=CARTESIAN_POINT('Origin',(22.4506403026729,-21.43125,22.4506403026729));
#302671=CARTESIAN_POINT('Origin',(0.,-21.2328125,31.75));
#302672=CARTESIAN_POINT('',(-1.45809509523482E-16,-21.2328125,32.940625));
#302673=CARTESIAN_POINT('Origin',(0.,-21.2328125,31.75));
#302674=CARTESIAN_POINT('',(-1.45809509523482E-16,-21.43125,32.940625));
#302675=CARTESIAN_POINT('',(-1.45809509523482E-16,-21.2328125,32.940625));
#302676=CARTESIAN_POINT('Origin',(0.,-21.43125,31.75));
#302677=CARTESIAN_POINT('Origin',(0.,132.185697587277,0.));
#302678=CARTESIAN_POINT('',(-6.76664131233047E-15,-21.43125,55.2538194444444));
#302679=CARTESIAN_POINT('Origin',(0.,-21.43125,0.));
#302680=CARTESIAN_POINT('',(-6.76664131233047E-15,16.66875,55.2538194444444));
#302681=CARTESIAN_POINT('',(-6.76664131233047E-15,132.185697587277,55.2538194444444));
#302682=CARTESIAN_POINT('Origin',(0.,16.66875,0.));
#302683=CARTESIAN_POINT('Origin',(1.50669826507598E-15,16.66875,0.));
#302684=CARTESIAN_POINT('',(-3.9516490262161E-15,-15.478125,-44.5707880434783));
#302685=CARTESIAN_POINT('Origin',(1.50669826507598E-15,-15.478125,0.));
#302686=CARTESIAN_POINT('',(-3.9516490262161E-15,2.03437500000001,-44.5707880434783));
#302687=CARTESIAN_POINT('',(-3.9516490262161E-15,16.66875,-44.5707880434783));
#302688=CARTESIAN_POINT('Origin',(1.50669826507598E-15,2.03437500000001,
0.));
#302689=CARTESIAN_POINT('Origin',(0.,-9.56874999999999,0.));
#302690=CARTESIAN_POINT('',(-22.4667164334275,2.03437500000001,0.));
#302691=CARTESIAN_POINT('Origin',(2.48195539786777E-18,2.03437500000001,
0.));
#302692=CARTESIAN_POINT('',(-5.54781797994763E-16,9.29993150981749,-16.8332621659243));
#302693=CARTESIAN_POINT('Origin',(1.13459982601988E-17,9.29993150981749,
0.));
#302694=CARTESIAN_POINT('Origin',(1.50669826507598E-15,16.271875,0.));
#302695=CARTESIAN_POINT('',(-3.9516490262161E-15,16.271875,-44.5707880434783));
#302696=CARTESIAN_POINT('Origin',(1.50669826507598E-15,16.271875,0.));
#302697=CARTESIAN_POINT('',(-4.00025219605726E-15,16.66875,-44.9676630434783));
#302698=CARTESIAN_POINT('Origin',(-4.00025219605726E-15,16.271875,-44.9676630434783));
#302699=CARTESIAN_POINT('Origin',(1.50669826507598E-15,16.66875,0.));
#302700=CARTESIAN_POINT('Origin',(1.50669826507598E-15,14.684375,0.));
#302701=CARTESIAN_POINT('',(-6.03384967835924E-16,15.08125,17.2301371659243));
#302702=CARTESIAN_POINT('Origin',(1.50669826507598E-15,15.08125,0.));
#302703=CARTESIAN_POINT('',(-5.54781797994763E-16,14.684375,16.8332621659243));
#302704=CARTESIAN_POINT('Origin',(-6.03384967835924E-16,14.684375,17.2301371659243));
#302705=CARTESIAN_POINT('',(3.56817832814672E-15,14.684375,-16.8332621659243));
#302706=CARTESIAN_POINT('Origin',(1.50669826507598E-15,14.684375,0.));
#302707=CARTESIAN_POINT('Origin',(1.50669826507598E-15,14.684375,0.));
#302708=CARTESIAN_POINT('Origin',(1.50669826507598E-15,16.66875,0.));
#302709=CARTESIAN_POINT('',(-5.54781797994763E-16,16.66875,-16.8332621659243));
#302710=CARTESIAN_POINT('Origin',(0.,15.71625,0.));
#302711=CARTESIAN_POINT('',(-5.38058221954622E-15,15.08125,-43.9357880434783));
#302712=CARTESIAN_POINT('Origin',(1.50669826507598E-15,15.08125,0.));
#302713=CARTESIAN_POINT('',(-5.45834729129208E-15,15.71625,-44.5707880434783));
#302714=CARTESIAN_POINT('Origin',(-5.38058221954622E-15,15.71625,-43.9357880434783));
#302715=CARTESIAN_POINT('Origin',(1.50669826507598E-15,15.71625,0.));
#302716=CARTESIAN_POINT('Origin',(1.50669826507598E-15,16.66875,0.));
#302717=CARTESIAN_POINT('',(-3.9516490262161E-15,16.66875,-44.5707880434783));
#302718=CARTESIAN_POINT('Origin',(0.,16.66875,0.));
#302719=CARTESIAN_POINT('Origin',(-43.9357880434783,15.08125,0.));
#302720=CARTESIAN_POINT('Origin',(-44.5707880434783,-15.478125,0.));
#302721=CARTESIAN_POINT('Origin',(-16.8332621659243,2.03437500000001,0.));
#302722=CARTESIAN_POINT('Origin',(0.,-21.2328125,31.75));
#302723=CARTESIAN_POINT('Origin',(22.4506403026729,-21.2328125,22.4506403026729));
#302724=CARTESIAN_POINT('Origin',(31.75,-21.2328125,1.73472347597681E-15));
#302725=CARTESIAN_POINT('Origin',(22.4506403026729,-21.2328125,-22.4506403026729));
#302726=CARTESIAN_POINT('Origin',(3.46944695195361E-15,-21.2328125,-31.75));
#302727=CARTESIAN_POINT('Origin',(-22.4506403026729,-21.2328125,-22.4506403026729));
#302728=CARTESIAN_POINT('Origin',(-31.75,-21.2328125,-6.93889390390723E-15));
#302729=CARTESIAN_POINT('Origin',(-22.4506403026729,-21.2328125,22.4506403026729));
#302730=CARTESIAN_POINT('Origin',(0.,-21.2328125,0.));
#302731=CARTESIAN_POINT('Origin',(0.,-21.43125,0.));
#310592=UNCERTAINTY_MEASURE_WITH_UNIT(LENGTH_MEASURE(0.01),#310624,
'DISTANCE_ACCURACY_VALUE',
'Maximum model space distance between geometric entities at asserted c
onnectivities');
#310601=UNCERTAINTY_MEASURE_WITH_UNIT(LENGTH_MEASURE(0.01),#310624,
'DISTANCE_ACCURACY_VALUE',
'Maximum model space distance between geometric entities at asserted c
onnectivities');
#310614=(
GEOMETRIC_REPRESENTATION_CONTEXT(3)
GLOBAL_UNCERTAINTY_ASSIGNED_CONTEXT((#310592))
GLOBAL_UNIT_ASSIGNED_CONTEXT((#310624,#310626,#310627))
REPRESENTATION_CONTEXT('','3D')
);
#310623=(
GEOMETRIC_REPRESENTATION_CONTEXT(3)
GLOBAL_UNCERTAINTY_ASSIGNED_CONTEXT((#310601))
GLOBAL_UNIT_ASSIGNED_CONTEXT((#310624,#310626,#310627))
REPRESENTATION_CONTEXT('','3D')
);
#310624=(
LENGTH_UNIT()
NAMED_UNIT(*)
SI_UNIT(.MILLI.,.METRE.)
);
#310626=(
NAMED_UNIT(*)
PLANE_ANGLE_UNIT()
SI_UNIT($,.RADIAN.)
);
#310627=(
NAMED_UNIT(*)
SI_UNIT($,.STERADIAN.)
SOLID_ANGLE_UNIT()
);
#310640=SHAPE_DEFINITION_REPRESENTATION(#310799,#310905);
#310799=PRODUCT_DEFINITION_SHAPE('',$,#310927);
#310905=SHAPE_REPRESENTATION('',(#104248),#310614);
#310914=PRODUCT_DEFINITION_CONTEXT('part definition',#310979,'design');
#310927=PRODUCT_DEFINITION('Base Anchor Foot','Base Anchor Foot',#310948,
#310914);
#310948=PRODUCT_DEFINITION_FORMATION('',$,#310993);
#310979=APPLICATION_CONTEXT(
'Core Data for Automotive Mechanical Design Process');
#310980=PRODUCT_CONTEXT('part definition',#310979,'mechanical');
#310993=PRODUCT('Base Anchor Foot','Base Anchor Foot',$,(#310980));
#311005=PRESENTATION_STYLE_ASSIGNMENT((#311012));
#311012=SURFACE_STYLE_USAGE(.BOTH.,#311019);
#311019=SURFACE_SIDE_STYLE('',(#311026));
#311026=SURFACE_STYLE_FILL_AREA(#311033);
#311033=FILL_AREA_STYLE('Opaque(20,51,87)',(#311040));
#311040=FILL_AREA_STYLE_COLOUR('Opaque(20,51,87)',#311047);
#311047=COLOUR_RGB('Opaque(20,51,87)',0.0784313725490196,0.2,0.341176470588235);
ENDSEC;
END-ISO-10303-21;
